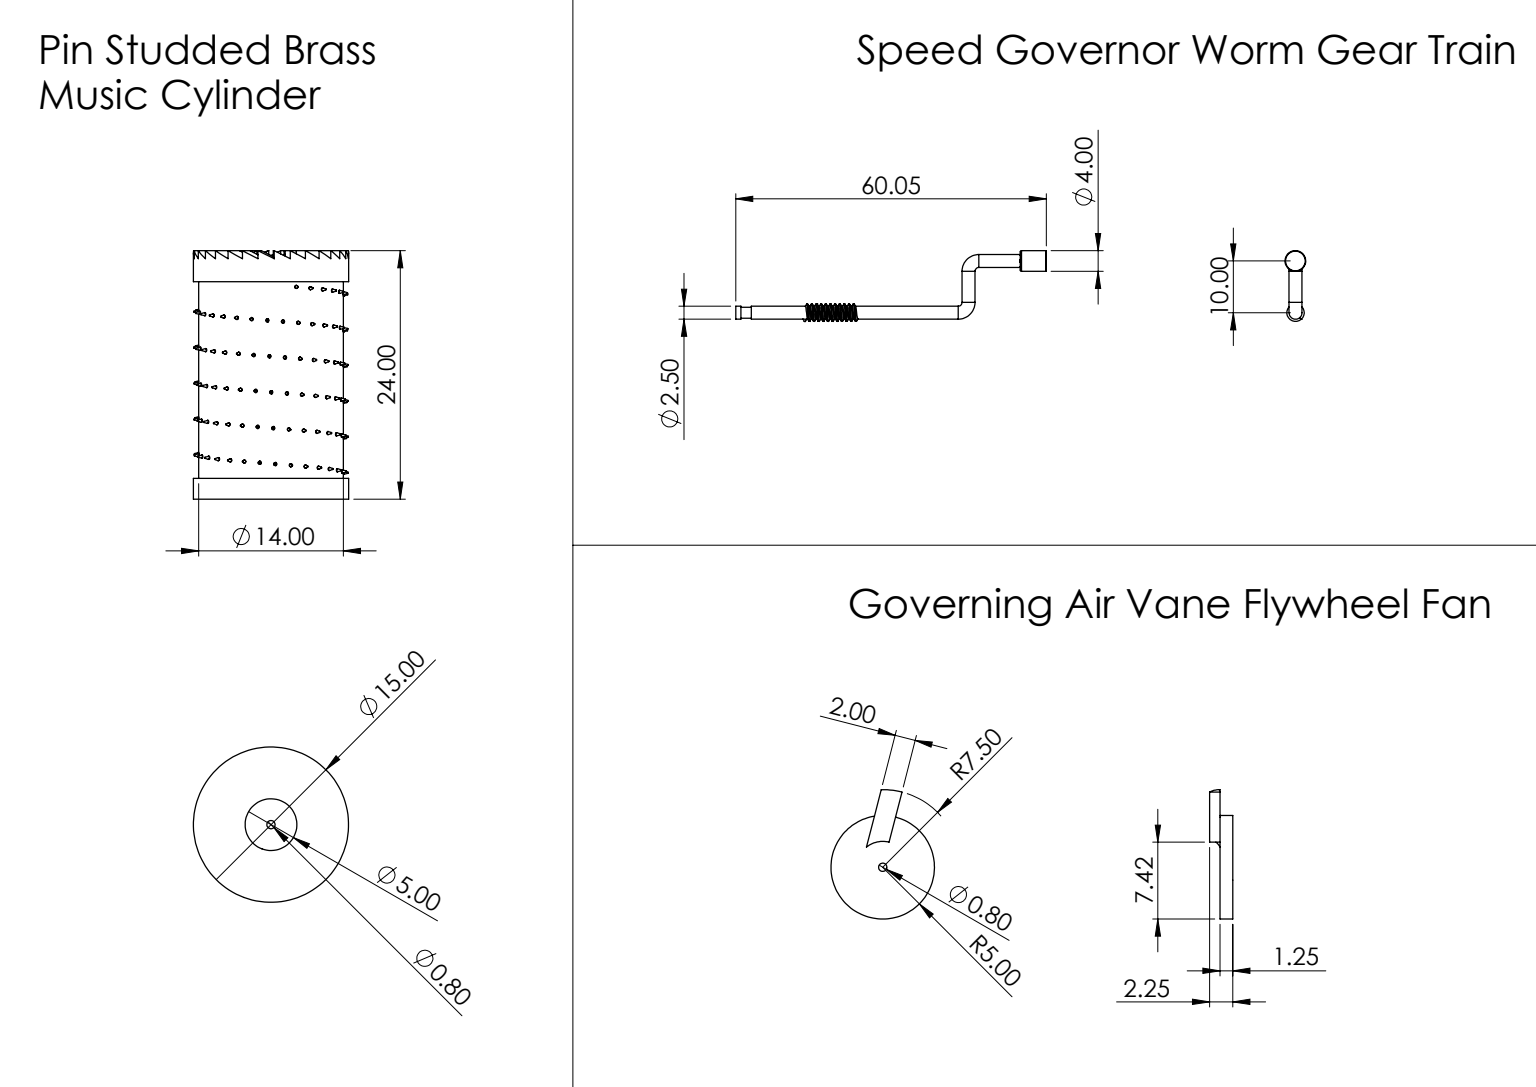
ISO-10303-21;
HEADER;
FILE_DESCRIPTION (('STEP AP214'),
    '1' );
FILE_NAME ('Pin Studded Brass Music Cylinder.step',
    '2026-10-09T09:51:18',
    ( '' ),
    ( '' ),
    'SwSTEP 2.0',
    'SolidWorks 2026',
    '' );
FILE_SCHEMA (( 'AUTOMOTIVE_DESIGN' ));
ENDSEC;

DATA;
#2=ADVANCED_FACE ( 'NONE', ( #22899 ), #34188, .F. ) ;
#3=CARTESIAN_POINT ( 'NONE',  ( -10.03625575236388201, -13.84871804469525891, 57.54850793716612856 ) ) ;
#4=CARTESIAN_POINT ( 'NONE',  ( -11.98370840013613225, -9.620047919863830899, 54.02312124697528617 ) ) ;
#8=ORIENTED_EDGE ( 'NONE', *, *, #40110, .F. ) ;
#9=CARTESIAN_POINT ( 'NONE',  ( -24.74075724160099554, -16.21284971877490122, 62.77824058731629009 ) ) ;
#10=CARTESIAN_POINT ( 'NONE',  ( -15.47038646904106685, -21.58309222549749506, 72.34575460768671462 ) ) ;
#11=CARTESIAN_POINT ( 'NONE',  ( -11.58081676984627073, -10.85831292256293068, 57.30083494179207548 ) ) ;
#13=EDGE_CURVE ( 'NONE', #13987, #23723, #5050, .T. ) ;
#14=VERTEX_POINT ( 'NONE', #21494 ) ;
#15=AXIS2_PLACEMENT_3D ( 'NONE', #40029, #47896, #25252 ) ;
#17=B_SPLINE_CURVE_WITH_KNOTS ( 'NONE', 3,
 ( #43534, #12980, #31711, #43034, #46503, #38613, #46737, #9313, #19907, #1178 ),
 .UNSPECIFIED., .F., .F.,
 ( 4, 2, 2, 2, 4 ),
 ( 0.1272669073658292960, 0.2522669073463885137, 0.3772669073268680728, 0.5022669073073477986, 0.6272669072878274132 ),
 .UNSPECIFIED. ) ;
#18=DIRECTION ( 'NONE',  ( 0.9939059412784551073, 0.1102314832132140626, 5.576311685107536405E-08 ) ) ;
#19=ORIENTED_EDGE ( 'NONE', *, *, #29500, .F. ) ;
#21=CARTESIAN_POINT ( 'NONE',  ( -10.31364510401727053, -17.03300888149450998, 57.80265138661536639 ) ) ;
#22=DIRECTION ( 'NONE',  ( -0.7107718805962432995, -0.7034225854731134264, -7.722840056494082694E-09 ) ) ;
#24=CARTESIAN_POINT ( 'NONE',  ( -21.68606299684865135, -9.256084799238676553, 66.66150029161380530 ) ) ;
#25=VERTEX_POINT ( 'NONE', #6474 ) ;
#26=PLANE ( 'NONE',  #30712 ) ;
#27=FACE_OUTER_BOUND ( 'NONE', #8967, .T. ) ;
#28=VERTEX_POINT ( 'NONE', #28867 ) ;
#30=CARTESIAN_POINT ( 'NONE',  ( -19.85891393954322837, -21.37210614461000091, 75.49999999999994316 ) ) ;
#32=CARTESIAN_POINT ( 'NONE',  ( -20.17268404433175633, -8.371407854712250796, 70.55100341248845552 ) ) ;
#34=CARTESIAN_POINT ( 'NONE',  ( -10.76587051450098542, -16.97017341121004463, 57.68760522235623966 ) ) ;
#36=CARTESIAN_POINT ( 'NONE',  ( -14.44705700679302574, -7.979876293330282699, 63.93978841086359211 ) ) ;
#37=ORIENTED_EDGE ( 'NONE', *, *, #6492, .T. ) ;
#40=LINE ( 'NONE', #15026, #36087 ) ;
#41=DIRECTION ( 'NONE',  ( -0.9942595023566571655, 0.1069955231469581908, -3.800058679842194246E-08 ) ) ;
#43=LINE ( 'NONE', #45603, #5826 ) ;
#46=AXIS2_PLACEMENT_3D ( 'NONE', #24798, #28249, #13682 ) ;
#47=CARTESIAN_POINT ( 'NONE',  ( -16.84904657224188540, -21.78683024590906925, 72.39373074617707005 ) ) ;
#48=CARTESIAN_POINT ( 'NONE',  ( -13.27770768808251134, -9.107454094634595876, 63.90946529206384241 ) ) ;
#50=CARTESIAN_POINT ( 'NONE',  ( -24.00746423591236933, -17.19188279365308603, 73.11165851276361138 ) ) ;
#51=CARTESIAN_POINT ( 'NONE',  ( -24.18314854330451169, -12.98801962294919932, 66.30246782466414857 ) ) ;
#52=CARTESIAN_POINT ( 'NONE',  ( -11.64944166978149909, -18.76574910929434736, 64.81995021385422717 ) ) ;
#53=CARTESIAN_POINT ( 'NONE',  ( -24.72694767484942702, -16.28301260341204326, 62.70833288210281609 ) ) ;
#54=DIRECTION ( 'NONE',  ( 0.5088156898428700670, 0.8608754809899750171, 5.922709712265242817E-08 ) ) ;
#55=CARTESIAN_POINT ( 'NONE',  ( -19.57699614054808634, -21.94144247634149281, 62.17999043330664222 ) ) ;
#57=CARTESIAN_POINT ( 'NONE',  ( -12.74071866071660075, -9.015263582886822391, 70.96429948631303830 ) ) ;
#58=DIRECTION ( 'NONE',  ( 0.5088156898428700670, 0.8608754809899751281, 5.922709712265243479E-08 ) ) ;
#59=CARTESIAN_POINT ( 'NONE',  ( -10.02934067034867915, -15.71522136325494579, 61.14450729704604015 ) ) ;
#60=ORIENTED_EDGE ( 'NONE', *, *, #2656, .T. ) ;
#61=CARTESIAN_POINT ( 'NONE',  ( -10.21764062494887781, -12.91954801228597915, 67.92327636273336111 ) ) ;
#63=VECTOR ( 'NONE', #41726, 1000.000000000000114 ) ;
#67=CARTESIAN_POINT ( 'NONE',  ( -11.89176969907138570, -10.51836715134331079, 74.66715118432504994 ) ) ;
#69=ORIENTED_EDGE ( 'NONE', *, *, #36924, .F. ) ;
#72=EDGE_CURVE ( 'NONE', #44245, #17093, #1589, .T. ) ;
#74=FACE_OUTER_BOUND ( 'NONE', #13777, .T. ) ;
#75=AXIS2_PLACEMENT_3D ( 'NONE', #46607, #16288, #28114 ) ;
#77=CYLINDRICAL_SURFACE ( 'NONE', #4036, 0.1500000000000066835 ) ;
#79=B_SPLINE_CURVE_WITH_KNOTS ( 'NONE', 1,
 ( #16390, #46203 ),
 .UNSPECIFIED., .F., .F.,
 ( 2, 2 ),
 ( 0.000000000000000000, 1.000000000000000000 ),
 .UNSPECIFIED. ) ;
#81=DIRECTION ( 'NONE',  ( 3.549360974555109863E-17, 1.977132801529350715E-16, 1.000000000000000000 ) ) ;
#82=CARTESIAN_POINT ( 'NONE',  ( -18.31357640787765817, -21.80286941108919763, 68.81514702304139064 ) ) ;
#85=PLANE ( 'NONE',  #90 ) ;
#86=CARTESIAN_POINT ( 'NONE',  ( -24.16097951573440383, -12.71927508598556322, 66.51066513624088827 ) ) ;
#87=ORIENTED_EDGE ( 'NONE', *, *, #46598, .F. ) ;
#88=CARTESIAN_POINT ( 'NONE',  ( -22.33685117127641817, -20.40992557423668430, 62.42777465437541196 ) ) ;
#89=EDGE_CURVE ( 'NONE', #5768, #15899, #14150, .T. ) ;
#90=AXIS2_PLACEMENT_3D ( 'NONE', #14327, #11160, #7719 ) ;
#91=CARTESIAN_POINT ( 'NONE',  ( -13.88293259567353743, -20.90532631576516565, 68.45625136994867432 ) ) ;
#92=EDGE_CURVE ( 'NONE', #20698, #38947, #146, .T. ) ;
#95=CARTESIAN_POINT ( 'NONE',  ( -10.02191625022346955, -15.65273779443635327, 61.15293638507743168 ) ) ;
#98=CARTESIAN_POINT ( 'NONE',  ( -10.46033444208452501, -13.68630826424936231, 57.74825279763368968 ) ) ;
#101=CARTESIAN_POINT ( 'NONE',  ( -11.81042834955647258, -10.54382735031610174, 74.45357240259568243 ) ) ;
#103=EDGE_LOOP ( 'NONE', ( #13179, #38410, #7478, #14746, #26186 ) ) ;
#104=CARTESIAN_POINT ( 'NONE',  ( -9.980660856333416930, -14.49625842079804272, 68.05788908589504160 ) ) ;
#106=CARTESIAN_POINT ( 'NONE',  ( -11.75774202113761113, -19.00384077433692909, 71.83685884782747166 ) ) ;
#107=CARTESIAN_POINT ( 'NONE',  ( -18.72484419698154667, -9.451406241145487996, 53.88362224778186516 ) ) ;
#108=CARTESIAN_POINT ( 'NONE',  ( -16.15310590563917970, -7.468295795601643583, 60.37745339520409971 ) ) ;
#109=CARTESIAN_POINT ( 'NONE',  ( -10.49291302059963193, -15.78914242734984263, 64.80771630040662501 ) ) ;
#111=AXIS2_PLACEMENT_3D ( 'NONE', #10985, #396, #26489 ) ;
#113=CARTESIAN_POINT ( 'NONE',  ( -16.59261295876471820, -7.800382739013279831, 60.34461612587266899 ) ) ;
#114=CARTESIAN_POINT ( 'NONE',  ( -14.54391382047218784, -7.937654553327920581, 63.97634087063163122 ) ) ;
#117=DIRECTION ( 'NONE',  ( 3.549360974554993999E-17, -6.371834667797928663E-18, -1.000000000000000000 ) ) ;
#119=( BOUNDED_CURVE ( )  B_SPLINE_CURVE ( 3, ( #27341, #33989, #3973, #288 ),
 .UNSPECIFIED., .F., .F. ) 
 B_SPLINE_CURVE_WITH_KNOTS ( ( 4, 4 ),
 ( 0.000000000000000000, 0.4074455897393676196 ),
 .UNSPECIFIED. ) 
 CURVE ( )  GEOMETRIC_REPRESENTATION_ITEM ( )  RATIONAL_B_SPLINE_CURVE ( ( 1.000000000000000000, 0.4567392136813337444, 0.3561768502900309330, 0.6983129098260915102 ) ) 
 REPRESENTATION_ITEM ( '' )  );
#120=ORIENTED_EDGE ( 'NONE', *, *, #48681, .F. ) ;
#121=( BOUNDED_SURFACE ( )  B_SPLINE_SURFACE ( 3, 1, ( 
 ( #32470, #2427 ),
 ( #20663, #20424 ),
 ( #39116, #24112 ),
 ( #35421, #5884 ),
 ( #1706, #35896 ),
 ( #28292, #43320 ),
 ( #17438, #47493 ) ),
 .UNSPECIFIED., .T., .F., .F. ) 
 B_SPLINE_SURFACE_WITH_KNOTS ( ( 4, 3, 4 ),
 ( 2, 2 ),
 ( 0.000000000000000000, 0.5000000000000000000, 1.000000000000000000 ),
 ( 0.000000000000000000, 1.000000000000000000 ),
 .UNSPECIFIED. ) 
 GEOMETRIC_REPRESENTATION_ITEM ( )  RATIONAL_B_SPLINE_SURFACE ( (
 ( 1.000000000000000000, 1.000000000000000000),
 ( 0.3333333333333335369, 0.3333333333333330373),
 ( 0.3333333333333335369, 0.3333333333333330373),
 ( 1.000000000000000000, 1.000000000000000000),
 ( 0.3333333333333333703, 0.3333333333333333703),
 ( 0.3333333333333333703, 0.3333333333333333703),
 ( 1.000000000000000000, 1.000000000000000000) ) ) 
 REPRESENTATION_ITEM ( '' )  SURFACE ( )  );
#122=DIRECTION ( 'NONE',  ( 0.06306825763707678278, -0.9980092158285026605, -2.415158932408153704E-08 ) ) ;
#125=EDGE_LOOP ( 'NONE', ( #26058, #18123, #34416, #18514, #29920 ) ) ;
#128=CARTESIAN_POINT ( 'NONE',  ( -14.34311167289324196, -8.523215816031258996, 71.01341051612104138 ) ) ;
#133=( BOUNDED_CURVE ( )  B_SPLINE_CURVE ( 3, ( #21288, #36284, #8992, #43458 ),
 .UNSPECIFIED., .F., .F. ) 
 B_SPLINE_CURVE_WITH_KNOTS ( ( 4, 4 ),
 ( 0.000000000000000000, 0.4074455897393643999 ),
 .UNSPECIFIED. ) 
 CURVE ( )  GEOMETRIC_REPRESENTATION_ITEM ( )  RATIONAL_B_SPLINE_CURVE ( ( 1.000000000000000000, 0.4567392136813379078, 0.3561768502900324873, 0.6983129098260837386 ) ) 
 REPRESENTATION_ITEM ( '' )  );
#134=ORIENTED_EDGE ( 'NONE', *, *, #4016, .F. ) ;
#137=ADVANCED_FACE ( 'NONE', ( #48154 ), #33338, .T. ) ;
#138=B_SPLINE_CURVE_WITH_KNOTS ( 'NONE', 1,
 ( #27125, #38191 ),
 .UNSPECIFIED., .F., .F.,
 ( 2, 2 ),
 ( 0.000000000000000000, 1.000000000000000000 ),
 .UNSPECIFIED. ) ;
#139=CARTESIAN_POINT ( 'NONE',  ( -10.44538189632046787, -14.26369805489357212, 61.02707267863189600 ) ) ;
#143=ORIENTED_EDGE ( 'NONE', *, *, #11819, .T. ) ;
#144=CARTESIAN_POINT ( 'NONE',  ( -15.46105799208929454, -21.99670631207736449, 72.15920124769014876 ) ) ;
#146=B_SPLINE_CURVE_WITH_KNOTS ( 'NONE', 3,
 ( #35431, #29443, #1718, #7046, #39128, #9108, #29205, #44244, #25744, #48389 ),
 .UNSPECIFIED., .F., .F.,
 ( 4, 2, 2, 2, 4 ),
 ( 0.000000000000000000, 0.2500000000000000000, 0.5000000000000000000, 0.7500000000000000000, 1.000000000000000000 ),
 .UNSPECIFIED. ) ;
#147=CARTESIAN_POINT ( 'NONE',  ( -23.80321451250838649, -17.81075939459467961, 59.00378417737415049 ) ) ;
#148=EDGE_LOOP ( 'NONE', ( #25559, #28549, #5036, #6443 ) ) ;
#149=DIRECTION ( 'NONE',  ( 0.3478314405900310158, 0.9375570856950865561, -9.567072274253695189E-17 ) ) ;
#150=EDGE_CURVE ( 'NONE', #31901, #23884, #35863, .T. ) ;
#153=CARTESIAN_POINT ( 'NONE',  ( -21.39967327233876304, -20.63170314183283693, 72.80974286114339122 ) ) ;
#154=CARTESIAN_POINT ( 'NONE',  ( -24.83423444544265379, -14.03910623769390220, 73.31609816701728732 ) ) ;
#157=ADVANCED_FACE ( 'NONE', ( #22300 ), #19091, .T. ) ;
#158=CARTESIAN_POINT ( 'NONE',  ( -11.08846142298070880, -18.82290330472913098, 53.49999999999994316 ) ) ;
#160=VECTOR ( 'NONE', #789, 1000.000000000000227 ) ;
#161=ORIENTED_EDGE ( 'NONE', *, *, #28229, .T. ) ;
#162=CARTESIAN_POINT ( 'NONE',  ( -10.40121522062585591, -17.29573862802152817, 61.20097198354311274 ) ) ;
#163=CARTESIAN_POINT ( 'NONE',  ( -24.09124995986085338, -12.51712822272146042, 73.53665784698486618 ) ) ;
#164=CARTESIAN_POINT ( 'NONE',  ( -23.56138404952065457, -11.33988834032952830, 70.19210750372964469 ) ) ;
#165=CYLINDRICAL_SURFACE ( 'NONE', #41008, 0.1500000000000034084 ) ;
#166=VERTEX_POINT ( 'NONE', #48638 ) ;
#168=CARTESIAN_POINT ( 'NONE',  ( -13.14998806103231566, -9.265559761403904915, 67.67942786032521951 ) ) ;
#170=FACE_BOUND ( 'NONE', #41683, .T. ) ;
#171=ORIENTED_EDGE ( 'NONE', *, *, #31245, .F. ) ;
#173=CARTESIAN_POINT ( 'NONE',  ( -15.68784259522275981, -9.576290808195315307, 53.69233794759168887 ) ) ;
#174=CARTESIAN_POINT ( 'NONE',  ( -9.939267784769082681, -14.33236412611010913, 54.27966884056655061 ) ) ;
#175=CARTESIAN_POINT ( 'NONE',  ( -21.55884032038934350, -8.611816057827914150, 73.78624026056009200 ) ) ;
#178=ORIENTED_EDGE ( 'NONE', *, *, #7182, .F. ) ;
#179=CARTESIAN_POINT ( 'NONE',  ( -12.18170095131842068, -10.17053037870675780, 64.02914326641410980 ) ) ;
#181=B_SPLINE_CURVE_WITH_KNOTS ( 'NONE', 1,
 ( #24932, #10158 ),
 .UNSPECIFIED., .F., .F.,
 ( 2, 2 ),
 ( 0.000000000000000000, 1.000000000000000000 ),
 .UNSPECIFIED. ) ;
#183=ORIENTED_EDGE ( 'NONE', *, *, #25838, .F. ) ;
#188=VERTEX_POINT ( 'NONE', #389 ) ;
#189=CARTESIAN_POINT ( 'NONE',  ( -15.39235221195410652, -21.97689038623625635, 72.08929527613493349 ) ) ;
#190=FACE_OUTER_BOUND ( 'NONE', #18555, .T. ) ;
#191=CARTESIAN_POINT ( 'NONE',  ( -24.42668993457695592, -13.99045928592870780, 73.40799407547365263 ) ) ;
#192=CARTESIAN_POINT ( 'NONE',  ( -11.32469211327616065, -18.34471187850051166, 57.95714594245092854 ) ) ;
#193=FACE_OUTER_BOUND ( 'NONE', #16201, .T. ) ;
#194=CARTESIAN_POINT ( 'NONE',  ( -14.55015457993596328, -8.362855509585410019, 70.87390454733632339 ) ) ;
#195=CARTESIAN_POINT ( 'NONE',  ( -15.34465393633500518, -21.54586957516256263, 68.86120835375241711 ) ) ;
#196=EDGE_LOOP ( 'NONE', ( #10385, #20529 ) ) ;
#197=ORIENTED_EDGE ( 'NONE', *, *, #3825, .F. ) ;
#198=CARTESIAN_POINT ( 'NONE',  ( -16.19792114999740562, -7.866354181730329742, 60.48556343814865954 ) ) ;
#199=B_SPLINE_CURVE_WITH_KNOTS ( 'NONE', 3,
 ( #36213, #17003, #17258, #47556, #32053, #25388, #10127, #47073, #46828, #2496 ),
 .UNSPECIFIED., .F., .F.,
 ( 4, 2, 2, 2, 4 ),
 ( 0.000000000000000000, 0.2500000000000000000, 0.5000000000000000000, 0.7500000000000000000, 1.000000000000000000 ),
 .UNSPECIFIED. ) ;
#201=EDGE_CURVE ( 'NONE', #20782, #44291, #26002, .T. ) ;
#202=CARTESIAN_POINT ( 'NONE',  ( -22.54212894027171643, -20.22308674935842276, 65.88138641420671604 ) ) ;
#204=CARTESIAN_POINT ( 'NONE',  ( -21.56183007311343758, -9.162502203718322136, 70.41516033260253948 ) ) ;
#207=ORIENTED_EDGE ( 'NONE', *, *, #41740, .T. ) ;
#210=DIRECTION ( 'NONE',  ( 0.2196488028684550897, 0.9755790093059856227, -7.835600157377411709E-08 ) ) ;
#211=( BOUNDED_SURFACE ( )  B_SPLINE_SURFACE ( 3, 1, ( 
 ( #3331, #29681 ),
 ( #37286, #39375 ),
 ( #13247, #28301 ),
 ( #9599, #24612 ),
 ( #39614, #20905 ),
 ( #29932, #18842 ),
 ( #11449, #11220 ) ),
 .UNSPECIFIED., .T., .F., .F. ) 
 B_SPLINE_SURFACE_WITH_KNOTS ( ( 4, 3, 4 ),
 ( 2, 2 ),
 ( 0.000000000000000000, 0.5000000000000000000, 1.000000000000000000 ),
 ( 0.000000000000000000, 1.000000000000000000 ),
 .UNSPECIFIED. ) 
 GEOMETRIC_REPRESENTATION_ITEM ( )  RATIONAL_B_SPLINE_SURFACE ( (
 ( 1.000000000000000000, 1.000000000000000000),
 ( 0.3333333333333335369, 0.3333333333333330373),
 ( 0.3333333333333335369, 0.3333333333333330373),
 ( 1.000000000000000000, 1.000000000000000000),
 ( 0.3333333333333333703, 0.3333333333333333703),
 ( 0.3333333333333333703, 0.3333333333333333703),
 ( 1.000000000000000000, 1.000000000000000000) ) ) 
 REPRESENTATION_ITEM ( '' )  SURFACE ( )  );
#212=ORIENTED_EDGE ( 'NONE', *, *, #4432, .T. ) ;
#213=B_SPLINE_CURVE_WITH_KNOTS ( 'NONE', 1,
 ( #33678, #3925 ),
 .UNSPECIFIED., .F., .F.,
 ( 2, 2 ),
 ( 0.000000000000000000, 1.000000000000000000 ),
 .UNSPECIFIED. ) ;
#214=CYLINDRICAL_SURFACE ( 'NONE', #2262, 0.1500000000000026867 ) ;
#215=CARTESIAN_POINT ( 'NONE',  ( -10.49912617938483628, -17.55847672437320028, 64.74084113084838066 ) ) ;
#216=EDGE_CURVE ( 'NONE', #42645, #18548, #11212, .T. ) ;
#218=EDGE_LOOP ( 'NONE', ( #34553, #46126, #27909, #171, #16080 ) ) ;
#219=DIRECTION ( 'NONE',  ( -0.03181436478788690625, -0.9994937949748078365, -6.982004198809110323E-09 ) ) ;
#220=CARTESIAN_POINT ( 'NONE',  ( -10.13411916705081950, -16.34564720852668884, 71.62467237673240561 ) ) ;
#221=CARTESIAN_POINT ( 'NONE',  ( -9.974215857974789046, -14.86484893678357544, 74.91283499353951925 ) ) ;
#223=CARTESIAN_POINT ( 'NONE',  ( -24.67958393122153282, -16.50120980550295613, 59.26299101463538221 ) ) ;
#225=CARTESIAN_POINT ( 'NONE',  ( -10.33531725737393181, -17.10115422170377641, 57.87255955594724810 ) ) ;
#227=EDGE_CURVE ( 'NONE', #31196, #14322, #2991, .T. ) ;
#228=DIRECTION ( 'NONE',  ( -0.8743548079231423520, -0.4852872034802501178, 5.778319183281970132E-08 ) ) ;
#230=CARTESIAN_POINT ( 'NONE',  ( -23.84087120742880117, -12.00869232914290841, 59.55405921996587892 ) ) ;
#231=EDGE_CURVE ( 'NONE', #5198, #11939, #41252, .T. ) ;
#232=CARTESIAN_POINT ( 'NONE',  ( -20.59081119662036485, -8.510278447070987795, 63.31681297810601450 ) ) ;
#234=CARTESIAN_POINT ( 'NONE',  ( -17.85728874018076340, -21.84618329174708151, 61.89007996730683203 ) ) ;
#235=CARTESIAN_POINT ( 'NONE',  ( -22.25933006198147623, -19.87095799428289666, 65.71924198175659626 ) ) ;
#236=LINE ( 'NONE', #3923, #40839 ) ;
#238=CARTESIAN_POINT ( 'NONE',  ( -24.03160980685186487, -17.26750534774173929, 69.41339792588560442 ) ) ;
#239=CARTESIAN_POINT ( 'NONE',  ( -20.81693178527791943, -20.99322608020143477, 65.67634157851000509 ) ) ;
#240=EDGE_CURVE ( 'NONE', #21614, #9195, #13538, .T. ) ;
#243=CARTESIAN_POINT ( 'NONE',  ( -10.49020387924836761, -15.76942919235743013, 61.26462351667871076 ) ) ;
#245=CARTESIAN_POINT ( 'NONE',  ( -19.86569447268030686, -19.73755174630646536, 54.07175714974878389 ) ) ;
#248=CARTESIAN_POINT ( 'NONE',  ( -24.42668993457695592, -13.99045928592870958, 73.40799407547365263 ) ) ;
#249=CARTESIAN_POINT ( 'NONE',  ( -11.10300703817161327, -10.86615712478015539, 57.39398594787093089 ) ) ;
#250=CARTESIAN_POINT ( 'NONE',  ( -20.50783493979771421, -8.027295371342848540, 66.96599508560271374 ) ) ;
#251=CARTESIAN_POINT ( 'NONE',  ( -9.974485213446937948, -14.88680260109476805, 74.89804658166208640 ) ) ;
#253=B_SPLINE_CURVE_WITH_KNOTS ( 'NONE', 3,
 ( #32293, #44346, #6180, #32750, #21450, #2715, #14493, #36434, #43618, #13547 ),
 .UNSPECIFIED., .F., .F.,
 ( 4, 2, 2, 2, 4 ),
 ( 0.6272669072877669061, 0.7522669073072844048, 0.8772669073268017925, 1.002266907346319291, 1.127266907365836790 ),
 .UNSPECIFIED. ) ;
#254=DIRECTION ( 'NONE',  ( -0.5022914217388750879, 0.8646984027090224290, 6.766381827299039861E-08 ) ) ;
#255=VECTOR ( 'NONE', #23047, 1000.000000000000000 ) ;
#256=CARTESIAN_POINT ( 'NONE',  ( -10.44916039635137039, -15.83526825291551177, 64.50771589744864798 ) ) ;
#257=FACE_OUTER_BOUND ( 'NONE', #41727, .T. ) ;
#258=( BOUNDED_SURFACE ( )  B_SPLINE_SURFACE ( 3, 1, ( 
 ( #12645, #30891 ),
 ( #19547, #27669 ),
 ( #35286, #42701 ),
 ( #8965, #19806 ),
 ( #23985, #34558 ),
 ( #34807, #16808 ),
 ( #38986, #27907 ) ),
 .UNSPECIFIED., .T., .F., .F. ) 
 B_SPLINE_SURFACE_WITH_KNOTS ( ( 4, 3, 4 ),
 ( 2, 2 ),
 ( 0.000000000000000000, 0.5000000000000000000, 1.000000000000000000 ),
 ( 0.000000000000000000, 1.000000000000000000 ),
 .UNSPECIFIED. ) 
 GEOMETRIC_REPRESENTATION_ITEM ( )  RATIONAL_B_SPLINE_SURFACE ( (
 ( 1.000000000000000000, 1.000000000000000000),
 ( 0.3333333333333335369, 0.3333333333333330373),
 ( 0.3333333333333335369, 0.3333333333333330373),
 ( 1.000000000000000000, 1.000000000000000000),
 ( 0.3333333333333333703, 0.3333333333333333703),
 ( 0.3333333333333333703, 0.3333333333333333703),
 ( 1.000000000000000000, 1.000000000000000000) ) ) 
 REPRESENTATION_ITEM ( '' )  SURFACE ( )  );
#259=EDGE_LOOP ( 'NONE', ( #11996, #26220, #36249, #37738, #32112 ) ) ;
#260=VERTEX_POINT ( 'NONE', #11960 ) ;
#263=DIRECTION ( 'NONE',  ( 0.8398192074808117358, 0.5428661886195298436, 7.907900705247678986E-08 ) ) ;
#264=FACE_OUTER_BOUND ( 'NONE', #3313, .T. ) ;
#265=ADVANCED_FACE ( 'NONE', ( #8266 ), #28714, .T. ) ;
#266=EDGE_LOOP ( 'NONE', ( #5129, #25117, #30541, #44712, #25689 ) ) ;
#267=( BOUNDED_SURFACE ( )  B_SPLINE_SURFACE ( 3, 1, ( 
 ( #4799, #23276 ),
 ( #30184, #27440 ),
 ( #41983, #42225 ),
 ( #11696, #4317 ),
 ( #23767, #8256 ),
 ( #38762, #38256 ),
 ( #19824, #20056 ) ),
 .UNSPECIFIED., .T., .F., .F. ) 
 B_SPLINE_SURFACE_WITH_KNOTS ( ( 4, 3, 4 ),
 ( 2, 2 ),
 ( 0.000000000000000000, 0.5000000000000000000, 1.000000000000000000 ),
 ( 0.000000000000000000, 1.000000000000000000 ),
 .UNSPECIFIED. ) 
 GEOMETRIC_REPRESENTATION_ITEM ( )  RATIONAL_B_SPLINE_SURFACE ( (
 ( 1.000000000000000000, 1.000000000000000000),
 ( 0.3333333333333335369, 0.3333333333333330373),
 ( 0.3333333333333335369, 0.3333333333333330373),
 ( 1.000000000000000000, 1.000000000000000000),
 ( 0.3333333333333333703, 0.3333333333333333703),
 ( 0.3333333333333333703, 0.3333333333333333703),
 ( 1.000000000000000000, 1.000000000000000000) ) ) 
 REPRESENTATION_ITEM ( '' )  SURFACE ( )  );
#268=CARTESIAN_POINT ( 'NONE',  ( -23.54782545260626136, -11.41793123268749532, 66.49502567849339130 ) ) ;
#269=CARTESIAN_POINT ( 'NONE',  ( -14.16114181629738589, -8.110937519819053421, 67.37319822901852717 ) ) ;
#270=EDGE_CURVE ( 'NONE', #48679, #8571, #43948, .T. ) ;
#272=CARTESIAN_POINT ( 'NONE',  ( -22.79960313759534074, -9.650943445293346912, 73.66656413195866548 ) ) ;
#273=CARTESIAN_POINT ( 'NONE',  ( -10.88209246082447912, -17.29963176008448400, 64.92739380462948873 ) ) ;
#274=ORIENTED_EDGE ( 'NONE', *, *, #1986, .F. ) ;
#275=CARTESIAN_POINT ( 'NONE',  ( -17.53144753494939323, -7.808750373834428160, 67.24869371032770005 ) ) ;
#276=ORIENTED_EDGE ( 'NONE', *, *, #38105, .F. ) ;
#277=ADVANCED_FACE ( 'NONE', ( #22486 ), #33722, .T. ) ;
#278=CARTESIAN_POINT ( 'NONE',  ( -22.73317970229575025, -20.03675580610048712, 72.83055794290764595 ) ) ;
#279=CARTESIAN_POINT ( 'NONE',  ( -11.10386160987148862, -10.86480171160796893, 57.25257256893876701 ) ) ;
#280=ORIENTED_EDGE ( 'NONE', *, *, #26061, .T. ) ;
#282=CARTESIAN_POINT ( 'NONE',  ( -10.40830226666251157, -14.07974499963562920, 64.47983968490285633 ) ) ;
#283=ADVANCED_FACE ( 'NONE', ( #26188 ), #36999, .T. ) ;
#285=CARTESIAN_POINT ( 'NONE',  ( -10.37840828709523322, -12.38598989307629061, 60.98508858522948373 ) ) ;
#287=PLANE ( 'NONE',  #36864 ) ;
#288=CARTESIAN_POINT ( 'NONE',  ( -10.48067290732983281, -16.03043740265091444, 67.97767830707738312 ) ) ;
#290=ORIENTED_EDGE ( 'NONE', *, *, #4920, .T. ) ;
#292=CARTESIAN_POINT ( 'NONE',  ( -13.12613471901881113, -20.89454346209081947, 58.16154795605982031 ) ) ;
#293=CARTESIAN_POINT ( 'NONE',  ( -23.48344415125163565, -18.41350569598871090, 73.04896097104848707 ) ) ;
#295=CARTESIAN_POINT ( 'NONE',  ( -24.20309392561631512, -13.06392267828124432, 63.11798765125330135 ) ) ;
#298=CARTESIAN_POINT ( 'NONE',  ( -16.94342153774571713, -21.79279417793566154, 72.16543237156788848 ) ) ;
#299=DIRECTION ( 'NONE',  ( 0.3636930986378153485, 0.9315188296557532777, -1.850371886801397451E-09 ) ) ;
#300=VERTEX_POINT ( 'NONE', #7486 ) ;
#301=CARTESIAN_POINT ( 'NONE',  ( -10.40860991809309155, -15.50898095412354571, 57.85320721669017985 ) ) ;
#302=CARTESIAN_POINT ( 'NONE',  ( -14.96339028783852676, -21.42433367428847291, 68.72025781230657060 ) ) ;
#303=CARTESIAN_POINT ( 'NONE',  ( -15.53265176333180619, -21.60105060138385014, 72.33103357390284316 ) ) ;
#304=CARTESIAN_POINT ( 'NONE',  ( -17.20139284005516700, -7.812749994621428051, 70.79035839633094440 ) ) ;
#305=EDGE_CURVE ( 'NONE', #24134, #2153, #45318, .T. ) ;
#306=CARTESIAN_POINT ( 'NONE',  ( -21.54495561387301450, -21.01579894740183363, 72.63172296156072605 ) ) ;
#308=CARTESIAN_POINT ( 'NONE',  ( -24.64621740481133116, -16.83181165628401033, 53.49999999999994316 ) ) ;
#311=DIRECTION ( 'NONE',  ( 0.9000732436326450703, 0.4357386327795698677, -2.072980810833656879E-08 ) ) ;
#313=VERTEX_POINT ( 'NONE', #41198 ) ;
#314=ORIENTED_EDGE ( 'NONE', *, *, #26794, .T. ) ;
#317=FACE_OUTER_BOUND ( 'NONE', #17345, .T. ) ;
#319=CARTESIAN_POINT ( 'NONE',  ( -14.41428173599358331, -7.994163662063686893, 63.97474278339937115 ) ) ;
#320=EDGE_CURVE ( 'NONE', #35558, #5311, #25190, .T. ) ;
#321=CARTESIAN_POINT ( 'NONE',  ( -13.54823245630065998, -20.69819609872913801, 61.81646323537676579 ) ) ;
#322=CARTESIAN_POINT ( 'NONE',  ( -16.10183008998876275, -22.14097689426727911, 58.47923897578370145 ) ) ;
#324=CARTESIAN_POINT ( 'NONE',  ( -15.94298218261998912, -7.507746547262916792, 63.83044349608796608 ) ) ;
#325=DIRECTION ( 'NONE',  ( -5.255974128148611414E-06, 1.684062796621483993E-06, 0.9999999999847694054 ) ) ;
#327=CARTESIAN_POINT ( 'NONE',  ( -11.49500183448702906, -10.99442376238782515, 57.22375354680192316 ) ) ;
#328=CARTESIAN_POINT ( 'NONE',  ( -23.97105477456146261, -17.28687578273886061, 69.41339789080815592 ) ) ;
#329=EDGE_LOOP ( 'NONE', ( #13838, #9851, #9267, #15936, #24444 ) ) ;
#330=CARTESIAN_POINT ( 'NONE',  ( -11.12758687547136383, -10.82717111148205547, 57.40914419403284086 ) ) ;
#331=CARTESIAN_POINT ( 'NONE',  ( -21.30368986256526043, -21.17021271237730318, 69.24105570176159574 ) ) ;
#332=B_SPLINE_CURVE_WITH_KNOTS ( 'NONE', 3,
 ( #32504, #47759, #36419, #3183, #39890, #36180, #13765, #28808, #48006, #29048 ),
 .UNSPECIFIED., .F., .F.,
 ( 4, 2, 2, 2, 4 ),
 ( 0.1272669073658393157, 0.2522669073463362222, 0.3772669073268331008, 0.5022669073073300350, 0.6272669072878269692 ),
 .UNSPECIFIED. ) ;
#334=ORIENTED_EDGE ( 'NONE', *, *, #2116, .T. ) ;
#335=CARTESIAN_POINT ( 'NONE',  ( -19.71243508403738076, -21.42506817177905631, 69.21865898670732520 ) ) ;
#336=EDGE_CURVE ( 'NONE', #12470, #9257, #14096, .T. ) ;
#337=CARTESIAN_POINT ( 'NONE',  ( -23.00442008925061899, -19.11762375203660724, 59.18410642057862248 ) ) ;
#338=ADVANCED_FACE ( 'NONE', ( #40464 ), #45710, .T. ) ;
#340=CARTESIAN_POINT ( 'NONE',  ( -10.93232766038821424, -17.55941949638709687, 68.38249893951126523 ) ) ;
#342=CARTESIAN_POINT ( 'NONE',  ( -14.78766009005058635, -21.34800739930362568, 58.45145834864037937 ) ) ;
#344=CARTESIAN_POINT ( 'NONE',  ( -23.52687218415512760, -18.35477548540580273, 69.44938804596051796 ) ) ;
#345=CARTESIAN_POINT ( 'NONE',  ( -23.93414946104399377, -11.18647762192129314, 70.05357276016361823 ) ) ;
#346=AXIS2_PLACEMENT_3D ( 'NONE', #48605, #22512, #26210 ) ;
#351=ORIENTED_EDGE ( 'NONE', *, *, #40500, .T. ) ;
#352=CARTESIAN_POINT ( 'NONE',  ( -23.66133310609451712, -18.88359296917171903, 69.40876596050124192 ) ) ;
#354=ORIENTED_EDGE ( 'NONE', *, *, #17755, .F. ) ;
#355=CARTESIAN_POINT ( 'NONE',  ( -22.36289160583321944, -19.84024478656301937, 69.17417986619062731 ) ) ;
#356=CARTESIAN_POINT ( 'NONE',  ( -24.45810293133404656, -14.28236561102681534, 73.42271650780452319 ) ) ;
#357=CARTESIAN_POINT ( 'NONE',  ( -10.37762151648083808, -12.38827872426728050, 57.44202070861023657 ) ) ;
#359=ORIENTED_EDGE ( 'NONE', *, *, #35784, .F. ) ;
#361=CARTESIAN_POINT ( 'NONE',  ( -10.37534642380570027, -14.67419306300129733, 71.32782691282784526 ) ) ;
#362=CARTESIAN_POINT ( 'NONE',  ( -10.05862335131466700, -15.92885902279982524, 64.69266873560974318 ) ) ;
#363=CARTESIAN_POINT ( 'NONE',  ( -18.41375667457423759, -22.19335022249702050, 68.97548045702603758 ) ) ;
#364=EDGE_LOOP ( 'NONE', ( #29959, #8982, #8125, #35145, #33682 ) ) ;
#366=CARTESIAN_POINT ( 'NONE',  ( -11.64235247690698927, -18.84330696305777764, 68.51689631558762983 ) ) ;
#367=CARTESIAN_POINT ( 'NONE',  ( -24.80769062643263467, -15.80232089486973557, 69.71802876059763321 ) ) ;
#368=CARTESIAN_POINT ( 'NONE',  ( -21.95692851765875631, -9.409391401937881483, 60.01611433801762985 ) ) ;
#377=LINE ( 'NONE', #48205, #37863 ) ;
#378=CARTESIAN_POINT ( 'NONE',  ( -10.25416474409032652, -12.78293385988982678, 67.92487701448251869 ) ) ;
#382=( BOUNDED_SURFACE ( )  B_SPLINE_SURFACE ( 3, 1, ( 
 ( #13535, #28583 ),
 ( #23695, #17952 ),
 ( #6413, #44567 ),
 ( #40381, #25848 ),
 ( #9867, #14250 ),
 ( #43853, #25598 ),
 ( #24883, #43609 ) ),
 .UNSPECIFIED., .T., .F., .F. ) 
 B_SPLINE_SURFACE_WITH_KNOTS ( ( 4, 3, 4 ),
 ( 2, 2 ),
 ( 0.000000000000000000, 0.5000000000000000000, 1.000000000000000000 ),
 ( 0.000000000000000000, 1.000000000000000000 ),
 .UNSPECIFIED. ) 
 GEOMETRIC_REPRESENTATION_ITEM ( )  RATIONAL_B_SPLINE_SURFACE ( (
 ( 1.000000000000000000, 1.000000000000000000),
 ( 0.3333333333333335369, 0.3333333333333330373),
 ( 0.3333333333333335369, 0.3333333333333330373),
 ( 1.000000000000000000, 1.000000000000000000),
 ( 0.3333333333333333703, 0.3333333333333333703),
 ( 0.3333333333333333703, 0.3333333333333333703),
 ( 1.000000000000000000, 1.000000000000000000) ) ) 
 REPRESENTATION_ITEM ( '' )  SURFACE ( )  );
#383=VERTEX_POINT ( 'NONE', #19774 ) ;
#384=CARTESIAN_POINT ( 'NONE',  ( -23.03651728895758666, -18.99332342978600252, 62.63790370423207321 ) ) ;
#385=EDGE_CURVE ( 'NONE', #1629, #41284, #30866, .T. ) ;
#386=ORIENTED_EDGE ( 'NONE', *, *, #34512, .T. ) ;
#387=CARTESIAN_POINT ( 'NONE',  ( -13.33011785382929126, -9.069340661520646663, 63.92418669539090814 ) ) ;
#388=CARTESIAN_POINT ( 'NONE',  ( -23.42532328873747005, -19.22384396101403681, 62.46911485589509994 ) ) ;
#389=CARTESIAN_POINT ( 'NONE',  ( -19.22579631480732587, -21.57336711704104104, 58.82507384991394872 ) ) ;
#392=CARTESIAN_POINT ( 'NONE',  ( -17.98584054083101691, -22.23808389992613499, 62.06031238270200845 ) ) ;
#393=DIRECTION ( 'NONE',  ( 0.9372362738803844406, 0.3486949482324239735, -5.386914174890154601E-09 ) ) ;
#394=( BOUNDED_CURVE ( )  B_SPLINE_CURVE ( 3, ( #3848, #18104, #7543, #37546 ),
 .UNSPECIFIED., .F., .F. ) 
 B_SPLINE_CURVE_WITH_KNOTS ( ( 4, 4 ),
 ( 0.9074455897393690629, 1.000000000000000000 ),
 .UNSPECIFIED. ) 
 CURVE ( )  GEOMETRIC_REPRESENTATION_ITEM ( )  RATIONAL_B_SPLINE_CURVE ( ( 0.6983129098260929535, 0.7760317562606982023, 0.8765941196520005141, 1.000000000000000000 ) ) 
 REPRESENTATION_ITEM ( '' )  );
#395=CARTESIAN_POINT ( 'NONE',  ( -14.09914643654217947, -8.649277595337252933, 74.49954655170296292 ) ) ;
#396=DIRECTION ( 'NONE',  ( -0.9000732436326450703, -0.4357386327795698677, 2.072980810273451787E-08 ) ) ;
#397=ORIENTED_EDGE ( 'NONE', *, *, #17162, .F. ) ;
#398=FACE_OUTER_BOUND ( 'NONE', #46859, .T. ) ;
#399=CARTESIAN_POINT ( 'NONE',  ( -10.90759844528708911, -17.49952021360972765, 68.24721944423116327 ) ) ;
#400=( BOUNDED_SURFACE ( )  B_SPLINE_SURFACE ( 3, 1, ( 
 ( #20895, #24356 ),
 ( #27793, #42821 ),
 ( #39365, #5650 ),
 ( #4919, #20658 ),
 ( #35890, #2171 ),
 ( #13488, #43558 ),
 ( #34933, #1199 ) ),
 .UNSPECIFIED., .T., .F., .F. ) 
 B_SPLINE_SURFACE_WITH_KNOTS ( ( 4, 3, 4 ),
 ( 2, 2 ),
 ( 0.000000000000000000, 0.5000000000000000000, 1.000000000000000000 ),
 ( 0.000000000000000000, 1.000000000000000000 ),
 .UNSPECIFIED. ) 
 GEOMETRIC_REPRESENTATION_ITEM ( )  RATIONAL_B_SPLINE_SURFACE ( (
 ( 1.000000000000000000, 1.000000000000000000),
 ( 0.3333333333333335369, 0.3333333333333330373),
 ( 0.3333333333333335369, 0.3333333333333330373),
 ( 1.000000000000000000, 1.000000000000000000),
 ( 0.3333333333333333703, 0.3333333333333333703),
 ( 0.3333333333333333703, 0.3333333333333333703),
 ( 1.000000000000000000, 1.000000000000000000) ) ) 
 REPRESENTATION_ITEM ( '' )  SURFACE ( )  );
#401=CARTESIAN_POINT ( 'NONE',  ( -23.27571566865760033, -18.75553318983527262, 72.90801392080540211 ) ) ;
#402=FACE_BOUND ( 'NONE', #15605, .T. ) ;
#404=ORIENTED_EDGE ( 'NONE', *, *, #13134, .T. ) ;
#405=EDGE_CURVE ( 'NONE', #45877, #29512, #47050, .T. ) ;
#406=CARTESIAN_POINT ( 'NONE',  ( -10.33531692083374587, -17.10115316349580894, 57.87255846826901262 ) ) ;
#407=CARTESIAN_POINT ( 'NONE',  ( -18.18338144371267617, -21.81849904615365432, 65.63060065626805795 ) ) ;
#408=CARTESIAN_POINT ( 'NONE',  ( -23.11971029740161754, -18.96910916387263768, 66.23878312252503520 ) ) ;
#411=CARTESIAN_POINT ( 'NONE',  ( -11.64902330566212463, -10.02396254413167576, 54.27966884056655061 ) ) ;
#412=EDGE_LOOP ( 'NONE', ( #31242, #8262, #36518, #17032, #48604 ) ) ;
#414=CARTESIAN_POINT ( 'NONE',  ( -20.84119928492008000, -20.97572016636869918, 62.41471400470057773 ) ) ;
#417=( BOUNDED_SURFACE ( )  B_SPLINE_SURFACE ( 3, 1, ( 
 ( #9732, #43708 ),
 ( #24518, #28912 ),
 ( #16610, #13866 ),
 ( #28443, #43468 ),
 ( #32380, #47398 ),
 ( #9963, #10214 ),
 ( #28194, #17083 ) ),
 .UNSPECIFIED., .T., .F., .F. ) 
 B_SPLINE_SURFACE_WITH_KNOTS ( ( 4, 3, 4 ),
 ( 2, 2 ),
 ( 0.000000000000000000, 0.5000000000000000000, 1.000000000000000000 ),
 ( 0.000000000000000000, 1.000000000000000000 ),
 .UNSPECIFIED. ) 
 GEOMETRIC_REPRESENTATION_ITEM ( )  RATIONAL_B_SPLINE_SURFACE ( (
 ( 1.000000000000000000, 1.000000000000000000),
 ( 0.3333333333333335369, 0.3333333333333330373),
 ( 0.3333333333333335369, 0.3333333333333330373),
 ( 1.000000000000000000, 1.000000000000000000),
 ( 0.3333333333333333703, 0.3333333333333333703),
 ( 0.3333333333333333703, 0.3333333333333333703),
 ( 1.000000000000000000, 1.000000000000000000) ) ) 
 REPRESENTATION_ITEM ( '' )  SURFACE ( )  );
#418=AXIS2_PLACEMENT_3D ( 'NONE', #26156, #2536, #11134 ) ;
#420=ORIENTED_EDGE ( 'NONE', *, *, #27980, .F. ) ;
#424=CARTESIAN_POINT ( 'NONE',  ( -15.49416032233947504, -8.028509233753512220, 74.07985659018982005 ) ) ;
#425=CARTESIAN_POINT ( 'NONE',  ( -22.31677934746245384, -19.81551963994498777, 69.17417984703425304 ) ) ;
#426=CARTESIAN_POINT ( 'NONE',  ( -12.84615363328625826, -20.17103110633857455, 72.09181604382622766 ) ) ;
#427=CARTESIAN_POINT ( 'NONE',  ( -16.65185932245351808, -21.81708442718849383, 65.51092266128213737 ) ) ;
#429=EDGE_CURVE ( 'NONE', #3477, #10747, #43455, .T. ) ;
#431=CARTESIAN_POINT ( 'NONE',  ( -12.49710231520240988, -20.39756436883700630, 71.96800174581260023 ) ) ;
#433=ORIENTED_EDGE ( 'NONE', *, *, #28932, .T. ) ;
#435=CARTESIAN_POINT ( 'NONE',  ( -17.70854774853812330, -7.363889232077062807, 63.73712292196469065 ) ) ;
#436=EDGE_CURVE ( 'NONE', #14770, #31554, #12369, .T. ) ;
#437=ADVANCED_FACE ( 'NONE', ( #38213 ), #30235, .T. ) ;
#438=ADVANCED_FACE ( 'NONE', ( #31329 ), #8225, .T. ) ;
#439=B_SPLINE_CURVE_WITH_KNOTS ( 'NONE', 3,
 ( #35789, #17792, #14089, #39984, #9946, #6255, #13849, #21279, #28423, #32818 ),
 .UNSPECIFIED., .F., .F.,
 ( 4, 2, 2, 2, 4 ),
 ( 0.6272669072782633970, 0.7522669073001574391, 0.8772669073220515923, 1.002266907343945634, 1.127266907365839677 ),
 .UNSPECIFIED. ) ;
#440=CARTESIAN_POINT ( 'NONE',  ( -11.87789744022826355, -9.834800395276692697, 64.16880944724786673 ) ) ;
#441=CARTESIAN_POINT ( 'NONE',  ( -13.50285511730657184, -21.14374568559905399, 65.13628878216876217 ) ) ;
#442=CARTESIAN_POINT ( 'NONE',  ( -23.70015231925135168, -18.82353928378165975, 69.47867257277708575 ) ) ;
#443=ORIENTED_EDGE ( 'NONE', *, *, #4482, .T. ) ;
#445=VERTEX_POINT ( 'NONE', #23953 ) ;
#446=CARTESIAN_POINT ( 'NONE',  ( -14.71758685070772366, -21.32224385381664788, 62.05089037315948275 ) ) ;
#447=CARTESIAN_POINT ( 'NONE',  ( -16.78411710364782650, -21.83009890335197767, 68.99560651669348488 ) ) ;
#448=DIRECTION ( 'NONE',  ( 0.6478992145799701285, -0.7617260713318518839, 1.927832152310587152E-08 ) ) ;
#449=EDGE_LOOP ( 'NONE', ( #43040, #18031 ) ) ;
#450=B_SPLINE_CURVE_WITH_KNOTS ( 'NONE', 1,
 ( #9421, #42674 ),
 .UNSPECIFIED., .F., .F.,
 ( 2, 2 ),
 ( 0.000000000000000000, 1.000000000000000000 ),
 .UNSPECIFIED. ) ;
#453=CARTESIAN_POINT ( 'NONE',  ( -24.20884359724224311, -11.73171579724705005, 59.59740298356196320 ) ) ;
#455=DIRECTION ( 'NONE',  ( 0.9904243694481096316, 0.1380563957348939774, 6.973877024228147881E-08 ) ) ;
#456=CARTESIAN_POINT ( 'NONE',  ( -10.04844915070208344, -15.85969764522557668, 64.76417530519553623 ) ) ;
#457=ORIENTED_EDGE ( 'NONE', *, *, #29503, .T. ) ;
#458=FACE_OUTER_BOUND ( 'NONE', #9913, .T. ) ;
#459=EDGE_LOOP ( 'NONE', ( #3422, #20688, #46896, #525, #3593 ) ) ;
#460=CARTESIAN_POINT ( 'NONE',  ( -23.21283044961208830, -10.11939778159179859, 63.25681392212788268 ) ) ;
#462=ORIENTED_EDGE ( 'NONE', *, *, #6730, .F. ) ;
#463=DIRECTION ( 'NONE',  ( -1.404489950266683237E-08, 6.428047446179355909E-07, 0.9999999999997932765 ) ) ;
#464=CARTESIAN_POINT ( 'NONE',  ( -24.57916482434842820, -12.73107666121563142, 69.95898344571149607 ) ) ;
#465=CARTESIAN_POINT ( 'NONE',  ( -24.24046553926340408, -13.21446260159300934, 62.84880869836692341 ) ) ;
#466=EDGE_CURVE ( 'NONE', #32966, #27479, #6623, .T. ) ;
#468=DIRECTION ( 'NONE',  ( 0.6621635203543606574, 0.7493593746073508033, 2.316976118889566110E-08 ) ) ;
#469=CARTESIAN_POINT ( 'NONE',  ( -22.20320178312271153, -19.92390373660361291, 65.70421731406698029 ) ) ;
#470=CARTESIAN_POINT ( 'NONE',  ( -10.95381480682210373, -17.48044017699314523, 68.09721944380058289 ) ) ;
#472=CARTESIAN_POINT ( 'NONE',  ( -22.42594789675818845, -19.77792426076253918, 69.45945937764655298 ) ) ;
#473=CARTESIAN_POINT ( 'NONE',  ( -21.35994700726987006, -8.956524206332462157, 70.01643677269403554 ) ) ;
#474=EDGE_LOOP ( 'NONE', ( #18767, #45773, #10429, #4944, #46509 ) ) ;
#475=ORIENTED_EDGE ( 'NONE', *, *, #24304, .T. ) ;
#476=CARTESIAN_POINT ( 'NONE',  ( -23.23616409499837587, -18.79948708312782557, 65.82389430043846801 ) ) ;
#477=CARTESIAN_POINT ( 'NONE',  ( -10.16749015965427105, -13.12235144340169235, 71.39323866028058774 ) ) ;
#478=CARTESIAN_POINT ( 'NONE',  ( -23.00190342510993347, -19.12578814502481350, 62.76895730438863552 ) ) ;
#481=CARTESIAN_POINT ( 'NONE',  ( -24.37683887807358474, -15.97618392648307584, 66.36324926629207255 ) ) ;
#482=CARTESIAN_POINT ( 'NONE',  ( -12.45682740369385044, -20.36257741321750103, 68.45002181329043367 ) ) ;
#483=CARTESIAN_POINT ( 'NONE',  ( -17.00835460083030881, -7.370762356853859387, 74.06744117325925458 ) ) ;
#484=CARTESIAN_POINT ( 'NONE',  ( -19.85891393954322837, -21.37210614461000446, 56.49999999999994316 ) ) ;
#486=VERTEX_POINT ( 'NONE', #35972 ) ;
#488=ADVANCED_FACE ( 'NONE', ( #39448 ), #12614, .T. ) ;
#490=CARTESIAN_POINT ( 'NONE',  ( -10.90759836534377492, -17.49952001658422063, 68.39721944423101263 ) ) ;
#493=EDGE_CURVE ( 'NONE', #23300, #44829, #34132, .T. ) ;
#495=CARTESIAN_POINT ( 'NONE',  ( -19.92081508208725182, -21.34881959396637541, 69.03314256940365112 ) ) ;
#496=CARTESIAN_POINT ( 'NONE',  ( -11.73260704738458671, -10.00184175524024610, 67.61401452035728710 ) ) ;
#497=DIRECTION ( 'NONE',  ( 0.04108628546905145756, 0.9991556020692450302, -4.908153721456555400E-18 ) ) ;
#498=ORIENTED_EDGE ( 'NONE', *, *, #14731, .T. ) ;
#502=CARTESIAN_POINT ( 'NONE',  ( -17.00708426123225436, -7.821638799215111071, 74.26018273346642218 ) ) ;
#503=CARTESIAN_POINT ( 'NONE',  ( -24.14992822999210276, -18.01341164000503525, 59.11882993461590274 ) ) ;
#504=EDGE_LOOP ( 'NONE', ( #46695, #33574, #44849, #33318, #47655 ) ) ;
#505=CARTESIAN_POINT ( 'NONE',  ( -11.65812116532299036, -18.87225936251257252, 64.74706785490784000 ) ) ;
#506=AXIS2_PLACEMENT_3D ( 'NONE', #33969, #37910, #7652 ) ;
#508=VERTEX_POINT ( 'NONE', #15199 ) ;
#510=CARTESIAN_POINT ( 'NONE',  ( -14.90981263331598150, -21.39562362703504306, 61.93600440604522817 ) ) ;
#511=ORIENTED_EDGE ( 'NONE', *, *, #39173, .T. ) ;
#512=CARTESIAN_POINT ( 'NONE',  ( -10.49862840407593367, -15.82799419795606966, 64.80771590052736997 ) ) ;
#513=DIRECTION ( 'NONE',  ( 0.9939059412784551073, 0.1102314832132140626, 5.576311685107536405E-08 ) ) ;
#515=DIRECTION ( 'NONE',  ( 0.7437128929774846631, -0.6684991644116392573, 1.736198598216997869E-08 ) ) ;
#519=CARTESIAN_POINT ( 'NONE',  ( -8.185066236809714013, -9.969861568386987116, 54.58422952202461431 ) ) ;
#520=CARTESIAN_POINT ( 'NONE',  ( -18.15518557434651825, -21.77104687284236917, 65.34532137711126154 ) ) ;
#521=FACE_BOUND ( 'NONE', #21781, .T. ) ;
#522=FACE_OUTER_BOUND ( 'NONE', #47386, .T. ) ;
#523=CARTESIAN_POINT ( 'NONE',  ( -17.12428427367203199, -7.815570071381127804, 70.50538321838570255 ) ) ;
#524=EDGE_LOOP ( 'NONE', ( #29055, #13582, #18581, #24516, #22203 ) ) ;
#525=ORIENTED_EDGE ( 'NONE', *, *, #13658, .F. ) ;
#526=DIRECTION ( 'NONE',  ( 1.770046472388780670E-07, -8.183081107261190203E-08, -0.9999999999999809042 ) ) ;
#527=CARTESIAN_POINT ( 'NONE',  ( -19.98813031515369332, -21.37641424997302053, 72.70478737316021522 ) ) ;
#528=ORIENTED_EDGE ( 'NONE', *, *, #23306, .F. ) ;
#530=CARTESIAN_POINT ( 'NONE',  ( -15.73904783414571362, -7.552099178812579083, 67.27860723075241367 ) ) ;
#531=CARTESIAN_POINT ( 'NONE',  ( -10.28012408155893986, -12.69583279732615821, 64.36812482108923916 ) ) ;
#532=CARTESIAN_POINT ( 'NONE',  ( -24.72842049104188433, -16.27552959397571897, 62.70054543384251389 ) ) ;
#533=( BOUNDED_SURFACE ( )  B_SPLINE_SURFACE ( 3, 1, ( 
 ( #15389, #11243 ),
 ( #34355, #642 ),
 ( #3600, #25764 ),
 ( #3357, #18603 ),
 ( #48657, #29958 ),
 ( #39030, #9249 ),
 ( #1607, #15643 ) ),
 .UNSPECIFIED., .T., .F., .F. ) 
 B_SPLINE_SURFACE_WITH_KNOTS ( ( 4, 3, 4 ),
 ( 2, 2 ),
 ( 0.000000000000000000, 0.5000000000000000000, 1.000000000000000000 ),
 ( 0.000000000000000000, 1.000000000000000000 ),
 .UNSPECIFIED. ) 
 GEOMETRIC_REPRESENTATION_ITEM ( )  RATIONAL_B_SPLINE_SURFACE ( (
 ( 1.000000000000000000, 1.000000000000000000),
 ( 0.3333333333333335369, 0.3333333333333330373),
 ( 0.3333333333333335369, 0.3333333333333330373),
 ( 1.000000000000000000, 1.000000000000000000),
 ( 0.3333333333333333703, 0.3333333333333333703),
 ( 0.3333333333333333703, 0.3333333333333333703),
 ( 1.000000000000000000, 1.000000000000000000) ) ) 
 REPRESENTATION_ITEM ( '' )  SURFACE ( )  );
#534=CARTESIAN_POINT ( 'NONE',  ( -12.04615335961045908, -19.96505441190284813, 61.53645242954323891 ) ) ;
#535=CARTESIAN_POINT ( 'NONE',  ( -11.41043474416280823, -19.20696576352171903, 71.80969020189922958 ) ) ;
#537=CARTESIAN_POINT ( 'NONE',  ( -24.38600087812161377, -15.53966288334215307, 73.00303710413747638 ) ) ;
#538=EDGE_CURVE ( 'NONE', #30207, #6304, #36209, .T. ) ;
#539=CARTESIAN_POINT ( 'NONE',  ( -14.48548941065489970, -8.400516866317895293, 67.27447142263336843 ) ) ;
#540=CARTESIAN_POINT ( 'NONE',  ( -24.17882124642622088, -12.77733483093900091, 73.54225673225543858 ) ) ;
#541=PLANE ( 'NONE',  #23265 ) ;
#542=CARTESIAN_POINT ( 'NONE',  ( -12.77099621783261263, -20.03938943333788814, 71.82270288656182800 ) ) ;
#544=( BOUNDED_CURVE ( )  B_SPLINE_CURVE ( 3, ( #29925, #40748, #21791, #48141 ),
 .UNSPECIFIED., .F., .F. ) 
 B_SPLINE_CURVE_WITH_KNOTS ( ( 4, 4 ),
 ( 0.000000000000000000, 0.4074455897393696180 ),
 .UNSPECIFIED. ) 
 CURVE ( )  GEOMETRIC_REPRESENTATION_ITEM ( )  RATIONAL_B_SPLINE_CURVE ( ( 1.000000000000000000, 0.4567392136813236969, 0.3561768502900272138, 0.6983129098261106060 ) ) 
 REPRESENTATION_ITEM ( '' )  );
#545=VERTEX_POINT ( 'NONE', #33927 ) ;
#552=CARTESIAN_POINT ( 'NONE',  ( -11.71665266943325534, -18.96132379659194100, 64.90273906658698877 ) ) ;
#553=EDGE_CURVE ( 'NONE', #43090, #13641, #7363, .T. ) ;
#554=CARTESIAN_POINT ( 'NONE',  ( -16.53261792465593771, -21.75226837608146369, 61.82856087129801637 ) ) ;
#556=ADVANCED_FACE ( 'NONE', ( #40403 ), #3646, .T. ) ;
#557=CARTESIAN_POINT ( 'NONE',  ( -12.84690951644825851, -8.931012861620404308, 67.56438176077992352 ) ) ;
#558=CARTESIAN_POINT ( 'NONE',  ( -16.15628411965152722, -22.15059256196195037, 58.47859698976697729 ) ) ;
#560=ORIENTED_EDGE ( 'NONE', *, *, #10649, .F. ) ;
#561=B_SPLINE_CURVE_WITH_KNOTS ( 'NONE', 3,
 ( #45712, #8272, #26976, #30926, #4564, #8764, #34595, #879, #15881, #45938 ),
 .UNSPECIFIED., .F., .F.,
 ( 4, 2, 2, 2, 4 ),
 ( 0.6272669072877743446, 0.7522669073072931756, 0.8772669073268121176, 1.002266907346331060, 1.127266907365849891 ),
 .UNSPECIFIED. ) ;
#562=CARTESIAN_POINT ( 'NONE',  ( -20.95714566783631483, -8.250050064981410358, 60.00271774409104353 ) ) ;
#563=CARTESIAN_POINT ( 'NONE',  ( -17.57575749508838925, -7.360700902354934350, 63.65718735946740736 ) ) ;
#564=EDGE_LOOP ( 'NONE', ( #27318, #12069 ) ) ;
#565=DIRECTION ( 'NONE',  ( 0.5420872618288284928, 0.8403222004463034578, -7.592316861453148064E-08 ) ) ;
#566=VERTEX_POINT ( 'NONE', #10386 ) ;
#567=CARTESIAN_POINT ( 'NONE',  ( -11.14114473067313682, -10.80566704772025233, 57.32407823191172014 ) ) ;
#569=CARTESIAN_POINT ( 'NONE',  ( -12.37350074511489595, -12.59798860466149861, 53.69233794759168887 ) ) ;
#571=CARTESIAN_POINT ( 'NONE',  ( -19.66015584026798280, -21.44380816191627659, 69.00652708242157019 ) ) ;
#572=CARTESIAN_POINT ( 'NONE',  ( -11.77150565662344484, -19.02841119382535950, 68.42509345399683696 ) ) ;
#573=CARTESIAN_POINT ( 'NONE',  ( -14.56525312440409081, -21.68886035253952116, 58.36629080999882291 ) ) ;
#575=VERTEX_POINT ( 'NONE', #221 ) ;
#579=FACE_OUTER_BOUND ( 'NONE', #40950, .T. ) ;
#580=CYLINDRICAL_SURFACE ( 'NONE', #31369, 0.1499999999999984401 ) ;
#584=CARTESIAN_POINT ( 'NONE',  ( -15.11195830621016256, -21.41632612911037370, 65.40596681519618016 ) ) ;
#585=CARTESIAN_POINT ( 'NONE',  ( -24.28035819322802880, -16.22076492358945998, 59.35005677771162880 ) ) ;
#586=ORIENTED_EDGE ( 'NONE', *, *, #6608, .F. ) ;
#587=CARTESIAN_POINT ( 'NONE',  ( -17.19980194945414809, -7.762775306501539241, 70.64035839668011363 ) ) ;
#588=VECTOR ( 'NONE', #14745, 1000.000000000000114 ) ;
#590=DIRECTION ( 'NONE',  ( -0.6105870317843966610, -0.7919491628991827126, 6.540688078712155195E-08 ) ) ;
#591=EDGE_CURVE ( 'NONE', #27215, #5198, #21725, .T. ) ;
#592=ORIENTED_EDGE ( 'NONE', *, *, #8079, .F. ) ;
#593=CARTESIAN_POINT ( 'NONE',  ( -10.37857782286507025, -14.46928323978489317, 71.62782678106509593 ) ) ;
#594=CARTESIAN_POINT ( 'NONE',  ( -10.43972881942000086, -15.77115500203794873, 64.52243715390834211 ) ) ;
#596=VERTEX_POINT ( 'NONE', #40174 ) ;
#598=CARTESIAN_POINT ( 'NONE',  ( -24.14981099001045095, -11.60321323961852258, 59.59580478148293992 ) ) ;
#602=ORIENTED_EDGE ( 'NONE', *, *, #29857, .F. ) ;
#603=EDGE_LOOP ( 'NONE', ( #36733, #18281 ) ) ;
#605=DIRECTION ( 'NONE',  ( -5.731567514496413899E-31, -1.020425574103664789E-16, -1.000000000000000000 ) ) ;
#606=ADVANCED_FACE ( 'NONE', ( #47562 ), #26776, .T. ) ;
#607=CARTESIAN_POINT ( 'NONE',  ( -10.45137630651438698, -14.19109027996143801, 61.20355913676015547 ) ) ;
#608=LINE ( 'NONE', #7525, #26051 ) ;
#609=EDGE_CURVE ( 'NONE', #19293, #40234, #36450, .T. ) ;
#610=AXIS2_PLACEMENT_3D ( 'NONE', #22135, #10795, #30262 ) ;
#612=EDGE_CURVE ( 'NONE', #42866, #14276, #37609, .T. ) ;
#613=CARTESIAN_POINT ( 'NONE',  ( -20.35208293893518672, -8.450992964911224092, 67.08104082230126153 ) ) ;
#615=( BOUNDED_CURVE ( )  B_SPLINE_CURVE ( 3, ( #7951, #41907, #8185, #539 ),
 .UNSPECIFIED., .F., .F. ) 
 B_SPLINE_CURVE_WITH_KNOTS ( ( 4, 4 ),
 ( 0.4074455897393645665, 0.5000000000000000000 ),
 .UNSPECIFIED. ) 
 CURVE ( )  GEOMETRIC_REPRESENTATION_ITEM ( )  RATIONAL_B_SPLINE_CURVE ( ( 0.6983129098261017242, 0.7760317562606843245, 0.8765941196519773104, 0.9999999999999659162 ) ) 
 REPRESENTATION_ITEM ( '' )  );
#617=CYLINDRICAL_SURFACE ( 'NONE', #6832, 0.1500000000000042966 ) ;
#618=EDGE_CURVE ( 'NONE', #14550, #43562, #17736, .T. ) ;
#619=EDGE_LOOP ( 'NONE', ( #6254, #15796, #31967, #18011, #32295 ) ) ;
#620=CARTESIAN_POINT ( 'NONE',  ( -9.927469056236301270, -15.37997598727726611, 54.02312124697527906 ) ) ;
#622=ORIENTED_EDGE ( 'NONE', *, *, #12533, .F. ) ;
#623=CARTESIAN_POINT ( 'NONE',  ( -13.22529448846758804, -9.145569705956512863, 64.19474388871357462 ) ) ;
#624=CARTESIAN_POINT ( 'NONE',  ( -9.975093145215874202, -14.93635225021824198, 74.98274299234972773 ) ) ;
#625=CARTESIAN_POINT ( 'NONE',  ( -19.11145557798581152, -7.964112677450091660, 63.73089235102099792 ) ) ;
#626=CARTESIAN_POINT ( 'NONE',  ( -18.11514229927295716, -22.22721396694290164, 65.46815266832128088 ) ) ;
#627=ORIENTED_EDGE ( 'NONE', *, *, #4548, .T. ) ;
#628=CARTESIAN_POINT ( 'NONE',  ( -10.78967749848787427, -12.41559940729129785, 61.21342246320382685 ) ) ;
#631=CARTESIAN_POINT ( 'NONE',  ( -19.36518065869528726, -8.031383756764064685, 59.97565108339750850 ) ) ;
#633=CARTESIAN_POINT ( 'NONE',  ( -18.30602013973305020, -21.80685202924323463, 72.69999788315199396 ) ) ;
#636=DIRECTION ( 'NONE',  ( -0.3478314405900309603, -0.9375570856950864451, 0.000000000000000000 ) ) ;
#637=ORIENTED_EDGE ( 'NONE', *, *, #2970, .F. ) ;
#638=CARTESIAN_POINT ( 'NONE',  ( -22.15985579531568916, -19.96414753270404674, 62.46112518014844284 ) ) ;
#639=CARTESIAN_POINT ( 'NONE',  ( -15.32718698399739132, -9.710093178977245998, 53.88362224778187226 ) ) ;
#640=CARTESIAN_POINT ( 'NONE',  ( -12.27729947935473476, -9.991218615320081042, 60.85918086709605745 ) ) ;
#641=AXIS2_PLACEMENT_3D ( 'NONE', #12908, #32598, #42958 ) ;
#642=CARTESIAN_POINT ( 'NONE',  ( -15.88847107554206062, -7.518423027132939751, 63.78355628068795369 ) ) ;
#643=ORIENTED_EDGE ( 'NONE', *, *, #45775, .F. ) ;
#644=CARTESIAN_POINT ( 'NONE',  ( -10.53028993777715883, -16.28642212234895226, 71.73278239416407587 ) ) ;
#647=CARTESIAN_POINT ( 'NONE',  ( -17.85555652284939043, -7.772123375420258107, 60.09532845646905486 ) ) ;
#648=CARTESIAN_POINT ( 'NONE',  ( -22.97806213383195484, -10.54588184283626262, 63.18259140678883767 ) ) ;
#651=VECTOR ( 'NONE', #27035, 1000.000000000000000 ) ;
#654=ORIENTED_EDGE ( 'NONE', *, *, #8134, .F. ) ;
#655=ORIENTED_EDGE ( 'NONE', *, *, #42876, .F. ) ;
#656=VERTEX_POINT ( 'NONE', #26546 ) ;
#657=CARTESIAN_POINT ( 'NONE',  ( -17.98584054083101691, -22.23808389992613499, 62.06031238270200845 ) ) ;
#661=CARTESIAN_POINT ( 'NONE',  ( -24.13556280029956724, -12.81997495155604483, 66.52920008143310326 ) ) ;
#662=CARTESIAN_POINT ( 'NONE',  ( -11.81594133544200709, -9.904820009267291780, 64.20631235510137458 ) ) ;
#664=DIRECTION ( 'NONE',  ( 0.8565259173193583431, -0.5161040137028850561, 6.301967848571307172E-08 ) ) ;
#668=CARTESIAN_POINT ( 'NONE',  ( -12.77013062424865630, -8.927826924028671840, 54.27966884056655061 ) ) ;
#670=CARTESIAN_POINT ( 'NONE',  ( -23.62338436797153918, -18.94230004192412409, 69.48027381658378943 ) ) ;
#672=( BOUNDED_CURVE ( )  B_SPLINE_CURVE ( 3, ( #30748, #35382, #4629, #16422 ),
 .UNSPECIFIED., .F., .F. ) 
 B_SPLINE_CURVE_WITH_KNOTS ( ( 4, 4 ),
 ( 0.000000000000000000, 0.4074455897393622905 ),
 .UNSPECIFIED. ) 
 CURVE ( )  GEOMETRIC_REPRESENTATION_ITEM ( )  RATIONAL_B_SPLINE_CURVE ( ( 1.000000000000000000, 0.4567392136813403503, 0.3561768502900334310, 0.6983129098260791867 ) ) 
 REPRESENTATION_ITEM ( '' )  );
#674=ORIENTED_EDGE ( 'NONE', *, *, #17450, .F. ) ;
#677=CARTESIAN_POINT ( 'NONE',  ( -10.47203305924008632, -16.00180800482426235, 71.53930669669551889 ) ) ;
#679=B_SPLINE_CURVE_WITH_KNOTS ( 'NONE', 3,
 ( #24698, #25641, #33011, #47812, #14293, #21236, #32326, #29343, #28392, #40655 ),
 .UNSPECIFIED., .F., .F.,
 ( 4, 2, 2, 2, 4 ),
 ( 0.000000000000000000, 0.2500000000000000000, 0.5000000000000000000, 0.7500000000000000000, 1.000000000000000000 ),
 .UNSPECIFIED. ) ;
#680=CARTESIAN_POINT ( 'NONE',  ( -13.43921569888383694, -8.993430976374535035, 60.58950277493168812 ) ) ;
#683=ORIENTED_EDGE ( 'NONE', *, *, #38447, .F. ) ;
#684=CARTESIAN_POINT ( 'NONE',  ( -18.50931870666621037, -21.77518001355031529, 72.28510940651260341 ) ) ;
#685=( BOUNDED_CURVE ( )  B_SPLINE_CURVE ( 3, ( #11024, #29002, #44052, #44773 ),
 .UNSPECIFIED., .F., .F. ) 
 B_SPLINE_CURVE_WITH_KNOTS ( ( 4, 4 ),
 ( 0.4074455897393601256, 0.5000000000000000000 ),
 .UNSPECIFIED. ) 
 CURVE ( )  GEOMETRIC_REPRESENTATION_ITEM ( )  RATIONAL_B_SPLINE_CURVE ( ( 0.6983129098260726364, 0.7760317562606952047, 0.8765941196520086187, 1.000000000000023093 ) ) 
 REPRESENTATION_ITEM ( '' )  );
#686=AXIS2_PLACEMENT_3D ( 'NONE', #14516, #18238, #33745 ) ;
#688=FACE_OUTER_BOUND ( 'NONE', #15519, .T. ) ;
#692=CARTESIAN_POINT ( 'NONE',  ( -24.87290000513101873, -14.67112934921935974, 62.82801050733710468 ) ) ;
#694=CARTESIAN_POINT ( 'NONE',  ( -22.47468696571113256, -17.02042448482726300, 53.69233794759168887 ) ) ;
#697=CARTESIAN_POINT ( 'NONE',  ( -11.12358174778395714, -11.75903488045733347, 71.38860871064898106 ) ) ;
#699=( BOUNDED_SURFACE ( )  B_SPLINE_SURFACE ( 3, 1, ( 
 ( #9049, #1648 ),
 ( #43268, #35371 ),
 ( #31689, #46714 ),
 ( #27984, #43009 ),
 ( #5601, #26605 ),
 ( #35609, #1886 ),
 ( #31927, #24558 ) ),
 .UNSPECIFIED., .T., .F., .F. ) 
 B_SPLINE_SURFACE_WITH_KNOTS ( ( 4, 3, 4 ),
 ( 2, 2 ),
 ( 0.000000000000000000, 0.5000000000000000000, 1.000000000000000000 ),
 ( 0.000000000000000000, 1.000000000000000000 ),
 .UNSPECIFIED. ) 
 GEOMETRIC_REPRESENTATION_ITEM ( )  RATIONAL_B_SPLINE_SURFACE ( (
 ( 1.000000000000000000, 1.000000000000000000),
 ( 0.3333333333333335369, 0.3333333333333330373),
 ( 0.3333333333333335369, 0.3333333333333330373),
 ( 1.000000000000000000, 1.000000000000000000),
 ( 0.3333333333333333703, 0.3333333333333333703),
 ( 0.3333333333333333703, 0.3333333333333333703),
 ( 1.000000000000000000, 1.000000000000000000) ) ) 
 REPRESENTATION_ITEM ( '' )  SURFACE ( )  );
#700=VERTEX_POINT ( 'NONE', #42551 ) ;
#702=ORIENTED_EDGE ( 'NONE', *, *, #13629, .T. ) ;
#704=CARTESIAN_POINT ( 'NONE',  ( -16.59509239138002101, -21.81331869282671221, 61.64079261740195648 ) ) ;
#709=LINE ( 'NONE', #30519, #41682 ) ;
#710=CARTESIAN_POINT ( 'NONE',  ( -24.69852204723760281, -16.41745771733451775, 59.30827817708741634 ) ) ;
#711=ORIENTED_EDGE ( 'NONE', *, *, #23137, .T. ) ;
#712=CARTESIAN_POINT ( 'NONE',  ( -14.97188219925329378, -8.199429090594037461, 56.84999999999995168 ) ) ;
#713=CARTESIAN_POINT ( 'NONE',  ( -12.76547314785493192, -9.517330534081262172, 74.60450883341005124 ) ) ;
#715=ORIENTED_EDGE ( 'NONE', *, *, #7569, .F. ) ;
#723=CARTESIAN_POINT ( 'NONE',  ( -11.68391713028079515, -10.70246380009546527, 71.12460117624890188 ) ) ;
#724=CARTESIAN_POINT ( 'NONE',  ( -23.28150499554093500, -18.64225713161144782, 69.29372035757846504 ) ) ;
#726=VECTOR ( 'NONE', #11983, 1000.000000000000000 ) ;
#727=CARTESIAN_POINT ( 'NONE',  ( -11.13733870171179596, -11.61806121328042174, 67.90392505421056057 ) ) ;
#728=ORIENTED_EDGE ( 'NONE', *, *, #17278, .F. ) ;
#729=CARTESIAN_POINT ( 'NONE',  ( -22.52972399543339677, -9.943266245822872662, 69.89689837695897268 ) ) ;
#731=CARTESIAN_POINT ( 'NONE',  ( -10.03104929242693544, -13.88935366066504251, 57.55486709734128681 ) ) ;
#735=EDGE_CURVE ( 'NONE', #35067, #41098, #33494, .T. ) ;
#736=CARTESIAN_POINT ( 'NONE',  ( -20.54979492810923603, -8.489990406890694175, 63.46121512946601229 ) ) ;
#739=CARTESIAN_POINT ( 'NONE',  ( -10.16925234506895670, -13.11493237325164429, 71.40102718425720241 ) ) ;
#740=ORIENTED_EDGE ( 'NONE', *, *, #28298, .F. ) ;
#741=CARTESIAN_POINT ( 'NONE',  ( -23.53718313364170456, -11.39868142885006641, 69.89210781356229063 ) ) ;
#746=CARTESIAN_POINT ( 'NONE',  ( -12.93303430567921808, -20.17867969065821399, 72.03327057247898324 ) ) ;
#747=CARTESIAN_POINT ( 'NONE',  ( -14.01837044221388595, -8.636059239884618322, 74.48482605064899076 ) ) ;
#748=VERTEX_POINT ( 'NONE', #46232 ) ;
#749=CARTESIAN_POINT ( 'NONE',  ( -12.74802523442671465, -20.09592109768945889, 65.02242199588995675 ) ) ;
#752=EDGE_CURVE ( 'NONE', #21025, #27231, #29425, .T. ) ;
#753=EDGE_LOOP ( 'NONE', ( #38139, #35733, #34548, #4648, #26737 ) ) ;
#755=CARTESIAN_POINT ( 'NONE',  ( -11.17842666812006769, -10.74653426074781848, 57.39558607234117460 ) ) ;
#759=EDGE_CURVE ( 'NONE', #33339, #19087, #2389, .T. ) ;
#760=FACE_OUTER_BOUND ( 'NONE', #17758, .T. ) ;
#762=CARTESIAN_POINT ( 'NONE',  ( -24.47161816259883338, -14.62087121170030635, 63.01296490870000611 ) ) ;
#763=CARTESIAN_POINT ( 'NONE',  ( -10.52750029887962491, -17.62704889381915407, 68.29060234424891007 ) ) ;
#765=ORIENTED_EDGE ( 'NONE', *, *, #18837, .F. ) ;
#766=CARTESIAN_POINT ( 'NONE',  ( -10.43360882127813838, -14.44320667503941458, 64.46091912948344316 ) ) ;
#769=DIRECTION ( 'NONE',  ( 2.654446662475610288E-06, -3.134491601460476904E-06, 0.9999999999915645255 ) ) ;
#770=CARTESIAN_POINT ( 'NONE',  ( -24.76424570620368115, -16.08454870407971882, 66.24137714576976066 ) ) ;
#771=VECTOR ( 'NONE', #3922, 1000.000000000000000 ) ;
#772=ORIENTED_EDGE ( 'NONE', *, *, #31833, .F. ) ;
#773=VERTEX_POINT ( 'NONE', #35134 ) ;
#774=CARTESIAN_POINT ( 'NONE',  ( -21.40187103850036721, -9.048701367307623755, 73.61745452359328112 ) ) ;
#776=ORIENTED_EDGE ( 'NONE', *, *, #46959, .F. ) ;
#777=CARTESIAN_POINT ( 'NONE',  ( -20.99713037368098156, -21.34662133218488833, 62.23754514806859817 ) ) ;
#778=CARTESIAN_POINT ( 'NONE',  ( -15.08687585379459506, -21.46369733121157708, 68.99081615631787656 ) ) ;
#780=CARTESIAN_POINT ( 'NONE',  ( -24.73909915436057716, -16.22127400844152234, 62.69990344863494869 ) ) ;
#781=CARTESIAN_POINT ( 'NONE',  ( -24.38811233016677704, -14.09928486418781901, 73.42271532469474948 ) ) ;
#782=CARTESIAN_POINT ( 'NONE',  ( -11.19706266256277694, -11.50303319689152914, 67.63336710488009373 ) ) ;
#783=CARTESIAN_POINT ( 'NONE',  ( -13.96760974046062920, -8.722112190022174971, 74.39057940708781302 ) ) ;
#784=VERTEX_POINT ( 'NONE', #9055 ) ;
#785=CARTESIAN_POINT ( 'NONE',  ( -12.23301264461619553, -10.03852782535897958, 60.84446034103241630 ) ) ;
#786=EDGE_CURVE ( 'NONE', #31226, #12218, #6500, .T. ) ;
#788=CARTESIAN_POINT ( 'NONE',  ( -13.71338950266841472, -20.80363499509022773, 64.98628881289567971 ) ) ;
#789=DIRECTION ( 'NONE',  ( 0.5327540375067997269, 0.8462701315302331162, 7.203825861310633201E-08 ) ) ;
#793=EDGE_LOOP ( 'NONE', ( #35327, #32327, #24506, #37244, #18270 ) ) ;
#794=CARTESIAN_POINT ( 'NONE',  ( -20.10179291524702805, -21.76144317846600629, 72.66124644823618439 ) ) ;
#795=EDGE_LOOP ( 'NONE', ( #9092, #33098, #976, #11055, #17567 ) ) ;
#797=EDGE_CURVE ( 'NONE', #30726, #47586, #41867, .T. ) ;
#798=CARTESIAN_POINT ( 'NONE',  ( -10.47387877723939731, -13.58059689071059495, 57.59258137113961595 ) ) ;
#799=AXIS2_PLACEMENT_3D ( 'NONE', #38007, #22270, #37510 ) ;
#800=CARTESIAN_POINT ( 'NONE',  ( -16.23116076413911557, -7.455249184188991407, 60.31533086125586607 ) ) ;
#802=CARTESIAN_POINT ( 'NONE',  ( -17.91716493482169525, -7.374790294242734134, 60.26716059546817661 ) ) ;
#805=ORIENTED_EDGE ( 'NONE', *, *, #5345, .T. ) ;
#806=CARTESIAN_POINT ( 'NONE',  ( -18.39951368268757648, -22.19516171751901368, 69.00010101991060196 ) ) ;
#807=CARTESIAN_POINT ( 'NONE',  ( -13.82689732469268407, -20.87277619789260186, 68.47097268802275494 ) ) ;
#808=ORIENTED_EDGE ( 'NONE', *, *, #15982, .F. ) ;
#810=CARTESIAN_POINT ( 'NONE',  ( -16.78181722113097152, -22.23154757984593388, 68.73914717078854153 ) ) ;
#811=CARTESIAN_POINT ( 'NONE',  ( -17.15134030326023051, -7.364115279526828317, 70.67531275522621570 ) ) ;
#813=EDGE_CURVE ( 'NONE', #22280, #24254, #2851, .T. ) ;
#814=CARTESIAN_POINT ( 'NONE',  ( -24.11099954625066744, -11.52470009423637620, 63.05244027053452527 ) ) ;
#817=( BOUNDED_CURVE ( )  B_SPLINE_CURVE ( 3, ( #15565, #572, #29890, #7247 ),
 .UNSPECIFIED., .F., .F. ) 
 B_SPLINE_CURVE_WITH_KNOTS ( ( 4, 4 ),
 ( 0.000000000000000000, 0.4074455897393677306 ),
 .UNSPECIFIED. ) 
 CURVE ( )  GEOMETRIC_REPRESENTATION_ITEM ( )  RATIONAL_B_SPLINE_CURVE ( ( 1.000000000000000000, 0.4567392136813272496, 0.3561768502900285460, 0.6983129098261039447 ) ) 
 REPRESENTATION_ITEM ( '' )  );
#818=CARTESIAN_POINT ( 'NONE',  ( -14.52870633129714406, -21.67373273928137323, 58.32764366538068401 ) ) ;
#824=EDGE_CURVE ( 'NONE', #29117, #42781, #29212, .T. ) ;
#825=ADVANCED_FACE ( 'NONE', ( #25279 ), #2620, .T. ) ;
#828=VERTEX_POINT ( 'NONE', #14155 ) ;
#829=EDGE_CURVE ( 'NONE', #42076, #28542, #17636, .T. ) ;
#830=FACE_OUTER_BOUND ( 'NONE', #37021, .T. ) ;
#831=DIRECTION ( 'NONE',  ( 4.924618305738831318E-06, 4.007739938527551184E-06, 0.9999999999798430128 ) ) ;
#832=ORIENTED_EDGE ( 'NONE', *, *, #19343, .T. ) ;
#833=DIRECTION ( 'NONE',  ( 2.846534188916127659E-06, 1.189262794724463340E-05, 0.9999999999252312533 ) ) ;
#834=VECTOR ( 'NONE', #24049, 999.9999999999998863 ) ;
#835=CARTESIAN_POINT ( 'NONE',  ( -21.51679988820674438, -20.55329806219026523, 72.40957539702174017 ) ) ;
#840=( BOUNDED_CURVE ( )  B_SPLINE_CURVE ( 3, ( #7888, #8613, #41856, #11814 ),
 .UNSPECIFIED., .F., .F. ) 
 B_SPLINE_CURVE_WITH_KNOTS ( ( 4, 4 ),
 ( 0.5000000000000000000, 0.9074455897393669535 ),
 .UNSPECIFIED. ) 
 CURVE ( )  GEOMETRIC_REPRESENTATION_ITEM ( )  RATIONAL_B_SPLINE_CURVE ( ( 1.000000000000006883, 0.4567392136813371306, 0.3561768502900272693, 0.6983129098260848489 ) ) 
 REPRESENTATION_ITEM ( '' )  );
#841=CARTESIAN_POINT ( 'NONE',  ( -24.42310880397785411, -14.69177626764110300, 59.43403519634394172 ) ) ;
#843=ADVANCED_FACE ( 'NONE', ( #17390 ), #6566, .T. ) ;
#844=ORIENTED_EDGE ( 'NONE', *, *, #40091, .F. ) ;
#845=AXIS2_PLACEMENT_3D ( 'NONE', #36479, #32795, #13827 ) ;
#847=CARTESIAN_POINT ( 'NONE',  ( -24.20817551436923765, -11.73026151181330512, 59.73881638530829008 ) ) ;
#848=CARTESIAN_POINT ( 'NONE',  ( -20.37299714182666222, -8.405577154986387356, 67.08104082189564110 ) ) ;
#850=CARTESIAN_POINT ( 'NONE',  ( -23.12753516214766591, -18.86773028979367695, 62.63941477998005780 ) ) ;
#851=B_SPLINE_CURVE_WITH_KNOTS ( 'NONE', 1,
 ( #38087, #15187 ),
 .UNSPECIFIED., .F., .F.,
 ( 2, 2 ),
 ( 0.000000000000000000, 1.000000000000000000 ),
 .UNSPECIFIED. ) ;
#852=ORIENTED_EDGE ( 'NONE', *, *, #26295, .F. ) ;
#853=ORIENTED_EDGE ( 'NONE', *, *, #18315, .F. ) ;
#855=CARTESIAN_POINT ( 'NONE',  ( -19.13461862846645900, -7.969822530380906933, 63.43089260374607363 ) ) ;
#860=CARTESIAN_POINT ( 'NONE',  ( -17.93190708896392493, -21.84390349538901077, 58.29064763788917958 ) ) ;
#861=CARTESIAN_POINT ( 'NONE',  ( -15.27269024242438533, -21.52607325516635939, 72.46064223565690554 ) ) ;
#862=CARTESIAN_POINT ( 'NONE',  ( -10.37795889460693033, -14.56696403379599403, 68.14328054657653411 ) ) ;
#863=AXIS2_PLACEMENT_3D ( 'NONE', #23090, #7832, #22851 ) ;
#866=ORIENTED_EDGE ( 'NONE', *, *, #5394, .T. ) ;
#867=CARTESIAN_POINT ( 'NONE',  ( -21.52107272639815960, -9.068161724387254097, 66.54661176836198422 ) ) ;
#868=CARTESIAN_POINT ( 'NONE',  ( -18.92057448382017526, -7.919863665830077615, 67.20071783788056052 ) ) ;
#869=ORIENTED_EDGE ( 'NONE', *, *, #30060, .T. ) ;
#870=PLANE ( 'NONE',  #23720 ) ;
#871=DIRECTION ( 'NONE',  ( 0.6264825908887947659, -0.7794354131762691873, 3.858680029754496192E-08 ) ) ;
#872=EDGE_LOOP ( 'NONE', ( #3030, #44945, #18541, #2230, #9303 ) ) ;
#873=EDGE_CURVE ( 'NONE', #19668, #43006, #40632, .T. ) ;
#875=EDGE_LOOP ( 'NONE', ( #46633, #12055, #15072, #2979, #36505 ) ) ;
#876=FACE_OUTER_BOUND ( 'NONE', #32788, .T. ) ;
#877=B_SPLINE_CURVE_WITH_KNOTS ( 'NONE', 3,
 ( #3640, #3903, #18909, #33656, #30250, #45269, #11518, #7845, #22865, #4148 ),
 .UNSPECIFIED., .F., .F.,
 ( 4, 2, 2, 2, 4 ),
 ( 0.1272669073657703986, 0.2522669073462747713, 0.3772669073267791440, 0.5022669073072835166, 0.6272669072877878893 ),
 .UNSPECIFIED. ) ;
#878=CARTESIAN_POINT ( 'NONE',  ( -21.67414471755420635, -8.689506427787394571, 70.24477150985708818 ) ) ;
#879=CARTESIAN_POINT ( 'NONE',  ( -20.92525905000154296, -8.233149033200417577, 59.94151005296296120 ) ) ;
#880=EDGE_LOOP ( 'NONE', ( #22050, #8932, #18939, #35498, #20588 ) ) ;
#881=CARTESIAN_POINT ( 'NONE',  ( -10.32029913342570815, -17.05393162916765348, 57.78786302709333000 ) ) ;
#882=CARTESIAN_POINT ( 'NONE',  ( -17.70776835051902864, -22.25388969026799657, 58.52057945155585372 ) ) ;
#883=CARTESIAN_POINT ( 'NONE',  ( -23.84653597794508784, -18.58622903642730151, 72.87712840465626130 ) ) ;
#884=CYLINDRICAL_SURFACE ( 'NONE', #28170, 7.000000000000000888 ) ;
#886=B_SPLINE_CURVE_WITH_KNOTS ( 'NONE', 3,
 ( #32581, #5996, #36496, #32358, #36018, #2778, #5527, #43684, #20547, #16819 ),
 .UNSPECIFIED., .F., .F.,
 ( 4, 2, 2, 2, 4 ),
 ( 0.000000000000000000, 0.2500000000000000000, 0.5000000000000000000, 0.7500000000000000000, 1.000000000000000000 ),
 .UNSPECIFIED. ) ;
#887=CARTESIAN_POINT ( 'NONE',  ( -22.17083152876919527, -19.95395936491961209, 62.42542368773413131 ) ) ;
#891=VERTEX_POINT ( 'NONE', #28962 ) ;
#892=CARTESIAN_POINT ( 'NONE',  ( -12.91576191806997365, -9.388722997169709927, 71.13453240065665284 ) ) ;
#893=ADVANCED_FACE ( 'NONE', ( #21099 ), #39805, .T. ) ;
#894=ORIENTED_EDGE ( 'NONE', *, *, #44461, .T. ) ;
#895=DIRECTION ( 'NONE',  ( 0.7621627669932625748, -0.6473854467078884456, 3.680865982637999047E-08 ) ) ;
#897=VERTEX_POINT ( 'NONE', #43756 ) ;
#899=CARTESIAN_POINT ( 'NONE',  ( -10.99582121268164414, -11.91441617825094923, 74.70840195586961840 ) ) ;
#900=CARTESIAN_POINT ( 'NONE',  ( -12.69123082366038702, -9.055659981287114135, 71.04199494340680587 ) ) ;
#902=ORIENTED_EDGE ( 'NONE', *, *, #1866, .F. ) ;
#903=ORIENTED_EDGE ( 'NONE', *, *, #44528, .F. ) ;
#904=CARTESIAN_POINT ( 'NONE',  ( -10.39906353449755372, -15.43672942677450521, 61.45277822496478848 ) ) ;
#907=CARTESIAN_POINT ( 'NONE',  ( -16.59183161123116079, -7.337091670555837553, 53.76227901944321985 ) ) ;
#909=CARTESIAN_POINT ( 'NONE',  ( -17.44602373156464026, -7.359070285474746065, 67.16006197583749326 ) ) ;
#910=CARTESIAN_POINT ( 'NONE',  ( -10.27345486655506868, -12.71824029969684844, 64.45331411623358520 ) ) ;
#913=EDGE_LOOP ( 'NONE', ( #34629, #10370 ) ) ;
#915=CARTESIAN_POINT ( 'NONE',  ( -11.87343833590673192, -9.839839846620931141, 64.15197417175610894 ) ) ;
#916=CARTESIAN_POINT ( 'NONE',  ( -21.02300714775091706, -21.33228198917356977, 62.21497154950080954 ) ) ;
#917=FACE_OUTER_BOUND ( 'NONE', #9999, .T. ) ;
#918=VERTEX_POINT ( 'NONE', #21585 ) ;
#920=ORIENTED_EDGE ( 'NONE', *, *, #12268, .T. ) ;
#922=CARTESIAN_POINT ( 'NONE',  ( -16.07504053214564976, -21.67928428602438018, 58.35755945890704766 ) ) ;
#923=CARTESIAN_POINT ( 'NONE',  ( -19.08829560879351206, -7.958403603969639306, 63.73089209831277202 ) ) ;
#925=CARTESIAN_POINT ( 'NONE',  ( -24.64621740481133116, -16.83181165628401033, 54.27966884056654351 ) ) ;
#926=ADVANCED_FACE ( 'NONE', ( #44984 ), #7796, .T. ) ;
#928=CARTESIAN_POINT ( 'NONE',  ( -14.36817892824948473, -8.455618309860652104, 67.54503025475186462 ) ) ;
#929=CARTESIAN_POINT ( 'NONE',  ( -10.60176812795113932, -13.01736012961602817, 64.26835978638996494 ) ) ;
#930=CARTESIAN_POINT ( 'NONE',  ( -24.17299910500858928, -11.65368927744445315, 59.64269123915968152 ) ) ;
#931=ORIENTED_EDGE ( 'NONE', *, *, #15875, .F. ) ;
#932=VECTOR ( 'NONE', #39496, 1000.000000000000114 ) ;
#934=CARTESIAN_POINT ( 'NONE',  ( -17.43166475307565122, -7.359124600834268115, 67.13544264266099049 ) ) ;
#936=VERTEX_POINT ( 'NONE', #44482 ) ;
#937=CARTESIAN_POINT ( 'NONE',  ( -18.92057448382017526, -7.919863665830077615, 67.20071783788056052 ) ) ;
#938=ORIENTED_EDGE ( 'NONE', *, *, #45364, .F. ) ;
#942=CARTESIAN_POINT ( 'NONE',  ( -16.29760782986628342, -22.17363506107604110, 61.87072849596245305 ) ) ;
#943=CARTESIAN_POINT ( 'NONE',  ( -15.99215991861623110, -7.498114659224332179, 63.82011026836138967 ) ) ;
#944=CARTESIAN_POINT ( 'NONE',  ( -14.21141923640507443, -8.087321911531361707, 67.42008472022612864 ) ) ;
#945=ADVANCED_FACE ( 'NONE', ( #22813 ), #37804, .T. ) ;
#946=VERTEX_POINT ( 'NONE', #25750 ) ;
#952=ORIENTED_EDGE ( 'NONE', *, *, #23272, .T. ) ;
#955=CARTESIAN_POINT ( 'NONE',  ( -11.39216336840796373, -18.45920852072106300, 61.29182966166492719 ) ) ;
#956=VERTEX_POINT ( 'NONE', #29693 ) ;
#961=EDGE_CURVE ( 'NONE', #37207, #21586, #14391, .T. ) ;
#964=( BOUNDED_CURVE ( )  B_SPLINE_CURVE ( 3, ( #31982, #46997, #18156, #19569 ),
 .UNSPECIFIED., .F., .F. ) 
 B_SPLINE_CURVE_WITH_KNOTS ( ( 4, 4 ),
 ( 0.4074455897393637893, 0.5000000000000000000 ),
 .UNSPECIFIED. ) 
 CURVE ( )  GEOMETRIC_REPRESENTATION_ITEM ( )  RATIONAL_B_SPLINE_CURVE ( ( 0.6983129098261027234, 0.7760317562606876551, 0.8765941196519810852, 0.9999999999999698019 ) ) 
 REPRESENTATION_ITEM ( '' )  );
#965=CARTESIAN_POINT ( 'NONE',  ( -12.16393509928502503, -9.533249887265045075, 57.25082014697580490 ) ) ;
#967=CARTESIAN_POINT ( 'NONE',  ( -11.39127492490111315, -11.16067319722467843, 60.69357916181100876 ) ) ;
#968=ORIENTED_EDGE ( 'NONE', *, *, #7075, .F. ) ;
#971=CARTESIAN_POINT ( 'NONE',  ( -11.85857808612905195, -10.56289456917895642, 74.72268611605147726 ) ) ;
#972=CARTESIAN_POINT ( 'NONE',  ( -17.22941483204795432, -7.758281381365547347, 74.05198360041919159 ) ) ;
#973=CARTESIAN_POINT ( 'NONE',  ( -19.05639634586962572, -7.942579960324152921, 70.51501210008177623 ) ) ;
#974=ADVANCED_FACE ( 'NONE', ( #10732 ), #37298, .T. ) ;
#975=( BOUNDED_SURFACE ( )  B_SPLINE_SURFACE ( 3, 1, ( 
 ( #15684, #37861 ),
 ( #45763, #35130 ),
 ( #8324, #12015 ),
 ( #1395, #19394 ),
 ( #42293, #16414 ),
 ( #42050, #15927 ),
 ( #30498, #4874 ) ),
 .UNSPECIFIED., .T., .F., .F. ) 
 B_SPLINE_SURFACE_WITH_KNOTS ( ( 4, 3, 4 ),
 ( 2, 2 ),
 ( 0.000000000000000000, 0.5000000000000000000, 1.000000000000000000 ),
 ( 0.000000000000000000, 1.000000000000000000 ),
 .UNSPECIFIED. ) 
 GEOMETRIC_REPRESENTATION_ITEM ( )  RATIONAL_B_SPLINE_SURFACE ( (
 ( 1.000000000000000000, 1.000000000000000000),
 ( 0.3333333333333335369, 0.3333333333333330373),
 ( 0.3333333333333335369, 0.3333333333333330373),
 ( 1.000000000000000000, 1.000000000000000000),
 ( 0.3333333333333333703, 0.3333333333333333703),
 ( 0.3333333333333333703, 0.3333333333333333703),
 ( 1.000000000000000000, 1.000000000000000000) ) ) 
 REPRESENTATION_ITEM ( '' )  SURFACE ( )  );
#976=ORIENTED_EDGE ( 'NONE', *, *, #26378, .F. ) ;
#977=EDGE_CURVE ( 'NONE', #20038, #21955, #394, .T. ) ;
#980=FACE_OUTER_BOUND ( 'NONE', #44154, .T. ) ;
#981=CYLINDRICAL_SURFACE ( 'NONE', #44959, 0.1499999999999991063 ) ;
#983=B_SPLINE_CURVE_WITH_KNOTS ( 'NONE', 3,
 ( #47931, #10510, #28251, #25516, #40529, #21823, #43277, #9548, #5844, #20858 ),
 .UNSPECIFIED., .F., .F.,
 ( 4, 2, 2, 2, 4 ),
 ( 0.000000000000000000, 0.2500000000000000000, 0.5000000000000000000, 0.7500000000000000000, 1.000000000000000000 ),
 .UNSPECIFIED. ) ;
#984=ADVANCED_FACE ( 'NONE', ( #19099 ), #165, .T. ) ;
#985=ORIENTED_EDGE ( 'NONE', *, *, #33172, .T. ) ;
#986=CARTESIAN_POINT ( 'NONE',  ( -13.11378338524245812, -9.291623327890567552, 71.03852466965894052 ) ) ;
#987=( BOUNDED_CURVE ( )  B_SPLINE_CURVE ( 3, ( #24182, #17000, #25146, #42894 ),
 .UNSPECIFIED., .F., .F. ) 
 B_SPLINE_CURVE_WITH_KNOTS ( ( 4, 4 ),
 ( 0.5000000000000000000, 0.9074455897393701731 ),
 .UNSPECIFIED. ) 
 CURVE ( )  GEOMETRIC_REPRESENTATION_ITEM ( )  RATIONAL_B_SPLINE_CURVE ( ( 0.9999999999999765743, 0.4567392136813188119, 0.3561768502900417022, 0.6983129098261199319 ) ) 
 REPRESENTATION_ITEM ( '' )  );
#989=EDGE_LOOP ( 'NONE', ( #28713, #41829, #48612, #29103, #37851 ) ) ;
#990=CARTESIAN_POINT ( 'NONE',  ( -14.01118748589247964, -10.49619482288619565, 54.07175714974879099 ) ) ;
#991=CARTESIAN_POINT ( 'NONE',  ( -22.20320197231171733, -19.92390356480266433, 66.00421731406686376 ) ) ;
#994=ORIENTED_EDGE ( 'NONE', *, *, #18757, .T. ) ;
#995=DIRECTION ( 'NONE',  ( 1.069446452691264255E-06, -1.103879811633194674E-06, 0.9999999999988189447 ) ) ;
#996=CARTESIAN_POINT ( 'NONE',  ( -20.84119837601463487, -20.97572066283330727, 62.26471400470415318 ) ) ;
#997=VERTEX_POINT ( 'NONE', #15378 ) ;
#998=CARTESIAN_POINT ( 'NONE',  ( -24.85359104829803911, -14.25571788259268402, 69.76779960783916579 ) ) ;
#999=DIRECTION ( 'NONE',  ( -1.011289380576387089E-05, 7.260693218591336108E-06, -0.9999999999225059888 ) ) ;
#1001=CARTESIAN_POINT ( 'NONE',  ( -17.59048621110443023, -21.80850830133927687, 58.47723572191701891 ) ) ;
#1002=CARTESIAN_POINT ( 'NONE',  ( -22.26145519751894852, -9.143288655575599222, 59.82196963377553089 ) ) ;
#1003=CARTESIAN_POINT ( 'NONE',  ( -13.40837994833333546, -8.534074693662999422, 57.16306079917540472 ) ) ;
#1004=ORIENTED_EDGE ( 'NONE', *, *, #35816, .F. ) ;
#1005=CARTESIAN_POINT ( 'NONE',  ( -19.15013611399638904, -21.59351999776188080, 58.80890875055925449 ) ) ;
#1008=EDGE_CURVE ( 'NONE', #1447, #6775, #44248, .T. ) ;
#1009=CARTESIAN_POINT ( 'NONE',  ( -22.47245519635065492, -19.73066437834766873, 72.65872596779033188 ) ) ;
#1010=CARTESIAN_POINT ( 'NONE',  ( -20.78261395438590853, -20.95102100293006941, 62.11471427793520661 ) ) ;
#1011=ORIENTED_EDGE ( 'NONE', *, *, #31859, .F. ) ;
#1012=VERTEX_POINT ( 'NONE', #18856 ) ;
#1013=EDGE_CURVE ( 'NONE', #39358, #7816, #7643, .T. ) ;
#1015=FACE_OUTER_BOUND ( 'NONE', #21866, .T. ) ;
#1016=EDGE_LOOP ( 'NONE', ( #44504, #29127 ) ) ;
#1017=CARTESIAN_POINT ( 'NONE',  ( -10.38423141237398895, -15.23952324640539935, 57.98281521108167880 ) ) ;
#1018=FACE_OUTER_BOUND ( 'NONE', #3445, .T. ) ;
#1020=CARTESIAN_POINT ( 'NONE',  ( -24.73624204583532205, -16.23579025085892269, 62.69305037171274364 ) ) ;
#1021=CARTESIAN_POINT ( 'NONE',  ( -23.08280660609100110, -10.60377317445056811, 59.61675562601556067 ) ) ;
#1022=CARTESIAN_POINT ( 'NONE',  ( -12.22219652746809793, -10.12507141233243502, 60.78591508415431832 ) ) ;
#1023=CARTESIAN_POINT ( 'NONE',  ( -14.09914604623946488, -8.649277798895779412, 74.19954655170327840 ) ) ;
#1024=ORIENTED_EDGE ( 'NONE', *, *, #31564, .F. ) ;
#1027=CARTESIAN_POINT ( 'NONE',  ( -23.05195072219661512, -10.55808160950470409, 63.48674805708738234 ) ) ;
#1028=FACE_OUTER_BOUND ( 'NONE', #36065, .T. ) ;
#1029=CARTESIAN_POINT ( 'NONE',  ( -12.83007325466668114, -20.09077588727113550, 72.10653676829758751 ) ) ;
#1030=EDGE_CURVE ( 'NONE', #42456, #13644, #12331, .T. ) ;
#1033=ORIENTED_EDGE ( 'NONE', *, *, #19899, .F. ) ;
#1034=CARTESIAN_POINT ( 'NONE',  ( -20.04849592361258104, -21.35284569240296548, 72.69006679631316103 ) ) ;
#1035=ORIENTED_EDGE ( 'NONE', *, *, #3687, .F. ) ;
#1036=EDGE_CURVE ( 'NONE', #25854, #1499, #47567, .T. ) ;
#1039=CARTESIAN_POINT ( 'NONE',  ( -11.21695167451617792, -18.92928555840075688, 64.79061121450172323 ) ) ;
#1040=CARTESIAN_POINT ( 'NONE',  ( -24.09512891293812586, -12.68832253202152671, 70.05777624906316703 ) ) ;
#1041=ORIENTED_EDGE ( 'NONE', *, *, #14345, .F. ) ;
#1042=DIRECTION ( 'NONE',  ( -5.731567514496413899E-31, -1.020425574103664789E-16, -1.000000000000000000 ) ) ;
#1044=EDGE_LOOP ( 'NONE', ( #8822, #28243, #26604, #26293, #18594 ) ) ;
#1045=CARTESIAN_POINT ( 'NONE',  ( -17.77205755976807566, -21.85076284820492987, 58.69993615557697098 ) ) ;
#1046=CARTESIAN_POINT ( 'NONE',  ( -19.17604249790256077, -21.63836284480991878, 58.53979515915469278 ) ) ;
#1047=ORIENTED_EDGE ( 'NONE', *, *, #28049, .F. ) ;
#1048=CARTESIAN_POINT ( 'NONE',  ( -20.11870507851999079, -21.33255209822014820, 69.09049654866474555 ) ) ;
#1049=CARTESIAN_POINT ( 'NONE',  ( -13.38554957454228500, -8.548802447020154460, 57.11967752468037673 ) ) ;
#1050=ORIENTED_EDGE ( 'NONE', *, *, #3461, .T. ) ;
#1051=CARTESIAN_POINT ( 'NONE',  ( -11.89179040387956832, -10.43929601004734664, 70.96893105543333036 ) ) ;
#1055=CARTESIAN_POINT ( 'NONE',  ( -10.43949455435184603, -13.84896052950683476, 57.46297163929641982 ) ) ;
#1057=CARTESIAN_POINT ( 'NONE',  ( -17.76558202972499245, -21.80099470530900163, 58.40553380166819153 ) ) ;
#1058=CARTESIAN_POINT ( 'NONE',  ( -11.54697730414119228, -10.23050705058286525, 71.10746578893807168 ) ) ;
#1059=CARTESIAN_POINT ( 'NONE',  ( -21.35673258969865174, -10.96416394607318701, 54.07175714974879099 ) ) ;
#1060=DIRECTION ( 'NONE',  ( -0.3478314405900308492, -0.9375570856950864451, 0.000000000000000000 ) ) ;
#1061=CYLINDRICAL_SURFACE ( 'NONE', #12882, 0.1500000000000023259 ) ;
#1063=CARTESIAN_POINT ( 'NONE',  ( -24.31482341358216104, -13.31912415075585088, 59.51267924675325816 ) ) ;
#1064=CARTESIAN_POINT ( 'NONE',  ( -22.14133254371160930, -20.05921860014851532, 69.31850691956374533 ) ) ;
#1066=VERTEX_POINT ( 'NONE', #31148 ) ;
#1067=EDGE_CURVE ( 'NONE', #31867, #31795, #5431, .T. ) ;
#1068=CARTESIAN_POINT ( 'NONE',  ( -21.79028809537168243, -9.273590339475653366, 63.47681654923867711 ) ) ;
#1069=CARTESIAN_POINT ( 'NONE',  ( -24.25171796977671335, -16.35308120058899206, 59.42332432118549690 ) ) ;
#1071=CARTESIAN_POINT ( 'NONE',  ( -15.09544296547830022, -21.46351980780830715, 65.25596681500472585 ) ) ;
#1072=FACE_OUTER_BOUND ( 'NONE', #12499, .T. ) ;
#1073=CARTESIAN_POINT ( 'NONE',  ( -20.27839375093418184, -21.74978099588899028, 54.02222386812612598 ) ) ;
#1074=ORIENTED_EDGE ( 'NONE', *, *, #35715, .T. ) ;
#1075=CARTESIAN_POINT ( 'NONE',  ( -24.41055578522490066, -14.37307875356631648, 66.46827409029781109 ) ) ;
#1076=CARTESIAN_POINT ( 'NONE',  ( -10.04844915070208344, -15.85969764522557668, 64.76417530519553623 ) ) ;
#1077=DIRECTION ( 'NONE',  ( -5.731567514496413899E-31, -1.020425574103664789E-16, -1.000000000000000000 ) ) ;
#1078=ORIENTED_EDGE ( 'NONE', *, *, #40792, .F. ) ;
#1079=VECTOR ( 'NONE', #1783, 1000.000000000000000 ) ;
#1080=CARTESIAN_POINT ( 'NONE',  ( -18.53556552080321751, -22.17591605216722428, 72.40015545304112266 ) ) ;
#1081=CARTESIAN_POINT ( 'NONE',  ( -24.38910862430834570, -17.45374016378893955, 69.57486276871010489 ) ) ;
#1082=CARTESIAN_POINT ( 'NONE',  ( -10.40245588357037043, -14.17414831712846990, 61.20349182037644198 ) ) ;
#1083=CARTESIAN_POINT ( 'NONE',  ( -15.61945779041031201, -7.581001026129836617, 70.86635785818099009 ) ) ;
#1084=B_SPLINE_CURVE_WITH_KNOTS ( 'NONE', 1,
 ( #15887, #15640 ),
 .UNSPECIFIED., .F., .F.,
 ( 2, 2 ),
 ( 0.000000000000000000, 1.000000000000000000 ),
 .UNSPECIFIED. ) ;
#1086=VERTEX_POINT ( 'NONE', #42491 ) ;
#1087=ORIENTED_EDGE ( 'NONE', *, *, #5470, .F. ) ;
#1089=EDGE_CURVE ( 'NONE', #566, #12811, #46892, .T. ) ;
#1090=EDGE_CURVE ( 'NONE', #31795, #26956, #3163, .T. ) ;
#1091=CARTESIAN_POINT ( 'NONE',  ( -10.73979281777117301, -12.56761926564778875, 60.80413345197664654 ) ) ;
#1092=CARTESIAN_POINT ( 'NONE',  ( -23.34884119489251475, -11.08117399487719545, 73.58866568711046341 ) ) ;
#1093=EDGE_CURVE ( 'NONE', #8618, #44086, #38759, .T. ) ;
#1094=EDGE_CURVE ( 'NONE', #2492, #18208, #561, .T. ) ;
#1095=CARTESIAN_POINT ( 'NONE',  ( -23.14423626907140985, -18.93653154422199236, 58.88410448318015256 ) ) ;
#1098=ORIENTED_EDGE ( 'NONE', *, *, #43731, .F. ) ;
#1100=FACE_OUTER_BOUND ( 'NONE', #23068, .T. ) ;
#1103=CARTESIAN_POINT ( 'NONE',  ( -13.37018359880637064, -21.05987222909415735, 61.67679642377481741 ) ) ;
#1105=VERTEX_POINT ( 'NONE', #16362 ) ;
#1106=DIRECTION ( 'NONE',  ( 0.3124635249310678264, 0.8422251632096484641, -0.4393441931380601684 ) ) ;
#1109=CARTESIAN_POINT ( 'NONE',  ( -23.85820194903862657, -17.69173191509663567, 62.48833042115954584 ) ) ;
#1111=CARTESIAN_POINT ( 'NONE',  ( -20.88948204121561503, -21.40431582783964970, 58.82192061885749013 ) ) ;
#1112=CARTESIAN_POINT ( 'NONE',  ( -10.88909980223564666, -11.23174460660519713, 64.32598909751834526 ) ) ;
#1113=( BOUNDED_CURVE ( )  B_SPLINE_CURVE ( 3, ( #40647, #6685, #32776, #6455 ),
 .UNSPECIFIED., .F., .F. ) 
 B_SPLINE_CURVE_WITH_KNOTS ( ( 4, 4 ),
 ( 0.000000000000000000, 0.4074455897393638448 ),
 .UNSPECIFIED. ) 
 CURVE ( )  GEOMETRIC_REPRESENTATION_ITEM ( )  RATIONAL_B_SPLINE_CURVE ( ( 1.000000000000000000, 0.4567392136813325787, 0.3561768502900305444, 0.6983129098260937306 ) ) 
 REPRESENTATION_ITEM ( '' )  );
#1114=FACE_BOUND ( 'NONE', #9980, .T. ) ;
#1116=CARTESIAN_POINT ( 'NONE',  ( -22.05923734882601295, -20.05472318235705131, 62.53439162613685909 ) ) ;
#1119=EDGE_LOOP ( 'NONE', ( #2792, #21677 ) ) ;
#1120=CARTESIAN_POINT ( 'NONE',  ( -7.112004074929013875, -11.66554931205259749, 54.49999999999995026 ) ) ;
#1122=CARTESIAN_POINT ( 'NONE',  ( -20.08692735517319861, -21.76724714254084248, 72.54445348735094967 ) ) ;
#1123=CARTESIAN_POINT ( 'NONE',  ( -16.79037046003568179, -22.23232723477725514, 68.81747882983158604 ) ) ;
#1126=FACE_BOUND ( 'NONE', #38167, .T. ) ;
#1129=ORIENTED_EDGE ( 'NONE', *, *, #22650, .F. ) ;
#1131=FACE_OUTER_BOUND ( 'NONE', #31473, .T. ) ;
#1133=CARTESIAN_POINT ( 'NONE',  ( -21.76676701690912807, -20.36762673175126181, 59.06443059911789106 ) ) ;
#1134=CARTESIAN_POINT ( 'NONE',  ( -10.31379496977684340, -12.58270390103710668, 64.45491433821949556 ) ) ;
#1136=VERTEX_POINT ( 'NONE', #42244 ) ;
#1137=VERTEX_POINT ( 'NONE', #1109 ) ;
#1139=B_SPLINE_CURVE_WITH_KNOTS ( 'NONE', 3,
 ( #28112, #43139, #5725, #9663, #31572, #46605, #12612, #20971, #42669, #35970 ),
 .UNSPECIFIED., .F., .F.,
 ( 4, 2, 2, 2, 4 ),
 ( 0.000000000000000000, 0.2500000000000000000, 0.5000000000000000000, 0.7500000000000000000, 1.000000000000000000 ),
 .UNSPECIFIED. ) ;
#1140=EDGE_CURVE ( 'NONE', #18330, #38687, #43488, .T. ) ;
#1142=CARTESIAN_POINT ( 'NONE',  ( -10.51635438871963579, -15.94466521842666573, 68.26151329549378488 ) ) ;
#1143=CARTESIAN_POINT ( 'NONE',  ( -19.60046948880987117, -21.46228020301366257, 65.76486213989072382 ) ) ;
#1144=ORIENTED_EDGE ( 'NONE', *, *, #15305, .F. ) ;
#1146=B_SPLINE_CURVE_WITH_KNOTS ( 'NONE', 3,
 ( #11930, #13594, #21257, #28153, #25427, #9697, #3003, #21500, #17541, #14065 ),
 .UNSPECIFIED., .F., .F.,
 ( 4, 2, 2, 2, 4 ),
 ( 0.1272669073658299899, 0.2522669073463197353, 0.3772669073268094531, 0.5022669073072967283, 0.6272669072877841145 ),
 .UNSPECIFIED. ) ;
#1147=EDGE_CURVE ( 'NONE', #22754, #16663, #38134, .T. ) ;
#1149=CARTESIAN_POINT ( 'NONE',  ( -13.27770768808251134, -9.107454094634597652, 63.90946529206384241 ) ) ;
#1150=CARTESIAN_POINT ( 'NONE',  ( -12.60165769527841384, -19.96275654529059906, 61.55245915020547898 ) ) ;
#1151=EDGE_CURVE ( 'NONE', #13240, #35848, #24263, .T. ) ;
#1152=B_SPLINE_CURVE_WITH_KNOTS ( 'NONE', 3,
 ( #34203, #26107, #3694, #33459, #11566, #14993, #41123, #37398, #3946, #22408 ),
 .UNSPECIFIED., .F., .F.,
 ( 4, 2, 2, 2, 4 ),
 ( 0.000000000000000000, 0.2500000000000000000, 0.5000000000000000000, 0.7500000000000000000, 1.000000000000000000 ),
 .UNSPECIFIED. ) ;
#1153=CARTESIAN_POINT ( 'NONE',  ( -18.53556552080321751, -22.17591605216722428, 72.40015545304112266 ) ) ;
#1154=EDGE_CURVE ( 'NONE', #38392, #6133, #13214, .T. ) ;
#1155=ORIENTED_EDGE ( 'NONE', *, *, #22793, .F. ) ;
#1158=CARTESIAN_POINT ( 'NONE',  ( -18.15831417771707379, -22.22293841580443186, 65.49532158008852889 ) ) ;
#1159=ORIENTED_EDGE ( 'NONE', *, *, #43377, .F. ) ;
#1161=CARTESIAN_POINT ( 'NONE',  ( -17.43006558257920346, -7.359130651351934560, 67.27685495689534889 ) ) ;
#1162=CARTESIAN_POINT ( 'NONE',  ( -12.35277332135121675, -20.26681466537264242, 68.45162004874669037 ) ) ;
#1163=ORIENTED_EDGE ( 'NONE', *, *, #43106, .T. ) ;
#1165=VERTEX_POINT ( 'NONE', #31647 ) ;
#1166=VECTOR ( 'NONE', #3129, 1000.000000000000114 ) ;
#1167=CARTESIAN_POINT ( 'NONE',  ( -24.30164805153987473, -16.37256343635084477, 63.00817566860099106 ) ) ;
#1169=LINE ( 'NONE', #30984, #35251 ) ;
#1172=DIRECTION ( 'NONE',  ( -0.8324837747691418155, -0.5540494244615011832, 1.585791776141941048E-16 ) ) ;
#1173=DIRECTION ( 'NONE',  ( 0.7841839494287637935, -0.6205284308219133349, 1.653628654373097423E-16 ) ) ;
#1174=VERTEX_POINT ( 'NONE', #40250 ) ;
#1175=CARTESIAN_POINT ( 'NONE',  ( -9.992360566757833240, -14.28769768793135242, 64.58792641534920165 ) ) ;
#1176=CARTESIAN_POINT ( 'NONE',  ( -20.56282556578965881, -8.552218022744439097, 63.61121530278081337 ) ) ;
#1177=CARTESIAN_POINT ( 'NONE',  ( -20.91306683646873310, -8.226686726328479082, 59.99125248244220643 ) ) ;
#1178=CARTESIAN_POINT ( 'NONE',  ( -23.46741973463711872, -19.16603908095663655, 62.53902270128352825 ) ) ;
#1182=ORIENTED_EDGE ( 'NONE', *, *, #7623, .F. ) ;
#1183=ORIENTED_EDGE ( 'NONE', *, *, #16284, .T. ) ;
#1185=CARTESIAN_POINT ( 'NONE',  ( -10.69671328391030229, -11.60805651651419446, 71.24894240167931514 ) ) ;
#1187=( BOUNDED_CURVE ( )  B_SPLINE_CURVE ( 3, ( #39103, #5387, #31961, #47229 ),
 .UNSPECIFIED., .F., .F. ) 
 B_SPLINE_CURVE_WITH_KNOTS ( ( 4, 4 ),
 ( 0.000000000000000000, 0.4074455897393669535 ),
 .UNSPECIFIED. ) 
 CURVE ( )  GEOMETRIC_REPRESENTATION_ITEM ( )  RATIONAL_B_SPLINE_CURVE ( ( 1.000000000000000000, 0.4567392136813300807, 0.3561768502900296007, 0.6983129098260987266 ) ) 
 REPRESENTATION_ITEM ( '' )  );
#1189=CARTESIAN_POINT ( 'NONE',  ( -14.27319436148695431, -8.558459998996717388, 71.02957628730779049 ) ) ;
#1190=EDGE_CURVE ( 'NONE', #8240, #40764, #32130, .T. ) ;
#1191=PLANE ( 'NONE',  #1559 ) ;
#1192=CARTESIAN_POINT ( 'NONE',  ( -18.64436893707341980, -7.459652816704011258, 73.98031072975879852 ) ) ;
#1193=CARTESIAN_POINT ( 'NONE',  ( -12.39637281836977145, -9.867031899960309715, 57.38935535270289279 ) ) ;
#1194=EDGE_LOOP ( 'NONE', ( #42954, #43904 ) ) ;
#1195=ORIENTED_EDGE ( 'NONE', *, *, #20298, .T. ) ;
#1199=CARTESIAN_POINT ( 'NONE',  ( -13.35550522631041837, -8.568183888810063209, 57.15463030501995689 ) ) ;
#1200=CARTESIAN_POINT ( 'NONE',  ( -23.91010245674826251, -17.57297063409389537, 62.75888927877479517 ) ) ;
#1201=AXIS2_PLACEMENT_3D ( 'NONE', #10044, #25064, #40081 ) ;
#1204=AXIS2_PLACEMENT_3D ( 'NONE', #899, #11308, #33434 ) ;
#1205=CARTESIAN_POINT ( 'NONE',  ( -23.49605051889219709, -11.22618518380361330, 73.37665428612797314 ) ) ;
#1208=CARTESIAN_POINT ( 'NONE',  ( -15.83660554694375477, -7.530134340792297820, 67.27973953361981785 ) ) ;
#1209=EDGE_CURVE ( 'NONE', #24622, #36187, #40491, .T. ) ;
#1210=ORIENTED_EDGE ( 'NONE', *, *, #10005, .F. ) ;
#1211=CARTESIAN_POINT ( 'NONE',  ( -22.22370946352282672, -9.111183370010303761, 59.90666632495347699 ) ) ;
#1213=CARTESIAN_POINT ( 'NONE',  ( -24.36028583763659583, -16.11466138999042030, 69.67740616536292464 ) ) ;
#1214=VERTEX_POINT ( 'NONE', #43216 ) ;
#1215=PLANE ( 'NONE',  #24172 ) ;
#1216=EDGE_CURVE ( 'NONE', #24840, #28874, #3510, .T. ) ;
#1217=CARTESIAN_POINT ( 'NONE',  ( -13.85393748347032528, -8.270264590973253505, 74.38449983516251507 ) ) ;
#1218=EDGE_LOOP ( 'NONE', ( #25656, #20939 ) ) ;
#1219=CARTESIAN_POINT ( 'NONE',  ( -23.68696726785515949, -18.84393668709636671, 69.49360751211669651 ) ) ;
#1220=VERTEX_POINT ( 'NONE', #5793 ) ;
#1221=CYLINDRICAL_SURFACE ( 'NONE', #33799, 0.1500000000000061007 ) ;
#1222=CARTESIAN_POINT ( 'NONE',  ( -21.55884032038934350, -8.611816057827914150, 73.78624026056009200 ) ) ;
#1223=VERTEX_POINT ( 'NONE', #13390 ) ;
#1224=CARTESIAN_POINT ( 'NONE',  ( -24.26499744607890818, -17.75976858747020160, 62.65856309191605789 ) ) ;
#1225=CARTESIAN_POINT ( 'NONE',  ( -10.29794926819780088, -12.63594297046838477, 64.40802751477502852 ) ) ;
#1227=CARTESIAN_POINT ( 'NONE',  ( -11.95536787350534169, -10.43947220190359637, 70.96893134409420156 ) ) ;
#1228=( BOUNDED_SURFACE ( )  B_SPLINE_SURFACE ( 3, 1, ( 
 ( #16012, #34743 ),
 ( #46073, #12578 ),
 ( #42386, #27354 ),
 ( #8656, #23682 ),
 ( #43101, #4964 ),
 ( #1977, #9632 ),
 ( #35692, #19973 ) ),
 .UNSPECIFIED., .T., .F., .F. ) 
 B_SPLINE_SURFACE_WITH_KNOTS ( ( 4, 3, 4 ),
 ( 2, 2 ),
 ( 0.000000000000000000, 0.5000000000000000000, 1.000000000000000000 ),
 ( 0.000000000000000000, 1.000000000000000000 ),
 .UNSPECIFIED. ) 
 GEOMETRIC_REPRESENTATION_ITEM ( )  RATIONAL_B_SPLINE_SURFACE ( (
 ( 1.000000000000000000, 1.000000000000000000),
 ( 0.3333333333333335369, 0.3333333333333330373),
 ( 0.3333333333333335369, 0.3333333333333330373),
 ( 1.000000000000000000, 1.000000000000000000),
 ( 0.3333333333333333703, 0.3333333333333333703),
 ( 0.3333333333333333703, 0.3333333333333333703),
 ( 1.000000000000000000, 1.000000000000000000) ) ) 
 REPRESENTATION_ITEM ( '' )  SURFACE ( )  );
#1229=CARTESIAN_POINT ( 'NONE',  ( -23.85748962928175132, -11.92509172808648543, 59.49707787073156595 ) ) ;
#1232=CARTESIAN_POINT ( 'NONE',  ( -23.89706228095030482, -17.47391663821368724, 62.66464254354016106 ) ) ;
#1233=CARTESIAN_POINT ( 'NONE',  ( -17.13503149044196761, -7.764836982087094164, 70.77563787455143540 ) ) ;
#1234=VECTOR ( 'NONE', #9390, 1000.000000000000114 ) ;
#1235=DIRECTION ( 'NONE',  ( 2.842893050599252319E-07, -1.090087279701840163E-07, 0.9999999999999535927 ) ) ;
#1237=EDGE_LOOP ( 'NONE', ( #17891, #42021, #3568, #14310, #27860 ) ) ;
#1238=ORIENTED_EDGE ( 'NONE', *, *, #42119, .T. ) ;
#1239=DIRECTION ( 'NONE',  ( -0.9930145540378109148, 0.1179919296777755394, 4.526730167978063816E-08 ) ) ;
#1240=CARTESIAN_POINT ( 'NONE',  ( -10.36108929241354382, -12.43876823780533947, 60.93820193749152025 ) ) ;
#1242=CARTESIAN_POINT ( 'NONE',  ( -24.32752796592761158, -15.96791130369872391, 66.06324927019940674 ) ) ;
#1243=CARTESIAN_POINT ( 'NONE',  ( -15.73882891167430564, -7.552148466825388873, 67.30040598401383534 ) ) ;
#1244=CARTESIAN_POINT ( 'NONE',  ( -20.75918756122348441, -8.147305293919229641, 63.42626095967343502 ) ) ;
#1247=CARTESIAN_POINT ( 'NONE',  ( -10.60635910294346651, -17.81289749453643978, 71.82364097624930821 ) ) ;
#1249=( BOUNDED_CURVE ( )  B_SPLINE_CURVE ( 3, ( #38551, #45061, #26087, #37376 ),
 .UNSPECIFIED., .F., .F. ) 
 B_SPLINE_CURVE_WITH_KNOTS ( ( 4, 4 ),
 ( 0.000000000000000000, 0.4074455897393611248 ),
 .UNSPECIFIED. ) 
 CURVE ( )  GEOMETRIC_REPRESENTATION_ITEM ( )  RATIONAL_B_SPLINE_CURVE ( ( 1.000000000000000000, 0.4567392136813308023, 0.3561768502900298783, 0.6983129098260971723 ) ) 
 REPRESENTATION_ITEM ( '' )  );
#1250=CARTESIAN_POINT ( 'NONE',  ( -19.41474593944376537, -21.52019035999878938, 61.99503644832097393 ) ) ;
#1251=VERTEX_POINT ( 'NONE', #9961 ) ;
#1254=CARTESIAN_POINT ( 'NONE',  ( -10.44916082259176093, -15.83527127794237543, 64.80771589743309846 ) ) ;
#1255=CARTESIAN_POINT ( 'NONE',  ( -13.87409053989354923, -20.84236645762476314, 68.45625181054862196 ) ) ;
#1256=CARTESIAN_POINT ( 'NONE',  ( -11.86732220369407997, -9.846751984446582284, 64.28560238571537866 ) ) ;
#1257=B_SPLINE_CURVE_WITH_KNOTS ( 'NONE', 1,
 ( #34397, #692 ),
 .UNSPECIFIED., .F., .F.,
 ( 2, 2 ),
 ( 0.000000000000000000, 1.000000000000000000 ),
 .UNSPECIFIED. ) ;
#1258=ADVANCED_FACE ( 'NONE', ( #24981 ), #10468, .T. ) ;
#1259=ORIENTED_EDGE ( 'NONE', *, *, #41275, .F. ) ;
#1260=VERTEX_POINT ( 'NONE', #26196 ) ;
#1262=ORIENTED_EDGE ( 'NONE', *, *, #42956, .T. ) ;
#1263=DIRECTION ( 'NONE',  ( 0.1675476790616363121, -0.9858639740050647582, 1.006000811662237932E-16 ) ) ;
#1264=CARTESIAN_POINT ( 'NONE',  ( -10.99225178418778448, -18.56881356696312579, 57.91376274275113900 ) ) ;
#1270=VERTEX_POINT ( 'NONE', #37243 ) ;
#1272=CARTESIAN_POINT ( 'NONE',  ( -15.96549791049196543, -7.503336649694742455, 63.77672698436073517 ) ) ;
#1273=EDGE_CURVE ( 'NONE', #48456, #39905, #41114, .T. ) ;
#1274=CARTESIAN_POINT ( 'NONE',  ( -23.77826927976139970, -17.74977700416402726, 62.58433988291946548 ) ) ;
#1277=CARTESIAN_POINT ( 'NONE',  ( -17.59331747086620368, -7.761237804118462869, 63.85057029381062677 ) ) ;
#1278=ORIENTED_EDGE ( 'NONE', *, *, #12418, .F. ) ;
#1279=CARTESIAN_POINT ( 'NONE',  ( -22.17130234749883044, -20.55096496926394778, 58.87947491310501391 ) ) ;
#1280=CARTESIAN_POINT ( 'NONE',  ( -19.43748438392636402, -21.56872497219108098, 58.41018533341049590 ) ) ;
#1283=CARTESIAN_POINT ( 'NONE',  ( -22.22619359738691003, -20.50513629785891823, 58.94938195453792673 ) ) ;
#1288=CARTESIAN_POINT ( 'NONE',  ( -20.50877865959810364, -8.469702366710405883, 63.60561728082600297 ) ) ;
#1290=CARTESIAN_POINT ( 'NONE',  ( -14.42683419600289163, -8.428067575814653267, 67.55975083869262221 ) ) ;
#1291=CARTESIAN_POINT ( 'NONE',  ( -13.15543723850287172, -20.91502918201612005, 58.19650074752242830 ) ) ;
#1292=DIRECTION ( 'NONE',  ( 0.2573866790907599622, 0.9663084897829603559, 6.714855467380900338E-08 ) ) ;
#1293=ADVANCED_FACE ( 'NONE', ( #3040 ), #14576, .T. ) ;
#1294=EDGE_CURVE ( 'NONE', #9944, #13421, #17053, .T. ) ;
#1296=EDGE_LOOP ( 'NONE', ( #29061, #23387 ) ) ;
#1297=CARTESIAN_POINT ( 'NONE',  ( -15.70730708645226237, -24.91091750872855215, 53.49999999999995026 ) ) ;
#1299=EDGE_LOOP ( 'NONE', ( #12670, #21956, #20899, #18516 ) ) ;
#1301=CARTESIAN_POINT ( 'NONE',  ( -14.13242279744181573, -8.574497162196568212, 74.21426705364891063 ) ) ;
#1302=CARTESIAN_POINT ( 'NONE',  ( -21.17484060445739757, -20.78220707328100403, 72.93935319279944451 ) ) ;
#1303=CARTESIAN_POINT ( 'NONE',  ( -12.68381388925888587, -19.95990997655619381, 68.63657438305759229 ) ) ;
#1305=ORIENTED_EDGE ( 'NONE', *, *, #4285, .F. ) ;
#1308=CARTESIAN_POINT ( 'NONE',  ( -20.66848101912799862, -8.549761622307149977, 60.12653141481577990 ) ) ;
#1309=CARTESIAN_POINT ( 'NONE',  ( -14.54176566789882585, -21.67913831930545854, 58.28122448549703449 ) ) ;
#1310=ORIENTED_EDGE ( 'NONE', *, *, #609, .T. ) ;
#1311=CARTESIAN_POINT ( 'NONE',  ( -18.56068362409587280, -22.17200289566820715, 72.48522146388405929 ) ) ;
#1312=CARTESIAN_POINT ( 'NONE',  ( -24.56076101444288184, -12.67091080028054684, 69.95055769627768427 ) ) ;
#1313=CARTESIAN_POINT ( 'NONE',  ( -21.71949691563504459, -8.721965781586035860, 70.26985989995344539 ) ) ;
#1314=B_SPLINE_CURVE_WITH_KNOTS ( 'NONE', 3,
 ( #34476, #30573, #38411, #45109, #4700, #8645, #15024, #1005, #34732, #4450 ),
 .UNSPECIFIED., .F., .F.,
 ( 4, 2, 2, 2, 4 ),
 ( 0.000000000000000000, 0.2500000000000000000, 0.5000000000000000000, 0.7500000000000000000, 1.000000000000000000 ),
 .UNSPECIFIED. ) ;
#1316=ORIENTED_EDGE ( 'NONE', *, *, #11587, .F. ) ;
#1317=VERTEX_POINT ( 'NONE', #18540 ) ;
#1319=EDGE_CURVE ( 'NONE', #38388, #48213, #47870, .T. ) ;
#1320=LINE ( 'NONE', #16332, #34267 ) ;
#1321=CARTESIAN_POINT ( 'NONE',  ( -19.02055866782680482, -21.67977764378408878, 58.61687627430667646 ) ) ;
#1322=ADVANCED_FACE ( 'NONE', ( #14104 ), #48109, .T. ) ;
#1324=CARTESIAN_POINT ( 'NONE',  ( -10.21764062494887781, -12.91954801228597915, 67.92327636273336111 ) ) ;
#1325=CARTESIAN_POINT ( 'NONE',  ( -9.985760891864103428, -14.37924521898145258, 68.04455407903930109 ) ) ;
#1326=CARTESIAN_POINT ( 'NONE',  ( -24.23356459391621343, -17.83169477672529624, 62.65173719855710033 ) ) ;
#1327=ORIENTED_EDGE ( 'NONE', *, *, #34215, .T. ) ;
#1328=CARTESIAN_POINT ( 'NONE',  ( -21.95217610637629946, -9.395202297576263462, 66.80583047767832738 ) ) ;
#1334=DIRECTION ( 'NONE',  ( -0.2479245821708770392, -0.9687793358424796608, -2.626836608334273943E-18 ) ) ;
#1335=ORIENTED_EDGE ( 'NONE', *, *, #12126, .T. ) ;
#1336=CARTESIAN_POINT ( 'NONE',  ( -10.90759852523040330, -17.49952041063523467, 68.09721944423131390 ) ) ;
#1339=DIRECTION ( 'NONE',  ( -0.04108628546905146450, -0.9991556020692451412, 1.019563928860402566E-16 ) ) ;
#1340=CARTESIAN_POINT ( 'NONE',  ( -24.46752114747617313, -17.23684389422572849, 72.99061869212614795 ) ) ;
#1341=ORIENTED_EDGE ( 'NONE', *, *, #15090, .T. ) ;
#1342=FACE_OUTER_BOUND ( 'NONE', #17900, .T. ) ;
#1343=CARTESIAN_POINT ( 'NONE',  ( -20.54031095723443556, -8.042250736733803862, 66.93104081865082833 ) ) ;
#1344=CARTESIAN_POINT ( 'NONE',  ( -10.92380316157302467, -11.16921865325121388, 64.25607897268513113 ) ) ;
#1345=ADVANCED_FACE ( 'NONE', ( #6990 ), #22113, .T. ) ;
#1348=B_SPLINE_CURVE_WITH_KNOTS ( 'NONE', 3,
 ( #18275, #25673, #13843, #13610, #33280, #2554, #47612, #7228, #6726, #32583 ),
 .UNSPECIFIED., .F., .F.,
 ( 4, 2, 2, 2, 4 ),
 ( 0.000000000000000000, 0.2500000000000000000, 0.5000000000000000000, 0.7500000000000000000, 1.000000000000000000 ),
 .UNSPECIFIED. ) ;
#1352=CARTESIAN_POINT ( 'NONE',  ( -14.21975182572090901, -8.525335417369671376, 67.25975088330713447 ) ) ;
#1354=ORIENTED_EDGE ( 'NONE', *, *, #2508, .T. ) ;
#1355=DIRECTION ( 'NONE',  ( 0.8788484374452886216, -0.3260506722428096471, 0.3483050145059451985 ) ) ;
#1356=VERTEX_POINT ( 'NONE', #45397 ) ;
#1357=CARTESIAN_POINT ( 'NONE',  ( -11.21157628577468657, -11.58358644131346082, 67.61864608155907774 ) ) ;
#1358=CARTESIAN_POINT ( 'NONE',  ( -14.80624607021532135, -8.317144234858641738, 60.31996281969095719 ) ) ;
#1360=CARTESIAN_POINT ( 'NONE',  ( -23.89200480383413350, -11.11192299349349533, 70.07706151945906470 ) ) ;
#1362=FACE_BOUND ( 'NONE', #14356, .T. ) ;
#1364=ORIENTED_EDGE ( 'NONE', *, *, #30212, .F. ) ;
#1365=VERTEX_POINT ( 'NONE', #1059 ) ;
#1366=CARTESIAN_POINT ( 'NONE',  ( -10.02210521578421520, -15.65432817399831045, 61.29434977362033976 ) ) ;
#1368=( BOUNDED_SURFACE ( )  B_SPLINE_SURFACE ( 3, 1, ( 
 ( #11356, #10627 ),
 ( #29339, #10866 ),
 ( #41388, #7191 ),
 ( #6689, #36689 ),
 ( #22198, #7680 ),
 ( #15025, #14045 ),
 ( #37185, #18481 ) ),
 .UNSPECIFIED., .T., .F., .F. ) 
 B_SPLINE_SURFACE_WITH_KNOTS ( ( 4, 3, 4 ),
 ( 2, 2 ),
 ( 0.000000000000000000, 0.5000000000000000000, 1.000000000000000000 ),
 ( 0.000000000000000000, 1.000000000000000000 ),
 .UNSPECIFIED. ) 
 GEOMETRIC_REPRESENTATION_ITEM ( )  RATIONAL_B_SPLINE_SURFACE ( (
 ( 1.000000000000000000, 1.000000000000000000),
 ( 0.3333333333333335369, 0.3333333333333330373),
 ( 0.3333333333333335369, 0.3333333333333330373),
 ( 1.000000000000000000, 1.000000000000000000),
 ( 0.3333333333333333703, 0.3333333333333333703),
 ( 0.3333333333333333703, 0.3333333333333333703),
 ( 1.000000000000000000, 1.000000000000000000) ) ) 
 REPRESENTATION_ITEM ( '' )  SURFACE ( )  );
#1369=CARTESIAN_POINT ( 'NONE',  ( -21.30260081908322078, -8.981780046862946065, 73.60128699524366880 ) ) ;
#1370=CARTESIAN_POINT ( 'NONE',  ( -10.29339667142563819, -12.65123896477911103, 64.52482037846105811 ) ) ;
#1375=ORIENTED_EDGE ( 'NONE', *, *, #8206, .T. ) ;
#1378=CARTESIAN_POINT ( 'NONE',  ( -22.73618463404748624, -20.03370227938794912, 69.28762739622011679 ) ) ;
#1379=CARTESIAN_POINT ( 'NONE',  ( -21.13453391143521287, -20.81317186429504673, 62.27038425631170782 ) ) ;
#1380=AXIS2_PLACEMENT_3D ( 'NONE', #46005, #19661, #23351 ) ;
#1382=( BOUNDED_CURVE ( )  B_SPLINE_CURVE ( 3, ( #26147, #36954, #36698, #41158 ),
 .UNSPECIFIED., .F., .F. ) 
 B_SPLINE_CURVE_WITH_KNOTS ( ( 4, 4 ),
 ( 1.570796326794896780, 1.780235837034217283 ),
 .UNSPECIFIED. ) 
 CURVE ( )  GEOMETRIC_REPRESENTATION_ITEM ( )  RATIONAL_B_SPLINE_CURVE ( ( 1.000000000000000000, 0.9963479302455154896, 0.9963479302455154896, 1.000000000000000000 ) ) 
 REPRESENTATION_ITEM ( '' )  );
#1384=( BOUNDED_CURVE ( )  B_SPLINE_CURVE ( 3, ( #40696, #6976, #39986, #29140 ),
 .UNSPECIFIED., .F., .F. ) 
 B_SPLINE_CURVE_WITH_KNOTS ( ( 4, 4 ),
 ( 0.4074455897393629566, 0.5000000000000000000 ),
 .UNSPECIFIED. ) 
 CURVE ( )  GEOMETRIC_REPRESENTATION_ITEM ( )  RATIONAL_B_SPLINE_CURVE ( ( 0.6983129098260889567, 0.7760317562606786623, 0.8765941196519776435, 0.9999999999999744649 ) ) 
 REPRESENTATION_ITEM ( '' )  );
#1385=VECTOR ( 'NONE', #24930, 1000.000000000000227 ) ;
#1386=ORIENTED_EDGE ( 'NONE', *, *, #25635, .F. ) ;
#1387=CARTESIAN_POINT ( 'NONE',  ( -14.72722737765066725, -21.75407789377580059, 61.81413171700139486 ) ) ;
#1388=CARTESIAN_POINT ( 'NONE',  ( -12.00744322407076226, -19.92521668911118482, 61.58333889064303435 ) ) ;
#1389=DIRECTION ( 'NONE',  ( -1.198821490631147214E-05, 1.588017923320057101E-05, -0.9999999998020512315 ) ) ;
#1390=ORIENTED_EDGE ( 'NONE', *, *, #13785, .F. ) ;
#1392=( BOUNDED_CURVE ( )  B_SPLINE_CURVE ( 3, ( #29079, #29560, #17975, #40635 ),
 .UNSPECIFIED., .F., .F. ) 
 B_SPLINE_CURVE_WITH_KNOTS ( ( 4, 4 ),
 ( 0.000000000000000000, 0.4074455897393638448 ),
 .UNSPECIFIED. ) 
 CURVE ( )  GEOMETRIC_REPRESENTATION_ITEM ( )  RATIONAL_B_SPLINE_CURVE ( ( 1.000000000000000000, 0.4567392136813337444, 0.3561768502900309330, 0.6983129098260915102 ) ) 
 REPRESENTATION_ITEM ( '' )  );
#1393=CARTESIAN_POINT ( 'NONE',  ( -22.75144419618436586, -9.600271701911582412, 73.59505825258622735 ) ) ;
#1395=CARTESIAN_POINT ( 'NONE',  ( -12.45873566688478107, -9.804017486950373339, 57.10407583662104258 ) ) ;
#1396=ORIENTED_EDGE ( 'NONE', *, *, #19094, .T. ) ;
#1398=CARTESIAN_POINT ( 'NONE',  ( -10.43905172760979028, -15.29054532034250968, 57.67865882576857928 ) ) ;
#1399=B_SPLINE_CURVE_WITH_KNOTS ( 'NONE', 1,
 ( #10508, #44486 ),
 .UNSPECIFIED., .F., .F.,
 ( 2, 2 ),
 ( 0.000000000000000000, 1.000000000000000000 ),
 .UNSPECIFIED. ) ;
#1402=ORIENTED_EDGE ( 'NONE', *, *, #48076, .F. ) ;
#1403=CARTESIAN_POINT ( 'NONE',  ( -10.40245588357037043, -14.17414831712846990, 61.20349182037644198 ) ) ;
#1405=VECTOR ( 'NONE', #20685, 1000.000000000000114 ) ;
#1406=VERTEX_POINT ( 'NONE', #42678 ) ;
#1407=CARTESIAN_POINT ( 'NONE',  ( -19.15875595501757545, -7.563798684503558967, 63.56942691188406513 ) ) ;
#1408=CARTESIAN_POINT ( 'NONE',  ( -16.36003348549149550, -21.72797215718117414, 61.75568179790091961 ) ) ;
#1409=B_SPLINE_CURVE_WITH_KNOTS ( 'NONE', 3,
 ( #19579, #27449, #16355, #8039, #38033, #31387, #42236, #8264, #34336, #624 ),
 .UNSPECIFIED., .F., .F.,
 ( 4, 2, 2, 2, 4 ),
 ( 0.1272669073658067862, 0.2522669073462858735, 0.3772669073267650441, 0.5022669073072441037, 0.6272669072877232743 ),
 .UNSPECIFIED. ) ;
#1411=ADVANCED_FACE ( 'NONE', ( #41942 ), #27138, .T. ) ;
#1412=CARTESIAN_POINT ( 'NONE',  ( -16.43749525924751964, -22.19434601430465293, 61.86912739712975906 ) ) ;
#1413=CARTESIAN_POINT ( 'NONE',  ( -24.25757938109993717, -13.28409109838451663, 62.94337370252653585 ) ) ;
#1415=ORIENTED_EDGE ( 'NONE', *, *, #28603, .T. ) ;
#1416=CARTESIAN_POINT ( 'NONE',  ( -11.06939607882469190, -17.86905163984256006, 71.45229597776977926 ) ) ;
#1419=CARTESIAN_POINT ( 'NONE',  ( -10.46944733747312917, -15.96661384539355133, 67.99239968927004441 ) ) ;
#1421=CARTESIAN_POINT ( 'NONE',  ( -23.38410589725464916, -10.33907962427212190, 59.71708035543083071 ) ) ;
#1425=ORIENTED_EDGE ( 'NONE', *, *, #13096, .T. ) ;
#1427=ADVANCED_FACE ( 'NONE', ( #30872 ), #32174, .T. ) ;
#1429=CARTESIAN_POINT ( 'NONE',  ( -19.85889901765038346, -21.37233916515964438, 69.21353063550283480 ) ) ;
#1433=CARTESIAN_POINT ( 'NONE',  ( -18.75025350711597483, -7.885019284943789231, 70.37068061249377138 ) ) ;
#1434=CARTESIAN_POINT ( 'NONE',  ( -23.55661029900229053, -18.29303667177271464, 72.64879359478229048 ) ) ;
#1436=CARTESIAN_POINT ( 'NONE',  ( -11.19706266256277694, -11.50303319689152914, 67.63336710488009373 ) ) ;
#1437=VERTEX_POINT ( 'NONE', #28614 ) ;
#1439=DIRECTION ( 'NONE',  ( -0.9959323210854038599, 0.09010444948746665350, 2.601165157765156148E-08 ) ) ;
#1440=ADVANCED_FACE ( 'NONE', ( #20254 ), #9182, .T. ) ;
#1442=CARTESIAN_POINT ( 'NONE',  ( -22.02472224376031562, -20.08502103662938865, 58.95546057814475205 ) ) ;
#1444=CARTESIAN_POINT ( 'NONE',  ( -18.69688219364054049, -7.467975623574482746, 70.48412626434020467 ) ) ;
#1446=AXIS2_PLACEMENT_3D ( 'NONE', #48714, #34408, #463 ) ;
#1447=VERTEX_POINT ( 'NONE', #24199 ) ;
#1448=CARTESIAN_POINT ( 'NONE',  ( -12.23301264461619553, -10.03852782535897958, 60.84446034103241630 ) ) ;
#1449=CARTESIAN_POINT ( 'NONE',  ( -23.78758865751629514, -10.93498413477609255, 73.40547355347567304 ) ) ;
#1451=CARTESIAN_POINT ( 'NONE',  ( -13.88719209496301943, -21.36615830865247645, 72.11881843497792488 ) ) ;
#1452=AXIS2_PLACEMENT_3D ( 'NONE', #39269, #42964, #17079 ) ;
#1454=CARTESIAN_POINT ( 'NONE',  ( -24.44689184067228638, -14.18710713894228093, 69.93803194250310185 ) ) ;
#1456=EDGE_LOOP ( 'NONE', ( #20244, #40710 ) ) ;
#1457=CARTESIAN_POINT ( 'NONE',  ( -22.62555253132729050, -20.14304347834919540, 69.33564472231955733 ) ) ;
#1458=CARTESIAN_POINT ( 'NONE',  ( -13.91686182480500200, -8.236299899141551251, 74.31459327626868117 ) ) ;
#1459=EDGE_CURVE ( 'NONE', #35558, #25977, #35780, .T. ) ;
#1461=CARTESIAN_POINT ( 'NONE',  ( -10.49786169981450712, -13.78684623552789290, 57.67654978352396000 ) ) ;
#1464=CARTESIAN_POINT ( 'NONE',  ( -10.42407743915653562, -14.83384553516632032, 71.40070817709548123 ) ) ;
#1466=CARTESIAN_POINT ( 'NONE',  ( -10.70566809389435647, -16.94585225683366048, 57.68760548748759476 ) ) ;
#1468=CARTESIAN_POINT ( 'NONE',  ( -21.79028809537168243, -9.273590339475653366, 63.47681654923867711 ) ) ;
#1473=( BOUNDED_CURVE ( )  B_SPLINE_CURVE ( 3, ( #20747, #32073, #35025, #24694 ),
 .UNSPECIFIED., .F., .F. ) 
 B_SPLINE_CURVE_WITH_KNOTS ( ( 4, 4 ),
 ( 0.5000000000000000000, 0.9074455897393608472 ),
 .UNSPECIFIED. ) 
 CURVE ( )  GEOMETRIC_REPRESENTATION_ITEM ( )  RATIONAL_B_SPLINE_CURVE ( ( 0.9999999999999960032, 0.4567392136813388515, 0.3561768502900354849, 0.6983129098260817402 ) ) 
 REPRESENTATION_ITEM ( '' )  );
#1475=CARTESIAN_POINT ( 'NONE',  ( -24.10630238842451689, -12.71861100898961361, 73.35298647045775056 ) ) ;
#1476=CARTESIAN_POINT ( 'NONE',  ( -14.73375663737576247, -21.75657035701089370, 61.75105113489106401 ) ) ;
#1477=ORIENTED_EDGE ( 'NONE', *, *, #13657, .F. ) ;
#1478=CARTESIAN_POINT ( 'NONE',  ( -23.89140331848801679, -17.48778192296385470, 62.70034397296751649 ) ) ;
#1479=AXIS2_PLACEMENT_3D ( 'NONE', #19965, #27346, #5685 ) ;
#1481=CARTESIAN_POINT ( 'NONE',  ( -11.42962537269896117, -10.38539323336976494, 74.62380298385740218 ) ) ;
#1483=CARTESIAN_POINT ( 'NONE',  ( -20.52907107024056188, -8.037074714175183487, 66.88080459870857908 ) ) ;
#1484=CARTESIAN_POINT ( 'NONE',  ( -24.77597654615908240, -16.01465712210608316, 66.25599054112966257 ) ) ;
#1485=ORIENTED_EDGE ( 'NONE', *, *, #10961, .T. ) ;
#1486=ORIENTED_EDGE ( 'NONE', *, *, #25832, .T. ) ;
#1488=CARTESIAN_POINT ( 'NONE',  ( -21.36950980536903444, -9.026885639815656504, 73.60128804931920854 ) ) ;
#1489=CARTESIAN_POINT ( 'NONE',  ( -24.29232374648589854, -16.16102685949518403, 62.89328677060923667 ) ) ;
#1490=ORIENTED_EDGE ( 'NONE', *, *, #35013, .F. ) ;
#1492=CARTESIAN_POINT ( 'NONE',  ( -21.94242186726961208, -9.397052521110282441, 60.00699132926281010 ) ) ;
#1494=CARTESIAN_POINT ( 'NONE',  ( -10.27146132483092522, -12.72493829394020892, 64.39023348442692907 ) ) ;
#1495=EDGE_CURVE ( 'NONE', #25885, #2066, #44599, .T. ) ;
#1496=CARTESIAN_POINT ( 'NONE',  ( -23.82727386091907462, -11.00084565854733043, 73.54006079994626077 ) ) ;
#1497=CARTESIAN_POINT ( 'NONE',  ( -11.01197672498280866, -17.74032467813711378, 71.85246142747085685 ) ) ;
#1498=CARTESIAN_POINT ( 'NONE',  ( -16.27008412796014625, -7.904986034540439022, 60.20028479263386600 ) ) ;
#1499=VERTEX_POINT ( 'NONE', #23961 ) ;
#1501=CARTESIAN_POINT ( 'NONE',  ( -16.43513463834741728, -22.19403045546258468, 65.41219756188628764 ) ) ;
#1502=CARTESIAN_POINT ( 'NONE',  ( -19.30978178441422699, -7.601027468210772575, 63.61744607541091767 ) ) ;
#1503=CARTESIAN_POINT ( 'NONE',  ( -24.34502428176253019, -17.56683243011407924, 66.12852677468319484 ) ) ;
#1504=CARTESIAN_POINT ( 'NONE',  ( -19.85890256509918572, -21.37233786973231275, 68.95612130754568625 ) ) ;
#1505=CARTESIAN_POINT ( 'NONE',  ( -12.72909380574049187, -20.00294183919138291, 71.87823903238121659 ) ) ;
#1507=B_SPLINE_CURVE_WITH_KNOTS ( 'NONE', 3,
 ( #9863, #43104, #32276, #5696, #5922, #46803, #28080, #16977, #1749, #12581 ),
 .UNSPECIFIED., .F., .F.,
 ( 4, 2, 2, 2, 4 ),
 ( 0.000000000000000000, 0.2500000000000000000, 0.5000000000000000000, 0.7500000000000000000, 1.000000000000000000 ),
 .UNSPECIFIED. ) ;
#1508=ORIENTED_EDGE ( 'NONE', *, *, #17222, .F. ) ;
#1510=VERTEX_POINT ( 'NONE', #35983 ) ;
#1511=B_SPLINE_CURVE_WITH_KNOTS ( 'NONE', 1,
 ( #39387, #24131 ),
 .UNSPECIFIED., .F., .F.,
 ( 2, 2 ),
 ( 0.000000000000000000, 1.000000000000000000 ),
 .UNSPECIFIED. ) ;
#1512=CARTESIAN_POINT ( 'NONE',  ( -24.47066272824306665, -14.57993217219608795, 62.99824437345093031 ) ) ;
#1513=CARTESIAN_POINT ( 'NONE',  ( -19.98813031515369332, -21.37641424997302053, 72.70478737316020101 ) ) ;
#1514=ORIENTED_EDGE ( 'NONE', *, *, #11665, .T. ) ;
#1517=CARTESIAN_POINT ( 'NONE',  ( -22.23733845922741637, -19.96043711175405733, 66.00421731380802726 ) ) ;
#1518=CARTESIAN_POINT ( 'NONE',  ( -23.65624057141237202, -11.51332318074561911, 66.72214514605293800 ) ) ;
#1519=ORIENTED_EDGE ( 'NONE', *, *, #553, .F. ) ;
#1520=CARTESIAN_POINT ( 'NONE',  ( -10.63483715323753565, -17.87674169505483235, 71.75213630217804450 ) ) ;
#1522=CARTESIAN_POINT ( 'NONE',  ( -23.17996796428253603, -10.73203099773195568, 59.69383679455673075 ) ) ;
#1523=ORIENTED_EDGE ( 'NONE', *, *, #46433, .T. ) ;
#1526=EDGE_CURVE ( 'NONE', #35369, #1693, #24644, .T. ) ;
#1527=CARTESIAN_POINT ( 'NONE',  ( -10.13628521134413774, -13.26287664204559391, 74.78543499488121427 ) ) ;
#1528=ORIENTED_EDGE ( 'NONE', *, *, #27294, .F. ) ;
#1529=CARTESIAN_POINT ( 'NONE',  ( -16.02724665508026192, -7.491242618400526077, 63.78515750052793010 ) ) ;
#1530=CARTESIAN_POINT ( 'NONE',  ( -19.17604249790256077, -21.63836284480991878, 58.53979515915469278 ) ) ;
#1531=VERTEX_POINT ( 'NONE', #39455 ) ;
#1532=CARTESIAN_POINT ( 'NONE',  ( -24.24515474721203745, -17.80517362172114559, 62.57386731182483430 ) ) ;
#1533=CARTESIAN_POINT ( 'NONE',  ( -9.979603215878100286, -14.52052451035377345, 68.04295550616701860 ) ) ;
#1534=CARTESIAN_POINT ( 'NONE',  ( -19.49109506855409180, -21.54969648977046148, 62.28031529404344013 ) ) ;
#1535=CARTESIAN_POINT ( 'NONE',  ( -15.45014681279580238, -8.041036458835323586, 74.37425853534905684 ) ) ;
#1536=CARTESIAN_POINT ( 'NONE',  ( -21.24554520941113367, -21.20453976546471608, 65.76949229983627276 ) ) ;
#1537=CARTESIAN_POINT ( 'NONE',  ( -20.52513369171654745, -21.08626508430529611, 58.71645414705509580 ) ) ;
#1538=VERTEX_POINT ( 'NONE', #2021 ) ;
#1540=( BOUNDED_SURFACE ( )  B_SPLINE_SURFACE ( 3, 1, ( 
 ( #28727, #2623 ),
 ( #39139, #5422 ),
 ( #36344, #4945 ),
 ( #36099, #998 ),
 ( #2381, #17394 ),
 ( #12313, #43760 ),
 ( #46301, #10014 ) ),
 .UNSPECIFIED., .T., .F., .F. ) 
 B_SPLINE_SURFACE_WITH_KNOTS ( ( 4, 3, 4 ),
 ( 2, 2 ),
 ( 0.000000000000000000, 0.5000000000000000000, 1.000000000000000000 ),
 ( 0.000000000000000000, 1.000000000000000000 ),
 .UNSPECIFIED. ) 
 GEOMETRIC_REPRESENTATION_ITEM ( )  RATIONAL_B_SPLINE_SURFACE ( (
 ( 1.000000000000000000, 1.000000000000000000),
 ( 0.3333333333333335369, 0.3333333333333330373),
 ( 0.3333333333333335369, 0.3333333333333330373),
 ( 1.000000000000000000, 1.000000000000000000),
 ( 0.3333333333333333703, 0.3333333333333333703),
 ( 0.3333333333333333703, 0.3333333333333333703),
 ( 1.000000000000000000, 1.000000000000000000) ) ) 
 REPRESENTATION_ITEM ( '' )  SURFACE ( )  );
#1542=CARTESIAN_POINT ( 'NONE',  ( -16.23116076413911557, -7.455249184188991407, 60.31533086125586607 ) ) ;
#1544=CARTESIAN_POINT ( 'NONE',  ( -22.07022430586338402, -11.86582892075562334, 54.07175714974878389 ) ) ;
#1547=ADVANCED_FACE ( 'NONE', ( #5737 ), #42910, .T. ) ;
#1550=CARTESIAN_POINT ( 'NONE',  ( -11.01935386438909426, -11.00369580034137229, 60.87896987096186763 ) ) ;
#1554=CARTESIAN_POINT ( 'NONE',  ( -17.98584164848810474, -22.23808382151284491, 62.06031347038508983 ) ) ;
#1556=CARTESIAN_POINT ( 'NONE',  ( -16.94046182855944949, -22.24350478419641419, 72.26568972578677119 ) ) ;
#1557=ORIENTED_EDGE ( 'NONE', *, *, #33788, .T. ) ;
#1558=CARTESIAN_POINT ( 'NONE',  ( -23.73600443614001776, -11.78168025344282555, 63.23601694537735085 ) ) ;
#1559=AXIS2_PLACEMENT_3D ( 'NONE', #31240, #24098, #39593 ) ;
#1560=CARTESIAN_POINT ( 'NONE',  ( -16.26183941974026581, -7.855670460422400581, 60.35028478908645155 ) ) ;
#1562=CYLINDRICAL_SURFACE ( 'NONE', #14930, 0.1499999999999990508 ) ;
#1565=EDGE_CURVE ( 'NONE', #24279, #997, #4665, .T. ) ;
#1566=CARTESIAN_POINT ( 'NONE',  ( -23.48885089983262020, -11.31111638938591568, 73.43363640969468520 ) ) ;
#1567=CARTESIAN_POINT ( 'NONE',  ( -10.39693166811831304, -15.37990016280386740, 57.58264896457095006 ) ) ;
#1568=CARTESIAN_POINT ( 'NONE',  ( -15.62222905942472018, -7.993050613273783966, 70.89517703929612935 ) ) ;
#1569=CARTESIAN_POINT ( 'NONE',  ( -10.73729132840935740, -12.73729855581346371, 64.55219560051592964 ) ) ;
#1573=CARTESIAN_POINT ( 'NONE',  ( -22.98291842025556164, -9.849094896122194243, 70.20516821032623511 ) ) ;
#1574=CARTESIAN_POINT ( 'NONE',  ( -13.26872317195175199, -21.05283485551296607, 54.27966884056655061 ) ) ;
#1577=CARTESIAN_POINT ( 'NONE',  ( -14.23618716594424960, -8.577114723333041368, 71.02957618500911963 ) ) ;
#1580=B_SPLINE_CURVE_WITH_KNOTS ( 'NONE', 3,
 ( #11793, #26560, #45784, #18930, #12032, #3658, #27044, #30272, #15702, #8340 ),
 .UNSPECIFIED., .F., .F.,
 ( 4, 2, 2, 2, 4 ),
 ( 0.000000000000000000, 0.2500000000000000000, 0.5000000000000000000, 0.7500000000000000000, 1.000000000000000000 ),
 .UNSPECIFIED. ) ;
#1582=FACE_OUTER_BOUND ( 'NONE', #1299, .T. ) ;
#1584=CARTESIAN_POINT ( 'NONE',  ( -18.18338144371267617, -21.81849904615365432, 65.63060065626805795 ) ) ;
#1585=ORIENTED_EDGE ( 'NONE', *, *, #46453, .F. ) ;
#1586=CARTESIAN_POINT ( 'NONE',  ( -23.94599579101543796, -17.50730996363388314, 59.15945600998260545 ) ) ;
#1587=VECTOR ( 'NONE', #20656, 1000.000000000000000 ) ;
#1589=( BOUNDED_CURVE ( )  B_SPLINE_CURVE ( 3, ( #26328, #41341, #26575, #7634 ),
 .UNSPECIFIED., .F., .F. ) 
 B_SPLINE_CURVE_WITH_KNOTS ( ( 4, 4 ),
 ( 0.4074455897393671755, 0.5000000000000000000 ),
 .UNSPECIFIED. ) 
 CURVE ( )  GEOMETRIC_REPRESENTATION_ITEM ( )  RATIONAL_B_SPLINE_CURVE ( ( 0.6983129098261091627, 0.7760317562607096376, 0.8765941196520059542, 0.9999999999999961142 ) ) 
 REPRESENTATION_ITEM ( '' )  );
#1591=DIRECTION ( 'NONE',  ( 0.9858639740050647582, 0.1675476790616363121, 8.494556375077916271E-17 ) ) ;
#1592=CARTESIAN_POINT ( 'NONE',  ( -11.30598245021123560, -18.31969919398564528, 61.57711092061642688 ) ) ;
#1595=PLANE ( 'NONE',  #42242 ) ;
#1596=AXIS2_PLACEMENT_3D ( 'NONE', #28882, #21509, #13601 ) ;
#1597=LINE ( 'NONE', #38043, #29795 ) ;
#1598=CARTESIAN_POINT ( 'NONE',  ( -24.47217469005601131, -14.64471752244405067, 62.71296487297676947 ) ) ;
#1599=EDGE_LOOP ( 'NONE', ( #1789, #47994, #48137, #2642, #27619 ) ) ;
#1600=B_SPLINE_CURVE_WITH_KNOTS ( 'NONE', 1,
 ( #12862, #38970 ),
 .UNSPECIFIED., .F., .F.,
 ( 2, 2 ),
 ( 0.000000000000000000, 1.000000000000000000 ),
 .UNSPECIFIED. ) ;
#1601=CARTESIAN_POINT ( 'NONE',  ( -18.53714847821261458, -22.17566945187693506, 72.54156883610106377 ) ) ;
#1602=CARTESIAN_POINT ( 'NONE',  ( -24.37683822056718697, -15.97618770311995462, 66.06324926631656069 ) ) ;
#1603=CARTESIAN_POINT ( 'NONE',  ( -16.45566506110110438, -21.79267588865899086, 62.04095995016087528 ) ) ;
#1604=FACE_BOUND ( 'NONE', #24485, .T. ) ;
#1606=CARTESIAN_POINT ( 'NONE',  ( -17.50157081909136991, -7.358860168393607459, 67.20694839074946003 ) ) ;
#1607=CARTESIAN_POINT ( 'NONE',  ( -16.00544582274271477, -7.903112417841744453, 63.95538887075813506 ) ) ;
#1609=FACE_OUTER_BOUND ( 'NONE', #22444, .T. ) ;
#1610=ORIENTED_EDGE ( 'NONE', *, *, #4998, .T. ) ;
#1611=CARTESIAN_POINT ( 'NONE',  ( -11.45656716003344933, -19.26928393672501727, 71.73039932227760573 ) ) ;
#1612=CARTESIAN_POINT ( 'NONE',  ( -13.30358910455570332, -20.46953808992088852, 58.27480040995169475 ) ) ;
#1614=CARTESIAN_POINT ( 'NONE',  ( -16.84865286310842336, -21.83598151670433296, 68.98088545748413480 ) ) ;
#1615=CARTESIAN_POINT ( 'NONE',  ( -12.75166747855125493, -9.006326174502946813, 71.01071880285634563 ) ) ;
#1617=ORIENTED_EDGE ( 'NONE', *, *, #34829, .T. ) ;
#1618=ORIENTED_EDGE ( 'NONE', *, *, #4581, .F. ) ;
#1622=CARTESIAN_POINT ( 'NONE',  ( -17.98657259272421172, -21.83703102787368167, 62.16063850355641307 ) ) ;
#1623=CARTESIAN_POINT ( 'NONE',  ( -24.43362379028604536, -14.05489247495133753, 73.12271507725591846 ) ) ;
#1624=CARTESIAN_POINT ( 'NONE',  ( -21.33694466872984918, -9.004932385753821933, 73.90128753631783809 ) ) ;
#1625=CARTESIAN_POINT ( 'NONE',  ( -11.85383375607109713, -9.861995938241047810, 64.12940074489686992 ) ) ;
#1629=VERTEX_POINT ( 'NONE', #17744 ) ;
#1631=DIRECTION ( 'NONE',  ( -0.5263399769092093061, 0.8502742079512979334, 7.678741024442198749E-08 ) ) ;
#1632=CARTESIAN_POINT ( 'NONE',  ( -20.89788161767221197, -20.94431024770144489, 62.39999296070408974 ) ) ;
#1634=CARTESIAN_POINT ( 'NONE',  ( -12.64995486802317082, -19.99670083032576429, 68.33657438322859434 ) ) ;
#1636=ADVANCED_FACE ( 'NONE', ( #2977 ), #48524, .T. ) ;
#1637=ORIENTED_EDGE ( 'NONE', *, *, #35530, .F. ) ;
#1638=ADVANCED_FACE ( 'NONE', ( #48045 ), #14760, .T. ) ;
#1639=ADVANCED_FACE ( 'NONE', ( #25163 ), #32775, .T. ) ;
#1640=CARTESIAN_POINT ( 'NONE',  ( -23.02753126890070590, -10.61360989481728367, 59.90203474228974301 ) ) ;
#1642=CARTESIAN_POINT ( 'NONE',  ( -23.83043773139749888, -11.86620498678314384, 59.78235732590889739 ) ) ;
#1644=CARTESIAN_POINT ( 'NONE',  ( -12.43502697965553416, -19.72161038572663472, 64.97747870948867899 ) ) ;
#1646=CARTESIAN_POINT ( 'NONE',  ( -11.68335550665270794, -18.81469308649876737, 68.21689631955439381 ) ) ;
#1648=CARTESIAN_POINT ( 'NONE',  ( -9.974456290884534226, -14.72748455880875795, 71.51278017970571454 ) ) ;
#1649=CARTESIAN_POINT ( 'NONE',  ( -21.40283924303304985, -8.989053705293313712, 73.60688577834839919 ) ) ;
#1650=CARTESIAN_POINT ( 'NONE',  ( -14.40787616456130493, -7.996955972674248514, 63.91166111565177488 ) ) ;
#1651=CIRCLE ( 'NONE', #4022, 7.500000000000002665 ) ;
#1653=CARTESIAN_POINT ( 'NONE',  ( -14.30855566557790404, -8.484641631233271752, 70.74429704309763167 ) ) ;
#1654=CARTESIAN_POINT ( 'NONE',  ( -24.82316860084702981, -15.68024280754056576, 73.14270404762098110 ) ) ;
#1656=VERTEX_POINT ( 'NONE', #25402 ) ;
#1657=CARTESIAN_POINT ( 'NONE',  ( -10.00731251637046881, -14.10555026099538978, 61.10316585833331260 ) ) ;
#1660=CARTESIAN_POINT ( 'NONE',  ( -19.16569461048236889, -7.565509106446075549, 63.55276450808027278 ) ) ;
#1661=PLANE ( 'NONE',  #32724 ) ;
#1663=DIRECTION ( 'NONE',  ( -0.1539336739619741878, -0.9880811829098681276, -6.607022904161600477E-08 ) ) ;
#1664=CARTESIAN_POINT ( 'NONE',  ( -10.42492065060444872, -12.25670954885047692, 57.58503240040955262 ) ) ;
#1665=ADVANCED_FACE ( 'NONE', ( #7187 ), #10860, .T. ) ;
#1666=CARTESIAN_POINT ( 'NONE',  ( -13.18362886651731358, -8.683667069837246899, 60.62445550483372614 ) ) ;
#1667=PLANE ( 'NONE',  #25087 ) ;
#1669=FACE_OUTER_BOUND ( 'NONE', #19095, .T. ) ;
#1670=AXIS2_PLACEMENT_3D ( 'NONE', #43867, #36919, #25140 ) ;
#1672=( BOUNDED_CURVE ( )  B_SPLINE_CURVE ( 3, ( #30031, #34181, #23127, #7627 ),
 .UNSPECIFIED., .F., .F. ) 
 B_SPLINE_CURVE_WITH_KNOTS ( ( 4, 4 ),
 ( 0.5000000000000000000, 0.9074455897393662873 ),
 .UNSPECIFIED. ) 
 CURVE ( )  GEOMETRIC_REPRESENTATION_ITEM ( )  RATIONAL_B_SPLINE_CURVE ( ( 1.000000000000003553, 0.4567392136813320791, 0.3561768502900277689, 0.6983129098260943968 ) ) 
 REPRESENTATION_ITEM ( '' )  );
#1673=CARTESIAN_POINT ( 'NONE',  ( -20.48427295952909688, -21.16374346551129548, 59.05963865090804887 ) ) ;
#1674=CARTESIAN_POINT ( 'NONE',  ( -10.44503168371052837, -15.82779754136115002, 68.39256704124431963 ) ) ;
#1675=ORIENTED_EDGE ( 'NONE', *, *, #18667, .F. ) ;
#1676=CARTESIAN_POINT ( 'NONE',  ( -16.20274916913749408, -7.857711080649619539, 67.28440454693885897 ) ) ;
#1681=ORIENTED_EDGE ( 'NONE', *, *, #24884, .T. ) ;
#1686=DIRECTION ( 'NONE',  ( -0.8201047403141396019, 0.5722134347551370848, 7.883065731424289661E-08 ) ) ;
#1688=CARTESIAN_POINT ( 'NONE',  ( -20.03282965983824226, -21.84088468745754597, 53.89198173725360874 ) ) ;
#1689=CARTESIAN_POINT ( 'NONE',  ( -18.63772371551852913, -7.458595371860563539, 73.96347537936300398 ) ) ;
#1690=( BOUNDED_SURFACE ( )  B_SPLINE_SURFACE ( 3, 1, ( 
 ( #31567, #12129 ),
 ( #24434, #8928 ),
 ( #12843, #32051 ),
 ( #1046, #27146 ),
 ( #31809, #23947 ),
 ( #38949, #16530 ),
 ( #28107, #46601 ) ),
 .UNSPECIFIED., .T., .F., .F. ) 
 B_SPLINE_SURFACE_WITH_KNOTS ( ( 4, 3, 4 ),
 ( 2, 2 ),
 ( 0.000000000000000000, 0.5000000000000000000, 1.000000000000000000 ),
 ( 0.000000000000000000, 1.000000000000000000 ),
 .UNSPECIFIED. ) 
 GEOMETRIC_REPRESENTATION_ITEM ( )  RATIONAL_B_SPLINE_SURFACE ( (
 ( 1.000000000000000000, 1.000000000000000000),
 ( 0.3333333333333335369, 0.3333333333333330373),
 ( 0.3333333333333335369, 0.3333333333333330373),
 ( 1.000000000000000000, 1.000000000000000000),
 ( 0.3333333333333333703, 0.3333333333333333703),
 ( 0.3333333333333333703, 0.3333333333333333703),
 ( 1.000000000000000000, 1.000000000000000000) ) ) 
 REPRESENTATION_ITEM ( '' )  SURFACE ( )  );
#1691=FACE_OUTER_BOUND ( 'NONE', #46233, .T. ) ;
#1693=VERTEX_POINT ( 'NONE', #10623 ) ;
#1694=AXIS2_PLACEMENT_3D ( 'NONE', #37655, #18697, #48252 ) ;
#1695=FACE_OUTER_BOUND ( 'NONE', #989, .T. ) ;
#1698=CARTESIAN_POINT ( 'NONE',  ( -19.81157080418587313, -21.44583120317290081, 65.34997476282926243 ) ) ;
#1700=CARTESIAN_POINT ( 'NONE',  ( -11.10553262954647380, -11.79631758389720986, 71.08860856935916672 ) ) ;
#1701=B_SPLINE_CURVE_WITH_KNOTS ( 'NONE', 3,
 ( #20000, #8923, #5221, #12838, #46822, #42165, #13066, #42415, #31076, #34769 ),
 .UNSPECIFIED., .F., .F.,
 ( 4, 2, 2, 2, 4 ),
 ( 0.000000000000000000, 0.2500000000000000000, 0.5000000000000000000, 0.7500000000000000000, 1.000000000000000000 ),
 .UNSPECIFIED. ) ;
#1703=ORIENTED_EDGE ( 'NONE', *, *, #4007, .T. ) ;
#1704=EDGE_CURVE ( 'NONE', #3004, #2922, #3547, .T. ) ;
#1705=EDGE_CURVE ( 'NONE', #16276, #23858, #39886, .T. ) ;
#1706=CARTESIAN_POINT ( 'NONE',  ( -19.67573413203048460, -21.49838315979392789, 72.54911470401957274 ) ) ;
#1710=VERTEX_POINT ( 'NONE', #41638 ) ;
#1711=CARTESIAN_POINT ( 'NONE',  ( -10.55459683810411775, -16.15489166977095437, 68.20441073976071777 ) ) ;
#1712=EDGE_CURVE ( 'NONE', #28108, #14347, #13600, .T. ) ;
#1717=B_SPLINE_CURVE_WITH_KNOTS ( 'NONE', 1,
 ( #29535, #22159 ),
 .UNSPECIFIED., .F., .F.,
 ( 2, 2 ),
 ( 0.000000000000000000, 1.000000000000000000 ),
 .UNSPECIFIED. ) ;
#1718=CARTESIAN_POINT ( 'NONE',  ( -24.42364818358896272, -14.92042579261047131, 59.25916823501875541 ) ) ;
#1719=FACE_OUTER_BOUND ( 'NONE', #11856, .T. ) ;
#1722=CARTESIAN_POINT ( 'NONE',  ( -20.30948038729556515, -7.940514767581826838, 70.42817259598375301 ) ) ;
#1724=CARTESIAN_POINT ( 'NONE',  ( -19.19606154404358378, -7.572994735369867669, 63.63078005410717708 ) ) ;
#1725=CARTESIAN_POINT ( 'NONE',  ( -18.66311988809301425, -7.868636481342422329, 70.65595886192740238 ) ) ;
#1730=AXIS2_PLACEMENT_3D ( 'NONE', #10893, #311, #44637 ) ;
#1731=VERTEX_POINT ( 'NONE', #41886 ) ;
#1732=CARTESIAN_POINT ( 'NONE',  ( -24.43107140960042756, -14.03117428492017105, 73.42271492810181144 ) ) ;
#1733=CARTESIAN_POINT ( 'NONE',  ( -24.10630227758727173, -12.71861067290860703, 73.43152628679671068 ) ) ;
#1734=CARTESIAN_POINT ( 'NONE',  ( -13.62541112515491903, -8.865852518713435160, 60.53130564717850604 ) ) ;
#1735=ORIENTED_EDGE ( 'NONE', *, *, #9269, .T. ) ;
#1736=CARTESIAN_POINT ( 'NONE',  ( -23.89679824780917627, -17.47455792287359344, 62.58247085085636030 ) ) ;
#1737=CARTESIAN_POINT ( 'NONE',  ( -10.42394424466950476, -17.36098423042032124, 64.81394647623933736 ) ) ;
#1739=CARTESIAN_POINT ( 'NONE',  ( -23.44980453451080749, -18.46889374286061525, 73.06368236440982855 ) ) ;
#1742=ORIENTED_EDGE ( 'NONE', *, *, #4645, .T. ) ;
#1743=CARTESIAN_POINT ( 'NONE',  ( -23.81024829756716343, -18.64597716098235836, 72.94863620959463901 ) ) ;
#1744=FACE_OUTER_BOUND ( 'NONE', #26665, .T. ) ;
#1745=ORIENTED_EDGE ( 'NONE', *, *, #45560, .T. ) ;
#1746=CARTESIAN_POINT ( 'NONE',  ( -24.33988733120284564, -15.89210004164691092, 66.34859510278248251 ) ) ;
#1747=CARTESIAN_POINT ( 'NONE',  ( -10.66703363856100317, -12.79807828486586629, 64.26836111018113229 ) ) ;
#1749=CARTESIAN_POINT ( 'NONE',  ( -10.42512903781134881, -14.93652116780334893, 75.09778865157521466 ) ) ;
#1751=CARTESIAN_POINT ( 'NONE',  ( -19.23866403772855449, -21.62168293227472660, 58.67507384656568092 ) ) ;
#1753=CARTESIAN_POINT ( 'NONE',  ( -16.64495962069230117, -22.21910613783234822, 65.33909019606271329 ) ) ;
#1754=CARTESIAN_POINT ( 'NONE',  ( -10.42334091404133645, -15.64104667191196185, 61.33789045260130024 ) ) ;
#1756=CARTESIAN_POINT ( 'NONE',  ( -22.79960237261627398, -9.650942640399760464, 73.66656521964461035 ) ) ;
#1758=EDGE_CURVE ( 'NONE', #11201, #12343, #4218, .T. ) ;
#1759=EDGE_LOOP ( 'NONE', ( #35753, #14719 ) ) ;
#1760=ORIENTED_EDGE ( 'NONE', *, *, #5934, .F. ) ;
#1762=EDGE_CURVE ( 'NONE', #9814, #25893, #21566, .T. ) ;
#1763=CARTESIAN_POINT ( 'NONE',  ( -17.63706249495991685, -7.362172851917661909, 63.80702937774674410 ) ) ;
#1765=CARTESIAN_POINT ( 'NONE',  ( -21.70346447568910264, -9.269547348209590254, 63.26441786439349357 ) ) ;
#1766=ORIENTED_EDGE ( 'NONE', *, *, #35518, .F. ) ;
#1767=CARTESIAN_POINT ( 'NONE',  ( -21.63336539757928634, -9.153348366551478321, 66.94677872351418557 ) ) ;
#1768=EDGE_CURVE ( 'NONE', #9708, #19538, #43282, .T. ) ;
#1769=LINE ( 'NONE', #1518, #6831 ) ;
#1770=ORIENTED_EDGE ( 'NONE', *, *, #47997, .F. ) ;
#1771=EDGE_CURVE ( 'NONE', #4886, #36512, #119, .T. ) ;
#1772=( BOUNDED_SURFACE ( )  B_SPLINE_SURFACE ( 3, 1, ( 
 ( #43639, #33236 ),
 ( #28843, #17509 ),
 ( #2733, #3224 ),
 ( #2506, #9901 ),
 ( #17741, #44598 ),
 ( #29086, #25878 ),
 ( #40892, #10139 ) ),
 .UNSPECIFIED., .T., .F., .F. ) 
 B_SPLINE_SURFACE_WITH_KNOTS ( ( 4, 3, 4 ),
 ( 2, 2 ),
 ( 0.000000000000000000, 0.5000000000000000000, 1.000000000000000000 ),
 ( 0.000000000000000000, 1.000000000000000000 ),
 .UNSPECIFIED. ) 
 GEOMETRIC_REPRESENTATION_ITEM ( )  RATIONAL_B_SPLINE_SURFACE ( (
 ( 1.000000000000000000, 1.000000000000000000),
 ( 0.3333333333333335369, 0.3333333333333330373),
 ( 0.3333333333333335369, 0.3333333333333330373),
 ( 1.000000000000000000, 1.000000000000000000),
 ( 0.3333333333333333703, 0.3333333333333333703),
 ( 0.3333333333333333703, 0.3333333333333333703),
 ( 1.000000000000000000, 1.000000000000000000) ) ) 
 REPRESENTATION_ITEM ( '' )  SURFACE ( )  );
#1773=CARTESIAN_POINT ( 'NONE',  ( -23.83833621072449560, -17.61232891644574394, 62.47360984984814536 ) ) ;
#1776=CARTESIAN_POINT ( 'NONE',  ( -10.81118781404325446, -12.51348630141821339, 57.61392014802877526 ) ) ;
#1777=ORIENTED_EDGE ( 'NONE', *, *, #43793, .T. ) ;
#1778=CARTESIAN_POINT ( 'NONE',  ( -10.55941254297143672, -13.20321188299672066, 71.50828559427667130 ) ) ;
#1779=VERTEX_POINT ( 'NONE', #45340 ) ;
#1780=CARTESIAN_POINT ( 'NONE',  ( -15.88847107554206062, -7.518423027132939751, 63.78355628068795369 ) ) ;
#1781=CARTESIAN_POINT ( 'NONE',  ( -13.43921569888383694, -8.993430976374535035, 60.58950277493168812 ) ) ;
#1782=ORIENTED_EDGE ( 'NONE', *, *, #41587, .T. ) ;
#1783=DIRECTION ( 'NONE',  ( -3.549360974554993999E-17, 6.371834667797928663E-18, 1.000000000000000000 ) ) ;
#1784=CARTESIAN_POINT ( 'NONE',  ( -14.62732312719877115, -7.904084895095371266, 60.51985068470025908 ) ) ;
#1786=CARTESIAN_POINT ( 'NONE',  ( -12.64995486802316904, -19.99670083032576429, 68.33657438322859434 ) ) ;
#1788=CARTESIAN_POINT ( 'NONE',  ( -11.93522140360746242, -14.45952210441258501, 53.49899999999994549 ) ) ;
#1789=ORIENTED_EDGE ( 'NONE', *, *, #26530, .F. ) ;
#1790=CARTESIAN_POINT ( 'NONE',  ( -17.55070634552562581, -7.810229109950414639, 63.55057029484540010 ) ) ;
#1791=CARTESIAN_POINT ( 'NONE',  ( -11.88868080670210503, -19.09397054066711164, 71.87788967464850032 ) ) ;
#1792=CARTESIAN_POINT ( 'NONE',  ( -14.09463846823036981, -8.088735815341543400, 54.27966884056655061 ) ) ;
#1793=CARTESIAN_POINT ( 'NONE',  ( -14.39716994511728387, -8.437976179034702540, 63.78978877716816243 ) ) ;
#1797=CARTESIAN_POINT ( 'NONE',  ( -21.06702863216100141, -20.84540773593991148, 65.86981821684420879 ) ) ;
#1798=CARTESIAN_POINT ( 'NONE',  ( -24.43827367352892210, -15.52193379869737377, 73.28831629023289906 ) ) ;
#1799=ORIENTED_EDGE ( 'NONE', *, *, #28644, .T. ) ;
#1800=CARTESIAN_POINT ( 'NONE',  ( -11.33476804054750531, -19.10151225439055978, 68.40184904730287485 ) ) ;
#1801=DIRECTION ( 'NONE',  ( -7.357566627711770083E-06, -1.068273751865974396E-05, 0.9999999999158726283 ) ) ;
#1802=CARTESIAN_POINT ( 'NONE',  ( -22.93054552543627977, -10.40195957496224644, 66.95671006072360854 ) ) ;
#1803=CARTESIAN_POINT ( 'NONE',  ( -19.36518065869528726, -8.031383756764064685, 59.97565108339750850 ) ) ;
#1804=CARTESIAN_POINT ( 'NONE',  ( -15.47038452772150841, -21.58309165278561537, 72.04575460769355288 ) ) ;
#1805=ORIENTED_EDGE ( 'NONE', *, *, #45521, .F. ) ;
#1806=CARTESIAN_POINT ( 'NONE',  ( -12.09877737032034872, -9.599088377814357642, 57.21122801541561387 ) ) ;
#1807=CARTESIAN_POINT ( 'NONE',  ( -17.01596658974409593, -7.370308080546169371, 74.07522964315150205 ) ) ;
#1808=FACE_OUTER_BOUND ( 'NONE', #20776, .T. ) ;
#1810=CARTESIAN_POINT ( 'NONE',  ( -17.26457240846633567, -7.760713630915982542, 70.50507891880883449 ) ) ;
#1811=CARTESIAN_POINT ( 'NONE',  ( -13.24838165316469052, -8.639299380175261334, 60.61763066408384759 ) ) ;
#1812=CARTESIAN_POINT ( 'NONE',  ( -10.40277073914389661, -15.44443991871667343, 57.56792809063193772 ) ) ;
#1813=ADVANCED_FACE ( 'NONE', ( #42371 ), #18634, .T. ) ;
#1814=CARTESIAN_POINT ( 'NONE',  ( -15.88442554950127139, -7.926310505211968227, 71.02478706424572863 ) ) ;
#1816=ORIENTED_EDGE ( 'NONE', *, *, #47084, .T. ) ;
#1818=B_SPLINE_CURVE_WITH_KNOTS ( 'NONE', 1,
 ( #2349, #36311 ),
 .UNSPECIFIED., .F., .F.,
 ( 2, 2 ),
 ( 0.000000000000000000, 1.000000000000000000 ),
 .UNSPECIFIED. ) ;
#1820=CARTESIAN_POINT ( 'NONE',  ( -21.23484681875272528, -20.74088929683185611, 69.33978048267414351 ) ) ;
#1822=CARTESIAN_POINT ( 'NONE',  ( -14.09489777434381530, -8.144396602184544420, 70.92295928270578997 ) ) ;
#1823=( BOUNDED_CURVE ( )  B_SPLINE_CURVE ( 3, ( #46798, #9378, #24397, #5690 ),
 .UNSPECIFIED., .F., .F. ) 
 B_SPLINE_CURVE_WITH_KNOTS ( ( 4, 4 ),
 ( 0.000000000000000000, 0.4074455897393636228 ),
 .UNSPECIFIED. ) 
 CURVE ( )  GEOMETRIC_REPRESENTATION_ITEM ( )  RATIONAL_B_SPLINE_CURVE ( ( 1.000000000000000000, 0.4567392136813388515, 0.3561768502900328204, 0.6983129098260818513 ) ) 
 REPRESENTATION_ITEM ( '' )  );
#1824=CARTESIAN_POINT ( 'NONE',  ( -11.59906938467913484, -10.16455840884576389, 71.22539037155303276 ) ) ;
#1826=CARTESIAN_POINT ( 'NONE',  ( -24.34216731694079527, -17.57390378916213436, 66.13631411268475802 ) ) ;
#1827=ORIENTED_EDGE ( 'NONE', *, *, #39300, .T. ) ;
#1828=EDGE_CURVE ( 'NONE', #30777, #24975, #38778, .T. ) ;
#1830=DIRECTION ( 'NONE',  ( 8.478320013641884810E-07, -8.009068454735622942E-06, 0.9999999999675679430 ) ) ;
#1831=EDGE_CURVE ( 'NONE', #7816, #31055, #36783, .T. ) ;
#1833=CARTESIAN_POINT ( 'NONE',  ( -23.89081516821958218, -17.62458393556817171, 58.88889748697027926 ) ) ;
#1834=( BOUNDED_CURVE ( )  B_SPLINE_CURVE ( 3, ( #35321, #46422, #13630, #28670 ),
 .UNSPECIFIED., .F., .F. ) 
 B_SPLINE_CURVE_WITH_KNOTS ( ( 4, 4 ),
 ( 0.9074455897393596260, 1.000000000000000000 ),
 .UNSPECIFIED. ) 
 CURVE ( )  GEOMETRIC_REPRESENTATION_ITEM ( )  RATIONAL_B_SPLINE_CURVE ( ( 0.6983129098260900669, 0.7760317562606956487, 0.8765941196519989598, 1.000000000000000000 ) ) 
 REPRESENTATION_ITEM ( '' )  );
#1835=CARTESIAN_POINT ( 'NONE',  ( -24.87417962317557496, -14.80849170857717567, 59.42795673386487465 ) ) ;
#1837=EDGE_CURVE ( 'NONE', #44556, #19371, #43833, .T. ) ;
#1839=CARTESIAN_POINT ( 'NONE',  ( -12.21605502382481490, -19.48707594822949218, 58.21065790830979125 ) ) ;
#1840=ORIENTED_EDGE ( 'NONE', *, *, #42876, .T. ) ;
#1841=CARTESIAN_POINT ( 'NONE',  ( -17.66159697976433307, -21.85550285805611637, 58.42025434932890704 ) ) ;
#1843=EDGE_CURVE ( 'NONE', #40764, #24808, #28001, .T. ) ;
#1844=CARTESIAN_POINT ( 'NONE',  ( -15.43182990062313564, -8.046249867383863830, 74.36513541778452918 ) ) ;
#1845=CARTESIAN_POINT ( 'NONE',  ( -11.09366621811533093, -17.79679521274233167, 71.67604308249768508 ) ) ;
#1846=VERTEX_POINT ( 'NONE', #13267 ) ;
#1847=CYLINDRICAL_SURFACE ( 'NONE', #44106, 0.1500000000000072387 ) ;
#1849=ADVANCED_FACE ( 'NONE', ( #6148 ), #39783, .T. ) ;
#1850=CARTESIAN_POINT ( 'NONE',  ( -12.37908165583508158, -20.29102667443158126, 68.48657438459629532 ) ) ;
#1851=PLANE ( 'NONE',  #30540 ) ;
#1852=CARTESIAN_POINT ( 'NONE',  ( -19.28352822169459202, -22.07505156356299381, 54.27966884056655061 ) ) ;
#1853=CARTESIAN_POINT ( 'NONE',  ( -21.99178464560338497, -9.439038884874848989, 59.87171213140518944 ) ) ;
#1862=VERTEX_POINT ( 'NONE', #9618 ) ;
#1864=CARTESIAN_POINT ( 'NONE',  ( -21.29196722032537537, -20.70380199363842877, 72.53918572867779346 ) ) ;
#1865=CARTESIAN_POINT ( 'NONE',  ( -23.78500256881436314, -11.88707711785523635, 59.48235732566631384 ) ) ;
#1866=EDGE_CURVE ( 'NONE', #34062, #1531, #36887, .T. ) ;
#1868=CARTESIAN_POINT ( 'NONE',  ( -14.37682202087475680, -19.38786730597467667, 53.49999999999995026 ) ) ;
#1869=CARTESIAN_POINT ( 'NONE',  ( -13.35650607536230261, -9.112225995665673040, 60.66623508672251575 ) ) ;
#1870=ORIENTED_EDGE ( 'NONE', *, *, #11942, .T. ) ;
#1871=ORIENTED_EDGE ( 'NONE', *, *, #38515, .F. ) ;
#1873=CARTESIAN_POINT ( 'NONE',  ( -21.65613231742964473, -20.94137680209911423, 72.63791026777079196 ) ) ;
#1874=CARTESIAN_POINT ( 'NONE',  ( -16.50258162057404832, -20.23145840177225452, 53.49899999999994549 ) ) ;
#1875=CARTESIAN_POINT ( 'NONE',  ( -10.37818533259200748, -17.22973363664382873, 61.27247698181179913 ) ) ;
#1877=EDGE_CURVE ( 'NONE', #46048, #31463, #48255, .T. ) ;
#1879=LINE ( 'NONE', #1149, #36667 ) ;
#1880=FACE_OUTER_BOUND ( 'NONE', #39765, .T. ) ;
#1882=CYLINDRICAL_SURFACE ( 'NONE', #14989, 0.1500000000000043521 ) ;
#1883=ORIENTED_EDGE ( 'NONE', *, *, #19647, .F. ) ;
#1884=CARTESIAN_POINT ( 'NONE',  ( -11.66088473761816324, -18.78248764865968568, 68.21689682892682072 ) ) ;
#1886=CARTESIAN_POINT ( 'NONE',  ( -9.975558569371616002, -14.65758674969880104, 71.58428599250275681 ) ) ;
#1887=CARTESIAN_POINT ( 'NONE',  ( -10.43128225812950305, -13.88506779950195202, 61.01001469056328119 ) ) ;
#1890=ORIENTED_EDGE ( 'NONE', *, *, #37328, .T. ) ;
#1891=B_SPLINE_CURVE_WITH_KNOTS ( 'NONE', 3,
 ( #14049, #36693, #2988, #37691, #18738, #30091, #41892, #295, #22951, #26630 ),
 .UNSPECIFIED., .F., .F.,
 ( 4, 2, 2, 2, 4 ),
 ( 0.000000000000000000, 0.2500000000000000000, 0.5000000000000000000, 0.7500000000000000000, 1.000000000000000000 ),
 .UNSPECIFIED. ) ;
#1894=CARTESIAN_POINT ( 'NONE',  ( -11.74434772961222961, -10.63247619797795629, 74.73325195789129793 ) ) ;
#1895=CARTESIAN_POINT ( 'NONE',  ( -18.11396590982544197, -21.77512906430638040, 65.64532159443497505 ) ) ;
#1896=EDGE_LOOP ( 'NONE', ( #20916, #20589 ) ) ;
#1898=ORIENTED_EDGE ( 'NONE', *, *, #25020, .T. ) ;
#1899=CARTESIAN_POINT ( 'NONE',  ( -9.975583804105555785, -14.65598652642324673, 71.44287259100559595 ) ) ;
#1900=CARTESIAN_POINT ( 'NONE',  ( -16.26649175736496744, -21.71412290693840319, 61.98398093021437916 ) ) ;
#1901=ORIENTED_EDGE ( 'NONE', *, *, #25081, .T. ) ;
#1902=CARTESIAN_POINT ( 'NONE',  ( -10.31364544024427410, -17.03300993871772562, 57.80265247535063367 ) ) ;
#1903=CARTESIAN_POINT ( 'NONE',  ( -21.91034545428830782, -20.18261758176410936, 58.76442899736473180 ) ) ;
#1904=CARTESIAN_POINT ( 'NONE',  ( -23.44980260057078070, -18.46889688393208573, 72.76368236443251192 ) ) ;
#1905=VERTEX_POINT ( 'NONE', #43832 ) ;
#1906=CARTESIAN_POINT ( 'NONE',  ( -9.996749499990320587, -14.22650194697012260, 64.54950375361089243 ) ) ;
#1907=CARTESIAN_POINT ( 'NONE',  ( -20.66696855643225561, -21.06909979829504209, 58.94475164909855636 ) ) ;
#1908=CARTESIAN_POINT ( 'NONE',  ( -15.28303595616968913, -7.672713470548185200, 74.19330299898706471 ) ) ;
#1909=ADVANCED_FACE ( 'NONE', ( #18179 ), #38192, .T. ) ;
#1911=CARTESIAN_POINT ( 'NONE',  ( -15.67484944857656082, -7.976566202440097619, 67.02518389757648265 ) ) ;
#1913=VECTOR ( 'NONE', #46444, 1000.000000000000227 ) ;
#1914=LINE ( 'NONE', #31953, #16475 ) ;
#1918=VERTEX_POINT ( 'NONE', #13985 ) ;
#1920=CARTESIAN_POINT ( 'NONE',  ( -14.88579407610268035, -21.33278181836255882, 58.27504001164205505 ) ) ;
#1921=PLANE ( 'NONE',  #3674 ) ;
#1922=CARTESIAN_POINT ( 'NONE',  ( -24.87384330133638599, -14.87999890626018384, 59.35804801245023299 ) ) ;
#1924=DIRECTION ( 'NONE',  ( -7.357566627711770083E-06, -1.068273751865974396E-05, 0.9999999999158726283 ) ) ;
#1925=CARTESIAN_POINT ( 'NONE',  ( -19.78726556874234888, -21.93198837902608744, 53.76173960638111993 ) ) ;
#1926=CARTESIAN_POINT ( 'NONE',  ( -13.14998806103231566, -9.265559761403904915, 67.67942786032521951 ) ) ;
#1927=CARTESIAN_POINT ( 'NONE',  ( -10.79572441526863180, -11.40795732096215254, 67.80359905390240272 ) ) ;
#1929=ORIENTED_EDGE ( 'NONE', *, *, #16604, .T. ) ;
#1930=CARTESIAN_POINT ( 'NONE',  ( -10.61641629527463770, -11.78277212779517136, 74.74335553404092991 ) ) ;
#1931=CARTESIAN_POINT ( 'NONE',  ( -21.94216005978649875, -20.15605564530504878, 59.06442870682581514 ) ) ;
#1932=CARTESIAN_POINT ( 'NONE',  ( -20.60942684424193416, -21.09890871138989965, 58.65947248567252359 ) ) ;
#1933=CARTESIAN_POINT ( 'NONE',  ( -22.37742512587845312, -19.75764156297556795, 72.75473533163390982 ) ) ;
#1934=PLANE ( 'NONE',  #7963 ) ;
#1935=ORIENTED_EDGE ( 'NONE', *, *, #21287, .T. ) ;
#1936=B_SPLINE_CURVE_WITH_KNOTS ( 'NONE', 3,
 ( #23055, #45715, #19843, #34843, #42002, #16110, #12437, #8275, #23291, #882 ),
 .UNSPECIFIED., .F., .F.,
 ( 4, 2, 2, 2, 4 ),
 ( 0.6272669072877771201, 0.7522669073072866253, 0.8772669073267960194, 1.002266907346305524, 1.127266907365815030 ),
 .UNSPECIFIED. ) ;
#1938=CARTESIAN_POINT ( 'NONE',  ( -14.96634385547669055, -21.36368446393953846, 61.63600446054231696 ) ) ;
#1941=CARTESIAN_POINT ( 'NONE',  ( -24.07704370891653767, -17.14264987453632827, 72.89808101046212130 ) ) ;
#1943=CARTESIAN_POINT ( 'NONE',  ( -11.86838291625971742, -9.845553222893467904, 64.14418898700822069 ) ) ;
#1948=CARTESIAN_POINT ( 'NONE',  ( -18.65633333895540602, -7.917218528759340401, 73.91234765977904431 ) ) ;
#1949=CARTESIAN_POINT ( 'NONE',  ( -16.77572482835368817, -7.785357162821431309, 73.96018178516708019 ) ) ;
#1951=CARTESIAN_POINT ( 'NONE',  ( -23.45015259912689132, -11.24725851716134883, 70.11884051640547000 ) ) ;
#1952=ORIENTED_EDGE ( 'NONE', *, *, #21868, .F. ) ;
#1953=CARTESIAN_POINT ( 'NONE',  ( -10.49991623338872415, -13.77081093687474578, 57.63752186588624937 ) ) ;
#1955=CARTESIAN_POINT ( 'NONE',  ( -19.24190894175819366, -7.584296403803404196, 63.54593838833191910 ) ) ;
#1956=FACE_OUTER_BOUND ( 'NONE', #11602, .T. ) ;
#1958=FACE_OUTER_BOUND ( 'NONE', #4292, .T. ) ;
#1960=ORIENTED_EDGE ( 'NONE', *, *, #10650, .F. ) ;
#1961=CARTESIAN_POINT ( 'NONE',  ( -17.93803624496681692, -7.826487624369620200, 60.26987800131050932 ) ) ;
#1962=CARTESIAN_POINT ( 'NONE',  ( -19.04853579327176760, -7.948602568230340282, 63.71617106789811658 ) ) ;
#1964=ORIENTED_EDGE ( 'NONE', *, *, #31188, .T. ) ;
#1965=( BOUNDED_CURVE ( )  B_SPLINE_CURVE ( 3, ( #15785, #42398, #24411, #35471 ),
 .UNSPECIFIED., .F., .F. ) 
 B_SPLINE_CURVE_WITH_KNOTS ( ( 4, 4 ),
 ( 0.5000000000000000000, 0.9074455897393689519 ),
 .UNSPECIFIED. ) 
 CURVE ( )  GEOMETRIC_REPRESENTATION_ITEM ( )  RATIONAL_B_SPLINE_CURVE ( ( 0.9999999999999952260, 0.4567392136813272496, 0.3561768502900317102, 0.6983129098261036116 ) ) 
 REPRESENTATION_ITEM ( '' )  );
#1968=CARTESIAN_POINT ( 'NONE',  ( -20.88147576600584543, -8.209942340109883219, 60.02620652709861560 ) ) ;
#1969=CARTESIAN_POINT ( 'NONE',  ( -23.38313847423633263, -10.33780256150599541, 59.85849373767491954 ) ) ;
#1972=ORIENTED_EDGE ( 'NONE', *, *, #4173, .T. ) ;
#1974=CARTESIAN_POINT ( 'NONE',  ( -10.40127070788197017, -12.32249518151173895, 57.51352764219546998 ) ) ;
#1976=VERTEX_POINT ( 'NONE', #48225 ) ;
#1977=CARTESIAN_POINT ( 'NONE',  ( -22.08699904183838214, -20.10091237387970153, 66.11910372887342646 ) ) ;
#1978=CARTESIAN_POINT ( 'NONE',  ( -19.37709988573221054, -21.53135720868301561, 62.29503678468425676 ) ) ;
#1980=CARTESIAN_POINT ( 'NONE',  ( -20.04849592361258104, -21.35284569240296548, 72.69006679631317525 ) ) ;
#1981=LINE ( 'NONE', #24159, #47153 ) ;
#1982=CARTESIAN_POINT ( 'NONE',  ( -12.21269597510284832, -10.13573543075226624, 60.66804197197834014 ) ) ;
#1983=( BOUNDED_CURVE ( )  B_SPLINE_CURVE ( 3, ( #30625, #34043, #23472, #30136 ),
 .UNSPECIFIED., .F., .F. ) 
 B_SPLINE_CURVE_WITH_KNOTS ( ( 4, 4 ),
 ( 4.712388980384689674, 4.921828490624008623 ),
 .UNSPECIFIED. ) 
 CURVE ( )  GEOMETRIC_REPRESENTATION_ITEM ( )  RATIONAL_B_SPLINE_CURVE ( ( 1.000000000000000000, 0.9963479302455156006, 0.9963479302455156006, 1.000000000000000000 ) ) 
 REPRESENTATION_ITEM ( '' )  );
#1985=EDGE_LOOP ( 'NONE', ( #44529, #25437, #11830, #4342 ) ) ;
#1986=EDGE_CURVE ( 'NONE', #15214, #38842, #45039, .T. ) ;
#1987=EDGE_CURVE ( 'NONE', #38799, #28542, #25823, .T. ) ;
#1988=CARTESIAN_POINT ( 'NONE',  ( -16.25451963475149952, -21.76959929332391397, 65.36997467570328979 ) ) ;
#1990=CARTESIAN_POINT ( 'NONE',  ( -13.03244235208782698, -8.791229364947284353, 64.00922890431560575 ) ) ;
#1992=FACE_OUTER_BOUND ( 'NONE', #28263, .T. ) ;
#1994=ORIENTED_EDGE ( 'NONE', *, *, #10445, .T. ) ;
#1995=VERTEX_POINT ( 'NONE', #22379 ) ;
#1996=ORIENTED_EDGE ( 'NONE', *, *, #29658, .T. ) ;
#1997=EDGE_CURVE ( 'NONE', #16426, #3920, #37880, .T. ) ;
#1998=CYLINDRICAL_SURFACE ( 'NONE', #35118, 0.1500000000000061007 ) ;
#1999=CARTESIAN_POINT ( 'NONE',  ( -22.53865852806102765, -10.02986705568149439, 70.23851888881135608 ) ) ;
#2000=CARTESIAN_POINT ( 'NONE',  ( -21.77718901952371766, -9.327210708589092292, 63.19153729619897319 ) ) ;
#2002=CARTESIAN_POINT ( 'NONE',  ( -10.52215087187021325, -13.37195826583270630, 74.67817647370829093 ) ) ;
#2005=CARTESIAN_POINT ( 'NONE',  ( -14.17008229276201625, -21.58685878473828268, 54.02312124697527906 ) ) ;
#2008=CARTESIAN_POINT ( 'NONE',  ( -16.84865286310842336, -21.83598151670433296, 68.98088545748413480 ) ) ;
#2009=ORIENTED_EDGE ( 'NONE', *, *, #14134, .T. ) ;
#2010=CARTESIAN_POINT ( 'NONE',  ( -10.82867520472564848, -11.34449427682889677, 67.73369198428547122 ) ) ;
#2016=ORIENTED_EDGE ( 'NONE', *, *, #28654, .F. ) ;
#2018=CARTESIAN_POINT ( 'NONE',  ( -14.61186971177858496, -7.910316301228372815, 60.51270451696741048 ) ) ;
#2019=CARTESIAN_POINT ( 'NONE',  ( -22.87594641915088900, -21.30847235828355579, 54.49999999999995026 ) ) ;
#2021=CARTESIAN_POINT ( 'NONE',  ( -18.60622205832422082, -22.16490843864383109, 72.47006330605313451 ) ) ;
#2022=B_SPLINE_CURVE_WITH_KNOTS ( 'NONE', 1,
 ( #3617, #8296 ),
 .UNSPECIFIED., .F., .F.,
 ( 2, 2 ),
 ( 0.000000000000000000, 1.000000000000000000 ),
 .UNSPECIFIED. ) ;
#2024=ORIENTED_EDGE ( 'NONE', *, *, #5945, .T. ) ;
#2026=CARTESIAN_POINT ( 'NONE',  ( -24.65205681464681930, -13.00370337554185340, 63.02538306434979631 ) ) ;
#2027=CARTESIAN_POINT ( 'NONE',  ( -24.86649340934961927, -14.46998543962672734, 66.30575816177258730 ) ) ;
#2028=CARTESIAN_POINT ( 'NONE',  ( -15.14827875528926349, -21.90310222313125266, 68.67618668865188170 ) ) ;
#2029=B_SPLINE_CURVE_WITH_KNOTS ( 'NONE', 1,
 ( #43508, #13438 ),
 .UNSPECIFIED., .F., .F.,
 ( 2, 2 ),
 ( 0.000000000000000000, 1.000000000000000000 ),
 .UNSPECIFIED. ) ;
#2030=CARTESIAN_POINT ( 'NONE',  ( -15.92022003474064995, -7.921321712309766561, 67.14567102837528978 ) ) ;
#2034=CARTESIAN_POINT ( 'NONE',  ( -22.66067231502460544, -10.16396745975044169, 66.73285430075826241 ) ) ;
#2035=EDGE_LOOP ( 'NONE', ( #12037, #14708, #12029, #7360, #35912 ) ) ;
#2038=CARTESIAN_POINT ( 'NONE',  ( -22.66414149941106260, -10.08832384041532926, 66.42693508874704378 ) ) ;
#2039=CYLINDRICAL_SURFACE ( 'NONE', #8558, 0.1499999999999953315 ) ;
#2040=CARTESIAN_POINT ( 'NONE',  ( -16.98134802626198336, -22.24608854931921087, 72.27204916158488857 ) ) ;
#2041=ORIENTED_EDGE ( 'NONE', *, *, #10651, .T. ) ;
#2043=CARTESIAN_POINT ( 'NONE',  ( -20.84119928492008000, -20.97572016636869918, 62.41471400470057773 ) ) ;
#2044=EDGE_CURVE ( 'NONE', #8287, #11201, #709, .T. ) ;
#2045=CARTESIAN_POINT ( 'NONE',  ( -20.63243265594276110, -8.084608023805090582, 63.42466202532494890 ) ) ;
#2046=ORIENTED_EDGE ( 'NONE', *, *, #2590, .T. ) ;
#2047=CARTESIAN_POINT ( 'NONE',  ( -9.981160085348813382, -14.48480431966832782, 68.00800125641796967 ) ) ;
#2048=CARTESIAN_POINT ( 'NONE',  ( -10.17575246482357088, -13.08756589590406172, 71.35828583495015209 ) ) ;
#2049=EDGE_CURVE ( 'NONE', #35577, #24336, #13021, .T. ) ;
#2050=ADVANCED_FACE ( 'NONE', ( #8109 ), #27287, .T. ) ;
#2051=CARTESIAN_POINT ( 'NONE',  ( -13.18362795047878144, -8.683667697493742565, 60.62445659250467145 ) ) ;
#2052=CARTESIAN_POINT ( 'NONE',  ( -20.81921389985186721, -21.44071754855728784, 58.75979745677555854 ) ) ;
#2054=CARTESIAN_POINT ( 'NONE',  ( -10.75774575360340002, -12.66857492743335634, 64.37909207168219439 ) ) ;
#2055=ORIENTED_EDGE ( 'NONE', *, *, #28089, .F. ) ;
#2056=ORIENTED_EDGE ( 'NONE', *, *, #23925, .F. ) ;
#2059=EDGE_CURVE ( 'NONE', #4075, #6465, #16471, .T. ) ;
#2060=CARTESIAN_POINT ( 'NONE',  ( -21.20019206555516078, -20.76270557045113208, 69.35450156465000759 ) ) ;
#2061=CARTESIAN_POINT ( 'NONE',  ( -15.43182990062313742, -8.046249867383863830, 74.36513541778452918 ) ) ;
#2062=B_SPLINE_CURVE_WITH_KNOTS ( 'NONE', 3,
 ( #46138, #45673, #26944, #4063, #42454, #841, #30653, #41964, #5027, #12163 ),
 .UNSPECIFIED., .F., .F.,
 ( 4, 2, 2, 2, 4 ),
 ( 0.000000000000000000, 0.2500000000000000000, 0.5000000000000000000, 0.7500000000000000000, 1.000000000000000000 ),
 .UNSPECIFIED. ) ;
#2063=B_SPLINE_CURVE_WITH_KNOTS ( 'NONE', 3,
 ( #40094, #19752, #10053, #30843, #31973, #23443, #47488, #6358, #15788, #25074 ),
 .UNSPECIFIED., .F., .F.,
 ( 4, 2, 2, 2, 4 ),
 ( 0.000000000000000000, 0.2500000000000000000, 0.5000000000000000000, 0.7500000000000000000, 1.000000000000000000 ),
 .UNSPECIFIED. ) ;
#2065=CARTESIAN_POINT ( 'NONE',  ( -24.32145319184211729, -17.62517394100480672, 66.13695529097154235 ) ) ;
#2066=VERTEX_POINT ( 'NONE', #4169 ) ;
#2067=CARTESIAN_POINT ( 'NONE',  ( -16.02724774380223849, -7.491242405164911133, 63.78515641179975404 ) ) ;
#2068=VERTEX_POINT ( 'NONE', #19665 ) ;
#2069=CARTESIAN_POINT ( 'NONE',  ( -24.42256168760463808, -14.59956870196896794, 66.37219723247810066 ) ) ;
#2070=CARTESIAN_POINT ( 'NONE',  ( -17.08524437268610896, -7.816974296902328589, 73.97634902203346030 ) ) ;
#2073=CARTESIAN_POINT ( 'NONE',  ( -10.55151208239364635, -17.68521041179895548, 68.28217381303441869 ) ) ;
#2074=ORIENTED_EDGE ( 'NONE', *, *, #44042, .T. ) ;
#2075=DIRECTION ( 'NONE',  ( -9.444166282346144476E-07, 1.975884201625194781E-06, 0.9999999999976019183 ) ) ;
#2078=CARTESIAN_POINT ( 'NONE',  ( -16.73854499263307716, -21.82594486583910864, 68.70120449160850740 ) ) ;
#2079=CARTESIAN_POINT ( 'NONE',  ( -11.04812374654697926, -17.69862217806955229, 71.86718199155660614 ) ) ;
#2080=ORIENTED_EDGE ( 'NONE', *, *, #22426, .F. ) ;
#2081=CARTESIAN_POINT ( 'NONE',  ( -14.31331640305492847, -8.538396089775591946, 67.36861181020977085 ) ) ;
#2082=CARTESIAN_POINT ( 'NONE',  ( -23.19494587819374942, -18.77118419879135303, 66.12389430422854275 ) ) ;
#2083=CYLINDRICAL_SURFACE ( 'NONE', #41994, 0.1500000000000002998 ) ;
#2086=DIRECTION ( 'NONE',  ( -0.02843338833657841139, 0.4463087971659328024, 0.8944271909999156334 ) ) ;
#2089=EDGE_CURVE ( 'NONE', #38102, #21018, #1580, .T. ) ;
#2090=DIRECTION ( 'NONE',  ( -7.105595949593054157E-06, -6.912614924914188927E-07, 0.9999999999745162738 ) ) ;
#2092=VERTEX_POINT ( 'NONE', #18668 ) ;
#2093=CARTESIAN_POINT ( 'NONE',  ( -13.89754221028031189, -8.246728053280408588, 74.29980400178126843 ) ) ;
#2094=CARTESIAN_POINT ( 'NONE',  ( -20.16691314815865255, -21.73601827195274794, 72.58974169946205279 ) ) ;
#2095=CARTESIAN_POINT ( 'NONE',  ( -24.29779380370725406, -16.39214576242591193, 62.68508962089565273 ) ) ;
#2096=ORIENTED_EDGE ( 'NONE', *, *, #6143, .T. ) ;
#2097=CARTESIAN_POINT ( 'NONE',  ( -19.74200936563730124, -21.46758226568296024, 68.94954551542706156 ) ) ;
#2098=ORIENTED_EDGE ( 'NONE', *, *, #46762, .T. ) ;
#2099=EDGE_LOOP ( 'NONE', ( #8926, #32290, #25724, #17549, #12791 ) ) ;
#2101=EDGE_CURVE ( 'NONE', #47078, #1710, #26793, .T. ) ;
#2102=CARTESIAN_POINT ( 'NONE',  ( -10.03204778417131315, -15.73800432700728891, 61.19822393253001991 ) ) ;
#2104=CYLINDRICAL_SURFACE ( 'NONE', #13770, 0.1500000000000006883 ) ;
#2105=B_SPLINE_CURVE_WITH_KNOTS ( 'NONE', 3,
 ( #5626, #18991, #19905, #8836, #31223, #12752, #12507, #20636, #1176, #35147 ),
 .UNSPECIFIED., .F., .F.,
 ( 4, 2, 2, 2, 4 ),
 ( 0.000000000000000000, 0.2500000000000000000, 0.5000000000000000000, 0.7500000000000000000, 1.000000000000000000 ),
 .UNSPECIFIED. ) ;
#2106=( BOUNDED_CURVE ( )  B_SPLINE_CURVE ( 3, ( #27989, #35377, #46720, #12962 ),
 .UNSPECIFIED., .F., .F. ) 
 B_SPLINE_CURVE_WITH_KNOTS ( ( 4, 4 ),
 ( 1.570796326794896780, 1.780235837034217727 ),
 .UNSPECIFIED. ) 
 CURVE ( )  GEOMETRIC_REPRESENTATION_ITEM ( )  RATIONAL_B_SPLINE_CURVE ( ( 1.000000000000000000, 0.9963479302455154896, 0.9963479302455154896, 1.000000000000000000 ) ) 
 REPRESENTATION_ITEM ( '' )  );
#2107=CYLINDRICAL_SURFACE ( 'NONE', #34581, 0.1499999999999994671 ) ;
#2108=CARTESIAN_POINT ( 'NONE',  ( -19.83021825064065524, -21.38439211167239051, 72.52195586376959113 ) ) ;
#2109=CARTESIAN_POINT ( 'NONE',  ( -10.74141492653277119, -16.89327574454988223, 57.68760574265544250 ) ) ;
#2111=ORIENTED_EDGE ( 'NONE', *, *, #20851, .T. ) ;
#2114=CARTESIAN_POINT ( 'NONE',  ( -24.28619334359350290, -16.42731978468327014, 59.13804568661029037 ) ) ;
#2116=EDGE_CURVE ( 'NONE', #32914, #3385, #19945, .T. ) ;
#2118=B_SPLINE_CURVE_WITH_KNOTS ( 'NONE', 1,
 ( #25903, #37199 ),
 .UNSPECIFIED., .F., .F.,
 ( 2, 2 ),
 ( 0.000000000000000000, 1.000000000000000000 ),
 .UNSPECIFIED. ) ;
#2119=( BOUNDED_CURVE ( )  B_SPLINE_CURVE ( 3, ( #13062, #28100, #41735, #30667 ),
 .UNSPECIFIED., .F., .F. ) 
 B_SPLINE_CURVE_WITH_KNOTS ( ( 4, 4 ),
 ( 0.4074455897393666204, 0.5000000000000000000 ),
 .UNSPECIFIED. ) 
 CURVE ( )  GEOMETRIC_REPRESENTATION_ITEM ( )  RATIONAL_B_SPLINE_CURVE ( ( 0.6983129098260953960, 0.7760317562607160768, 0.8765941196520221634, 1.000000000000025091 ) ) 
 REPRESENTATION_ITEM ( '' )  );
#2124=CARTESIAN_POINT ( 'NONE',  ( -10.47425561207849753, -17.49314520081206936, 64.81234810402725088 ) ) ;
#2126=CYLINDRICAL_SURFACE ( 'NONE', #37468, 0.1499999999999955536 ) ;
#2127=CARTESIAN_POINT ( 'NONE',  ( -22.39379392724509898, -9.879492423591733186, 73.59047181297640350 ) ) ;
#2128=CARTESIAN_POINT ( 'NONE',  ( -16.24765015213137076, -21.70976432975602677, 58.58585518740712672 ) ) ;
#2130=CARTESIAN_POINT ( 'NONE',  ( -19.99112905230247961, -8.296885111154901793, 73.72096600045514947 ) ) ;
#2133=ORIENTED_EDGE ( 'NONE', *, *, #7357, .T. ) ;
#2136=CYLINDRICAL_SURFACE ( 'NONE', #21103, 0.1500000000000035194 ) ;
#2138=EDGE_LOOP ( 'NONE', ( #7753, #21053, #39584, #11585, #9532 ) ) ;
#2141=CARTESIAN_POINT ( 'NONE',  ( -24.48810873059073856, -17.17637193698283582, 73.06831349224263761 ) ) ;
#2142=CARTESIAN_POINT ( 'NONE',  ( -21.19137721460013779, -21.23655545966798996, 65.77792262113059962 ) ) ;
#2144=CARTESIAN_POINT ( 'NONE',  ( -22.06133474718976117, -9.563836317021298328, 59.79341455809256445 ) ) ;
#2145=CARTESIAN_POINT ( 'NONE',  ( -11.29134393598116759, -11.33126488396075437, 64.16354160640879911 ) ) ;
#2147=ORIENTED_EDGE ( 'NONE', *, *, #36326, .F. ) ;
#2148=FACE_OUTER_BOUND ( 'NONE', #24875, .T. ) ;
#2151=CARTESIAN_POINT ( 'NONE',  ( -12.05749060505181269, -9.640721912800795934, 60.74573338552316670 ) ) ;
#2152=ORIENTED_EDGE ( 'NONE', *, *, #31958, .T. ) ;
#2153=VERTEX_POINT ( 'NONE', #42569 ) ;
#2155=CARTESIAN_POINT ( 'NONE',  ( -11.45752044641470668, -19.27057170535650954, 71.87181270239314301 ) ) ;
#2157=CARTESIAN_POINT ( 'NONE',  ( -13.43773910423563400, -20.62433115109003268, 58.33177939114180788 ) ) ;
#2160=CARTESIAN_POINT ( 'NONE',  ( -18.32857646159318676, -22.20418385865972155, 68.93019298464047040 ) ) ;
#2161=CARTESIAN_POINT ( 'NONE',  ( -19.48828226429125365, -21.49800194790059038, 62.28038260443739205 ) ) ;
#2162=CARTESIAN_POINT ( 'NONE',  ( -23.81024772113315890, -18.64597811008791695, 72.94863512192290500 ) ) ;
#2163=DIRECTION ( 'NONE',  ( 2.654446662475610288E-06, -3.134491601460476904E-06, 0.9999999999915645255 ) ) ;
#2164=CARTESIAN_POINT ( 'NONE',  ( -13.90650143624606017, -21.37666829811961478, 72.08641044951055221 ) ) ;
#2165=ORIENTED_EDGE ( 'NONE', *, *, #6143, .F. ) ;
#2166=ORIENTED_EDGE ( 'NONE', *, *, #44966, .F. ) ;
#2167=EDGE_CURVE ( 'NONE', #3943, #30787, #25048, .T. ) ;
#2168=CARTESIAN_POINT ( 'NONE',  ( -24.31477923169101629, -16.30090137217950996, 59.40860294853779777 ) ) ;
#2170=CARTESIAN_POINT ( 'NONE',  ( -19.42045769886998841, -21.57377358197381412, 65.87974951360257592 ) ) ;
#2171=CARTESIAN_POINT ( 'NONE',  ( -13.47433711440449144, -8.491526086692950059, 57.15623147539552917 ) ) ;
#2173=CARTESIAN_POINT ( 'NONE',  ( -20.88270717056239789, -21.40782548341276481, 58.82970473467946704 ) ) ;
#2175=ORIENTED_EDGE ( 'NONE', *, *, #39104, .F. ) ;
#2176=CARTESIAN_POINT ( 'NONE',  ( -23.27284462870851911, -18.74605969774991010, 66.10917289053097079 ) ) ;
#2177=DIRECTION ( 'NONE',  ( 0.02400335114476204179, -0.9997118780597843424, -1.529429985666831130E-10 ) ) ;
#2180=CARTESIAN_POINT ( 'NONE',  ( -18.17062816029565653, -22.22171889179154292, 65.44508531174115262 ) ) ;
#2183=CARTESIAN_POINT ( 'NONE',  ( -10.14072131497136198, -13.24157352934983578, 74.83964170301820218 ) ) ;
#2185=ADVANCED_FACE ( 'NONE', ( #34911 ), #10463, .T. ) ;
#2186=CARTESIAN_POINT ( 'NONE',  ( -14.74690617566109019, -21.27702427001963414, 58.46617884968173229 ) ) ;
#2187=ADVANCED_FACE ( 'NONE', ( #13640 ), #40259, .T. ) ;
#2188=CARTESIAN_POINT ( 'NONE',  ( -17.72612443559818018, -7.765381109175947927, 60.36588690973874094 ) ) ;
#2189=VECTOR ( 'NONE', #17984, 1000.000000000000227 ) ;
#2190=CARTESIAN_POINT ( 'NONE',  ( -15.62840352080693407, -7.578723969186683895, 70.73272974284665793 ) ) ;
#2191=CARTESIAN_POINT ( 'NONE',  ( -11.09893839327029674, -10.87261039219572289, 57.38620067505767963 ) ) ;
#2192=CARTESIAN_POINT ( 'NONE',  ( -24.39763799706551950, -15.84669482609578317, 69.54779622430706354 ) ) ;
#2193=EDGE_LOOP ( 'NONE', ( #17391, #27532, #19360, #48710, #15901 ) ) ;
#2194=CARTESIAN_POINT ( 'NONE',  ( -17.42409385541300892, -14.80920654474439324, 54.49999999999995026 ) ) ;
#2196=EDGE_LOOP ( 'NONE', ( #24186, #38155, #39682, #34907, #5739 ) ) ;
#2197=CARTESIAN_POINT ( 'NONE',  ( -13.60238289842205894, -8.884932333444998775, 57.26967755503795132 ) ) ;
#2198=CARTESIAN_POINT ( 'NONE',  ( -12.68532267716109985, -9.060482739934947460, 71.03420753023118550 ) ) ;
#2199=ORIENTED_EDGE ( 'NONE', *, *, #8542, .T. ) ;
#2201=EDGE_LOOP ( 'NONE', ( #2898, #13217, #22546, #31209, #5524 ) ) ;
#2202=CARTESIAN_POINT ( 'NONE',  ( -10.88209242003807908, -17.29963164818252608, 64.62739380462950578 ) ) ;
#2203=CARTESIAN_POINT ( 'NONE',  ( -16.59509239138002101, -21.81331869282671221, 61.64079261740195648 ) ) ;
#2204=B_SPLINE_CURVE_WITH_KNOTS ( 'NONE', 1,
 ( #8286, #38293 ),
 .UNSPECIFIED., .F., .F.,
 ( 2, 2 ),
 ( 0.000000000000000000, 1.000000000000000000 ),
 .UNSPECIFIED. ) ;
#2205=VERTEX_POINT ( 'NONE', #6277 ) ;
#2207=FACE_OUTER_BOUND ( 'NONE', #30152, .T. ) ;
#2210=EDGE_LOOP ( 'NONE', ( #34424, #7088, #36305, #33321, #23569 ) ) ;
#2212=CARTESIAN_POINT ( 'NONE',  ( -11.70705814868712835, -18.84866425382743671, 68.21689578225554840 ) ) ;
#2213=CARTESIAN_POINT ( 'NONE',  ( -21.30368986256526043, -21.17021271237730318, 69.24105570176159574 ) ) ;
#2216=CARTESIAN_POINT ( 'NONE',  ( -17.74687306060290837, -7.816529701066174951, 60.08060757092961524 ) ) ;
#2220=AXIS2_PLACEMENT_3D ( 'NONE', #12101, #45356, #41402 ) ;
#2222=CARTESIAN_POINT ( 'NONE',  ( -12.40526392040721682, -9.927684496520663870, 60.63088272232361930 ) ) ;
#2223=AXIS2_PLACEMENT_3D ( 'NONE', #6931, #44372, #25887 ) ;
#2225=ADVANCED_FACE ( 'NONE', ( #32615 ), #13400, .T. ) ;
#2226=CARTESIAN_POINT ( 'NONE',  ( -22.14133254371160930, -20.05921860014851532, 69.31850691956374533 ) ) ;
#2228=CARTESIAN_POINT ( 'NONE',  ( -12.47302444406249933, -9.241390648102244754, 74.43267637782378188 ) ) ;
#2230=ORIENTED_EDGE ( 'NONE', *, *, #32245, .F. ) ;
#2231=B_SPLINE_CURVE_WITH_KNOTS ( 'NONE', 3,
 ( #37857, #11767, #26788, #41811, #37349, #23099, #18640, #4371, #19389, #33652 ),
 .UNSPECIFIED., .F., .F.,
 ( 4, 2, 2, 2, 4 ),
 ( 0.000000000000000000, 0.2500000000000000000, 0.5000000000000000000, 0.7500000000000000000, 1.000000000000000000 ),
 .UNSPECIFIED. ) ;
#2234=CARTESIAN_POINT ( 'NONE',  ( -19.83346284351035393, -21.43866980266018274, 65.46486087551818400 ) ) ;
#2236=( BOUNDED_CURVE ( )  B_SPLINE_CURVE ( 3, ( #4241, #12585, #19980, #5455 ),
 .UNSPECIFIED., .F., .F. ) 
 B_SPLINE_CURVE_WITH_KNOTS ( ( 4, 4 ),
 ( 0.000000000000000000, 0.4074455897393641779 ),
 .UNSPECIFIED. ) 
 CURVE ( )  GEOMETRIC_REPRESENTATION_ITEM ( )  RATIONAL_B_SPLINE_CURVE ( ( 1.000000000000000000, 0.4567392136813311909, 0.3561768502900300448, 0.6983129098260966172 ) ) 
 REPRESENTATION_ITEM ( '' )  );
#2238=ADVANCED_FACE ( 'NONE', ( #32141 ), #2953, .T. ) ;
#2240=CARTESIAN_POINT ( 'NONE',  ( -10.00761937521931522, -15.51608998476985946, 57.75288115419267854 ) ) ;
#2241=ADVANCED_FACE ( 'NONE', ( #47640 ), #6431, .T. ) ;
#2243=VERTEX_POINT ( 'NONE', #10690 ) ;
#2244=CARTESIAN_POINT ( 'NONE',  ( -11.35719102664687874, -18.40077844947705543, 58.09242476654641507 ) ) ;
#2245=AXIS2_PLACEMENT_3D ( 'NONE', #4042, #46368, #1060 ) ;
#2246=CARTESIAN_POINT ( 'NONE',  ( -12.88266153074016529, -9.482350759114249072, 70.95811324639576867 ) ) ;
#2249=CARTESIAN_POINT ( 'NONE',  ( -22.71059208588729561, -10.14448404190931186, 70.02650598627910483 ) ) ;
#2250=ORIENTED_EDGE ( 'NONE', *, *, #12608, .T. ) ;
#2251=( BOUNDED_CURVE ( )  B_SPLINE_CURVE ( 3, ( #18763, #44636, #21976, #3260 ),
 .UNSPECIFIED., .F., .F. ) 
 B_SPLINE_CURVE_WITH_KNOTS ( ( 4, 4 ),
 ( 0.000000000000000000, 0.4074455897279358751 ),
 .UNSPECIFIED. ) 
 CURVE ( )  GEOMETRIC_REPRESENTATION_ITEM ( )  RATIONAL_B_SPLINE_CURVE ( ( 1.000000000000000000, 0.4567392136965727767, 0.3561768502956727533, 0.6983129097972999855 ) ) 
 REPRESENTATION_ITEM ( '' )  );
#2254=ORIENTED_EDGE ( 'NONE', *, *, #41350, .F. ) ;
#2255=CARTESIAN_POINT ( 'NONE',  ( -15.95707318215220205, -7.504986700048139170, 63.85506303619484214 ) ) ;
#2257=LINE ( 'NONE', #12616, #35981 ) ;
#2258=VERTEX_POINT ( 'NONE', #34061 ) ;
#2260=CARTESIAN_POINT ( 'NONE',  ( -24.21281492007539526, -12.87834259335418530, 73.38658464541695992 ) ) ;
#2261=CARTESIAN_POINT ( 'NONE',  ( -13.01616685277437568, -9.306763517318225709, 70.86397465682092900 ) ) ;
#2262=AXIS2_PLACEMENT_3D ( 'NONE', #44784, #42047, #11034 ) ;
#2264=CARTESIAN_POINT ( 'NONE',  ( -10.45720011525486015, -15.50224624050967037, 61.10959345291067280 ) ) ;
#2268=( BOUNDED_CURVE ( )  B_SPLINE_CURVE ( 3, ( #46000, #11783, #4161, #5121 ),
 .UNSPECIFIED., .F., .F. ) 
 B_SPLINE_CURVE_WITH_KNOTS ( ( 4, 4 ),
 ( 0.5000000000000000000, 0.9074455897393647330 ),
 .UNSPECIFIED. ) 
 CURVE ( )  GEOMETRIC_REPRESENTATION_ITEM ( )  RATIONAL_B_SPLINE_CURVE ( ( 1.000000000000011324, 0.4567392136813218095, 0.3561768502900186650, 0.6983129098261137147 ) ) 
 REPRESENTATION_ITEM ( '' )  );
#2269=CARTESIAN_POINT ( 'NONE',  ( -24.66912536856318994, -13.07314766736345746, 62.95547313412625101 ) ) ;
#2270=DIRECTION ( 'NONE',  ( 0.5729733056696845184, -0.8195740302071247152, -7.403245353804670970E-08 ) ) ;
#2271=LINE ( 'NONE', #14047, #18701 ) ;
#2272=CARTESIAN_POINT ( 'NONE',  ( -15.87557863975121641, -7.931372594209569193, 67.14007279017359053 ) ) ;
#2275=VERTEX_POINT ( 'NONE', #14350 ) ;
#2277=CARTESIAN_POINT ( 'NONE',  ( -24.82492784865917201, -15.66438054851105832, 73.25949685721523963 ) ) ;
#2279=CARTESIAN_POINT ( 'NONE',  ( -10.36968235478426870, -15.03336378326449285, 71.48349971081816534 ) ) ;
#2280=FACE_OUTER_BOUND ( 'NONE', #266, .T. ) ;
#2282=CARTESIAN_POINT ( 'NONE',  ( -22.62394951084894146, -10.04809318868971424, 70.29706442286226320 ) ) ;
#2284=ORIENTED_EDGE ( 'NONE', *, *, #40405, .F. ) ;
#2285=CARTESIAN_POINT ( 'NONE',  ( -24.83515304063678286, -14.04764234229505959, 73.23776096988058271 ) ) ;
#2287=EDGE_LOOP ( 'NONE', ( #25145, #9987, #602, #9804, #31501 ) ) ;
#2291=AXIS2_PLACEMENT_3D ( 'NONE', #23123, #45785, #8341 ) ;
#2292=CARTESIAN_POINT ( 'NONE',  ( -13.33887157028844150, -9.124797958614562887, 64.20946578470248767 ) ) ;
#2294=CARTESIAN_POINT ( 'NONE',  ( -24.14992822999210276, -18.01341164000503525, 59.11882993461590274 ) ) ;
#2295=FACE_OUTER_BOUND ( 'NONE', #8756, .T. ) ;
#2296=CARTESIAN_POINT ( 'NONE',  ( -11.52367966561213386, -11.04268899456634578, 57.20903262758894670 ) ) ;
#2302=CARTESIAN_POINT ( 'NONE',  ( -10.37462440636232053, -14.89569459299594278, 75.09778901493891112 ) ) ;
#2303=CARTESIAN_POINT ( 'NONE',  ( -12.83203711565397676, -20.76220377597121214, 54.02312124697528617 ) ) ;
#2307=CARTESIAN_POINT ( 'NONE',  ( -12.12094469647606942, -10.15824389949702322, 60.55918111604575671 ) ) ;
#2308=ORIENTED_EDGE ( 'NONE', *, *, #39276, .T. ) ;
#2309=FACE_OUTER_BOUND ( 'NONE', #25049, .T. ) ;
#2311=ORIENTED_EDGE ( 'NONE', *, *, #21050, .T. ) ;
#2312=CARTESIAN_POINT ( 'NONE',  ( -17.98584164848810474, -22.23808382151284491, 62.06031347038508983 ) ) ;
#2313=CARTESIAN_POINT ( 'NONE',  ( -17.08524326626993428, -7.816974356186509709, 74.24401709311408126 ) ) ;
#2316=ADVANCED_FACE ( 'NONE', ( #14586 ), #37255, .T. ) ;
#2318=CARTESIAN_POINT ( 'NONE',  ( -18.50162202296811742, -21.72577595440482057, 72.28510940981611554 ) ) ;
#2319=EDGE_LOOP ( 'NONE', ( #48567, #44736, #34467, #39848, #16752 ) ) ;
#2320=FACE_OUTER_BOUND ( 'NONE', #24702, .T. ) ;
#2321=ADVANCED_FACE ( 'NONE', ( #37503 ), #9879, .T. ) ;
#2322=CARTESIAN_POINT ( 'NONE',  ( -24.83498170362974022, -14.04605013716215822, 73.37917436033832530 ) ) ;
#2323=ADVANCED_FACE ( 'NONE', ( #37756 ), #40479, .T. ) ;
#2324=CARTESIAN_POINT ( 'NONE',  ( -15.49416032233947682, -8.028509233753512220, 74.07985659018983426 ) ) ;
#2325=CARTESIAN_POINT ( 'NONE',  ( -22.57384314992541263, -19.55061350403557441, 72.87073974848900093 ) ) ;
#2326=ORIENTED_EDGE ( 'NONE', *, *, #20906, .F. ) ;
#2327=DIRECTION ( 'NONE',  ( -0.9991556020692448081, 0.04108628546905851442, 9.785000776664589550E-17 ) ) ;
#2330=PLANE ( 'NONE',  #34101 ) ;
#2331=CARTESIAN_POINT ( 'NONE',  ( -11.96181355942711910, -19.87549434724351727, 58.11177690156993947 ) ) ;
#2332=B_SPLINE_CURVE_WITH_KNOTS ( 'NONE', 3,
 ( #45193, #8016, #18564, #15600, #44699, #38013, #22036, #25974, #34314, #37032 ),
 .UNSPECIFIED., .F., .F.,
 ( 4, 2, 2, 2, 4 ),
 ( 0.6272669072877752328, 0.7522669073072968393, 0.8772669073268184459, 1.002266907346339941, 1.127266907365861659 ),
 .UNSPECIFIED. ) ;
#2335=CARTESIAN_POINT ( 'NONE',  ( -16.85302834907681557, -22.23803867529147738, 68.80905311428833215 ) ) ;
#2336=CARTESIAN_POINT ( 'NONE',  ( -23.58616457878146377, -18.99640866789479432, 66.00884704819274873 ) ) ;
#2337=ORIENTED_EDGE ( 'NONE', *, *, #735, .F. ) ;
#2339=AXIS2_PLACEMENT_3D ( 'NONE', #46570, #16501, #17223 ) ;
#2341=CARTESIAN_POINT ( 'NONE',  ( -13.29033873113971076, -20.46027459610395027, 58.15723269990255062 ) ) ;
#2344=VERTEX_POINT ( 'NONE', #35030 ) ;
#2345=ORIENTED_EDGE ( 'NONE', *, *, #44104, .T. ) ;
#2346=EDGE_LOOP ( 'NONE', ( #48110, #34485, #12786, #14619, #18151 ) ) ;
#2347=CARTESIAN_POINT ( 'NONE',  ( -16.17465015159496744, -21.74764722426833075, 58.28585602925419806 ) ) ;
#2348=CARTESIAN_POINT ( 'NONE',  ( -23.11004562739756096, -18.89484649831948104, 66.01316609496412013 ) ) ;
#2349=CARTESIAN_POINT ( 'NONE',  ( -17.46222794319647775, -7.759011850482251837, 67.03511641684839617 ) ) ;
#2350=CARTESIAN_POINT ( 'NONE',  ( -17.18480517372767125, -21.85814792571105514, 72.05054515682328997 ) ) ;
#2353=VERTEX_POINT ( 'NONE', #34298 ) ;
#2356=CARTESIAN_POINT ( 'NONE',  ( -18.55956930788366677, -7.446158750330262421, 74.02559786541287679 ) ) ;
#2357=DIRECTION ( 'NONE',  ( 0.4846961512978548159, 0.8746825943832683414, 4.196010046976494103E-08 ) ) ;
#2358=VECTOR ( 'NONE', #20615, 999.9999999999998863 ) ;
#2359=EDGE_CURVE ( 'NONE', #46199, #23813, #14442, .T. ) ;
#2364=CARTESIAN_POINT ( 'NONE',  ( -10.37406300525030645, -14.84993649218493417, 74.80338706735179244 ) ) ;
#2365=CARTESIAN_POINT ( 'NONE',  ( -24.87406966366976135, -14.83187089386463775, 59.34276618600990361 ) ) ;
#2367=VERTEX_POINT ( 'NONE', #11921 ) ;
#2369=ORIENTED_EDGE ( 'NONE', *, *, #38500, .F. ) ;
#2372=CARTESIAN_POINT ( 'NONE',  ( -22.28468842640968006, -19.91619389767071269, 65.98949666203347419 ) ) ;
#2373=EDGE_CURVE ( 'NONE', #2586, #15392, #2704, .T. ) ;
#2374=VERTEX_POINT ( 'NONE', #5018 ) ;
#2378=CARTESIAN_POINT ( 'NONE',  ( -23.12302755141047683, -18.95946607990388699, 62.50406880580509750 ) ) ;
#2380=CARTESIAN_POINT ( 'NONE',  ( -24.83168737706420615, -15.60343295348776138, 73.10965427473990985 ) ) ;
#2381=CARTESIAN_POINT ( 'NONE',  ( -24.47853618617655158, -14.58602005854247174, 69.79708117814310242 ) ) ;
#2382=ORIENTED_EDGE ( 'NONE', *, *, #22006, .T. ) ;
#2383=CARTESIAN_POINT ( 'NONE',  ( -13.35685195715142193, -21.05109796036597913, 61.56000367517481919 ) ) ;
#2384=FACE_OUTER_BOUND ( 'NONE', #40725, .T. ) ;
#2385=ORIENTED_EDGE ( 'NONE', *, *, #5184, .T. ) ;
#2386=CARTESIAN_POINT ( 'NONE',  ( -13.17196901619666605, -8.691656238230125453, 60.57803720896963995 ) ) ;
#2387=CARTESIAN_POINT ( 'NONE',  ( -24.65023647254185590, -12.99629722456026393, 63.01759562046499497 ) ) ;
#2388=CARTESIAN_POINT ( 'NONE',  ( -24.16424020987968646, -16.88652737071335252, 72.76847378359866525 ) ) ;
#2389=B_SPLINE_CURVE_WITH_KNOTS ( 'NONE', 3,
 ( #16166, #12963, #20127, #19890, #19650, #42784, #31208, #15689, #34894, #1162 ),
 .UNSPECIFIED., .F., .F.,
 ( 4, 2, 2, 2, 4 ),
 ( 0.6272669072977071769, 0.7522669073147385532, 0.8772669073317700406, 1.002266907348801528, 1.127266907365832793 ),
 .UNSPECIFIED. ) ;
#2390=VECTOR ( 'NONE', #515, 1000.000000000000114 ) ;
#2392=ORIENTED_EDGE ( 'NONE', *, *, #47249, .F. ) ;
#2393=CYLINDRICAL_SURFACE ( 'NONE', #9540, 0.1500000000000057399 ) ;
#2395=CARTESIAN_POINT ( 'NONE',  ( -24.14981099001045095, -11.60321323961852258, 59.59580478148293992 ) ) ;
#2396=( BOUNDED_CURVE ( )  B_SPLINE_CURVE ( 3, ( #17141, #5621, #9554, #35389 ),
 .UNSPECIFIED., .F., .F. ) 
 B_SPLINE_CURVE_WITH_KNOTS ( ( 4, 4 ),
 ( 0.9074455897393687298, 1.000000000000000000 ),
 .UNSPECIFIED. ) 
 CURVE ( )  GEOMETRIC_REPRESENTATION_ITEM ( )  RATIONAL_B_SPLINE_CURVE ( ( 0.6983129098261148249, 0.7760317562607169650, 0.8765941196520120604, 1.000000000000000000 ) ) 
 REPRESENTATION_ITEM ( '' )  );
#2397=CARTESIAN_POINT ( 'NONE',  ( -10.83536385990051798, -17.31742045656482176, 64.77739380450887552 ) ) ;
#2401=CARTESIAN_POINT ( 'NONE',  ( -12.00971629994662493, -9.691756596678954949, 60.67422760384662439 ) ) ;
#2403=EDGE_LOOP ( 'NONE', ( #47008, #18455, #19113, #12704, #9164 ) ) ;
#2404=CARTESIAN_POINT ( 'NONE',  ( -24.18037300165767434, -17.94870813986570113, 59.18873840842728384 ) ) ;
#2405=CARTESIAN_POINT ( 'NONE',  ( -13.11130243257871264, -9.228466417706050251, 63.79457649077198056 ) ) ;
#2406=CARTESIAN_POINT ( 'NONE',  ( -10.02292926433220011, -15.66126330378499176, 61.23127357194864828 ) ) ;
#2410=CARTESIAN_POINT ( 'NONE',  ( -23.52949419687348964, -11.28347464189849703, 70.17738639980606763 ) ) ;
#2412=CARTESIAN_POINT ( 'NONE',  ( -12.22131315432520537, -20.14153059940332824, 65.06686082697517293 ) ) ;
#2413=( BOUNDED_SURFACE ( )  B_SPLINE_SURFACE ( 3, 1, ( 
 ( #12751, #39335 ),
 ( #46962, #12506 ),
 ( #27527, #43286 ),
 ( #42566, #8835 ),
 ( #23848, #27770 ),
 ( #38849, #14404 ),
 ( #44496, #44262 ) ),
 .UNSPECIFIED., .T., .F., .F. ) 
 B_SPLINE_SURFACE_WITH_KNOTS ( ( 4, 3, 4 ),
 ( 2, 2 ),
 ( 0.000000000000000000, 0.5000000000000000000, 1.000000000000000000 ),
 ( 0.000000000000000000, 1.000000000000000000 ),
 .UNSPECIFIED. ) 
 GEOMETRIC_REPRESENTATION_ITEM ( )  RATIONAL_B_SPLINE_SURFACE ( (
 ( 1.000000000000000000, 1.000000000000000000),
 ( 0.3333333333333335369, 0.3333333333333330373),
 ( 0.3333333333333335369, 0.3333333333333330373),
 ( 1.000000000000000000, 1.000000000000000000),
 ( 0.3333333333333333703, 0.3333333333333333703),
 ( 0.3333333333333333703, 0.3333333333333333703),
 ( 1.000000000000000000, 1.000000000000000000) ) ) 
 REPRESENTATION_ITEM ( '' )  SURFACE ( )  );
#2414=CARTESIAN_POINT ( 'NONE',  ( -23.20936678059565494, -18.85217346302747643, 59.03977614772677640 ) ) ;
#2419=CARTESIAN_POINT ( 'NONE',  ( -23.08461988266076048, -9.965480423839858659, 66.64843946037336764 ) ) ;
#2420=B_SPLINE_CURVE_WITH_KNOTS ( 'NONE', 1,
 ( #45954, #34611 ),
 .UNSPECIFIED., .F., .F.,
 ( 2, 2 ),
 ( 0.000000000000000000, 1.000000000000000000 ),
 .UNSPECIFIED. ) ;
#2421=CARTESIAN_POINT ( 'NONE',  ( -27.51331730537552289, -17.63476259924578926, 53.49999999999995026 ) ) ;
#2422=CARTESIAN_POINT ( 'NONE',  ( -10.99934521469463888, -17.58926687486790641, 71.85101586268936558 ) ) ;
#2423=CARTESIAN_POINT ( 'NONE',  ( -11.09028998197301874, -11.82864193257709751, 71.10363318086781703 ) ) ;
#2424=ADVANCED_FACE ( 'NONE', ( #31599 ), #4517, .T. ) ;
#2427=CARTESIAN_POINT ( 'NONE',  ( -20.16691211377460391, -21.73601867580754288, 72.58974061177721637 ) ) ;
#2430=CARTESIAN_POINT ( 'NONE',  ( -16.43682605374082684, -21.78988669087135222, 62.05008312678486249 ) ) ;
#2431=CARTESIAN_POINT ( 'NONE',  ( -10.43098718212803000, -15.70539730037032911, 61.32316937334011442 ) ) ;
#2432=ORIENTED_EDGE ( 'NONE', *, *, #42135, .F. ) ;
#2436=EDGE_CURVE ( 'NONE', #36242, #8916, #22700, .T. ) ;
#2437=CARTESIAN_POINT ( 'NONE',  ( -15.61268995836261375, -7.582723730348911673, 70.80328162622285504 ) ) ;
#2438=ADVANCED_FACE ( 'NONE', ( #46128 ), #46378, .T. ) ;
#2439=PLANE ( 'NONE',  #31439 ) ;
#2440=ORIENTED_EDGE ( 'NONE', *, *, #5872, .F. ) ;
#2441=CARTESIAN_POINT ( 'NONE',  ( -20.72573862760241070, -8.580110178657996300, 60.14125250079693785 ) ) ;
#2442=ORIENTED_EDGE ( 'NONE', *, *, #5184, .F. ) ;
#2443=CARTESIAN_POINT ( 'NONE',  ( -24.36926384684218050, -16.02131533650774031, 66.06884749925394829 ) ) ;
#2445=EDGE_CURVE ( 'NONE', #22471, #22864, #30025, .T. ) ;
#2446=VERTEX_POINT ( 'NONE', #23974 ) ;
#2449=CARTESIAN_POINT ( 'NONE',  ( -12.56171917241870695, -20.45376946399996854, 71.99148991968543498 ) ) ;
#2450=ORIENTED_EDGE ( 'NONE', *, *, #9696, .T. ) ;
#2452=EDGE_CURVE ( 'NONE', #3868, #47072, #33150, .T. ) ;
#2453=CARTESIAN_POINT ( 'NONE',  ( -10.64577744754535082, -11.71757184301072563, 74.67344733366148546 ) ) ;
#2454=CARTESIAN_POINT ( 'NONE',  ( -24.86287066056264550, -14.39952644145777327, 66.28954435112517274 ) ) ;
#2457=CARTESIAN_POINT ( 'NONE',  ( -17.19980177718173309, -7.762775310937221285, 70.49035839668022163 ) ) ;
#2460=CARTESIAN_POINT ( 'NONE',  ( -11.31430947714633994, -19.07219073454920277, 68.36689628406799102 ) ) ;
#2461=VERTEX_POINT ( 'NONE', #9440 ) ;
#2462=ORIENTED_EDGE ( 'NONE', *, *, #320, .T. ) ;
#2463=CARTESIAN_POINT ( 'NONE',  ( -11.72760323093659807, -18.87748041585143710, 68.50224213730197675 ) ) ;
#2464=CARTESIAN_POINT ( 'NONE',  ( -11.01197672498281044, -17.74032467813711733, 71.85246142747087106 ) ) ;
#2468=CARTESIAN_POINT ( 'NONE',  ( -22.88264614489240856, -10.34704276773305764, 63.35713876973677827 ) ) ;
#2469=EDGE_CURVE ( 'NONE', #20234, #33331, #5750, .T. ) ;
#2470=CARTESIAN_POINT ( 'NONE',  ( -13.89388974506275787, -21.36980381032900667, 72.11102993026078423 ) ) ;
#2471=CARTESIAN_POINT ( 'NONE',  ( -15.55171241031346696, -7.598245096497682205, 70.79485117658632021 ) ) ;
#2472=EDGE_CURVE ( 'NONE', #18626, #38687, #28140, .T. ) ;
#2473=ORIENTED_EDGE ( 'NONE', *, *, #41030, .T. ) ;
#2474=CYLINDRICAL_SURFACE ( 'NONE', #6091, 0.1499999999999986899 ) ;
#2477=CARTESIAN_POINT ( 'NONE',  ( -22.83135259498468628, -9.684349502702678691, 73.68172289069366343 ) ) ;
#2479=EDGE_CURVE ( 'NONE', #1105, #31075, #36241, .T. ) ;
#2480=ORIENTED_EDGE ( 'NONE', *, *, #3951, .F. ) ;
#2482=CARTESIAN_POINT ( 'NONE',  ( -17.56717618076180187, -7.360494862701306928, 63.73552352176282909 ) ) ;
#2483=AXIS2_PLACEMENT_3D ( 'NONE', #18053, #41205, #10682 ) ;
#2484=CARTESIAN_POINT ( 'NONE',  ( -22.63008487438422733, -10.12971324841507581, 70.31178520543817001 ) ) ;
#2488=B_SPLINE_CURVE_WITH_KNOTS ( 'NONE', 1,
 ( #31694, #45991 ),
 .UNSPECIFIED., .F., .F.,
 ( 2, 2 ),
 ( 0.000000000000000000, 1.000000000000000000 ),
 .UNSPECIFIED. ) ;
#2489=DIRECTION ( 'NONE',  ( -0.6771828760946863035, 0.7358147540815750398, -3.419290845356464001E-09 ) ) ;
#2491=CARTESIAN_POINT ( 'NONE',  ( -10.92672688430831229, -11.16395088679539249, 64.40527978002718612 ) ) ;
#2492=VERTEX_POINT ( 'NONE', #31837 ) ;
#2494=CARTESIAN_POINT ( 'NONE',  ( -23.56592830594333421, -19.02588402289573466, 65.97389426991706785 ) ) ;
#2495=CARTESIAN_POINT ( 'NONE',  ( -12.96547641683174312, -9.412684695659720546, 71.14925319132085235 ) ) ;
#2496=CARTESIAN_POINT ( 'NONE',  ( -15.88655729437939534, -7.980152340574909076, 67.44007279406643818 ) ) ;
#2497=EDGE_LOOP ( 'NONE', ( #26654, #9011, #31857, #48087, #29228 ) ) ;
#2498=CARTESIAN_POINT ( 'NONE',  ( -24.34138212120913991, -16.17068457824029792, 62.74328676669021831 ) ) ;
#2500=DIRECTION ( 'NONE',  ( -0.6264825908887947659, 0.7794354131762692983, -3.858680030446929083E-08 ) ) ;
#2501=CARTESIAN_POINT ( 'NONE',  ( -13.49409790474204840, -20.66256726344224504, 61.53118467422925164 ) ) ;
#2503=FACE_OUTER_BOUND ( 'NONE', #26474, .T. ) ;
#2506=CARTESIAN_POINT ( 'NONE',  ( -10.68551981713787136, -12.73596763222149519, 64.28308208171728211 ) ) ;
#2507=CARTESIAN_POINT ( 'NONE',  ( -17.42409385541300892, -14.80920654474439502, 77.49999999999994316 ) ) ;
#2508=EDGE_CURVE ( 'NONE', #47594, #260, #21486, .T. ) ;
#2510=CARTESIAN_POINT ( 'NONE',  ( -13.69528297853595511, -8.884503987240256251, 57.25351257252668091 ) ) ;
#2512=CARTESIAN_POINT ( 'NONE',  ( -10.40404453354760683, -17.30384760780096087, 61.27930367573277692 ) ) ;
#2514=DIRECTION ( 'NONE',  ( 0.7621627669932625748, -0.6473854467078884456, 3.680865982637999047E-08 ) ) ;
#2515=CARTESIAN_POINT ( 'NONE',  ( -12.14849447404118088, -10.12808629081546563, 67.91385578414299573 ) ) ;
#2516=CARTESIAN_POINT ( 'NONE',  ( -22.93575444817954079, -9.796624443348585842, 70.18895421311056282 ) ) ;
#2517=CARTESIAN_POINT ( 'NONE',  ( -13.72009916595086132, -20.81131062084115513, 61.40157432139535842 ) ) ;
#2518=DIRECTION ( 'NONE',  ( -0.5351595679979644915, -0.8447509909909737269, 1.882431089060611027E-16 ) ) ;
#2522=CARTESIAN_POINT ( 'NONE',  ( -22.73241942378198388, -10.24594066210862486, 66.54182232569581856 ) ) ;
#2523=CYLINDRICAL_SURFACE ( 'NONE', #18704, 0.1500000000000014655 ) ;
#2524=ORIENTED_EDGE ( 'NONE', *, *, #9769, .F. ) ;
#2525=CARTESIAN_POINT ( 'NONE',  ( -11.60526899143904345, -18.79015832504765271, 68.23161775275829655 ) ) ;
#2526=CARTESIAN_POINT ( 'NONE',  ( -10.11857101092534528, -16.26968670661729632, 71.70396332877544410 ) ) ;
#2529=CARTESIAN_POINT ( 'NONE',  ( -11.42622260759249286, -18.51434353338492400, 61.57710833179551457 ) ) ;
#2530=DIRECTION ( 'NONE',  ( 0.07061531369766044230, 0.9975036227860933913, 1.268851335910971019E-08 ) ) ;
#2531=ORIENTED_EDGE ( 'NONE', *, *, #20559, .F. ) ;
#2532=ADVANCED_FACE ( 'NONE', ( #39948 ), #43164, .T. ) ;
#2533=FACE_BOUND ( 'NONE', #17002, .T. ) ;
#2534=CARTESIAN_POINT ( 'NONE',  ( -13.43921408130402817, -8.993432070331126127, 60.73950277491898220 ) ) ;
#2536=DIRECTION ( 'NONE',  ( 0.7248509490090242480, -0.6889057277456162032, 1.880377065355303572E-09 ) ) ;
#2537=CARTESIAN_POINT ( 'NONE',  ( -23.72463700453396385, -17.86031891732679355, 59.01995031396651825 ) ) ;
#2538=ADVANCED_FACE ( 'NONE', ( #9194 ), #2523, .T. ) ;
#2540=ADVANCED_FACE ( 'NONE', ( #47585 ), #4550, .T. ) ;
#2542=PLANE ( 'NONE',  #3893 ) ;
#2543=CARTESIAN_POINT ( 'NONE',  ( -11.49052871324551717, -18.52330408776863280, 61.27710786653850761 ) ) ;
#2544=VECTOR ( 'NONE', #20952, 1000.000000000000227 ) ;
#2545=CARTESIAN_POINT ( 'NONE',  ( -23.00441852451001523, -19.11762575345012749, 58.88410642058937583 ) ) ;
#2546=CARTESIAN_POINT ( 'NONE',  ( -20.81300959806216966, -21.44393162792159657, 58.82287916276853679 ) ) ;
#2547=( BOUNDED_CURVE ( )  B_SPLINE_CURVE ( 3, ( #47206, #6806, #6323, #32191 ),
 .UNSPECIFIED., .F., .F. ) 
 B_SPLINE_CURVE_WITH_KNOTS ( ( 4, 4 ),
 ( 1.570796326794896780, 1.780235837034217727 ),
 .UNSPECIFIED. ) 
 CURVE ( )  GEOMETRIC_REPRESENTATION_ITEM ( )  RATIONAL_B_SPLINE_CURVE ( ( 1.000000000000000000, 0.9963479302455154896, 0.9963479302455154896, 1.000000000000000000 ) ) 
 REPRESENTATION_ITEM ( '' )  );
#2548=CARTESIAN_POINT ( 'NONE',  ( -10.73412800634210029, -11.53077167852495677, 71.20365559628196195 ) ) ;
#2549=CARTESIAN_POINT ( 'NONE',  ( -12.23220206747518013, -19.57856285391799034, 58.22682373937799838 ) ) ;
#2551=ORIENTED_EDGE ( 'NONE', *, *, #34875, .T. ) ;
#2554=CARTESIAN_POINT ( 'NONE',  ( -24.03565964049345283, -17.10859733140495464, 69.60443069367661906 ) ) ;
#2555=( BOUNDED_CURVE ( )  B_SPLINE_CURVE ( 3, ( #40590, #29775, #28796, #36408 ),
 .UNSPECIFIED., .F., .F. ) 
 B_SPLINE_CURVE_WITH_KNOTS ( ( 4, 4 ),
 ( 0.4074455897393630122, 0.5000000000000000000 ),
 .UNSPECIFIED. ) 
 CURVE ( )  GEOMETRIC_REPRESENTATION_ITEM ( )  RATIONAL_B_SPLINE_CURVE ( ( 0.6983129098260923984, 0.7760317562606954267, 0.8765941196519972944, 0.9999999999999964473 ) ) 
 REPRESENTATION_ITEM ( '' )  );
#2556=CARTESIAN_POINT ( 'NONE',  ( -15.35027035934970918, -7.653577032698213323, 74.26481056556292515 ) ) ;
#2558=CARTESIAN_POINT ( 'NONE',  ( -10.37541943412130863, -14.96049300415475436, 75.08306784598362071 ) ) ;
#2559=ORIENTED_EDGE ( 'NONE', *, *, #13, .F. ) ;
#2560=CARTESIAN_POINT ( 'NONE',  ( -19.33163353770262205, -22.01086598974156772, 58.72518590534810556 ) ) ;
#2562=ORIENTED_EDGE ( 'NONE', *, *, #47541, .F. ) ;
#2565=( BOUNDED_CURVE ( )  B_SPLINE_CURVE ( 3, ( #31181, #42758, #35102, #16866 ),
 .UNSPECIFIED., .F., .F. ) 
 B_SPLINE_CURVE_WITH_KNOTS ( ( 4, 4 ),
 ( 0.5000000000000000000, 0.9074455897393640669 ),
 .UNSPECIFIED. ) 
 CURVE ( )  GEOMETRIC_REPRESENTATION_ITEM ( )  RATIONAL_B_SPLINE_CURVE ( ( 1.000000000000005995, 0.4567392136813334114, 0.3561768502900266586, 0.6983129098260919543 ) ) 
 REPRESENTATION_ITEM ( '' )  );
#2566=ORIENTED_EDGE ( 'NONE', *, *, #39163, .T. ) ;
#2569=ORIENTED_EDGE ( 'NONE', *, *, #8542, .F. ) ;
#2570=CARTESIAN_POINT ( 'NONE',  ( -18.59601872632196518, -7.856991649524070809, 73.85536540707786912 ) ) ;
#2571=CARTESIAN_POINT ( 'NONE',  ( -24.10335570753463230, -17.07466383872621307, 69.29851186845237976 ) ) ;
#2572=CARTESIAN_POINT ( 'NONE',  ( -16.59344411340201475, -21.75974756046277747, 65.22564390621562325 ) ) ;
#2573=CARTESIAN_POINT ( 'NONE',  ( -22.53398831605844421, -19.59353892774318595, 72.92935240240784367 ) ) ;
#2574=VERTEX_POINT ( 'NONE', #37695 ) ;
#2575=CARTESIAN_POINT ( 'NONE',  ( -15.32518304399999387, -21.95751765168108349, 72.16080051677664642 ) ) ;
#2576=CARTESIAN_POINT ( 'NONE',  ( -24.06765785688162751, -12.42634649716644013, 69.92810001462744651 ) ) ;
#2577=CARTESIAN_POINT ( 'NONE',  ( -12.00910550946480093, -19.92697606054074910, 58.04027092519303466 ) ) ;
#2580=CARTESIAN_POINT ( 'NONE',  ( -16.78341102624552050, -22.23169286577646986, 68.88055947109249644 ) ) ;
#2581=CARTESIAN_POINT ( 'NONE',  ( -23.54659830298692569, -19.05403935986104003, 66.08035378328281695 ) ) ;
#2583=CARTESIAN_POINT ( 'NONE',  ( -23.58068229492725720, -11.36663999465536179, 73.66193538997137580 ) ) ;
#2585=CARTESIAN_POINT ( 'NONE',  ( -10.00543091975737831, -15.49190080042082940, 57.76781588145245649 ) ) ;
#2586=VERTEX_POINT ( 'NONE', #18000 ) ;
#2587=CARTESIAN_POINT ( 'NONE',  ( -19.78614083979442029, -21.39864764726399216, 69.23482476778590922 ) ) ;
#2588=B_SPLINE_CURVE_WITH_KNOTS ( 'NONE', 3,
 ( #3821, #34572, #15856, #12176, #33841, #42218, #1092, #8482, #4795, #34818 ),
 .UNSPECIFIED., .F., .F.,
 ( 4, 2, 2, 2, 4 ),
 ( 0.000000000000000000, 0.2500000000000000000, 0.5000000000000000000, 0.7500000000000000000, 1.000000000000000000 ),
 .UNSPECIFIED. ) ;
#2589=ORIENTED_EDGE ( 'NONE', *, *, #27980, .T. ) ;
#2590=EDGE_CURVE ( 'NONE', #42959, #3873, #28148, .T. ) ;
#2595=CARTESIAN_POINT ( 'NONE',  ( -21.34581862946232889, -20.66775363590295100, 72.52446429492309221 ) ) ;
#2596=DIRECTION ( 'NONE',  ( -3.298726454030011118E-06, 1.683524824177191357E-06, 0.9999999999931419303 ) ) ;
#2598=ORIENTED_EDGE ( 'NONE', *, *, #24802, .F. ) ;
#2601=EDGE_CURVE ( 'NONE', #5056, #18999, #47288, .T. ) ;
#2603=CARTESIAN_POINT ( 'NONE',  ( -14.81535805098777736, -7.777528402031247623, 53.89198173725363716 ) ) ;
#2604=CARTESIAN_POINT ( 'NONE',  ( -10.82849721076305194, -17.15437656679925738, 61.45743105333846756 ) ) ;
#2606=ORIENTED_EDGE ( 'NONE', *, *, #47427, .F. ) ;
#2607=EDGE_CURVE ( 'NONE', #17100, #6762, #1382, .T. ) ;
#2608=DIRECTION ( 'NONE',  ( -3.549360974554993999E-17, 6.371834667797928663E-18, 1.000000000000000000 ) ) ;
#2612=VERTEX_POINT ( 'NONE', #3242 ) ;
#2615=CARTESIAN_POINT ( 'NONE',  ( -19.03885666732217885, -7.536228653801991584, 67.15717731432056326 ) ) ;
#2617=VERTEX_POINT ( 'NONE', #29348 ) ;
#2618=CARTESIAN_POINT ( 'NONE',  ( -18.97948276208418150, -7.924750873940990203, 60.11659987143988815 ) ) ;
#2619=CARTESIAN_POINT ( 'NONE',  ( -11.36942910905634108, -11.19057675027386800, 64.24062247360485856 ) ) ;
#2620=CYLINDRICAL_SURFACE ( 'NONE', #45748, 0.1500000000000020206 ) ;
#2621=ORIENTED_EDGE ( 'NONE', *, *, #27337, .F. ) ;
#2622=CARTESIAN_POINT ( 'NONE',  ( -20.71200339104809274, -20.98905351909935035, 58.93009817979976361 ) ) ;
#2623=CARTESIAN_POINT ( 'NONE',  ( -24.84793648988037518, -14.18443574041886457, 69.83770584630335065 ) ) ;
#2624=ORIENTED_EDGE ( 'NONE', *, *, #12755, .F. ) ;
#2625=CARTESIAN_POINT ( 'NONE',  ( -10.64512080333459387, -11.71903002653516168, 74.81486074884371362 ) ) ;
#2628=CARTESIAN_POINT ( 'NONE',  ( -13.71293330176565384, -21.26916511146244915, 68.64120417180296840 ) ) ;
#2630=CARTESIAN_POINT ( 'NONE',  ( -22.73035995389123798, -10.24127042357611650, 70.20105554212841525 ) ) ;
#2632=CARTESIAN_POINT ( 'NONE',  ( -21.95939004544374740, -9.477125498926222136, 59.72171213236985921 ) ) ;
#2633=CARTESIAN_POINT ( 'NONE',  ( -18.97054302448013985, -7.521389842619064403, 67.08567168106696954 ) ) ;
#2634=CARTESIAN_POINT ( 'NONE',  ( -21.54712039243748833, -8.603915288790302540, 73.73982196406554124 ) ) ;
#2635=B_SPLINE_CURVE_WITH_KNOTS ( 'NONE', 3,
 ( #33569, #47894, #40492, #37772, #25720, #40735, #11430, #128, #37028, #48615 ),
 .UNSPECIFIED., .F., .F.,
 ( 4, 2, 2, 2, 4 ),
 ( 0.000000000000000000, 0.2500000000000000000, 0.5000000000000000000, 0.7500000000000000000, 1.000000000000000000 ),
 .UNSPECIFIED. ) ;
#2636=VERTEX_POINT ( 'NONE', #48 ) ;
#2637=CARTESIAN_POINT ( 'NONE',  ( -9.976559278833523337, -14.59036342035520306, 67.97144843379662404 ) ) ;
#2639=B_SPLINE_CURVE_WITH_KNOTS ( 'NONE', 3,
 ( #44834, #11087, #22659, #18700, #26109, #37657, #3949, #18961, #1451, #24115 ),
 .UNSPECIFIED., .F., .F.,
 ( 4, 2, 2, 2, 4 ),
 ( 0.1272669073657988204, 0.2522669073462828204, 0.3772669073267668205, 0.5022669073072507651, 0.6272669072877348206 ),
 .UNSPECIFIED. ) ;
#2641=VERTEX_POINT ( 'NONE', #25896 ) ;
#2642=ORIENTED_EDGE ( 'NONE', *, *, #41119, .F. ) ;
#2643=CARTESIAN_POINT ( 'NONE',  ( -18.35035633668588773, -22.20141378626043860, 68.91540458395735413 ) ) ;
#2644=FACE_OUTER_BOUND ( 'NONE', #29928, .T. ) ;
#2646=CARTESIAN_POINT ( 'NONE',  ( -10.45378225047720200, -13.70027870591744446, 74.83384660681542755 ) ) ;
#2647=CARTESIAN_POINT ( 'NONE',  ( -19.45739170982025357, -7.641871707264925817, 60.12239523375242101 ) ) ;
#2648=CARTESIAN_POINT ( 'NONE',  ( -12.40380833417894912, -19.68739609921301792, 61.39678633575574906 ) ) ;
#2649=CARTESIAN_POINT ( 'NONE',  ( -12.60227155074094441, -19.95281705956671559, 68.35129494334645983 ) ) ;
#2650=CARTESIAN_POINT ( 'NONE',  ( -20.63628304827270199, -8.086446354347476273, 66.96759359044023086 ) ) ;
#2651=ORIENTED_EDGE ( 'NONE', *, *, #6993, .F. ) ;
#2652=ORIENTED_EDGE ( 'NONE', *, *, #4389, .F. ) ;
#2653=EDGE_CURVE ( 'NONE', #7442, #5861, #37310, .T. ) ;
#2654=CARTESIAN_POINT ( 'NONE',  ( -13.25048244539004827, -9.122748337194952484, 60.43949979652826698 ) ) ;
#2656=EDGE_CURVE ( 'NONE', #32569, #18851, #21802, .T. ) ;
#2657=FACE_OUTER_BOUND ( 'NONE', #4683, .T. ) ;
#2658=CARTESIAN_POINT ( 'NONE',  ( -10.57990114081760957, -13.11695186304740979, 71.22300718686658172 ) ) ;
#2659=CARTESIAN_POINT ( 'NONE',  ( -18.97893323490226791, -7.523212336634692576, 67.00733453731432121 ) ) ;
#2660=CYLINDRICAL_SURFACE ( 'NONE', #30778, 0.1500000000000035194 ) ;
#2663=VERTEX_POINT ( 'NONE', #14053 ) ;
#2665=CARTESIAN_POINT ( 'NONE',  ( -10.22367903246940557, -12.89696208012659717, 67.83808713863969331 ) ) ;
#2667=FACE_OUTER_BOUND ( 'NONE', #21033, .T. ) ;
#2669=CARTESIAN_POINT ( 'NONE',  ( -10.57458986182457750, -16.25351003539013561, 71.74750329799698534 ) ) ;
#2670=CARTESIAN_POINT ( 'NONE',  ( -17.91716493482169525, -7.374790294242734134, 60.26716059546817661 ) ) ;
#2672=( BOUNDED_CURVE ( )  B_SPLINE_CURVE ( 3, ( #18114, #32892, #15152, #7554 ),
 .UNSPECIFIED., .F., .F. ) 
 B_SPLINE_CURVE_WITH_KNOTS ( ( 4, 4 ),
 ( 0.9074455897393624015, 1.000000000000000000 ),
 .UNSPECIFIED. ) 
 CURVE ( )  GEOMETRIC_REPRESENTATION_ITEM ( )  RATIONAL_B_SPLINE_CURVE ( ( 0.6983129098260865142, 0.7760317562606925401, 0.8765941196519970724, 1.000000000000000000 ) ) 
 REPRESENTATION_ITEM ( '' )  );
#2673=ORIENTED_EDGE ( 'NONE', *, *, #27858, .F. ) ;
#2674=CARTESIAN_POINT ( 'NONE',  ( -20.98580030992770418, -20.83533690608478040, 65.88453944791919525 ) ) ;
#2675=ORIENTED_EDGE ( 'NONE', *, *, #43911, .T. ) ;
#2676=VECTOR ( 'NONE', #40730, 1000.000000000000000 ) ;
#2678=CARTESIAN_POINT ( 'NONE',  ( -10.00972249263052838, -14.08138219831849014, 61.11810067724670148 ) ) ;
#2679=ORIENTED_EDGE ( 'NONE', *, *, #33077, .T. ) ;
#2684=CARTESIAN_POINT ( 'NONE',  ( -18.84909840123831160, -7.954480093619391567, 70.59898004676588812 ) ) ;
#2685=EDGE_CURVE ( 'NONE', #32730, #38697, #8034, .T. ) ;
#2687=CARTESIAN_POINT ( 'NONE',  ( -20.95545100651803594, -20.91135505560678354, 65.59926067308570907 ) ) ;
#2689=CARTESIAN_POINT ( 'NONE',  ( -19.94877900550811844, -21.81838596911105554, 69.13471258482660176 ) ) ;
#2690=( BOUNDED_CURVE ( )  B_SPLINE_CURVE ( 3, ( #21308, #28682, #2583, #17586 ),
 .UNSPECIFIED., .F., .F. ) 
 B_SPLINE_CURVE_WITH_KNOTS ( ( 4, 4 ),
 ( 0.5000000000000000000, 0.9074455897393649551 ),
 .UNSPECIFIED. ) 
 CURVE ( )  GEOMETRIC_REPRESENTATION_ITEM ( )  RATIONAL_B_SPLINE_CURVE ( ( 1.000000000000019540, 0.4567392136813264170, 0.3561768502900144462, 0.6983129098261048329 ) ) 
 REPRESENTATION_ITEM ( '' )  );
#2691=CARTESIAN_POINT ( 'NONE',  ( -10.95687064503993824, -18.50777464695341479, 57.92997716917032136 ) ) ;
#2692=CARTESIAN_POINT ( 'NONE',  ( -23.29452124531334434, -19.39641313704064629, 59.00693762799269848 ) ) ;
#2693=CYLINDRICAL_SURFACE ( 'NONE', #31866, 0.1500000000000002720 ) ;
#2694=ORIENTED_EDGE ( 'NONE', *, *, #16466, .T. ) ;
#2695=VERTEX_POINT ( 'NONE', #25415 ) ;
#2696=CARTESIAN_POINT ( 'NONE',  ( -22.54039128431939787, -19.66481624898402458, 69.38238023638768937 ) ) ;
#2697=CARTESIAN_POINT ( 'NONE',  ( -24.69852180232685157, -16.41745880042978101, 59.30827708941524889 ) ) ;
#2698=EDGE_LOOP ( 'NONE', ( #2462, #46521, #11217, #2598, #14273 ) ) ;
#2699=CARTESIAN_POINT ( 'NONE',  ( -23.80321479583337307, -17.81075880182941873, 59.30378417737343710 ) ) ;
#2701=CARTESIAN_POINT ( 'NONE',  ( -15.55326400670571196, -7.597850160029695488, 70.65343888371961611 ) ) ;
#2702=ORIENTED_EDGE ( 'NONE', *, *, #30237, .T. ) ;
#2703=CARTESIAN_POINT ( 'NONE',  ( -10.54203096409779050, -13.52967128519119200, 74.86920801952661009 ) ) ;
#2704=B_SPLINE_CURVE_WITH_KNOTS ( 'NONE', 3,
 ( #26937, #41955, #41711, #23015, #8231, #16067, #1550, #4287, #23246, #38734 ),
 .UNSPECIFIED., .F., .F.,
 ( 4, 2, 2, 2, 4 ),
 ( 0.1272669073658395933, 0.2522669073439455234, 0.3772669073220514813, 0.5022669073001573281, 0.6272669072782632860 ),
 .UNSPECIFIED. ) ;
#2706=CARTESIAN_POINT ( 'NONE',  ( -18.92057809895272413, -7.919864474132485732, 66.90071783790344284 ) ) ;
#2707=CARTESIAN_POINT ( 'NONE',  ( -13.57571756020798581, -20.65642803140422856, 61.51646323935151628 ) ) ;
#2708=EDGE_CURVE ( 'NONE', #1365, #25, #30583, .T. ) ;
#2709=EDGE_LOOP ( 'NONE', ( #11574, #17305 ) ) ;
#2711=ADVANCED_FACE ( 'NONE', ( #7936 ), #8654, .T. ) ;
#2715=CARTESIAN_POINT ( 'NONE',  ( -10.00816431203761780, -14.09700820520310671, 61.02482976538944826 ) ) ;
#2717=EDGE_CURVE ( 'NONE', #5348, #47871, #23400, .T. ) ;
#2718=ORIENTED_EDGE ( 'NONE', *, *, #25374, .F. ) ;
#2719=CARTESIAN_POINT ( 'NONE',  ( -24.23275881451340297, -13.18375842335132830, 59.47153824729769411 ) ) ;
#2720=CYLINDRICAL_SURFACE ( 'NONE', #46137, 0.1500000000000029365 ) ;
#2723=CARTESIAN_POINT ( 'NONE',  ( -12.57255317706665387, -20.46319310760117816, 71.96687053577548454 ) ) ;
#2724=DIRECTION ( 'NONE',  ( 0.3374354101627465297, 0.9413486835218388693, 1.423378189492272923E-08 ) ) ;
#2728=DIRECTION ( 'NONE',  ( -0.2196488028684550620, -0.9755790093059855117, 7.835600157697873389E-08 ) ) ;
#2729=CARTESIAN_POINT ( 'NONE',  ( -22.74914502862361587, -19.44157078561079999, 72.79967855327656423 ) ) ;
#2730=CARTESIAN_POINT ( 'NONE',  ( -19.37066084507306130, -21.53310995536324413, 58.71610482352626548 ) ) ;
#2732=CARTESIAN_POINT ( 'NONE',  ( -21.43551424305475450, -21.08722505841212680, 69.21483509587649507 ) ) ;
#2733=CARTESIAN_POINT ( 'NONE',  ( -10.60833884242739522, -12.99528357717770355, 64.15347367985145866 ) ) ;
#2735=B_SPLINE_CURVE_WITH_KNOTS ( 'NONE', 1,
 ( #17329, #21763 ),
 .UNSPECIFIED., .F., .F.,
 ( 2, 2 ),
 ( 0.000000000000000000, 1.000000000000000000 ),
 .UNSPECIFIED. ) ;
#2740=ORIENTED_EDGE ( 'NONE', *, *, #6979, .F. ) ;
#2741=DIRECTION ( 'NONE',  ( -0.3478314405900309603, -0.9375570856950864451, 9.567072274253696421E-17 ) ) ;
#2745=CARTESIAN_POINT ( 'NONE',  ( -10.99586697244644640, -11.04334986774487781, 60.86381167495338929 ) ) ;
#2746=CARTESIAN_POINT ( 'NONE',  ( -24.76540221579651302, -16.07765826482591365, 66.17829537637275905 ) ) ;
#2750=CARTESIAN_POINT ( 'NONE',  ( -21.24554520941113367, -21.20453976546471608, 65.76949229983627276 ) ) ;
#2751=DIRECTION ( 'NONE',  ( -0.8356905716187448263, 0.5492005722024784209, 7.728900804118606451E-08 ) ) ;
#2753=CARTESIAN_POINT ( 'NONE',  ( -11.64235137327199610, -18.84330536064715034, 68.36689631560025759 ) ) ;
#2755=CARTESIAN_POINT ( 'NONE',  ( -11.32868513771122743, -18.25189784781867530, 58.09098068066235498 ) ) ;
#2756=CARTESIAN_POINT ( 'NONE',  ( -11.82099749022622426, -9.899105802180386604, 64.21409645106085406 ) ) ;
#2757=CARTESIAN_POINT ( 'NONE',  ( -24.74075724160099554, -16.21284971877490122, 62.77824058731629009 ) ) ;
#2759=FACE_BOUND ( 'NONE', #17471, .T. ) ;
#2760=EDGE_CURVE ( 'NONE', #23333, #37436, #4711, .T. ) ;
#2761=CARTESIAN_POINT ( 'NONE',  ( -23.89968659910968185, -17.46782286739716028, 65.94357233134253704 ) ) ;
#2762=CARTESIAN_POINT ( 'NONE',  ( -23.19916440516392697, -19.59445054535707698, 54.27966884056655061 ) ) ;
#2763=CYLINDRICAL_SURFACE ( 'NONE', #13360, 0.1500000000000011879 ) ;
#2764=VERTEX_POINT ( 'NONE', #34972 ) ;
#2765=FACE_OUTER_BOUND ( 'NONE', #22404, .T. ) ;
#2766=LINE ( 'NONE', #41410, #46308 ) ;
#2767=B_SPLINE_CURVE_WITH_KNOTS ( 'NONE', 3,
 ( #19081, #4318, #26472, #33102, #44969, #7037, #7778, #15128, #26229, #30428 ),
 .UNSPECIFIED., .F., .F.,
 ( 4, 2, 2, 2, 4 ),
 ( 0.000000000000000000, 0.2500000000000000000, 0.5000000000000000000, 0.7500000000000000000, 1.000000000000000000 ),
 .UNSPECIFIED. ) ;
#2770=CARTESIAN_POINT ( 'NONE',  ( -24.18648589646226910, -17.93571655855329894, 59.16411793359512217 ) ) ;
#2771=CARTESIAN_POINT ( 'NONE',  ( -24.03385203260749847, -12.34657780677343375, 73.45045475050159212 ) ) ;
#2772=CARTESIAN_POINT ( 'NONE',  ( -24.87123160714014958, -14.59964084223042491, 62.89791924484052998 ) ) ;
#2774=ORIENTED_EDGE ( 'NONE', *, *, #14832, .F. ) ;
#2776=EDGE_CURVE ( 'NONE', #26191, #18567, #4861, .T. ) ;
#2777=ORIENTED_EDGE ( 'NONE', *, *, #12545, .T. ) ;
#2778=CARTESIAN_POINT ( 'NONE',  ( -13.18646824325598566, -9.237624247784513187, 64.10049605889102509 ) ) ;
#2779=FACE_OUTER_BOUND ( 'NONE', #6573, .T. ) ;
#2780=ADVANCED_FACE ( 'NONE', ( #1015 ), #9606, .T. ) ;
#2781=B_SPLINE_CURVE_WITH_KNOTS ( 'NONE', 3,
 ( #29394, #11171, #14100, #36286, #3035, #10451, #48587, #28905, #36747, #29150 ),
 .UNSPECIFIED., .F., .F.,
 ( 4, 2, 2, 2, 4 ),
 ( 0.1272669073657631822, 0.2522669073462648903, 0.3772669073267665429, 0.5022669073072681956, 0.6272669072877699037 ),
 .UNSPECIFIED. ) ;
#2782=DIRECTION ( 'NONE',  ( -5.731567514496413899E-31, -1.020425574103664789E-16, -1.000000000000000000 ) ) ;
#2783=LINE ( 'NONE', #7477, #19926 ) ;
#2787=VERTEX_POINT ( 'NONE', #27108 ) ;
#2788=LINE ( 'NONE', #32118, #47745 ) ;
#2789=EDGE_CURVE ( 'NONE', #46311, #784, #47891, .T. ) ;
#2790=CARTESIAN_POINT ( 'NONE',  ( -13.18904211892903078, -11.30002761096173813, 53.49999999999995026 ) ) ;
#2791=EDGE_CURVE ( 'NONE', #29130, #43276, #45840, .T. ) ;
#2792=ORIENTED_EDGE ( 'NONE', *, *, #42325, .F. ) ;
#2795=CARTESIAN_POINT ( 'NONE',  ( -9.979271025556270658, -14.52814615614862070, 68.03517031705335683 ) ) ;
#2796=EDGE_CURVE ( 'NONE', #31355, #46961, #19730, .T. ) ;
#2797=ORIENTED_EDGE ( 'NONE', *, *, #11598, .T. ) ;
#2798=ADVANCED_FACE ( 'NONE', ( #47291 ), #16736, .T. ) ;
#2800=CARTESIAN_POINT ( 'NONE',  ( -23.38668381416880138, -18.47650297087272975, 73.06368285098588444 ) ) ;
#2802=CARTESIAN_POINT ( 'NONE',  ( -23.94296205860991122, -17.35973477539799603, 65.95859725740298529 ) ) ;
#2803=ORIENTED_EDGE ( 'NONE', *, *, #48449, .F. ) ;
#2805=FACE_OUTER_BOUND ( 'NONE', #13035, .T. ) ;
#2806=CARTESIAN_POINT ( 'NONE',  ( -15.51710240044429590, -8.021979398744527145, 74.07985680213998592 ) ) ;
#2807=CARTESIAN_POINT ( 'NONE',  ( -14.42683416945219221, -8.428067588089273698, 67.40975083869261653 ) ) ;
#2811=CARTESIAN_POINT ( 'NONE',  ( -24.31823732957325745, -17.63313362019280106, 66.05861802595141796 ) ) ;
#2812=CARTESIAN_POINT ( 'NONE',  ( -13.22252872046149541, -18.37919617513480475, 53.88362224778187226 ) ) ;
#2814=( BOUNDED_SURFACE ( )  B_SPLINE_SURFACE ( 3, 1, ( 
 ( #3506, #34515 ),
 ( #15547, #41918 ),
 ( #12119, #26176 ),
 ( #18518, #34029 ),
 ( #798, #27135 ),
 ( #15795, #22979 ),
 ( #8198, #42162 ) ),
 .UNSPECIFIED., .T., .F., .F. ) 
 B_SPLINE_SURFACE_WITH_KNOTS ( ( 4, 3, 4 ),
 ( 2, 2 ),
 ( 0.000000000000000000, 0.5000000000000000000, 1.000000000000000000 ),
 ( 0.000000000000000000, 1.000000000000000000 ),
 .UNSPECIFIED. ) 
 GEOMETRIC_REPRESENTATION_ITEM ( )  RATIONAL_B_SPLINE_SURFACE ( (
 ( 1.000000000000000000, 1.000000000000000000),
 ( 0.3333333333333335369, 0.3333333333333330373),
 ( 0.3333333333333335369, 0.3333333333333330373),
 ( 1.000000000000000000, 1.000000000000000000),
 ( 0.3333333333333333703, 0.3333333333333333703),
 ( 0.3333333333333333703, 0.3333333333333333703),
 ( 1.000000000000000000, 1.000000000000000000) ) ) 
 REPRESENTATION_ITEM ( '' )  SURFACE ( )  );
#2815=ORIENTED_EDGE ( 'NONE', *, *, #13611, .T. ) ;
#2816=CARTESIAN_POINT ( 'NONE',  ( -10.04615901573667003, -15.84412989934948257, 64.66918126557563085 ) ) ;
#2817=AXIS2_PLACEMENT_3D ( 'NONE', #28652, #42942, #35546 ) ;
#2818=EDGE_LOOP ( 'NONE', ( #13739, #45229, #28599, #41545, #46357 ) ) ;
#2819=ORIENTED_EDGE ( 'NONE', *, *, #8829, .T. ) ;
#2820=ORIENTED_EDGE ( 'NONE', *, *, #43969, .T. ) ;
#2821=CYLINDRICAL_SURFACE ( 'NONE', #6860, 6.899999999999999467 ) ;
#2822=DIRECTION ( 'NONE',  ( 1.235321093103353499E-06, 4.801898924785047334E-07, 0.9999999999991215915 ) ) ;
#2824=CARTESIAN_POINT ( 'NONE',  ( -22.65132463393941364, -10.07854832284319890, 70.31178513642615258 ) ) ;
#2825=( BOUNDED_CURVE ( )  B_SPLINE_CURVE ( 3, ( #23416, #15507, #41387, #34232 ),
 .UNSPECIFIED., .F., .F. ) 
 B_SPLINE_CURVE_WITH_KNOTS ( ( 4, 4 ),
 ( 0.4074455897393645110, 0.5000000000000000000 ),
 .UNSPECIFIED. ) 
 CURVE ( )  GEOMETRIC_REPRESENTATION_ITEM ( )  RATIONAL_B_SPLINE_CURVE ( ( 0.6983129098261006140, 0.7760317562606882102, 0.8765941196519829726, 0.9999999999999736877 ) ) 
 REPRESENTATION_ITEM ( '' )  );
#2827=VERTEX_POINT ( 'NONE', #5917 ) ;
#2829=EDGE_CURVE ( 'NONE', #7981, #22280, #35037, .T. ) ;
#2831=LINE ( 'NONE', #7283, #21418 ) ;
#2833=( BOUNDED_SURFACE ( )  B_SPLINE_SURFACE ( 3, 1, ( 
 ( #4361, #8306 ),
 ( #41799, #19136 ),
 ( #30722, #45749 ),
 ( #12232, #30483 ),
 ( #27252, #11999 ),
 ( #42035, #38314 ),
 ( #45021, #41296 ) ),
 .UNSPECIFIED., .T., .F., .F. ) 
 B_SPLINE_SURFACE_WITH_KNOTS ( ( 4, 3, 4 ),
 ( 2, 2 ),
 ( 0.000000000000000000, 0.5000000000000000000, 1.000000000000000000 ),
 ( 0.000000000000000000, 1.000000000000000000 ),
 .UNSPECIFIED. ) 
 GEOMETRIC_REPRESENTATION_ITEM ( )  RATIONAL_B_SPLINE_SURFACE ( (
 ( 1.000000000000000000, 1.000000000000000000),
 ( 0.3333333333333335369, 0.3333333333333330373),
 ( 0.3333333333333335369, 0.3333333333333330373),
 ( 1.000000000000000000, 1.000000000000000000),
 ( 0.3333333333333333703, 0.3333333333333333703),
 ( 0.3333333333333333703, 0.3333333333333333703),
 ( 1.000000000000000000, 1.000000000000000000) ) ) 
 REPRESENTATION_ITEM ( '' )  SURFACE ( )  );
#2834=ORIENTED_EDGE ( 'NONE', *, *, #16274, .F. ) ;
#2835=CYLINDRICAL_SURFACE ( 'NONE', #36295, 5.500000000000000000 ) ;
#2837=ORIENTED_EDGE ( 'NONE', *, *, #17489, .F. ) ;
#2838=DIRECTION ( 'NONE',  ( -8.993561335472250294E-07, 8.977735684497376994E-07, 0.9999999999991925348 ) ) ;
#2842=VERTEX_POINT ( 'NONE', #13278 ) ;
#2844=CARTESIAN_POINT ( 'NONE',  ( -19.60046790782316251, -21.46228069541063732, 65.46486213989528835 ) ) ;
#2845=EDGE_CURVE ( 'NONE', #20172, #38891, #14574, .T. ) ;
#2846=EDGE_CURVE ( 'NONE', #14728, #2636, #43547, .T. ) ;
#2847=CARTESIAN_POINT ( 'NONE',  ( -10.40127070788197017, -12.32249518151173895, 57.51352764219546998 ) ) ;
#2848=VERTEX_POINT ( 'NONE', #17224 ) ;
#2849=CARTESIAN_POINT ( 'NONE',  ( -12.81450527785482230, -9.474959380418823685, 74.61923006088066757 ) ) ;
#2850=CARTESIAN_POINT ( 'NONE',  ( -22.83585279654753109, -10.36919270525743464, 63.35720607436116580 ) ) ;
#2851=LINE ( 'NONE', #47925, #29984 ) ;
#2852=ORIENTED_EDGE ( 'NONE', *, *, #16604, .F. ) ;
#2853=CARTESIAN_POINT ( 'NONE',  ( -23.61204160381034711, -11.53669949605622769, 66.42214514747726639 ) ) ;
#2854=DIRECTION ( 'NONE',  ( -0.6973657521612035559, 0.7167154300785205656, -1.015100525525034718E-08 ) ) ;
#2856=ORIENTED_EDGE ( 'NONE', *, *, #466, .T. ) ;
#2857=DIRECTION ( 'NONE',  ( -0.5497669574358331479, 0.8353180786453390239, 7.898837271846010071E-08 ) ) ;
#2858=EDGE_CURVE ( 'NONE', #12172, #21456, #30294, .T. ) ;
#2860=CARTESIAN_POINT ( 'NONE',  ( -11.00561500425097528, -11.89266776388777380, 74.55840173649494318 ) ) ;
#2861=CARTESIAN_POINT ( 'NONE',  ( -20.19231683483797468, -8.325423577284542631, 70.55100341277885434 ) ) ;
#2863=CARTESIAN_POINT ( 'NONE',  ( -24.31482381427648676, -13.31912605980313558, 59.36267924676594276 ) ) ;
#2864=ORIENTED_EDGE ( 'NONE', *, *, #37278, .T. ) ;
#2866=CARTESIAN_POINT ( 'NONE',  ( -14.72778340125292651, -21.32322296975913645, 58.46617885012763338 ) ) ;
#2867=DIRECTION ( 'NONE',  ( -0.8447509909909772796, 0.5351595679979588294, -3.339321029457348113E-17 ) ) ;
#2868=ORIENTED_EDGE ( 'NONE', *, *, #10235, .F. ) ;
#2869=CARTESIAN_POINT ( 'NONE',  ( -9.985760891864103428, -14.37924521898145258, 68.04455407903930109 ) ) ;
#2870=B_SPLINE_CURVE_WITH_KNOTS ( 'NONE', 3,
 ( #20789, #35794, #2070, #5289, #12669, #35066, #27694, #2313, #31637, #24253 ),
 .UNSPECIFIED., .F., .F.,
 ( 4, 2, 2, 2, 4 ),
 ( 0.000000000000000000, 0.2500000000000000000, 0.5000000000000000000, 0.7500000000000000000, 1.000000000000000000 ),
 .UNSPECIFIED. ) ;
#2871=CARTESIAN_POINT ( 'NONE',  ( -24.65023673758593148, -12.99629830290576038, 63.01759453279318279 ) ) ;
#2872=EDGE_CURVE ( 'NONE', #18814, #29649, #26858, .T. ) ;
#2873=VERTEX_POINT ( 'NONE', #32018 ) ;
#2874=ORIENTED_EDGE ( 'NONE', *, *, #17770, .F. ) ;
#2875=DIRECTION ( 'NONE',  ( 2.201155577252676169E-06, 7.355553122608190330E-06, 0.9999999999705252440 ) ) ;
#2876=CARTESIAN_POINT ( 'NONE',  ( -16.00544582274271477, -7.903112417841744453, 63.95538887075813506 ) ) ;
#2877=CARTESIAN_POINT ( 'NONE',  ( -23.82048026265336560, -11.84452950502918256, 59.78235734495926579 ) ) ;
#2878=CARTESIAN_POINT ( 'NONE',  ( -10.40277084706750621, -15.44444119821074679, 57.86792809062918508 ) ) ;
#2881=CARTESIAN_POINT ( 'NONE',  ( -14.80056147340629380, -21.78207226143426922, 61.82095877133116346 ) ) ;
#2882=VECTOR ( 'NONE', #26574, 1000.000000000000000 ) ;
#2884=EDGE_LOOP ( 'NONE', ( #1523, #40900, #27884, #43501, #37097, #9722, #42896, #35000, #19040, #35792, #47064, #39509, #13409, #25009, #19684, #35865, #7342, #1386, #11327, #8219, #32206, #23486, #2559, #24103, #30649, #7267, #45817, #22573, #43360, #8362, #48431, #22142, #2392, #41518 ) ) ;
#2885=ORIENTED_EDGE ( 'NONE', *, *, #22335, .T. ) ;
#2886=CARTESIAN_POINT ( 'NONE',  ( -19.11145865927416310, -7.964113456900453691, 63.43089235103782642 ) ) ;
#2887=CARTESIAN_POINT ( 'NONE',  ( -21.55204993259905066, -9.089641334111684401, 73.69309041467538179 ) ) ;
#2888=DIRECTION ( 'NONE',  ( 0.8459089628457130416, 0.5333273165489315071, -7.771812505054809235E-08 ) ) ;
#2889=CARTESIAN_POINT ( 'NONE',  ( -18.96371539328398725, -7.519906776682348415, 67.02258991573486924 ) ) ;
#2890=VECTOR ( 'NONE', #15166, 1000.000000000000000 ) ;
#2891=CARTESIAN_POINT ( 'NONE',  ( -10.00368807899092971, -15.89896712085359098, 53.49999999999994316 ) ) ;
#2894=ORIENTED_EDGE ( 'NONE', *, *, #29597, .F. ) ;
#2895=CARTESIAN_POINT ( 'NONE',  ( -22.05923648098858791, -20.05472392750071720, 62.23439162613904330 ) ) ;
#2897=CARTESIAN_POINT ( 'NONE',  ( -10.03035355355731006, -15.72374577095404824, 61.22284339518546403 ) ) ;
#2898=ORIENTED_EDGE ( 'NONE', *, *, #33030, .F. ) ;
#2899=CARTESIAN_POINT ( 'NONE',  ( -22.21990939174572333, -19.97672261113873660, 65.70421733412537435 ) ) ;
#2900=CARTESIAN_POINT ( 'NONE',  ( -17.70613249112851761, -7.363797380145674865, 60.19405475747598899 ) ) ;
#2901=EDGE_CURVE ( 'NONE', #30726, #42456, #39690, .T. ) ;
#2902=CARTESIAN_POINT ( 'NONE',  ( -21.56832988282965857, -21.00015211897737899, 72.67446426350551292 ) ) ;
#2903=CARTESIAN_POINT ( 'NONE',  ( -16.03618328653303848, -7.893388160315826241, 60.20028212586171890 ) ) ;
#2907=ORIENTED_EDGE ( 'NONE', *, *, #21080, .T. ) ;
#2908=CARTESIAN_POINT ( 'NONE',  ( -24.37288983953117594, -15.99971190300345292, 66.06324957111131368 ) ) ;
#2909=ADVANCED_FACE ( 'NONE', ( #1744 ), #13043, .T. ) ;
#2910=ADVANCED_FACE ( 'NONE', ( #9379 ), #30316, .T. ) ;
#2911=CARTESIAN_POINT ( 'NONE',  ( -11.25989503537269698, -11.38792718504117829, 64.29882039368452240 ) ) ;
#2913=CARTESIAN_POINT ( 'NONE',  ( -18.50162525266306091, -21.72577549820248421, 72.58510940979837756 ) ) ;
#2915=CARTESIAN_POINT ( 'NONE',  ( -12.84615363328625826, -20.17103110633857455, 72.09181604382622766 ) ) ;
#2919=ADVANCED_FACE ( 'NONE', ( #3670 ), #41960, .T. ) ;
#2921=CARTESIAN_POINT ( 'NONE',  ( -21.57897937893636353, -8.625392431642884716, 73.80117520113515184 ) ) ;
#2922=VERTEX_POINT ( 'NONE', #21658 ) ;
#2923=CARTESIAN_POINT ( 'NONE',  ( -19.90432934692537614, -21.83431937171774706, 69.04987052938618319 ) ) ;
#2924=B_SPLINE_CURVE_WITH_KNOTS ( 'NONE', 3,
 ( #47172, #10477, #28467, #6041, #44452, #3065, #21067, #10237, #48133, #47421 ),
 .UNSPECIFIED., .F., .F.,
 ( 4, 2, 2, 2, 4 ),
 ( 0.000000000000000000, 0.2500000000000000000, 0.5000000000000000000, 0.7500000000000000000, 1.000000000000000000 ),
 .UNSPECIFIED. ) ;
#2925=CARTESIAN_POINT ( 'NONE',  ( -24.04756562706866418, -17.22461864935846876, 69.70780031821135481 ) ) ;
#2926=DIRECTION ( 'NONE',  ( 0.3926557917762824590, -0.9196855055857630079, -5.808111619717073930E-09 ) ) ;
#2928=ORIENTED_EDGE ( 'NONE', *, *, #735, .T. ) ;
#2929=EDGE_LOOP ( 'NONE', ( #36857, #38318, #26533, #30939, #12333 ) ) ;
#2931=CARTESIAN_POINT ( 'NONE',  ( -11.84831518238830839, -10.57700509508930686, 71.04181123525845010 ) ) ;
#2932=CARTESIAN_POINT ( 'NONE',  ( -17.78823985852933731, -7.818684566706888717, 60.08060768393342954 ) ) ;
#2934=CARTESIAN_POINT ( 'NONE',  ( -22.88264614489240856, -10.34704276773305764, 63.35713876973677827 ) ) ;
#2935=CARTESIAN_POINT ( 'NONE',  ( -13.83108396514174565, -21.33561889020367630, 72.04112409899799729 ) ) ;
#2937=DIRECTION ( 'NONE',  ( 1.684279440454093594E-06, -5.535644408139047379E-06, 0.9999999999832598352 ) ) ;
#2938=ORIENTED_EDGE ( 'NONE', *, *, #34457, .T. ) ;
#2939=CARTESIAN_POINT ( 'NONE',  ( -10.54215788045047653, -13.52898884568911519, 74.78703633234691495 ) ) ;
#2940=CYLINDRICAL_SURFACE ( 'NONE', #40810, 0.1500000000000014932 ) ;
#2942=CARTESIAN_POINT ( 'NONE',  ( -12.35878062960998669, -9.253330100773967004, 53.76227901944321985 ) ) ;
#2943=( BOUNDED_SURFACE ( )  B_SPLINE_SURFACE ( 3, 1, ( 
 ( #44270, #47221 ),
 ( #13466, #36833 ),
 ( #5859, #3119 ),
 ( #21371, #2401 ),
 ( #21120, #2151 ),
 ( #25303, #36359 ),
 ( #6092, #20875 ) ),
 .UNSPECIFIED., .T., .F., .F. ) 
 B_SPLINE_SURFACE_WITH_KNOTS ( ( 4, 3, 4 ),
 ( 2, 2 ),
 ( 0.000000000000000000, 0.5000000000000000000, 1.000000000000000000 ),
 ( 0.000000000000000000, 1.000000000000000000 ),
 .UNSPECIFIED. ) 
 GEOMETRIC_REPRESENTATION_ITEM ( )  RATIONAL_B_SPLINE_SURFACE ( (
 ( 1.000000000000000000, 1.000000000000000000),
 ( 0.3333333333333335369, 0.3333333333333330373),
 ( 0.3333333333333335369, 0.3333333333333330373),
 ( 1.000000000000000000, 1.000000000000000000),
 ( 0.3333333333333333703, 0.3333333333333333703),
 ( 0.3333333333333333703, 0.3333333333333333703),
 ( 1.000000000000000000, 1.000000000000000000) ) ) 
 REPRESENTATION_ITEM ( '' )  SURFACE ( )  );
#2944=ORIENTED_EDGE ( 'NONE', *, *, #23691, .T. ) ;
#2946=ORIENTED_EDGE ( 'NONE', *, *, #46580, .T. ) ;
#2948=CARTESIAN_POINT ( 'NONE',  ( -22.60239429201187278, -10.09890714409725199, 70.01178508710252402 ) ) ;
#2949=CARTESIAN_POINT ( 'NONE',  ( -23.33763712988734440, -19.34056874305829510, 58.99072323483983382 ) ) ;
#2953=( BOUNDED_SURFACE ( )  B_SPLINE_SURFACE ( 3, 1, ( 
 ( #9739, #2336 ),
 ( #17344, #29166 ),
 ( #32387, #16182 ),
 ( #28680, #36527 ),
 ( #43715, #9969 ),
 ( #36298, #2581 ),
 ( #17584, #31224 ) ),
 .UNSPECIFIED., .T., .F., .F. ) 
 B_SPLINE_SURFACE_WITH_KNOTS ( ( 4, 3, 4 ),
 ( 2, 2 ),
 ( 0.000000000000000000, 0.5000000000000000000, 1.000000000000000000 ),
 ( 0.000000000000000000, 1.000000000000000000 ),
 .UNSPECIFIED. ) 
 GEOMETRIC_REPRESENTATION_ITEM ( )  RATIONAL_B_SPLINE_SURFACE ( (
 ( 1.000000000000000000, 1.000000000000000000),
 ( 0.3333333333333335369, 0.3333333333333330373),
 ( 0.3333333333333335369, 0.3333333333333330373),
 ( 1.000000000000000000, 1.000000000000000000),
 ( 0.3333333333333333703, 0.3333333333333333703),
 ( 0.3333333333333333703, 0.3333333333333333703),
 ( 1.000000000000000000, 1.000000000000000000) ) ) 
 REPRESENTATION_ITEM ( '' )  SURFACE ( )  );
#2955=CARTESIAN_POINT ( 'NONE',  ( -24.45714095472541771, -14.31630891555219165, 69.66747352629326429 ) ) ;
#2956=CARTESIAN_POINT ( 'NONE',  ( -11.29134393598116759, -11.33126488396075437, 64.16354160640879911 ) ) ;
#2958=ORIENTED_EDGE ( 'NONE', *, *, #33706, .F. ) ;
#2960=CARTESIAN_POINT ( 'NONE',  ( -24.47697530877170990, -14.85041752174647733, 63.12785080464042409 ) ) ;
#2961=DIRECTION ( 'NONE',  ( -0.9918916210775229336, -0.1270866320121812332, 6.503929234589265847E-08 ) ) ;
#2962=ORIENTED_EDGE ( 'NONE', *, *, #8108, .F. ) ;
#2963=DIRECTION ( 'NONE',  ( -0.9294853595766551235, -0.3688590060343601706, 1.396818737099928616E-16 ) ) ;
#2964=( BOUNDED_CURVE ( )  B_SPLINE_CURVE ( 3, ( #28897, #33534, #39990, #6740 ),
 .UNSPECIFIED., .F., .F. ) 
 B_SPLINE_CURVE_WITH_KNOTS ( ( 4, 4 ),
 ( 0.5000000000000000000, 0.9074455897393621795 ),
 .UNSPECIFIED. ) 
 CURVE ( )  GEOMETRIC_REPRESENTATION_ITEM ( )  RATIONAL_B_SPLINE_CURVE ( ( 1.000000000000000888, 0.4567392136813415160, 0.3561768502900331534, 0.6983129098260766332 ) ) 
 REPRESENTATION_ITEM ( '' )  );
#2965=ORIENTED_EDGE ( 'NONE', *, *, #48207, .F. ) ;
#2966=CARTESIAN_POINT ( 'NONE',  ( -10.99582063857411995, -11.91441743271276188, 74.55840195587596497 ) ) ;
#2968=LINE ( 'NONE', #32769, #20724 ) ;
#2969=CARTESIAN_POINT ( 'NONE',  ( -24.49635618495769407, -12.46679672499890046, 73.35730262454691797 ) ) ;
#2970=EDGE_CURVE ( 'NONE', #47542, #18577, #3182, .T. ) ;
#2972=B_SPLINE_CURVE_WITH_KNOTS ( 'NONE', 1,
 ( #44519, #3143 ),
 .UNSPECIFIED., .F., .F.,
 ( 2, 2 ),
 ( 0.000000000000000000, 1.000000000000000000 ),
 .UNSPECIFIED. ) ;
#2974=EDGE_CURVE ( 'NONE', #41284, #24527, #39070, .T. ) ;
#2975=AXIS2_PLACEMENT_3D ( 'NONE', #21900, #21437, #33442 ) ;
#2976=CARTESIAN_POINT ( 'NONE',  ( -24.86610161942810038, -14.46236550061385984, 66.29797407254456232 ) ) ;
#2977=FACE_OUTER_BOUND ( 'NONE', #38275, .T. ) ;
#2979=ORIENTED_EDGE ( 'NONE', *, *, #32814, .T. ) ;
#2980=CARTESIAN_POINT ( 'NONE',  ( -20.57801275890795267, -8.499987852562307822, 66.87284105708988591 ) ) ;
#2985=FACE_OUTER_BOUND ( 'NONE', #21104, .T. ) ;
#2986=EDGE_CURVE ( 'NONE', #12909, #43562, #43194, .T. ) ;
#2987=CARTESIAN_POINT ( 'NONE',  ( -16.52839481157216639, -21.81011260682906183, 58.44152394349971047 ) ) ;
#2988=CARTESIAN_POINT ( 'NONE',  ( -24.20300570612225499, -13.06358601049079482, 62.84766556631919343 ) ) ;
#2989=ORIENTED_EDGE ( 'NONE', *, *, #43931, .F. ) ;
#2991=B_SPLINE_CURVE_WITH_KNOTS ( 'NONE', 3,
 ( #15371, #3839, #22543, #15622, #30193, #26970, #14625, #44977, #11226, #30678 ),
 .UNSPECIFIED., .F., .F.,
 ( 4, 2, 2, 2, 4 ),
 ( 0.6272669072877863350, 0.7522669073072822954, 0.8772669073267782558, 1.002266907346274216, 1.127266907365770177 ),
 .UNSPECIFIED. ) ;
#2992=CARTESIAN_POINT ( 'NONE',  ( -16.98261445675647963, -21.79527095473675402, 72.46543221550747660 ) ) ;
#2994=ORIENTED_EDGE ( 'NONE', *, *, #25328, .T. ) ;
#2997=CARTESIAN_POINT ( 'NONE',  ( -11.34825743494507400, -18.28566363406474693, 58.10714629622172112 ) ) ;
#2999=CARTESIAN_POINT ( 'NONE',  ( -12.10599122619147749, -20.02663529450013513, 61.58173959111590534 ) ) ;
#3000=ADVANCED_FACE ( 'NONE', ( #44558 ), #25834, .T. ) ;
#3001=CARTESIAN_POINT ( 'NONE',  ( -24.83433702558981082, -14.04005949775414663, 73.22997357260834406 ) ) ;
#3002=CARTESIAN_POINT ( 'NONE',  ( -23.33103958787803478, -18.66444169543841269, 73.06368517745727331 ) ) ;
#3003=CARTESIAN_POINT ( 'NONE',  ( -14.84243821726248314, -7.820811810980328183, 57.05011197146747293 ) ) ;
#3004=VERTEX_POINT ( 'NONE', #10814 ) ;
#3006=CARTESIAN_POINT ( 'NONE',  ( -10.59656512619885227, -13.05092609425065220, 68.02360230423869325 ) ) ;
#3007=CARTESIAN_POINT ( 'NONE',  ( -18.05440415122280839, -21.83127237841607027, 65.36004252941745563 ) ) ;
#3008=CARTESIAN_POINT ( 'NONE',  ( -24.18639045584301428, -17.93591939540326408, 59.14231917793316740 ) ) ;
#3009=CYLINDRICAL_SURFACE ( 'NONE', #19699, 0.1499999999999981903 ) ;
#3011=VERTEX_POINT ( 'NONE', #22154 ) ;
#3014=ORIENTED_EDGE ( 'NONE', *, *, #17654, .F. ) ;
#3015=CARTESIAN_POINT ( 'NONE',  ( -16.98261445675647963, -21.79527095473675402, 72.46543221550747660 ) ) ;
#3020=VECTOR ( 'NONE', #117, 1000.000000000000000 ) ;
#3021=CARTESIAN_POINT ( 'NONE',  ( -15.74783386771837890, -7.961078896070159061, 70.62461975990308360 ) ) ;
#3022=CARTESIAN_POINT ( 'NONE',  ( -16.52839481157216639, -21.81011260682906183, 58.44152394349971047 ) ) ;
#3023=ORIENTED_EDGE ( 'NONE', *, *, #40879, .T. ) ;
#3024=CARTESIAN_POINT ( 'NONE',  ( -16.27008067537174796, -7.904986561263926959, 60.50028479261354875 ) ) ;
#3028=CARTESIAN_POINT ( 'NONE',  ( -24.42173158788804699, -14.58342405553281473, 66.41122531969938336 ) ) ;
#3029=CARTESIAN_POINT ( 'NONE',  ( -12.55198883488284878, -12.25722835735234639, 54.07175714974878389 ) ) ;
#3030=ORIENTED_EDGE ( 'NONE', *, *, #37682, .T. ) ;
#3031=CARTESIAN_POINT ( 'NONE',  ( -19.36683724782897897, -21.58655468785150688, 62.00975759738177118 ) ) ;
#3033=CARTESIAN_POINT ( 'NONE',  ( -9.978987780385143225, -14.53464483151434372, 67.99653628095502711 ) ) ;
#3034=ORIENTED_EDGE ( 'NONE', *, *, #36794, .T. ) ;
#3035=CARTESIAN_POINT ( 'NONE',  ( -20.19591720527444778, -7.893910298445437235, 73.89909326007249035 ) ) ;
#3037=CARTESIAN_POINT ( 'NONE',  ( -24.82767328945774210, -13.97813652794827988, 73.16625576376715401 ) ) ;
#3038=EDGE_CURVE ( 'NONE', #41056, #11741, #29724, .T. ) ;
#3039=CARTESIAN_POINT ( 'NONE',  ( -24.69822986944709697, -13.19963441799314197, 59.54763197719577761 ) ) ;
#3040=FACE_OUTER_BOUND ( 'NONE', #35287, .T. ) ;
#3042=DIRECTION ( 'NONE',  ( -2.584300828889512628E-08, -1.497441464807615962E-06, 0.9999999999988784527 ) ) ;
#3043=CARTESIAN_POINT ( 'NONE',  ( -22.92319923916556590, -10.39759239192951235, 63.07185995337425055 ) ) ;
#3044=EDGE_CURVE ( 'NONE', #13463, #20348, #16117, .T. ) ;
#3047=CYLINDRICAL_SURFACE ( 'NONE', #37681, 0.1500000000000007716 ) ;
#3048=CARTESIAN_POINT ( 'NONE',  ( -17.95017679193155047, -22.24060860892481628, 62.02535923035622289 ) ) ;
#3049=VERTEX_POINT ( 'NONE', #30769 ) ;
#3051=( BOUNDED_CURVE ( )  B_SPLINE_CURVE ( 3, ( #15242, #11570, #25611, #33463 ),
 .UNSPECIFIED., .F., .F. ) 
 B_SPLINE_CURVE_WITH_KNOTS ( ( 4, 4 ),
 ( 0.000000000000000000, 0.4074455897393602921 ),
 .UNSPECIFIED. ) 
 CURVE ( )  GEOMETRIC_REPRESENTATION_ITEM ( )  RATIONAL_B_SPLINE_CURVE ( ( 1.000000000000000000, 0.4567392136813441250, 0.3561768502900348188, 0.6983129098260720813 ) ) 
 REPRESENTATION_ITEM ( '' )  );
#3052=EDGE_CURVE ( 'NONE', #27215, #13964, #26178, .T. ) ;
#3053=CARTESIAN_POINT ( 'NONE',  ( -15.50784783684063051, -8.076599273749138774, 74.07985659288991087 ) ) ;
#3054=CARTESIAN_POINT ( 'NONE',  ( -18.56115164150112662, -7.446410555819776178, 73.88418448558978469 ) ) ;
#3055=B_SPLINE_CURVE_WITH_KNOTS ( 'NONE', 3,
 ( #24468, #13823, #16801, #43423, #39710, #28864, #17035, #39472, #13344, #36001 ),
 .UNSPECIFIED., .F., .F.,
 ( 4, 2, 2, 2, 4 ),
 ( 0.000000000000000000, 0.2500000000000000000, 0.5000000000000000000, 0.7500000000000000000, 1.000000000000000000 ),
 .UNSPECIFIED. ) ;
#3056=VERTEX_POINT ( 'NONE', #42080 ) ;
#3057=CARTESIAN_POINT ( 'NONE',  ( -10.05862351292959467, -15.92886012141397245, 64.69266982328383619 ) ) ;
#3059=B_SPLINE_CURVE_WITH_KNOTS ( 'NONE', 3,
 ( #19339, #1111, #27221, #23539, #23784, #31151, #38277, #42736, #38537, #30446 ),
 .UNSPECIFIED., .F., .F.,
 ( 4, 2, 2, 2, 4 ),
 ( 0.6272669072782822708, 0.7522669073001799767, 0.8772669073220777936, 1.002266907343975610, 1.127266907365873205 ),
 .UNSPECIFIED. ) ;
#3060=VERTEX_POINT ( 'NONE', #16192 ) ;
#3061=ORIENTED_EDGE ( 'NONE', *, *, #29431, .F. ) ;
#3062=ORIENTED_EDGE ( 'NONE', *, *, #43174, .F. ) ;
#3063=VECTOR ( 'NONE', #10142, 1000.000000000000114 ) ;
#3064=CARTESIAN_POINT ( 'NONE',  ( -11.32522400900782067, -11.27219014254736074, 60.96413645226084554 ) ) ;
#3065=CARTESIAN_POINT ( 'NONE',  ( -15.93141941972390008, -7.970206387582725149, 63.86114100741836808 ) ) ;
#3066=EDGE_CURVE ( 'NONE', #22327, #5003, #23365, .T. ) ;
#3072=B_SPLINE_CURVE_WITH_KNOTS ( 'NONE', 3,
 ( #28973, #6812, #13456, #20865, #21362, #2630, #36352, #10276, #21829, #18116 ),
 .UNSPECIFIED., .F., .F.,
 ( 4, 2, 2, 2, 4 ),
 ( 0.000000000000000000, 0.2500000000000000000, 0.5000000000000000000, 0.7500000000000000000, 1.000000000000000000 ),
 .UNSPECIFIED. ) ;
#3074=B_SPLINE_CURVE_WITH_KNOTS ( 'NONE', 3,
 ( #40611, #41116, #26588, #14483, #33963, #48247, #3196, #6895, #17955, #18445 ),
 .UNSPECIFIED., .F., .F.,
 ( 4, 2, 2, 2, 4 ),
 ( 0.000000000000000000, 0.2500000000000000000, 0.5000000000000000000, 0.7500000000000000000, 1.000000000000000000 ),
 .UNSPECIFIED. ) ;
#3075=CARTESIAN_POINT ( 'NONE',  ( -19.88388893082392528, -8.193741602349351894, 70.40667630031393287 ) ) ;
#3076=EDGE_CURVE ( 'NONE', #14119, #42743, #38360, .T. ) ;
#3077=CARTESIAN_POINT ( 'NONE',  ( -22.05923734882601295, -20.05472318235705131, 62.53439162613685909 ) ) ;
#3079=EDGE_LOOP ( 'NONE', ( #19123, #47899 ) ) ;
#3081=CARTESIAN_POINT ( 'NONE',  ( -22.11022017764905456, -20.07639638992645104, 62.53439153403956396 ) ) ;
#3082=CARTESIAN_POINT ( 'NONE',  ( -22.09234508783963236, -20.09219152016766685, 62.38439162497947166 ) ) ;
#3083=EDGE_LOOP ( 'NONE', ( #26250, #25541, #27967, #44915, #38356 ) ) ;
#3089=CARTESIAN_POINT ( 'NONE',  ( -24.83010077369927515, -14.00069395148988605, 73.32260284066204292 ) ) ;
#3090=CARTESIAN_POINT ( 'NONE',  ( -21.59804182614902146, -20.98026282434625500, 72.70941811628220819 ) ) ;
#3091=ORIENTED_EDGE ( 'NONE', *, *, #46108, .F. ) ;
#3092=CARTESIAN_POINT ( 'NONE',  ( -10.70532053225239366, -12.67267096592666675, 61.08381491717225487 ) ) ;
#3094=( BOUNDED_SURFACE ( )  B_SPLINE_SURFACE ( 3, 1, ( 
 ( #24431, #27863 ),
 ( #43386, #42890 ),
 ( #35488, #16766 ),
 ( #27629, #31805 ),
 ( #35720, #13069 ),
 ( #9406, #9655 ),
 ( #8685, #2240 ) ),
 .UNSPECIFIED., .T., .F., .F. ) 
 B_SPLINE_SURFACE_WITH_KNOTS ( ( 4, 3, 4 ),
 ( 2, 2 ),
 ( 0.000000000000000000, 0.5000000000000000000, 1.000000000000000000 ),
 ( 0.000000000000000000, 1.000000000000000000 ),
 .UNSPECIFIED. ) 
 GEOMETRIC_REPRESENTATION_ITEM ( )  RATIONAL_B_SPLINE_SURFACE ( (
 ( 1.000000000000000000, 1.000000000000000000),
 ( 0.3333333333333335369, 0.3333333333333330373),
 ( 0.3333333333333335369, 0.3333333333333330373),
 ( 1.000000000000000000, 1.000000000000000000),
 ( 0.3333333333333333703, 0.3333333333333333703),
 ( 0.3333333333333333703, 0.3333333333333333703),
 ( 1.000000000000000000, 1.000000000000000000) ) ) 
 REPRESENTATION_ITEM ( '' )  SURFACE ( )  );
#3095=CARTESIAN_POINT ( 'NONE',  ( -22.96475595555910942, -9.828888949534857034, 70.16178519762588905 ) ) ;
#3096=CARTESIAN_POINT ( 'NONE',  ( -10.09159279195849379, -16.12743201725144360, 68.17041960190522332 ) ) ;
#3097=ORIENTED_EDGE ( 'NONE', *, *, #33554, .T. ) ;
#3099=CARTESIAN_POINT ( 'NONE',  ( -21.36564388993269148, -20.65448255276599809, 72.82446398674419186 ) ) ;
#3100=CARTESIAN_POINT ( 'NONE',  ( -21.52725980274252393, -9.076272844571150245, 70.43132538913752683 ) ) ;
#3101=ORIENTED_EDGE ( 'NONE', *, *, #17983, .T. ) ;
#3102=LINE ( 'NONE', #11720, #25007 ) ;
#3103=ORIENTED_EDGE ( 'NONE', *, *, #32752, .F. ) ;
#3105=CARTESIAN_POINT ( 'NONE',  ( -13.12040755923265500, -20.89053954678383462, 58.22462863256119903 ) ) ;
#3106=CARTESIAN_POINT ( 'NONE',  ( -12.79725838692604434, -20.12850099319811292, 71.80653676770127447 ) ) ;
#3108=ADVANCED_FACE ( 'NONE', ( #11803 ), #34756, .T. ) ;
#3109=CARTESIAN_POINT ( 'NONE',  ( -21.17162584072666220, -21.24822939621656559, 65.72420603834571295 ) ) ;
#3111=CARTESIAN_POINT ( 'NONE',  ( -22.07364868997043672, -9.574310151912669653, 59.83244270001737419 ) ) ;
#3113=CARTESIAN_POINT ( 'NONE',  ( -11.16004581379495342, -11.56782820372427167, 64.03393219759587396 ) ) ;
#3114=B_SPLINE_CURVE_WITH_KNOTS ( 'NONE', 3,
 ( #6814, #39577, #21831, #29464, #21599, #32669, #10746, #39817, #32896, #40536 ),
 .UNSPECIFIED., .F., .F.,
 ( 4, 2, 2, 2, 4 ),
 ( 0.000000000000000000, 0.2500000000000000000, 0.5000000000000000000, 0.7500000000000000000, 1.000000000000000000 ),
 .UNSPECIFIED. ) ;
#3115=CARTESIAN_POINT ( 'NONE',  ( -15.41750689856725565, -7.634439986883705842, 74.33631595678771475 ) ) ;
#3116=ORIENTED_EDGE ( 'NONE', *, *, #38582, .F. ) ;
#3118=( BOUNDED_CURVE ( )  B_SPLINE_CURVE ( 3, ( #3780, #37739, #30382, #42181 ),
 .UNSPECIFIED., .F., .F. ) 
 B_SPLINE_CURVE_WITH_KNOTS ( ( 4, 4 ),
 ( 0.5000000000000000000, 0.9074455897393630677 ),
 .UNSPECIFIED. ) 
 CURVE ( )  GEOMETRIC_REPRESENTATION_ITEM ( )  RATIONAL_B_SPLINE_CURVE ( ( 0.9999999999999968914, 0.4567392136813352987, 0.3561768502900335975, 0.6983129098260885126 ) ) 
 REPRESENTATION_ITEM ( '' )  );
#3119=CARTESIAN_POINT ( 'NONE',  ( -11.96194199484143539, -9.742791280557115741, 60.60272182217008208 ) ) ;
#3120=ORIENTED_EDGE ( 'NONE', *, *, #23272, .F. ) ;
#3122=CARTESIAN_POINT ( 'NONE',  ( -14.93108437845038594, -21.82978844404615160, 65.36242591972883531 ) ) ;
#3124=CARTESIAN_POINT ( 'NONE',  ( -15.19549097431359463, -21.91815212410659086, 68.76088336006283441 ) ) ;
#3126=CARTESIAN_POINT ( 'NONE',  ( -23.46236539141196076, -19.17297946188329405, 62.46068554577072263 ) ) ;
#3127=DIRECTION ( 'NONE',  ( 1.916827916228666765E-06, 6.156520255201565618E-06, -0.9999999999792115180 ) ) ;
#3129=DIRECTION ( 'NONE',  ( 0.9753750245375037986, 0.2205528542287732707, 7.244220459260263973E-08 ) ) ;
#3130=CARTESIAN_POINT ( 'NONE',  ( -20.31413516131974362, -8.378470924821744603, 67.06632013881642251 ) ) ;
#3132=EDGE_CURVE ( 'NONE', #9892, #28, #32626, .T. ) ;
#3135=CARTESIAN_POINT ( 'NONE',  ( -24.30048588269890431, -16.36411231998812710, 59.12332431758469653 ) ) ;
#3136=EDGE_CURVE ( 'NONE', #35971, #9441, #7968, .T. ) ;
#3138=ADVANCED_FACE ( 'NONE', ( #43542 ), #1921, .F. ) ;
#3142=CARTESIAN_POINT ( 'NONE',  ( -18.96308807049092238, -7.519770507884219413, 67.07788641161226906 ) ) ;
#3143=CARTESIAN_POINT ( 'NONE',  ( -23.34092575347512266, -10.28207967581048088, 59.78698817202694471 ) ) ;
#3145=B_SPLINE_CURVE_WITH_KNOTS ( 'NONE', 3,
 ( #25114, #2692, #27050, #11799, #26085, #7871, #19415, #42075, #48474, #4397 ),
 .UNSPECIFIED., .F., .F.,
 ( 4, 2, 2, 2, 4 ),
 ( 0.1272669073658451999, 0.2522669073488033042, 0.3772669073317613808, 0.5022669073147194574, 0.6272669072976775340 ),
 .UNSPECIFIED. ) ;
#3149=CARTESIAN_POINT ( 'NONE',  ( -11.05034076241727625, -11.79557573020262318, 71.37388789199357575 ) ) ;
#3150=CARTESIAN_POINT ( 'NONE',  ( -18.20818224600564150, -22.21799970308342154, 65.50565518846025270 ) ) ;
#3152=CYLINDRICAL_SURFACE ( 'NONE', #21202, 0.1500000000000048794 ) ;
#3153=CARTESIAN_POINT ( 'NONE',  ( -21.39967327233876304, -20.63170314183283693, 72.80974286114339122 ) ) ;
#3155=VECTOR ( 'NONE', #7116, 1000.000000000000227 ) ;
#3156=ORIENTED_EDGE ( 'NONE', *, *, #27149, .T. ) ;
#3157=FACE_OUTER_BOUND ( 'NONE', #880, .T. ) ;
#3159=ORIENTED_EDGE ( 'NONE', *, *, #34982, .F. ) ;
#3160=DIRECTION ( 'NONE',  ( -3.549360974554993999E-17, 6.371834667797928663E-18, 1.000000000000000000 ) ) ;
#3162=ORIENTED_EDGE ( 'NONE', *, *, #23073, .T. ) ;
#3163=( BOUNDED_CURVE ( )  B_SPLINE_CURVE ( 3, ( #15631, #38274, #35075, #45457 ),
 .UNSPECIFIED., .F., .F. ) 
 B_SPLINE_CURVE_WITH_KNOTS ( ( 4, 4 ),
 ( 0.5000000000000000000, 0.9074455897393711723 ),
 .UNSPECIFIED. ) 
 CURVE ( )  GEOMETRIC_REPRESENTATION_ITEM ( )  RATIONAL_B_SPLINE_CURVE ( ( 0.9999999999999897859, 0.4567392136813225867, 0.3561768502900338751, 0.6983129098261126044 ) ) 
 REPRESENTATION_ITEM ( '' )  );
#3165=CARTESIAN_POINT ( 'NONE',  ( -17.65301634040397261, -7.362555908020970818, 63.69023642131870133 ) ) ;
#3166=VERTEX_POINT ( 'NONE', #1429 ) ;
#3168=CARTESIAN_POINT ( 'NONE',  ( -20.29576906775320921, -8.423958474866362067, 70.32270528577072355 ) ) ;
#3171=FACE_OUTER_BOUND ( 'NONE', #29667, .T. ) ;
#3174=CARTESIAN_POINT ( 'NONE',  ( -10.72552571836178181, -12.61109718544098612, 60.79853568372239891 ) ) ;
#3175=ORIENTED_EDGE ( 'NONE', *, *, #14116, .T. ) ;
#3176=CARTESIAN_POINT ( 'NONE',  ( -10.48067321144888808, -16.03043919553437036, 68.12767830706636119 ) ) ;
#3177=CARTESIAN_POINT ( 'NONE',  ( -11.36226365097591184, -11.30848497612717374, 60.69388164123920859 ) ) ;
#3178=CARTESIAN_POINT ( 'NONE',  ( -21.34582186320181307, -20.66775149956831115, 72.82446429489806405 ) ) ;
#3179=VERTEX_POINT ( 'NONE', #46745 ) ;
#3181=CARTESIAN_POINT ( 'NONE',  ( -14.07539661982785262, -8.605278201040592378, 74.34954655214895070 ) ) ;
#3182=LINE ( 'NONE', #44093, #3752 ) ;
#3183=CARTESIAN_POINT ( 'NONE',  ( -20.77185612116493374, -8.153571591454063849, 63.47268022219622452 ) ) ;
#3185=CARTESIAN_POINT ( 'NONE',  ( -15.87557486115803052, -7.931373420853707223, 67.44007279014866185 ) ) ;
#3186=CARTESIAN_POINT ( 'NONE',  ( -13.83248983650026709, -21.33638410845934885, 72.18253639678975730 ) ) ;
#3187=FACE_OUTER_BOUND ( 'NONE', #37840, .T. ) ;
#3189=ORIENTED_EDGE ( 'NONE', *, *, #40961, .T. ) ;
#3192=EDGE_CURVE ( 'NONE', #45223, #28690, #9572, .T. ) ;
#3194=AXIS2_PLACEMENT_3D ( 'NONE', #30568, #11591, #37930 ) ;
#3196=CARTESIAN_POINT ( 'NONE',  ( -13.57788044043476461, -8.959030902765807269, 60.66780251997597873 ) ) ;
#3200=ORIENTED_EDGE ( 'NONE', *, *, #45025, .F. ) ;
#3201=CARTESIAN_POINT ( 'NONE',  ( -11.46044050272623416, -11.04924139602722200, 57.20903212151935691 ) ) ;
#3203=ADVANCED_FACE ( 'NONE', ( #43297 ), #18051, .T. ) ;
#3207=ORIENTED_EDGE ( 'NONE', *, *, #41461, .F. ) ;
#3209=CARTESIAN_POINT ( 'NONE',  ( -23.79049241923990721, -17.71949969818489379, 59.01880874247220987 ) ) ;
#3210=EDGE_CURVE ( 'NONE', #26240, #37436, #40721, .T. ) ;
#3211=ORIENTED_EDGE ( 'NONE', *, *, #39961, .T. ) ;
#3212=CARTESIAN_POINT ( 'NONE',  ( -22.38280345442485242, -20.36932031849321589, 62.27793240076999126 ) ) ;
#3213=CARTESIAN_POINT ( 'NONE',  ( -19.77436091090941517, -21.87886160397694368, 65.64981624214608757 ) ) ;
#3215=ORIENTED_EDGE ( 'NONE', *, *, #16956, .T. ) ;
#3216=DIRECTION ( 'NONE',  ( 0.8467008005855415353, -0.3141239757129648535, 0.4294460177601879258 ) ) ;
#3217=ORIENTED_EDGE ( 'NONE', *, *, #47720, .F. ) ;
#3218=CARTESIAN_POINT ( 'NONE',  ( -23.78282461406436710, -10.92707771475091150, 73.53910168191997343 ) ) ;
#3220=FACE_OUTER_BOUND ( 'NONE', #9750, .T. ) ;
#3221=B_SPLINE_CURVE_WITH_KNOTS ( 'NONE', 3,
 ( #32464, #3142, #36377, #33160, #2889, #2659, #48197, #17895, #32921, #40559 ),
 .UNSPECIFIED., .F., .F.,
 ( 4, 2, 2, 2, 4 ),
 ( 0.6272669072877943286, 0.7522669073073021684, 0.8772669073268100082, 1.002266907346317737, 1.127266907365825688 ),
 .UNSPECIFIED. ) ;
#3223=CARTESIAN_POINT ( 'NONE',  ( -16.26195973558533581, -21.76306465430365122, 58.57113428431811997 ) ) ;
#3224=CARTESIAN_POINT ( 'NONE',  ( -10.27391136003569905, -12.71670657087258327, 64.31190181376453552 ) ) ;
#3228=CARTESIAN_POINT ( 'NONE',  ( -23.74985771237617627, -17.93965049410213197, 62.61793715156320417 ) ) ;
#3233=CARTESIAN_POINT ( 'NONE',  ( -24.46146587544552276, -14.38248120490118609, 66.46820668217904426 ) ) ;
#3234=FACE_OUTER_BOUND ( 'NONE', #10450, .T. ) ;
#3236=CARTESIAN_POINT ( 'NONE',  ( -13.82836502510361854, -20.88256612802230450, 61.67213144371572042 ) ) ;
#3237=LINE ( 'NONE', #36236, #20365 ) ;
#3240=ORIENTED_EDGE ( 'NONE', *, *, #27152, .F. ) ;
#3242=CARTESIAN_POINT ( 'NONE',  ( -20.98579777188748707, -20.83533835786949950, 65.58453944793343737 ) ) ;
#3243=ORIENTED_EDGE ( 'NONE', *, *, #6757, .F. ) ;
#3244=CARTESIAN_POINT ( 'NONE',  ( -14.72778380697628187, -21.32322314059345558, 58.16617885012796307 ) ) ;
#3247=CARTESIAN_POINT ( 'NONE',  ( -24.17271927670314113, -12.95015993349377048, 66.30246741691458112 ) ) ;
#3248=CARTESIAN_POINT ( 'NONE',  ( -12.36648897341435749, -9.886239853951966694, 64.17347106801278755 ) ) ;
#3249=CARTESIAN_POINT ( 'NONE',  ( -14.53767063111817137, -21.24453063237525541, 58.58106478802027084 ) ) ;
#3250=( BOUNDED_CURVE ( )  B_SPLINE_CURVE ( 3, ( #46075, #8901, #31541, #22960 ),
 .UNSPECIFIED., .F., .F. ) 
 B_SPLINE_CURVE_WITH_KNOTS ( ( 4, 4 ),
 ( 0.9074455897393663983, 1.000000000000000000 ),
 .UNSPECIFIED. ) 
 CURVE ( )  GEOMETRIC_REPRESENTATION_ITEM ( )  RATIONAL_B_SPLINE_CURVE ( ( 0.6983129098261016132, 0.7760317562607056407, 0.8765941196520050660, 1.000000000000000000 ) ) 
 REPRESENTATION_ITEM ( '' )  );
#3251=CARTESIAN_POINT ( 'NONE',  ( -22.07016944540107062, -20.11663773636943731, 66.00421750868065374 ) ) ;
#3252=LINE ( 'NONE', #2534, #14451 ) ;
#3253=DIRECTION ( 'NONE',  ( 2.846534188916127659E-06, 1.189262794724463340E-05, 0.9999999999252312533 ) ) ;
#3254=CARTESIAN_POINT ( 'NONE',  ( -22.51726279860821833, -19.68384809141796765, 72.64400547081167758 ) ) ;
#3257=FACE_OUTER_BOUND ( 'NONE', #18674, .T. ) ;
#3259=CARTESIAN_POINT ( 'NONE',  ( -16.77411572588129118, -21.83219480353551134, 72.58031927177887610 ) ) ;
#3260=CARTESIAN_POINT ( 'NONE',  ( -11.16720114480400383, -11.56054632708127450, 67.61864607954859707 ) ) ;
#3261=CARTESIAN_POINT ( 'NONE',  ( -24.57849813159777597, -12.72878314728456850, 66.41591366067137869 ) ) ;
#3262=CARTESIAN_POINT ( 'NONE',  ( -13.71293330176565384, -21.26916511146244915, 68.64120417180296840 ) ) ;
#3263=( BOUNDED_CURVE ( )  B_SPLINE_CURVE ( 3, ( #11578, #25618, #3962, #15005 ),
 .UNSPECIFIED., .F., .F. ) 
 B_SPLINE_CURVE_WITH_KNOTS ( ( 4, 4 ),
 ( 0.000000000000000000, 0.4074455897393636783 ),
 .UNSPECIFIED. ) 
 CURVE ( )  GEOMETRIC_REPRESENTATION_ITEM ( )  RATIONAL_B_SPLINE_CURVE ( ( 1.000000000000000000, 0.4567392136813336889, 0.3561768502900309330, 0.6983129098260917322 ) ) 
 REPRESENTATION_ITEM ( '' )  );
#3264=CARTESIAN_POINT ( 'NONE',  ( -22.16605834473193326, -9.587270374048046051, 60.02171285714800320 ) ) ;
#3265=( BOUNDED_SURFACE ( )  B_SPLINE_SURFACE ( 3, 1, ( 
 ( #7759, #38241 ),
 ( #26451, #41466 ),
 ( #22775, #27420 ),
 ( #594, #4524 ),
 ( #37766, #34069 ),
 ( #15842, #1076 ),
 ( #20036, #362 ) ),
 .UNSPECIFIED., .T., .F., .F. ) 
 B_SPLINE_SURFACE_WITH_KNOTS ( ( 4, 3, 4 ),
 ( 2, 2 ),
 ( 0.000000000000000000, 0.5000000000000000000, 1.000000000000000000 ),
 ( 0.000000000000000000, 1.000000000000000000 ),
 .UNSPECIFIED. ) 
 GEOMETRIC_REPRESENTATION_ITEM ( )  RATIONAL_B_SPLINE_SURFACE ( (
 ( 1.000000000000000000, 1.000000000000000000),
 ( 0.3333333333333335369, 0.3333333333333330373),
 ( 0.3333333333333335369, 0.3333333333333330373),
 ( 1.000000000000000000, 1.000000000000000000),
 ( 0.3333333333333333703, 0.3333333333333333703),
 ( 0.3333333333333333703, 0.3333333333333333703),
 ( 1.000000000000000000, 1.000000000000000000) ) ) 
 REPRESENTATION_ITEM ( '' )  SURFACE ( )  );
#3269=ADVANCED_FACE ( 'NONE', ( #40795 ), #22091, .T. ) ;
#3271=ORIENTED_EDGE ( 'NONE', *, *, #8686, .T. ) ;
#3272=CARTESIAN_POINT ( 'NONE',  ( -23.54137353425661061, -19.06164953464739753, 65.94672567501233118 ) ) ;
#3274=CARTESIAN_POINT ( 'NONE',  ( -20.02766381537926677, -8.311286447040620473, 74.02096589762064127 ) ) ;
#3276=( BOUNDED_SURFACE ( )  B_SPLINE_SURFACE ( 3, 1, ( 
 ( #1403, #1657 ),
 ( #31210, #42553 ),
 ( #15935, #42056 ),
 ( #16664, #27033 ),
 ( #8570, #34896 ),
 ( #8823, #16420 ),
 ( #12965, #46488 ) ),
 .UNSPECIFIED., .T., .F., .F. ) 
 B_SPLINE_SURFACE_WITH_KNOTS ( ( 4, 3, 4 ),
 ( 2, 2 ),
 ( 0.000000000000000000, 0.5000000000000000000, 1.000000000000000000 ),
 ( 0.000000000000000000, 1.000000000000000000 ),
 .UNSPECIFIED. ) 
 GEOMETRIC_REPRESENTATION_ITEM ( )  RATIONAL_B_SPLINE_SURFACE ( (
 ( 1.000000000000000000, 1.000000000000000000),
 ( 0.3333333333333335369, 0.3333333333333330373),
 ( 0.3333333333333335369, 0.3333333333333330373),
 ( 1.000000000000000000, 1.000000000000000000),
 ( 0.3333333333333333703, 0.3333333333333333703),
 ( 0.3333333333333333703, 0.3333333333333333703),
 ( 1.000000000000000000, 1.000000000000000000) ) ) 
 REPRESENTATION_ITEM ( '' )  SURFACE ( )  );
#3277=CARTESIAN_POINT ( 'NONE',  ( -18.29367245688808552, -17.15309925898211674, 47.99999999999994316 ) ) ;
#3278=CARTESIAN_POINT ( 'NONE',  ( -10.37051006938303388, -14.56035623187037942, 74.94211941000891386 ) ) ;
#3279=ORIENTED_EDGE ( 'NONE', *, *, #9605, .F. ) ;
#3281=VECTOR ( 'NONE', #9714, 1000.000000000000227 ) ;
#3282=CARTESIAN_POINT ( 'NONE',  ( -22.48940708121607202, -20.36508298871479283, 53.76227901944322696 ) ) ;
#3283=VERTEX_POINT ( 'NONE', #3368 ) ;
#3284=CARTESIAN_POINT ( 'NONE',  ( -24.66730449611544529, -13.06573935865489844, 62.94768786448354092 ) ) ;
#3285=LINE ( 'NONE', #29626, #22008 ) ;
#3287=DIRECTION ( 'NONE',  ( -5.215802026392426595E-06, 6.671378403414619972E-06, 0.9999999999641440152 ) ) ;
#3288=CARTESIAN_POINT ( 'NONE',  ( -15.06268261486706983, -8.219072439155830523, 56.86616596445847449 ) ) ;
#3290=CARTESIAN_POINT ( 'NONE',  ( -11.96654139922548232, -19.88064104245263408, 58.04869629833985556 ) ) ;
#3292=CARTESIAN_POINT ( 'NONE',  ( -24.44055745662519641, -14.11932379769929113, 73.13743607903229815 ) ) ;
#3294=CARTESIAN_POINT ( 'NONE',  ( -21.89264518680100835, -20.26253109894388160, 58.77915004610762395 ) ) ;
#3295=ORIENTED_EDGE ( 'NONE', *, *, #21753, .F. ) ;
#3298=CARTESIAN_POINT ( 'NONE',  ( -16.68462913526379765, -22.29107483173095261, 53.76227901944321275 ) ) ;
#3300=ORIENTED_EDGE ( 'NONE', *, *, #22565, .T. ) ;
#3301=CARTESIAN_POINT ( 'NONE',  ( -24.25486363958986757, -13.06355980472538292, 63.11792038370487035 ) ) ;
#3304=DIRECTION ( 'NONE',  ( -0.3478314405900308492, -0.9375570856950864451, 0.000000000000000000 ) ) ;
#3306=FACE_OUTER_BOUND ( 'NONE', #44471, .T. ) ;
#3308=B_SPLINE_CURVE_WITH_KNOTS ( 'NONE', 3,
 ( #28783, #13506, #9609, #43575, #25572, #24621, #40577, #33181, #40350, #2674 ),
 .UNSPECIFIED., .F., .F.,
 ( 4, 2, 2, 2, 4 ),
 ( 0.000000000000000000, 0.2500000000000000000, 0.5000000000000000000, 0.7500000000000000000, 1.000000000000000000 ),
 .UNSPECIFIED. ) ;
#3309=EDGE_LOOP ( 'NONE', ( #41914, #13118, #27432, #24464, #23819 ) ) ;
#3310=CARTESIAN_POINT ( 'NONE',  ( -19.96994565995125015, -21.32983830779690848, 72.70478737306767414 ) ) ;
#3311=ORIENTED_EDGE ( 'NONE', *, *, #42007, .T. ) ;
#3313=EDGE_LOOP ( 'NONE', ( #7667, #1305, #8375, #45381 ) ) ;
#3315=CARTESIAN_POINT ( 'NONE',  ( -11.18734459328334907, -11.50497870355291319, 60.83452645039198359 ) ) ;
#3316=DIRECTION ( 'NONE',  ( 1.011289380940303784E-05, -7.260693215641691253E-06, 0.9999999999225058778 ) ) ;
#3318=CARTESIAN_POINT ( 'NONE',  ( -13.24261710015883864, -8.643249176123326549, 60.55454998173587455 ) ) ;
#3319=ORIENTED_EDGE ( 'NONE', *, *, #26112, .F. ) ;
#3320=ORIENTED_EDGE ( 'NONE', *, *, #42961, .T. ) ;
#3322=EDGE_CURVE ( 'NONE', #1165, #33555, #19666, .T. ) ;
#3325=EDGE_CURVE ( 'NONE', #6697, #24590, #11429, .T. ) ;
#3329=CARTESIAN_POINT ( 'NONE',  ( -10.80526167902494805, -12.38110965600595215, 57.33417096153107195 ) ) ;
#3331=CARTESIAN_POINT ( 'NONE',  ( -11.56806251476610115, -18.73522173559940995, 65.03234934376791898 ) ) ;
#3333=VERTEX_POINT ( 'NONE', #40076 ) ;
#3336=ORIENTED_EDGE ( 'NONE', *, *, #16877, .F. ) ;
#3337=CARTESIAN_POINT ( 'NONE',  ( -13.22529448846758804, -9.145569705956512863, 64.19474388871357462 ) ) ;
#3338=CARTESIAN_POINT ( 'NONE',  ( -10.12334741456209208, -16.29302180943733802, 71.64761590623798782 ) ) ;
#3340=CARTESIAN_POINT ( 'NONE',  ( -13.65110067086344792, -21.23324738024127356, 68.57129742521463811 ) ) ;
#3341=VERTEX_POINT ( 'NONE', #3615 ) ;
#3342=CARTESIAN_POINT ( 'NONE',  ( -18.94833981748636376, -7.977060738621439384, 66.90071832655067396 ) ) ;
#3343=CARTESIAN_POINT ( 'NONE',  ( -24.20884359724224311, -11.73171579724705005, 59.59740298356196320 ) ) ;
#3344=( BOUNDED_CURVE ( )  B_SPLINE_CURVE ( 3, ( #20334, #31896, #17588, #9506 ),
 .UNSPECIFIED., .F., .F. ) 
 B_SPLINE_CURVE_WITH_KNOTS ( ( 4, 4 ),
 ( 0.4074455897393596260, 0.5000000000000000000 ),
 .UNSPECIFIED. ) 
 CURVE ( )  GEOMETRIC_REPRESENTATION_ITEM ( )  RATIONAL_B_SPLINE_CURVE ( ( 0.6983129098260822953, 0.7760317562606835473, 0.8765941196519878575, 0.9999999999999914513 ) ) 
 REPRESENTATION_ITEM ( '' )  );
#3345=CARTESIAN_POINT ( 'NONE',  ( -12.18836193727821460, -19.53083876418623532, 57.94154444592973618 ) ) ;
#3346=CARTESIAN_POINT ( 'NONE',  ( -10.07807850977444097, -16.05059584699720432, 68.13914376727996114 ) ) ;
#3348=CARTESIAN_POINT ( 'NONE',  ( -10.37459419693011853, -14.72189344584419679, 71.62782694350063650 ) ) ;
#3350=CARTESIAN_POINT ( 'NONE',  ( -17.39742543611924930, -7.759256981132186759, 67.32039592192056432 ) ) ;
#3351=ORIENTED_EDGE ( 'NONE', *, *, #24060, .F. ) ;
#3352=DIRECTION ( 'NONE',  ( -1.653275063147722522E-06, 1.135554159962570470E-05, 0.9999999999341591117 ) ) ;
#3353=ORIENTED_EDGE ( 'NONE', *, *, #18963, .F. ) ;
#3355=CARTESIAN_POINT ( 'NONE',  ( -14.06084784944548716, -21.00867483325099982, 68.34136283933983691 ) ) ;
#3356=CARTESIAN_POINT ( 'NONE',  ( -24.47354778464749003, -12.39902454472287197, 73.42720984402279782 ) ) ;
#3357=CARTESIAN_POINT ( 'NONE',  ( -16.13263948075386978, -7.878200451182638453, 63.68483172840383588 ) ) ;
#3358=ORIENTED_EDGE ( 'NONE', *, *, #3901, .T. ) ;
#3360=EDGE_LOOP ( 'NONE', ( #8963, #14168, #24898, #43631, #46606 ) ) ;
#3361=CARTESIAN_POINT ( 'NONE',  ( -17.79084088774826000, -7.768752266068899459, 60.08060768310445354 ) ) ;
#3364=CARTESIAN_POINT ( 'NONE',  ( -10.76785811675247118, -12.48515291162924434, 57.61385273545094066 ) ) ;
#3365=CARTESIAN_POINT ( 'NONE',  ( -13.47672066442975236, -20.59013050379473952, 58.06152457431510072 ) ) ;
#3368=CARTESIAN_POINT ( 'NONE',  ( -16.78341213209640159, -22.23169296657789928, 68.88056055876903372 ) ) ;
#3369=CARTESIAN_POINT ( 'NONE',  ( -18.31357888663954725, -21.80286911112441572, 69.11514702303101387 ) ) ;
#3370=CARTESIAN_POINT ( 'NONE',  ( -23.43824811396329011, -19.20609618851374023, 62.45432639691269117 ) ) ;
#3371=FACE_OUTER_BOUND ( 'NONE', #34261, .T. ) ;
#3372=CARTESIAN_POINT ( 'NONE',  ( -23.73684003905821527, -18.76684476618103403, 72.95023626440647035 ) ) ;
#3373=CARTESIAN_POINT ( 'NONE',  ( -14.06695675121984301, -8.606427752881131710, 70.61468953885895417 ) ) ;
#3374=ADVANCED_FACE ( 'NONE', ( #2644 ), #11452, .T. ) ;
#3375=CARTESIAN_POINT ( 'NONE',  ( -14.81397530905920235, -21.78719282451566386, 61.79633834696925732 ) ) ;
#3376=VERTEX_POINT ( 'NONE', #37831 ) ;
#3377=ORIENTED_EDGE ( 'NONE', *, *, #39188, .T. ) ;
#3379=B_SPLINE_CURVE_WITH_KNOTS ( 'NONE', 3,
 ( #36277, #39738, #9717, #29139, #28892, #43448, #2560, #13127, #43941, #44190 ),
 .UNSPECIFIED., .F., .F.,
 ( 4, 2, 2, 2, 4 ),
 ( 0.1272669073658177219, 0.2522669073463039702, 0.3772669073267902462, 0.5022669073072765222, 0.6272669072877627983 ),
 .UNSPECIFIED. ) ;
#3382=DIRECTION ( 'NONE',  ( -0.3722980621098836984, -0.2477784351981131006, 0.8944271909999157444 ) ) ;
#3385=VERTEX_POINT ( 'NONE', #33630 ) ;
#3386=EDGE_CURVE ( 'NONE', #21212, #29021, #3761, .T. ) ;
#3387=CARTESIAN_POINT ( 'NONE',  ( -24.34625376782045336, -15.85315735139701587, 69.54924175052593682 ) ) ;
#3388=CARTESIAN_POINT ( 'NONE',  ( -12.27604185553471616, -19.62628656662749549, 58.21210303282668264 ) ) ;
#3393=( BOUNDED_CURVE ( )  B_SPLINE_CURVE ( 3, ( #6132, #32479, #2903, #6618 ),
 .UNSPECIFIED., .F., .F. ) 
 B_SPLINE_CURVE_WITH_KNOTS ( ( 4, 4 ),
 ( 0.000000000000000000, 0.4074455897393625126 ),
 .UNSPECIFIED. ) 
 CURVE ( )  GEOMETRIC_REPRESENTATION_ITEM ( )  RATIONAL_B_SPLINE_CURVE ( ( 1.000000000000000000, 0.4567392136813230863, 0.3561768502900269917, 0.6983129098261117162 ) ) 
 REPRESENTATION_ITEM ( '' )  );
#3395=CARTESIAN_POINT ( 'NONE',  ( -21.62175721279969665, -9.207301523296434809, 66.96149954034976304 ) ) ;
#3396=EDGE_LOOP ( 'NONE', ( #6813, #12285, #24784, #12192, #34139 ) ) ;
#3397=CARTESIAN_POINT ( 'NONE',  ( -10.40888626530166405, -14.10966241957602207, 60.91821293886854249 ) ) ;
#3399=CARTESIAN_POINT ( 'NONE',  ( -10.40035142239662669, -15.50347837920617167, 64.65204674534754758 ) ) ;
#3400=VERTEX_POINT ( 'NONE', #33895 ) ;
#3402=( BOUNDED_CURVE ( )  B_SPLINE_CURVE ( 3, ( #44978, #48155, #28955, #48639 ),
 .UNSPECIFIED., .F., .F. ) 
 B_SPLINE_CURVE_WITH_KNOTS ( ( 4, 4 ),
 ( 0.000000000000000000, 0.4074455897393629566 ),
 .UNSPECIFIED. ) 
 CURVE ( )  GEOMETRIC_REPRESENTATION_ITEM ( )  RATIONAL_B_SPLINE_CURVE ( ( 1.000000000000000000, 0.4567392136813334114, 0.3561768502900308775, 0.6983129098260923984 ) ) 
 REPRESENTATION_ITEM ( '' )  );
#3403=EDGE_CURVE ( 'NONE', #25120, #17121, #41534, .T. ) ;
#3404=ORIENTED_EDGE ( 'NONE', *, *, #37848, .F. ) ;
#3405=CARTESIAN_POINT ( 'NONE',  ( -24.47423110178408479, -14.79660573996179451, 59.53740478059303598 ) ) ;
#3406=CARTESIAN_POINT ( 'NONE',  ( -24.87123160714014958, -14.59964084223042491, 62.89791924484052998 ) ) ;
#3407=ORIENTED_EDGE ( 'NONE', *, *, #35110, .T. ) ;
#3408=ADVANCED_FACE ( 'NONE', ( #7821 ), #24709, .T. ) ;
#3409=EDGE_CURVE ( 'NONE', #47072, #26020, #12954, .T. ) ;
#3412=B_SPLINE_CURVE_WITH_KNOTS ( 'NONE', 1,
 ( #40751, #33100 ),
 .UNSPECIFIED., .F., .F.,
 ( 2, 2 ),
 ( 0.000000000000000000, 1.000000000000000000 ),
 .UNSPECIFIED. ) ;
#3413=ORIENTED_EDGE ( 'NONE', *, *, #39062, .F. ) ;
#3415=CARTESIAN_POINT ( 'NONE',  ( -19.29727288544221864, -21.61407024248036635, 65.60919142207177401 ) ) ;
#3416=FACE_OUTER_BOUND ( 'NONE', #40906, .T. ) ;
#3418=CARTESIAN_POINT ( 'NONE',  ( -13.52677154722849906, -21.15855052895092214, 65.17903009207861942 ) ) ;
#3419=CARTESIAN_POINT ( 'NONE',  ( -10.78978129071826686, -12.42417052737943095, 57.32857332104951098 ) ) ;
#3422=ORIENTED_EDGE ( 'NONE', *, *, #45348, .F. ) ;
#3424=CARTESIAN_POINT ( 'NONE',  ( -22.93742361178516731, -14.77499336254049922, 53.69233794759168887 ) ) ;
#3425=DIRECTION ( 'NONE',  ( -0.003782665018460030538, -0.9999928456970870183, -9.532993539451315208E-09 ) ) ;
#3426=CARTESIAN_POINT ( 'NONE',  ( -23.48344415125163565, -18.41350569598871090, 73.04896097104848707 ) ) ;
#3428=DIRECTION ( 'NONE',  ( -0.7150252244155714809, 0.6990986543038555379, -2.983336731533474947E-17 ) ) ;
#3430=B_SPLINE_CURVE_WITH_KNOTS ( 'NONE', 3,
 ( #37914, #14999, #10603, #44580, #48258, #14496, #10840, #29552, #3446, #25860 ),
 .UNSPECIFIED., .F., .F.,
 ( 4, 2, 2, 2, 4 ),
 ( 0.6272669072877681273, 0.7522669073072665302, 0.8772669073267648221, 1.002266907346263114, 1.127266907365761517 ),
 .UNSPECIFIED. ) ;
#3432=CARTESIAN_POINT ( 'NONE',  ( -14.62687775177895766, -8.392386291203132842, 63.78978840643812021 ) ) ;
#3433=ORIENTED_EDGE ( 'NONE', *, *, #41305, .F. ) ;
#3434=DIRECTION ( 'NONE',  ( 0.9640890753730593232, -0.2655790932026004803, 6.310348465037888425E-08 ) ) ;
#3437=CARTESIAN_POINT ( 'NONE',  ( -12.10599200002982556, -20.02663609087960239, 61.58174067880212021 ) ) ;
#3440=EDGE_CURVE ( 'NONE', #14812, #9213, #20235, .T. ) ;
#3441=DIRECTION ( 'NONE',  ( -0.9345716196833626643, 0.3557750520798445559, 2.412542607589989711E-09 ) ) ;
#3442=CARTESIAN_POINT ( 'NONE',  ( -24.45422819554991278, -14.24171526414585287, 66.06804100909725719 ) ) ;
#3444=CARTESIAN_POINT ( 'NONE',  ( -11.68391713028079515, -10.70246380009546527, 71.12460117624890188 ) ) ;
#3445=EDGE_LOOP ( 'NONE', ( #42413, #47423 ) ) ;
#3446=CARTESIAN_POINT ( 'NONE',  ( -24.49392389907278655, -12.45956950672031738, 73.34951415186112911 ) ) ;
#3448=B_SPLINE_CURVE_WITH_KNOTS ( 'NONE', 1,
 ( #48618, #26461 ),
 .UNSPECIFIED., .F., .F.,
 ( 2, 2 ),
 ( 0.000000000000000000, 1.000000000000000000 ),
 .UNSPECIFIED. ) ;
#3450=VERTEX_POINT ( 'NONE', #23583 ) ;
#3451=CARTESIAN_POINT ( 'NONE',  ( -16.16748626245079379, -22.20318634978239203, 47.99999999999994316 ) ) ;
#3452=CARTESIAN_POINT ( 'NONE',  ( -13.60236376389480384, -20.73382277062339085, 61.80174179654961364 ) ) ;
#3453=CARTESIAN_POINT ( 'NONE',  ( -10.82872618853034119, -17.15944597561106377, 64.81666377234489573 ) ) ;
#3454=VERTEX_POINT ( 'NONE', #16886 ) ;
#3455=CARTESIAN_POINT ( 'NONE',  ( -12.20309502476489882, -20.12380431889209831, 64.98179558605960437 ) ) ;
#3457=CARTESIAN_POINT ( 'NONE',  ( -23.78315586890771982, -10.92762747184599625, 73.48380518477267742 ) ) ;
#3458=ORIENTED_EDGE ( 'NONE', *, *, #39803, .F. ) ;
#3459=LINE ( 'NONE', #28842, #27022 ) ;
#3460=ADVANCED_FACE ( 'NONE', ( #16158 ), #24557, .T. ) ;
#3461=EDGE_CURVE ( 'NONE', #15544, #20590, #26704, .T. ) ;
#3462=DIRECTION ( 'NONE',  ( 0.9904243694481097426, 0.1380563957348939774, 6.973877024228147881E-08 ) ) ;
#3464=CARTESIAN_POINT ( 'NONE',  ( -14.44809130310161471, -8.473323905341505480, 67.25975083863336579 ) ) ;
#3465=CARTESIAN_POINT ( 'NONE',  ( -24.46146587544552276, -14.38248120490118787, 66.46820668217904426 ) ) ;
#3466=CARTESIAN_POINT ( 'NONE',  ( -16.98027701540031487, -7.372437998827603423, 74.11018272214712965 ) ) ;
#3467=CARTESIAN_POINT ( 'NONE',  ( -21.94239094699587511, -20.22099839777041907, 58.91442899523080001 ) ) ;
#3469=CARTESIAN_POINT ( 'NONE',  ( -16.98991614605047218, -22.24663000551990777, 72.35038637723081933 ) ) ;
#3470=CARTESIAN_POINT ( 'NONE',  ( -18.71756812234623979, -7.929749856837892352, 70.67068030594712980 ) ) ;
#3471=CARTESIAN_POINT ( 'NONE',  ( -22.93140599106849464, -9.791786736557840598, 70.15032017024104505 ) ) ;
#3473=ADVANCED_FACE ( 'NONE', ( #12730 ), #31201, .T. ) ;
#3475=CARTESIAN_POINT ( 'NONE',  ( -16.40075914357782949, -21.78757426832101274, 58.17096681542334835 ) ) ;
#3477=VERTEX_POINT ( 'NONE', #39065 ) ;
#3478=ORIENTED_EDGE ( 'NONE', *, *, #38491, .T. ) ;
#3479=CARTESIAN_POINT ( 'NONE',  ( -15.03427660820159772, -21.44211488324610571, 65.12068745241758450 ) ) ;
#3480=CARTESIAN_POINT ( 'NONE',  ( -14.84921296472849583, -8.299983211734243582, 56.95852036331775281 ) ) ;
#3481=ORIENTED_EDGE ( 'NONE', *, *, #10775, .F. ) ;
#3482=CARTESIAN_POINT ( 'NONE',  ( -14.66790711817407278, -21.29843871104708342, 58.18089935161520287 ) ) ;
#3484=CYLINDRICAL_SURFACE ( 'NONE', #46347, 0.1500000000000049349 ) ;
#3485=CARTESIAN_POINT ( 'NONE',  ( -14.09463846823036981, -8.088735815341543400, 47.99999999999994316 ) ) ;
#3486=CARTESIAN_POINT ( 'NONE',  ( -24.38391081516821401, -14.06024225110868464, 73.12271507915593816 ) ) ;
#3487=CARTESIAN_POINT ( 'NONE',  ( -11.41081668282658157, -19.20748171390168579, 71.86498669792840133 ) ) ;
#3488=CARTESIAN_POINT ( 'NONE',  ( -24.45670955521185164, -12.20012290887857098, 53.49999999999995026 ) ) ;
#3490=CARTESIAN_POINT ( 'NONE',  ( -16.71068108117115969, -21.77319771387776726, 68.97944111337483264 ) ) ;
#3491=EDGE_CURVE ( 'NONE', #7972, #33406, #40361, .T. ) ;
#3492=ORIENTED_EDGE ( 'NONE', *, *, #16356, .T. ) ;
#3493=VECTOR ( 'NONE', #31047, 1000.000000000000227 ) ;
#3495=CARTESIAN_POINT ( 'NONE',  ( -11.49054114279358885, -18.52332417048542013, 61.57710786629046140 ) ) ;
#3497=CARTESIAN_POINT ( 'NONE',  ( -24.26595263201846109, -13.32969024507516309, 59.66267925069213618 ) ) ;
#3498=CARTESIAN_POINT ( 'NONE',  ( -12.10131192688100477, -10.18592936015514638, 64.31442259820508411 ) ) ;
#3499=PLANE ( 'NONE',  #36194 ) ;
#3500=CARTESIAN_POINT ( 'NONE',  ( -18.19230087906959170, -22.21957251972233749, 65.38886231616686473 ) ) ;
#3501=VERTEX_POINT ( 'NONE', #16656 ) ;
#3502=VERTEX_POINT ( 'NONE', #34885 ) ;
#3504=ORIENTED_EDGE ( 'NONE', *, *, #33188, .F. ) ;
#3505=CARTESIAN_POINT ( 'NONE',  ( -23.53756504580003650, -19.06719683152477174, 65.96356102755147788 ) ) ;
#3506=CARTESIAN_POINT ( 'NONE',  ( -10.42302287260171312, -13.97751933429587012, 57.73352905910142852 ) ) ;
#3507=CARTESIAN_POINT ( 'NONE',  ( -15.70814931713893792, -7.971180294065260519, 70.60989868072361730 ) ) ;
#3508=CARTESIAN_POINT ( 'NONE',  ( -15.56003183875577278, -7.596127455810019136, 70.71651511567537796 ) ) ;
#3509=ORIENTED_EDGE ( 'NONE', *, *, #24161, .T. ) ;
#3510=B_SPLINE_CURVE_WITH_KNOTS ( 'NONE', 1,
 ( #9490, #39513 ),
 .UNSPECIFIED., .F., .F.,
 ( 2, 2 ),
 ( 0.000000000000000000, 1.000000000000000000 ),
 .UNSPECIFIED. ) ;
#3511=CARTESIAN_POINT ( 'NONE',  ( -23.13029420580725315, -10.01925251292537489, 66.66465368338731423 ) ) ;
#3512=DIRECTION ( 'NONE',  ( -0.1847813031241906379, 0.9827796650397889744, -7.910442904995767160E-08 ) ) ;
#3515=B_SPLINE_CURVE_WITH_KNOTS ( 'NONE', 1,
 ( #11785, #3653 ),
 .UNSPECIFIED., .F., .F.,
 ( 2, 2 ),
 ( 0.000000000000000000, 1.000000000000000000 ),
 .UNSPECIFIED. ) ;
#3516=CARTESIAN_POINT ( 'NONE',  ( -24.35706328060247827, -15.77560928887050373, 69.53307488759497801 ) ) ;
#3517=AXIS2_PLACEMENT_3D ( 'NONE', #32216, #35882, #2163 ) ;
#3518=ORIENTED_EDGE ( 'NONE', *, *, #22100, .T. ) ;
#3519=CARTESIAN_POINT ( 'NONE',  ( -10.98611580423108336, -17.68970554115635352, 67.98233349607527032 ) ) ;
#3521=CARTESIAN_POINT ( 'NONE',  ( -23.24618082141521214, -10.81943526098172548, 59.74636554153219237 ) ) ;
#3523=CARTESIAN_POINT ( 'NONE',  ( -10.73343087151675590, -11.53221169192942597, 71.34506790255136366 ) ) ;
#3524=EDGE_CURVE ( 'NONE', #29406, #22557, #4370, .T. ) ;
#3527=( BOUNDED_CURVE ( )  B_SPLINE_CURVE ( 3, ( #12326, #31772, #5912, #23911 ),
 .UNSPECIFIED., .F., .F. ) 
 B_SPLINE_CURVE_WITH_KNOTS ( ( 4, 4 ),
 ( 0.9074455897393642889, 1.000000000000000000 ),
 .UNSPECIFIED. ) 
 CURVE ( )  GEOMETRIC_REPRESENTATION_ITEM ( )  RATIONAL_B_SPLINE_CURVE ( ( 0.6983129098260905110, 0.7760317562606959818, 0.8765941196519991818, 1.000000000000000000 ) ) 
 REPRESENTATION_ITEM ( '' )  );
#3529=CARTESIAN_POINT ( 'NONE',  ( -23.96395177782270380, -17.30542690858300503, 66.17030669039861834 ) ) ;
#3530=EDGE_LOOP ( 'NONE', ( #38837, #3924, #30214, #38755, #4332 ) ) ;
#3531=CARTESIAN_POINT ( 'NONE',  ( -9.979603215878100286, -14.52052451035377345, 68.04295550616701860 ) ) ;
#3534=CARTESIAN_POINT ( 'NONE',  ( -17.91839958824308709, -21.79173199888728263, 61.87535923606637311 ) ) ;
#3535=EDGE_CURVE ( 'NONE', #5056, #6304, #31687, .T. ) ;
#3540=CYLINDRICAL_SURFACE ( 'NONE', #7843, 2.500000000000001332 ) ;
#3545=CARTESIAN_POINT ( 'NONE',  ( -22.55199052693725648, -10.04362092364324255, 73.76544497664282574 ) ) ;
#3547=( BOUNDED_CURVE ( )  B_SPLINE_CURVE ( 3, ( #14512, #6925, #21945, #7924 ),
 .UNSPECIFIED., .F., .F. ) 
 B_SPLINE_CURVE_WITH_KNOTS ( ( 4, 4 ),
 ( 0.5000000000000000000, 0.9074455897393648440 ),
 .UNSPECIFIED. ) 
 CURVE ( )  GEOMETRIC_REPRESENTATION_ITEM ( )  RATIONAL_B_SPLINE_CURVE ( ( 1.000000000000029310, 0.4567392136813408499, 0.3561768502900130584, 0.6983129098260774104 ) ) 
 REPRESENTATION_ITEM ( '' )  );
#3548=VERTEX_POINT ( 'NONE', #29200 ) ;
#3549=( BOUNDED_CURVE ( )  B_SPLINE_CURVE ( 3, ( #23117, #4388, #38345, #15942 ),
 .UNSPECIFIED., .F., .F. ) 
 B_SPLINE_CURVE_WITH_KNOTS ( ( 4, 4 ),
 ( 0.9074455897393562953, 1.000000000000000000 ),
 .UNSPECIFIED. ) 
 CURVE ( )  GEOMETRIC_REPRESENTATION_ITEM ( )  RATIONAL_B_SPLINE_CURVE ( ( 0.6983129098260636436, 0.7760317562606728892, 0.8765941196519849710, 1.000000000000000000 ) ) 
 REPRESENTATION_ITEM ( '' )  );
#3551=CARTESIAN_POINT ( 'NONE',  ( -23.42858231244642297, -18.40751668988569634, 73.06368185858580944 ) ) ;
#3552=VERTEX_POINT ( 'NONE', #44240 ) ;
#3553=ADVANCED_FACE ( 'NONE', ( #18093 ), #36799, .T. ) ;
#3554=EDGE_LOOP ( 'NONE', ( #39142, #3633, #2694, #16363, #24608 ) ) ;
#3556=LINE ( 'NONE', #18073, #26339 ) ;
#3557=FACE_OUTER_BOUND ( 'NONE', #125, .T. ) ;
#3558=CARTESIAN_POINT ( 'NONE',  ( -24.85470879995478199, -14.26980839996429040, 69.81421776232033949 ) ) ;
#3559=CARTESIAN_POINT ( 'NONE',  ( -13.18362886651731358, -8.683667069837246899, 60.62445550483372614 ) ) ;
#3560=( BOUNDED_SURFACE ( )  B_SPLINE_SURFACE ( 3, 1, ( 
 ( #23002, #37746 ),
 ( #15088, #15327 ),
 ( #3787, #44927 ),
 ( #36347, #22254 ),
 ( #32663, #44672 ),
 ( #30387, #22755 ),
 ( #18797, #11655 ) ),
 .UNSPECIFIED., .T., .F., .F. ) 
 B_SPLINE_SURFACE_WITH_KNOTS ( ( 4, 3, 4 ),
 ( 2, 2 ),
 ( 0.000000000000000000, 0.5000000000000000000, 1.000000000000000000 ),
 ( 0.000000000000000000, 1.000000000000000000 ),
 .UNSPECIFIED. ) 
 GEOMETRIC_REPRESENTATION_ITEM ( )  RATIONAL_B_SPLINE_SURFACE ( (
 ( 1.000000000000000000, 1.000000000000000000),
 ( 0.3333333333333335369, 0.3333333333333330373),
 ( 0.3333333333333335369, 0.3333333333333330373),
 ( 1.000000000000000000, 1.000000000000000000),
 ( 0.3333333333333333703, 0.3333333333333333703),
 ( 0.3333333333333333703, 0.3333333333333333703),
 ( 1.000000000000000000, 1.000000000000000000) ) ) 
 REPRESENTATION_ITEM ( '' )  SURFACE ( )  );
#3562=VERTEX_POINT ( 'NONE', #10493 ) ;
#3568=ORIENTED_EDGE ( 'NONE', *, *, #41520, .F. ) ;
#3569=FACE_OUTER_BOUND ( 'NONE', #12241, .T. ) ;
#3570=CARTESIAN_POINT ( 'NONE',  ( -10.12326195556307695, -13.32541703369907893, 74.86313051124790263 ) ) ;
#3571=EDGE_CURVE ( 'NONE', #29274, #42743, #35490, .T. ) ;
#3572=ORIENTED_EDGE ( 'NONE', *, *, #36367, .T. ) ;
#3574=ORIENTED_EDGE ( 'NONE', *, *, #42354, .F. ) ;
#3575=B_SPLINE_CURVE_WITH_KNOTS ( 'NONE', 3,
 ( #5186, #40588, #17932, #21888, #25347, #2454, #47993, #36888, #7129, #11060 ),
 .UNSPECIFIED., .F., .F.,
 ( 4, 2, 2, 2, 4 ),
 ( 0.6272669072877600227, 0.7522669073072842938, 0.8772669073268084539, 1.002266907346332836, 1.127266907365856996 ),
 .UNSPECIFIED. ) ;
#3576=CARTESIAN_POINT ( 'NONE',  ( -22.27817835350360909, -9.157512823226451104, 59.83675901011532261 ) ) ;
#3577=CARTESIAN_POINT ( 'NONE',  ( -18.15846757210552553, -21.77219414362900807, 68.92587836579659211 ) ) ;
#3578=CARTESIAN_POINT ( 'NONE',  ( -17.42409385541300892, -14.80920654474439324, 54.49999999999995026 ) ) ;
#3579=CARTESIAN_POINT ( 'NONE',  ( -21.53281191010185935, -21.02392799970474258, 72.70259218005269020 ) ) ;
#3581=ORIENTED_EDGE ( 'NONE', *, *, #44647, .F. ) ;
#3582=CARTESIAN_POINT ( 'NONE',  ( -17.98657259272421172, -21.83703102787368167, 62.16063850355641307 ) ) ;
#3583=CARTESIAN_POINT ( 'NONE',  ( -24.18913222791875484, -11.68880796321081661, 59.68224518730406203 ) ) ;
#3585=CARTESIAN_POINT ( 'NONE',  ( -10.09291391017891115, -16.13494330055838333, 68.16263215882007387 ) ) ;
#3586=EDGE_LOOP ( 'NONE', ( #36254, #16648, #13382, #36993, #35217 ) ) ;
#3588=CARTESIAN_POINT ( 'NONE',  ( -17.13698961087219175, -7.364572068746518596, 70.65069232833010915 ) ) ;
#3591=FACE_BOUND ( 'NONE', #14029, .T. ) ;
#3592=B_SPLINE_CURVE_WITH_KNOTS ( 'NONE', 3,
 ( #8653, #1488, #774, #30825, #23185, #30342, #19970, #11604, #41649, #12332 ),
 .UNSPECIFIED., .F., .F.,
 ( 4, 2, 2, 2, 4 ),
 ( 0.000000000000000000, 0.2500000000000000000, 0.5000000000000000000, 0.7500000000000000000, 1.000000000000000000 ),
 .UNSPECIFIED. ) ;
#3593=ORIENTED_EDGE ( 'NONE', *, *, #39131, .F. ) ;
#3594=CARTESIAN_POINT ( 'NONE',  ( -18.31357764725860093, -21.80286926110680668, 68.96514702303620936 ) ) ;
#3596=CARTESIAN_POINT ( 'NONE',  ( -16.95565408849980216, -21.84366694028823730, 72.16543230909471163 ) ) ;
#3597=ADVANCED_FACE ( 'NONE', ( #32871 ), #36555, .T. ) ;
#3599=B_SPLINE_CURVE_WITH_KNOTS ( 'NONE', 1,
 ( #15858, #30906 ),
 .UNSPECIFIED., .F., .F.,
 ( 2, 2 ),
 ( 0.000000000000000000, 1.000000000000000000 ),
 .UNSPECIFIED. ) ;
#3600=CARTESIAN_POINT ( 'NONE',  ( -15.86712703025682103, -7.930203392541469221, 63.55522141739008646 ) ) ;
#3602=CARTESIAN_POINT ( 'NONE',  ( -10.45160174785924312, -14.17496227992596580, 64.61633729656794856 ) ) ;
#3605=CARTESIAN_POINT ( 'NONE',  ( -12.20772386052854408, -10.14112062039578532, 64.02914330961903033 ) ) ;
#3606=CARTESIAN_POINT ( 'NONE',  ( -10.98437665993992596, -18.55522755060170681, 58.00703366852174980 ) ) ;
#3608=EDGE_LOOP ( 'NONE', ( #25055, #15354, #3279, #37136, #40266 ) ) ;
#3609=CARTESIAN_POINT ( 'NONE',  ( -21.59804090337381410, -20.98026344205569771, 72.70941702861115630 ) ) ;
#3611=CARTESIAN_POINT ( 'NONE',  ( -18.35379419424621972, -22.20097654771712570, 69.01525906027519852 ) ) ;
#3613=ORIENTED_EDGE ( 'NONE', *, *, #16880, .T. ) ;
#3614=ORIENTED_EDGE ( 'NONE', *, *, #43918, .F. ) ;
#3615=CARTESIAN_POINT ( 'NONE',  ( -14.92764478915313653, -21.34891159457319532, 61.63600440564275829 ) ) ;
#3616=CARTESIAN_POINT ( 'NONE',  ( -20.57278596605185683, -8.057205637650621810, 66.89608763938375091 ) ) ;
#3617=CARTESIAN_POINT ( 'NONE',  ( -19.36518065869528726, -8.031383756764064685, 59.97565108339750850 ) ) ;
#3618=CARTESIAN_POINT ( 'NONE',  ( -20.85039448910245241, -8.638677133180788559, 63.45554403117525055 ) ) ;
#3620=LINE ( 'NONE', #23082, #37748 ) ;
#3621=CARTESIAN_POINT ( 'NONE',  ( -14.43441977789444763, -8.421195553735145722, 71.14446303425738449 ) ) ;
#3622=CARTESIAN_POINT ( 'NONE',  ( -14.74088078129247137, -21.75928990931933527, 61.74326270667029348 ) ) ;
#3624=ORIENTED_EDGE ( 'NONE', *, *, #27377, .T. ) ;
#3625=B_SPLINE_CURVE_WITH_KNOTS ( 'NONE', 3,
 ( #16092, #8255, #14435, #27439, #34574, #33170, #4081, #46156, #30183, #45201 ),
 .UNSPECIFIED., .F., .F.,
 ( 4, 2, 2, 2, 4 ),
 ( 0.000000000000000000, 0.2500000000000000000, 0.5000000000000000000, 0.7500000000000000000, 1.000000000000000000 ),
 .UNSPECIFIED. ) ;
#3626=CARTESIAN_POINT ( 'NONE',  ( -16.32575768948312600, -7.844986739114469643, 60.21500614002425777 ) ) ;
#3627=DIRECTION ( 'NONE',  ( 0.2393306345705741855, 0.3777841279832264143, 0.8944271909999157444 ) ) ;
#3628=CARTESIAN_POINT ( 'NONE',  ( -14.90981263331598328, -21.39562362703504306, 61.93600440604522817 ) ) ;
#3629=PLANE ( 'NONE',  #44132 ) ;
#3633=ORIENTED_EDGE ( 'NONE', *, *, #20792, .T. ) ;
#3634=CARTESIAN_POINT ( 'NONE',  ( -24.35164231460261064, -15.81449975624289728, 69.83307533819942137 ) ) ;
#3635=CARTESIAN_POINT ( 'NONE',  ( -13.35550429318260512, -8.568184490765622385, 57.15463139269148485 ) ) ;
#3636=LINE ( 'NONE', #14938, #15779 ) ;
#3637=( BOUNDED_SURFACE ( )  B_SPLINE_SURFACE ( 3, 1, ( 
 ( #23451, #38446 ),
 ( #34763, #47311 ),
 ( #43865, #16521 ),
 ( #13297, #20717 ),
 ( #13545, #24662 ),
 ( #31557, #1763 ),
 ( #6178, #2482 ) ),
 .UNSPECIFIED., .T., .F., .F. ) 
 B_SPLINE_SURFACE_WITH_KNOTS ( ( 4, 3, 4 ),
 ( 2, 2 ),
 ( 0.000000000000000000, 0.5000000000000000000, 1.000000000000000000 ),
 ( 0.000000000000000000, 1.000000000000000000 ),
 .UNSPECIFIED. ) 
 GEOMETRIC_REPRESENTATION_ITEM ( )  RATIONAL_B_SPLINE_SURFACE ( (
 ( 1.000000000000000000, 1.000000000000000000),
 ( 0.3333333333333335369, 0.3333333333333330373),
 ( 0.3333333333333335369, 0.3333333333333330373),
 ( 1.000000000000000000, 1.000000000000000000),
 ( 0.3333333333333333703, 0.3333333333333333703),
 ( 0.3333333333333333703, 0.3333333333333333703),
 ( 1.000000000000000000, 1.000000000000000000) ) ) 
 REPRESENTATION_ITEM ( '' )  SURFACE ( )  );
#3639=ORIENTED_EDGE ( 'NONE', *, *, #23925, .T. ) ;
#3640=CARTESIAN_POINT ( 'NONE',  ( -20.38226146016681994, -7.971588334861294811, 70.36604906519886526 ) ) ;
#3642=CARTESIAN_POINT ( 'NONE',  ( -13.41327373486474883, -20.54621981236622830, 58.04650078084816300 ) ) ;
#3643=ORIENTED_EDGE ( 'NONE', *, *, #27487, .F. ) ;
#3644=LINE ( 'NONE', #26542, #30478 ) ;
#3645=CARTESIAN_POINT ( 'NONE',  ( -10.03804196927290882, -15.78895246822652076, 64.69426957934942379 ) ) ;
#3646=PLANE ( 'NONE',  #15794 ) ;
#3648=PLANE ( 'NONE',  #35390 ) ;
#3651=CARTESIAN_POINT ( 'NONE',  ( -12.36756753426621813, -9.896138138887707214, 57.37463480816234096 ) ) ;
#3653=CARTESIAN_POINT ( 'NONE',  ( -24.77723895724858494, -16.00713575449774595, 66.24820309305337673 ) ) ;
#3654=DIRECTION ( 'NONE',  ( -0.9990515194385544140, -0.04354378839186318073, 1.103613758316041049E-08 ) ) ;
#3655=EDGE_CURVE ( 'NONE', #44694, #12297, #28439, .T. ) ;
#3656=ORIENTED_EDGE ( 'NONE', *, *, #33432, .T. ) ;
#3657=CARTESIAN_POINT ( 'NONE',  ( -22.06352374043166265, -8.980015506435984562, 63.37649162950052784 ) ) ;
#3658=CARTESIAN_POINT ( 'NONE',  ( -16.41802950720715160, -7.880257431743621588, 60.38955644688196855 ) ) ;
#3659=CARTESIAN_POINT ( 'NONE',  ( -24.32752796592761158, -15.96791130369872391, 66.06324927019940674 ) ) ;
#3660=ORIENTED_EDGE ( 'NONE', *, *, #4163, .T. ) ;
#3664=ADVANCED_FACE ( 'NONE', ( #25024 ), #2126, .T. ) ;
#3665=CARTESIAN_POINT ( 'NONE',  ( -20.95545100651803594, -20.91135505560678354, 65.59926067308570907 ) ) ;
#3668=ORIENTED_EDGE ( 'NONE', *, *, #35060, .T. ) ;
#3669=CARTESIAN_POINT ( 'NONE',  ( -22.30326020397728115, -9.709333660337318150, 73.63728338005337548 ) ) ;
#3670=FACE_OUTER_BOUND ( 'NONE', #8068, .T. ) ;
#3671=CARTESIAN_POINT ( 'NONE',  ( -23.32045150837215175, -18.68837265512984303, 62.50973769122266788 ) ) ;
#3673=EDGE_CURVE ( 'NONE', #10295, #4829, #43506, .T. ) ;
#3674=AXIS2_PLACEMENT_3D ( 'NONE', #39586, #35875, #24592 ) ;
#3676=CARTESIAN_POINT ( 'NONE',  ( -20.13271805750754595, -8.299978134201072777, 70.53628287813307907 ) ) ;
#3677=CARTESIAN_POINT ( 'NONE',  ( -24.10584550580110985, -12.56049697540380095, 73.54225570139644219 ) ) ;
#3678=CARTESIAN_POINT ( 'NONE',  ( -24.29205067375949056, -17.69794899492463713, 66.13012485676826202 ) ) ;
#3679=CARTESIAN_POINT ( 'NONE',  ( -14.69865266434688955, -8.361098232125304008, 63.80595424419050232 ) ) ;
#3680=EDGE_LOOP ( 'NONE', ( #23347, #40733 ) ) ;
#3681=B_SPLINE_CURVE_WITH_KNOTS ( 'NONE', 3,
 ( #41374, #34723, #3713, #18716, #4689, #30561, #34222, #7669, #41880, #11346 ),
 .UNSPECIFIED., .F., .F.,
 ( 4, 2, 2, 2, 4 ),
 ( 0.000000000000000000, 0.2500000000000000000, 0.5000000000000000000, 0.7500000000000000000, 1.000000000000000000 ),
 .UNSPECIFIED. ) ;
#3682=FACE_OUTER_BOUND ( 'NONE', #6869, .T. ) ;
#3684=CYLINDRICAL_SURFACE ( 'NONE', #7549, 0.1500000000000005218 ) ;
#3685=CARTESIAN_POINT ( 'NONE',  ( -14.66790711817407278, -21.29843871104708342, 58.18089935161520287 ) ) ;
#3687=EDGE_CURVE ( 'NONE', #19987, #31666, #40285, .T. ) ;
#3688=ORIENTED_EDGE ( 'NONE', *, *, #19369, .F. ) ;
#3689=EDGE_CURVE ( 'NONE', #18786, #26541, #33115, .T. ) ;
#3690=B_SPLINE_CURVE_WITH_KNOTS ( 'NONE', 3,
 ( #42909, #31822, #35263, #47339, #20980, #35982, #28125, #2510, #28613, #39931 ),
 .UNSPECIFIED., .F., .F.,
 ( 4, 2, 2, 2, 4 ),
 ( 0.000000000000000000, 0.2500000000000000000, 0.5000000000000000000, 0.7500000000000000000, 1.000000000000000000 ),
 .UNSPECIFIED. ) ;
#3691=ORIENTED_EDGE ( 'NONE', *, *, #20048, .F. ) ;
#3693=FACE_OUTER_BOUND ( 'NONE', #45163, .T. ) ;
#3694=CARTESIAN_POINT ( 'NONE',  ( -10.63166622156590790, -13.11537716526513186, 71.22445270976328402 ) ) ;
#3695=B_SPLINE_CURVE_WITH_KNOTS ( 'NONE', 3,
 ( #2707, #5704, #14007, #16750, #13057, #47052, #28088, #13292, #43373, #24888 ),
 .UNSPECIFIED., .F., .F.,
 ( 4, 2, 2, 2, 4 ),
 ( 0.000000000000000000, 0.2500000000000000000, 0.5000000000000000000, 0.7500000000000000000, 1.000000000000000000 ),
 .UNSPECIFIED. ) ;
#3697=CARTESIAN_POINT ( 'NONE',  ( -10.18562964238619806, -13.04598147208188053, 71.38641367950162930 ) ) ;
#3699=( BOUNDED_SURFACE ( )  B_SPLINE_SURFACE ( 3, 1, ( 
 ( #35061, #1324 ),
 ( #45202, #26471 ),
 ( #45442, #41486 ),
 ( #7777, #22795 ),
 ( #37789, #378 ),
 ( #26723, #15361 ),
 ( #30427, #23039 ) ),
 .UNSPECIFIED., .T., .F., .F. ) 
 B_SPLINE_SURFACE_WITH_KNOTS ( ( 4, 3, 4 ),
 ( 2, 2 ),
 ( 0.000000000000000000, 0.5000000000000000000, 1.000000000000000000 ),
 ( 0.000000000000000000, 1.000000000000000000 ),
 .UNSPECIFIED. ) 
 GEOMETRIC_REPRESENTATION_ITEM ( )  RATIONAL_B_SPLINE_SURFACE ( (
 ( 1.000000000000000000, 1.000000000000000000),
 ( 0.3333333333333335369, 0.3333333333333330373),
 ( 0.3333333333333335369, 0.3333333333333330373),
 ( 1.000000000000000000, 1.000000000000000000),
 ( 0.3333333333333333703, 0.3333333333333333703),
 ( 0.3333333333333333703, 0.3333333333333333703),
 ( 1.000000000000000000, 1.000000000000000000) ) ) 
 REPRESENTATION_ITEM ( '' )  SURFACE ( )  );
#3702=CARTESIAN_POINT ( 'NONE',  ( -14.36817892824948650, -8.455618309860652104, 67.54503025475185041 ) ) ;
#3703=ORIENTED_EDGE ( 'NONE', *, *, #8514, .T. ) ;
#3706=CARTESIAN_POINT ( 'NONE',  ( -10.99582063857411995, -11.91441743271276366, 74.55840195587596497 ) ) ;
#3707=CARTESIAN_POINT ( 'NONE',  ( -14.05440619237976385, -8.616608212056021898, 74.49954658714564459 ) ) ;
#3709=B_SPLINE_CURVE_WITH_KNOTS ( 'NONE', 3,
 ( #35428, #741, #15739, #13015, #44468, #9349, #44716, #18334, #48148, #48381 ),
 .UNSPECIFIED., .F., .F.,
 ( 4, 2, 2, 2, 4 ),
 ( 0.000000000000000000, 0.2500000000000000000, 0.5000000000000000000, 0.7500000000000000000, 1.000000000000000000 ),
 .UNSPECIFIED. ) ;
#3710=CARTESIAN_POINT ( 'NONE',  ( -12.25319814409069252, -20.17255476956438542, 64.91028984507975963 ) ) ;
#3713=CARTESIAN_POINT ( 'NONE',  ( -20.45830450918359489, -8.500926063925801301, 63.32623952627614017 ) ) ;
#3714=EDGE_LOOP ( 'NONE', ( #37591, #22018, #30444, #11654, #6115 ) ) ;
#3719=CARTESIAN_POINT ( 'NONE',  ( -24.29299122354570883, -17.69571185755203757, 62.58705726155704951 ) ) ;
#3722=ORIENTED_EDGE ( 'NONE', *, *, #11329, .F. ) ;
#3723=CARTESIAN_POINT ( 'NONE',  ( -10.43906310151734651, -14.34979072177226911, 64.68803843020796762 ) ) ;
#3724=CARTESIAN_POINT ( 'NONE',  ( -15.68503317936312236, -7.977064329016500643, 70.60989839961001735 ) ) ;
#3725=CARTESIAN_POINT ( 'NONE',  ( -18.11396590982544197, -21.77512906430638040, 65.64532159443497505 ) ) ;
#3726=CARTESIAN_POINT ( 'NONE',  ( -10.70566809389435647, -16.94585225683366048, 57.68760548748759476 ) ) ;
#3729=CARTESIAN_POINT ( 'NONE',  ( -13.12613380977788147, -20.89454282643029259, 58.16154686733092660 ) ) ;
#3730=ORIENTED_EDGE ( 'NONE', *, *, #43738, .T. ) ;
#3731=ORIENTED_EDGE ( 'NONE', *, *, #8386, .F. ) ;
#3732=CARTESIAN_POINT ( 'NONE',  ( -21.68499379980493558, -9.192514338196573931, 66.96149992326067490 ) ) ;
#3734=CARTESIAN_POINT ( 'NONE',  ( -15.37275756075460365, -7.647176670682967803, 74.17962025520618852 ) ) ;
#3735=CARTESIAN_POINT ( 'NONE',  ( -21.02603828283602283, -21.33060232236718434, 62.31482603073411042 ) ) ;
#3736=CARTESIAN_POINT ( 'NONE',  ( -15.30563816890515660, -21.53343246974097625, 68.87592909656478923 ) ) ;
#3737=CARTESIAN_POINT ( 'NONE',  ( -11.59700437785899574, -18.68821983113924645, 64.74707024157237356 ) ) ;
#3738=FACE_OUTER_BOUND ( 'NONE', #37025, .T. ) ;
#3739=FACE_BOUND ( 'NONE', #25058, .T. ) ;
#3740=CARTESIAN_POINT ( 'NONE',  ( -11.42008220035761923, -19.21999808210960836, 71.88024208098950396 ) ) ;
#3741=DIRECTION ( 'NONE',  ( 0.7029450532227031756, 0.7112441579020041260, -7.405715380709556396E-09 ) ) ;
#3743=EDGE_LOOP ( 'NONE', ( #21317, #36870, #18935, #3927, #36844 ) ) ;
#3744=CARTESIAN_POINT ( 'NONE',  ( -17.52853272358826686, -7.759682304905023642, 63.83584969886392457 ) ) ;
#3747=AXIS2_PLACEMENT_3D ( 'NONE', #36224, #47336, #10618 ) ;
#3749=CARTESIAN_POINT ( 'NONE',  ( -24.20371252810814866, -12.87440185077122834, 66.58774614429587757 ) ) ;
#3750=CARTESIAN_POINT ( 'NONE',  ( -14.78766009005058812, -21.34800739930362568, 58.45145834864037937 ) ) ;
#3751=CARTESIAN_POINT ( 'NONE',  ( -18.18338144371267617, -21.81849904615365432, 65.63060065626805795 ) ) ;
#3752=VECTOR ( 'NONE', #25357, 1000.000000000000114 ) ;
#3754=ORIENTED_EDGE ( 'NONE', *, *, #47592, .T. ) ;
#3755=ORIENTED_EDGE ( 'NONE', *, *, #3524, .F. ) ;
#3757=EDGE_LOOP ( 'NONE', ( #22338, #9402, #2962, #36549 ) ) ;
#3758=ADVANCED_FACE ( 'NONE', ( #14620 ), #8260, .T. ) ;
#3759=EDGE_CURVE ( 'NONE', #32800, #37610, #44835, .T. ) ;
#3760=CARTESIAN_POINT ( 'NONE',  ( -17.36874312174564139, -7.359362613910461093, 67.12701303326514335 ) ) ;
#3761=B_SPLINE_CURVE_WITH_KNOTS ( 'NONE', 1,
 ( #15404, #45249 ),
 .UNSPECIFIED., .F., .F.,
 ( 2, 2 ),
 ( 0.000000000000000000, 1.000000000000000000 ),
 .UNSPECIFIED. ) ;
#3763=B_SPLINE_CURVE_WITH_KNOTS ( 'NONE', 3,
 ( #3981, #45835, #12090, #18993, #33996, #27103, #8397, #38417, #4703, #35933 ),
 .UNSPECIFIED., .F., .F.,
 ( 4, 2, 2, 2, 4 ),
 ( 0.000000000000000000, 0.2500000000000000000, 0.5000000000000000000, 0.7500000000000000000, 1.000000000000000000 ),
 .UNSPECIFIED. ) ;
#3765=CARTESIAN_POINT ( 'NONE',  ( -18.12574864353739201, -7.786197982121914052, 60.22493603095571046 ) ) ;
#3767=CARTESIAN_POINT ( 'NONE',  ( -20.49170831689750472, -8.461258797198503601, 63.59649424907593129 ) ) ;
#3768=VECTOR ( 'NONE', #41992, 1000.000000000000114 ) ;
#3771=CARTESIAN_POINT ( 'NONE',  ( -14.90981300391231024, -21.39562377109201208, 61.63600440604547970 ) ) ;
#3772=CARTESIAN_POINT ( 'NONE',  ( -10.37141135217074961, -14.92372438906622811, 71.53602713937311819 ) ) ;
#3775=ORIENTED_EDGE ( 'NONE', *, *, #30141, .T. ) ;
#3776=CARTESIAN_POINT ( 'NONE',  ( -19.50844099596679371, -21.96177777289817357, 62.11008350414853396 ) ) ;
#3777=CARTESIAN_POINT ( 'NONE',  ( -15.48424059001683339, -21.53504990492328375, 72.04575460974366763 ) ) ;
#3778=CARTESIAN_POINT ( 'NONE',  ( -9.979977042000861331, -14.51194761097949382, 67.96461827199280492 ) ) ;
#3779=ORIENTED_EDGE ( 'NONE', *, *, #21152, .T. ) ;
#3780=CARTESIAN_POINT ( 'NONE',  ( -10.68551981713787136, -12.73596763222149164, 64.28308208171728211 ) ) ;
#3782=CARTESIAN_POINT ( 'NONE',  ( -24.34138212120913991, -16.17068457824029792, 62.74328676669021831 ) ) ;
#3784=CARTESIAN_POINT ( 'NONE',  ( -24.68345461824787890, -13.13130818398968103, 59.47612521039077649 ) ) ;
#3785=CARTESIAN_POINT ( 'NONE',  ( -10.93232766038821424, -17.55941949638709687, 68.38249893951126523 ) ) ;
#3786=ORIENTED_EDGE ( 'NONE', *, *, #13151, .T. ) ;
#3787=CARTESIAN_POINT ( 'NONE',  ( -24.34586551078590233, -16.16342498662110572, 59.00843562520186936 ) ) ;
#3788=DIRECTION ( 'NONE',  ( 0.9997277805376392212, -0.02333162706040292633, -9.101776391673708383E-09 ) ) ;
#3789=VECTOR ( 'NONE', #2751, 999.9999999999998863 ) ;
#3791=CARTESIAN_POINT ( 'NONE',  ( -19.45281838860202228, -9.697037067072807659, 53.49999999999995026 ) ) ;
#3792=CARTESIAN_POINT ( 'NONE',  ( -23.51785832295892931, -11.36449550514380036, 69.89210750611785272 ) ) ;
#3793=CARTESIAN_POINT ( 'NONE',  ( -10.49291259435924673, -15.78913940232298785, 64.50771630042218874 ) ) ;
#3795=EDGE_LOOP ( 'NONE', ( #28513, #48162, #21774, #2345, #32422 ) ) ;
#3796=EDGE_CURVE ( 'NONE', #18177, #21199, #14871, .T. ) ;
#3797=DIRECTION ( 'NONE',  ( -0.3688590060343601151, 0.9294853595766551235, -9.484706316669577488E-17 ) ) ;
#3798=CARTESIAN_POINT ( 'NONE',  ( -24.69856829750257177, -13.20119948815759159, 59.40621968628075678 ) ) ;
#3799=ORIENTED_EDGE ( 'NONE', *, *, #1828, .F. ) ;
#3802=DIRECTION ( 'NONE',  ( 3.549360974554993999E-17, -6.371834667797928663E-18, -1.000000000000000000 ) ) ;
#3804=CARTESIAN_POINT ( 'NONE',  ( -18.10946867608448940, -21.82882885753907942, 69.23003497527133732 ) ) ;
#3805=CARTESIAN_POINT ( 'NONE',  ( -18.41353416428395917, -22.19337852133874023, 68.95368170273926012 ) ) ;
#3808=AXIS2_PLACEMENT_3D ( 'NONE', #10988, #18354, #10507 ) ;
#3809=CARTESIAN_POINT ( 'NONE',  ( -12.83571665415373708, -8.939642480694315552, 67.51796240912459268 ) ) ;
#3811=CARTESIAN_POINT ( 'NONE',  ( -24.79781836340079337, -15.87314503134675014, 69.64812095075065201 ) ) ;
#3812=CARTESIAN_POINT ( 'NONE',  ( -18.92057448382017881, -7.919863665830077615, 67.20071783788056052 ) ) ;
#3816=ORIENTED_EDGE ( 'NONE', *, *, #47032, .T. ) ;
#3819=EDGE_CURVE ( 'NONE', #18099, #25345, #36597, .T. ) ;
#3820=ADVANCED_FACE ( 'NONE', ( #30674 ), #45697, .T. ) ;
#3821=CARTESIAN_POINT ( 'NONE',  ( -23.41977899678227004, -11.19648470850049904, 73.36193302072521760 ) ) ;
#3825=EDGE_CURVE ( 'NONE', #41834, #27306, #21987, .T. ) ;
#3827=ORIENTED_EDGE ( 'NONE', *, *, #29669, .T. ) ;
#3829=EDGE_CURVE ( 'NONE', #8929, #31196, #38989, .T. ) ;
#3830=CARTESIAN_POINT ( 'NONE',  ( -12.44869033171645611, -9.885248809711741913, 57.38935532200543577 ) ) ;
#3832=CARTESIAN_POINT ( 'NONE',  ( -24.43235039625237803, -15.64544980915412431, 66.21891754810816622 ) ) ;
#3833=( BOUNDED_SURFACE ( )  B_SPLINE_SURFACE ( 3, 1, ( 
 ( #30779, #19429 ),
 ( #38369, #34435 ),
 ( #729, #15722 ),
 ( #45800, #34692 ),
 ( #26099, #16693 ),
 ( #42593, #31008 ),
 ( #46028, #24350 ) ),
 .UNSPECIFIED., .T., .F., .F. ) 
 B_SPLINE_SURFACE_WITH_KNOTS ( ( 4, 3, 4 ),
 ( 2, 2 ),
 ( 0.000000000000000000, 0.5000000000000000000, 1.000000000000000000 ),
 ( 0.000000000000000000, 1.000000000000000000 ),
 .UNSPECIFIED. ) 
 GEOMETRIC_REPRESENTATION_ITEM ( )  RATIONAL_B_SPLINE_SURFACE ( (
 ( 1.000000000000000000, 1.000000000000000000),
 ( 0.3333333333333335369, 0.3333333333333330373),
 ( 0.3333333333333335369, 0.3333333333333330373),
 ( 1.000000000000000000, 1.000000000000000000),
 ( 0.3333333333333333703, 0.3333333333333333703),
 ( 0.3333333333333333703, 0.3333333333333333703),
 ( 1.000000000000000000, 1.000000000000000000) ) ) 
 REPRESENTATION_ITEM ( '' )  SURFACE ( )  );
#3834=ORIENTED_EDGE ( 'NONE', *, *, #35709, .T. ) ;
#3835=B_SPLINE_CURVE_WITH_KNOTS ( 'NONE', 3,
 ( #45782, #19408, #7865, #30271, #18665, #29768, #15211, #22886, #7373, #4392 ),
 .UNSPECIFIED., .F., .F.,
 ( 4, 2, 2, 2, 4 ),
 ( 0.000000000000000000, 0.2500000000000000000, 0.5000000000000000000, 0.7500000000000000000, 1.000000000000000000 ),
 .UNSPECIFIED. ) ;
#3836=ORIENTED_EDGE ( 'NONE', *, *, #34330, .F. ) ;
#3837=DIRECTION ( 'NONE',  ( -8.719004481856245202E-07, 8.513143972389065227E-07, -0.9999999999992574828 ) ) ;
#3838=CARTESIAN_POINT ( 'NONE',  ( -18.30727046116018286, -21.75326869042403288, 69.11514702556002021 ) ) ;
#3839=CARTESIAN_POINT ( 'NONE',  ( -24.42163167104895294, -17.36632341347029751, 69.59056710591525530 ) ) ;
#3840=CARTESIAN_POINT ( 'NONE',  ( -16.92014803599858652, -22.24222107688192196, 72.42189142509964483 ) ) ;
#3841=ADVANCED_FACE ( 'NONE', ( #37532 ), #45208, .T. ) ;
#3845=CARTESIAN_POINT ( 'NONE',  ( -15.38656303155622673, -21.97522069389735222, 72.23849606682514946 ) ) ;
#3846=AXIS2_PLACEMENT_3D ( 'NONE', #37091, #10528, #33148 ) ;
#3847=CARTESIAN_POINT ( 'NONE',  ( -12.84690951644825851, -8.931012861620404308, 67.56438176077992352 ) ) ;
#3848=CARTESIAN_POINT ( 'NONE',  ( -19.80301260837064703, -21.44571507605098404, 69.23482476707422961 ) ) ;
#3849=ORIENTED_EDGE ( 'NONE', *, *, #40961, .F. ) ;
#3850=CARTESIAN_POINT ( 'NONE',  ( -19.50112608350124788, -21.96394757316516433, 62.11786765711682534 ) ) ;
#3852=( BOUNDED_CURVE ( )  B_SPLINE_CURVE ( 3, ( #17480, #17710, #10585, #32279 ),
 .UNSPECIFIED., .F., .F. ) 
 B_SPLINE_CURVE_WITH_KNOTS ( ( 4, 4 ),
 ( 0.5000000000000000000, 0.9074455897393656212 ),
 .UNSPECIFIED. ) 
 CURVE ( )  GEOMETRIC_REPRESENTATION_ITEM ( )  RATIONAL_B_SPLINE_CURVE ( ( 0.9999999999999958922, 0.4567392136813264170, 0.3561768502900310995, 0.6983129098261053880 ) ) 
 REPRESENTATION_ITEM ( '' )  );
#3855=LINE ( 'NONE', #3350, #37224 ) ;
#3856=FACE_BOUND ( 'NONE', #24866, .T. ) ;
#3858=CARTESIAN_POINT ( 'NONE',  ( -13.13317054870913125, -20.89946229583447135, 58.23988401356517386 ) ) ;
#3862=ORIENTED_EDGE ( 'NONE', *, *, #39003, .T. ) ;
#3863=CARTESIAN_POINT ( 'NONE',  ( -10.13258914451759019, -16.33817228489381179, 71.63245656337019796 ) ) ;
#3865=VERTEX_POINT ( 'NONE', #34826 ) ;
#3866=DIRECTION ( 'NONE',  ( 0.7150252244155669290, -0.6990986543038600898, 2.983336731533460772E-17 ) ) ;
#3867=CARTESIAN_POINT ( 'NONE',  ( -10.99273270719357498, -18.56964325624270273, 57.99988733456820000 ) ) ;
#3868=VERTEX_POINT ( 'NONE', #45925 ) ;
#3869=CARTESIAN_POINT ( 'NONE',  ( -21.62450594022013206, -20.48119921038467695, 72.68013252948732372 ) ) ;
#3870=( BOUNDED_CURVE ( )  B_SPLINE_CURVE ( 3, ( #33231, #14275, #41138, #21465 ),
 .UNSPECIFIED., .F., .F. ) 
 B_SPLINE_CURVE_WITH_KNOTS ( ( 4, 4 ),
 ( 0.9074455897393656212, 1.000000000000000000 ),
 .UNSPECIFIED. ) 
 CURVE ( )  GEOMETRIC_REPRESENTATION_ITEM ( )  RATIONAL_B_SPLINE_CURVE ( ( 0.6983129098261039447, 0.7760317562607076392, 0.8765941196520062872, 1.000000000000000000 ) ) 
 REPRESENTATION_ITEM ( '' )  );
#3873=VERTEX_POINT ( 'NONE', #23523 ) ;
#3874=ORIENTED_EDGE ( 'NONE', *, *, #39353, .T. ) ;
#3875=CARTESIAN_POINT ( 'NONE',  ( -15.32518410995109193, -21.95751795911967008, 72.16080160551160816 ) ) ;
#3876=CARTESIAN_POINT ( 'NONE',  ( -20.43185948505062299, -8.432683554863363184, 66.79576150497511833 ) ) ;
#3877=CARTESIAN_POINT ( 'NONE',  ( -21.15336504700141163, -20.73310185707507713, 69.05450185101547333 ) ) ;
#3878=CARTESIAN_POINT ( 'NONE',  ( -10.03993391926675116, -13.82001047774868496, 57.62637814497484356 ) ) ;
#3879=ADVANCED_FACE ( 'NONE', ( #1100 ), #13301, .T. ) ;
#3881=CARTESIAN_POINT ( 'NONE',  ( -14.16804786125913118, -8.612086647834459541, 74.48338047236791226 ) ) ;
#3884=EDGE_LOOP ( 'NONE', ( #33436, #19522, #7565, #28926, #14538 ) ) ;
#3885=CARTESIAN_POINT ( 'NONE',  ( -16.16063142123006813, -7.467037929575190525, 60.38523757159160965 ) ) ;
#3887=CARTESIAN_POINT ( 'NONE',  ( -13.62460154206902807, -8.321601493802987193, 53.76227901944321985 ) ) ;
#3888=CARTESIAN_POINT ( 'NONE',  ( -10.90759844528708911, -17.49952021360972765, 68.24721944423116327 ) ) ;
#3889=CARTESIAN_POINT ( 'NONE',  ( -21.56413130975026959, -4.978830828776663608, 54.49999999999995026 ) ) ;
#3893=AXIS2_PLACEMENT_3D ( 'NONE', #2047, #25194, #32093 ) ;
#3896=CARTESIAN_POINT ( 'NONE',  ( -10.63004074901718532, -12.92571453866564823, 67.75304464120749515 ) ) ;
#3897=CARTESIAN_POINT ( 'NONE',  ( -12.45907596150898300, -19.82553632194446180, 58.08249573729000304 ) ) ;
#3898=EDGE_CURVE ( 'NONE', #2764, #21586, #14880, .T. ) ;
#3899=CARTESIAN_POINT ( 'NONE',  ( -10.42302287260171312, -13.97751933429587012, 57.73352905910142852 ) ) ;
#3901=EDGE_CURVE ( 'NONE', #16737, #11137, #43713, .T. ) ;
#3902=ORIENTED_EDGE ( 'NONE', *, *, #13741, .F. ) ;
#3903=CARTESIAN_POINT ( 'NONE',  ( -20.38927765283500904, -7.974583868351674099, 70.37383423426267370 ) ) ;
#3904=B_SPLINE_CURVE_WITH_KNOTS ( 'NONE', 3,
 ( #17533, #43907, #10160, #33257, #29590, #25181, #40428, #29351, #44621, #6471 ),
 .UNSPECIFIED., .F., .F.,
 ( 4, 2, 2, 2, 4 ),
 ( 0.000000000000000000, 0.2500000000000000000, 0.5000000000000000000, 0.7500000000000000000, 1.000000000000000000 ),
 .UNSPECIFIED. ) ;
#3905=CARTESIAN_POINT ( 'NONE',  ( -14.56495137627929637, -8.364837042462607286, 64.08419083274510797 ) ) ;
#3907=ADVANCED_FACE ( 'NONE', ( #39258 ), #38492, .T. ) ;
#3908=CARTESIAN_POINT ( 'NONE',  ( -19.30128557755455532, -21.60500301973953086, 58.81035253397666196 ) ) ;
#3911=CARTESIAN_POINT ( 'NONE',  ( -24.43362360091611052, -14.05489060867666495, 73.42271507725004653 ) ) ;
#3914=CARTESIAN_POINT ( 'NONE',  ( -24.87140955007623333, -14.60726545267721121, 62.90570658404245563 ) ) ;
#3915=EDGE_LOOP ( 'NONE', ( #39075, #32708, #30699, #40497, #32037 ) ) ;
#3916=CARTESIAN_POINT ( 'NONE',  ( -13.28240554951661245, -9.100331501070346718, 67.79431631125400770 ) ) ;
#3917=CARTESIAN_POINT ( 'NONE',  ( -24.18470913683765389, -12.80901137141652768, 69.78715111652664405 ) ) ;
#3918=PLANE ( 'NONE',  #11620 ) ;
#3920=VERTEX_POINT ( 'NONE', #23279 ) ;
#3922=DIRECTION ( 'NONE',  ( 3.549360974554993999E-17, -6.371834667797928663E-18, -1.000000000000000000 ) ) ;
#3923=CARTESIAN_POINT ( 'NONE',  ( -19.80301260837064703, -21.44571507605098404, 69.23482476707422961 ) ) ;
#3924=ORIENTED_EDGE ( 'NONE', *, *, #12671, .F. ) ;
#3925=CARTESIAN_POINT ( 'NONE',  ( -12.50776634899986384, -20.40684016789016297, 71.92158251742569064 ) ) ;
#3926=CARTESIAN_POINT ( 'NONE',  ( -23.56138519289638822, -11.33989039198723248, 69.89210750373884196 ) ) ;
#3927=ORIENTED_EDGE ( 'NONE', *, *, #6598, .T. ) ;
#3928=EDGE_LOOP ( 'NONE', ( #9167, #36625, #48192, #24682, #2797, #15200, #46207, #43881, #1183, #45781, #28563, #23263 ) ) ;
#3929=FACE_OUTER_BOUND ( 'NONE', #11304, .T. ) ;
#3930=CARTESIAN_POINT ( 'NONE',  ( -19.24190894175819366, -7.584296403803404196, 63.54593838833191910 ) ) ;
#3931=DIRECTION ( 'NONE',  ( 0.8788484374452892878, -0.3260506722428099247, -0.3483050145059431446 ) ) ;
#3934=CARTESIAN_POINT ( 'NONE',  ( -24.39774143530919304, -13.72145442755526545, 73.27838554735291154 ) ) ;
#3935=EDGE_CURVE ( 'NONE', #42856, #25718, #36605, .T. ) ;
#3937=CARTESIAN_POINT ( 'NONE',  ( -16.93047781583662470, -7.375409967019452395, 74.09871763077661910 ) ) ;
#3938=CARTESIAN_POINT ( 'NONE',  ( -17.13503149044196761, -7.764836982087094164, 70.77563787455143540 ) ) ;
#3939=ORIENTED_EDGE ( 'NONE', *, *, #14171, .F. ) ;
#3940=CARTESIAN_POINT ( 'NONE',  ( -20.52762743779272014, -8.534807845156915818, 63.31121513079826713 ) ) ;
#3943=VERTEX_POINT ( 'NONE', #10200 ) ;
#3946=CARTESIAN_POINT ( 'NONE',  ( -10.62264639038924408, -13.15335193860895302, 71.50828630683409415 ) ) ;
#3949=CARTESIAN_POINT ( 'NONE',  ( -13.85341075922988985, -21.34777127333467561, 72.12618907608873542 ) ) ;
#3951=EDGE_CURVE ( 'NONE', #12784, #31348, #23131, .T. ) ;
#3954=DIRECTION ( 'NONE',  ( -0.3303050442826436783, 0.9438742382973703826, 3.829623549872328964E-09 ) ) ;
#3956=CARTESIAN_POINT ( 'NONE',  ( -22.23733827145997566, -19.96043728507621395, 65.70421731380814379 ) ) ;
#3958=CARTESIAN_POINT ( 'NONE',  ( -24.65023647254185590, -12.99629722456026393, 63.01759562046499497 ) ) ;
#3962=CARTESIAN_POINT ( 'NONE',  ( -22.90552330334707420, -10.36975038659888249, 59.60203168817258046 ) ) ;
#3963=ORIENTED_EDGE ( 'NONE', *, *, #11242, .F. ) ;
#3964=CARTESIAN_POINT ( 'NONE',  ( -17.43688419659117983, -7.809108078509128248, 67.32039585984551877 ) ) ;
#3966=FACE_OUTER_BOUND ( 'NONE', #11525, .T. ) ;
#3968=B_SPLINE_CURVE_WITH_KNOTS ( 'NONE', 3,
 ( #7784, #7534, #45211, #22541, #18583, #37796, #26968, #4092, #33855, #15620 ),
 .UNSPECIFIED., .F., .F.,
 ( 4, 2, 2, 2, 4 ),
 ( 0.1272669073658358463, 0.2522669073463222333, 0.3772669073268086759, 0.5022669073072950630, 0.6272669072877814500 ),
 .UNSPECIFIED. ) ;
#3969=ORIENTED_EDGE ( 'NONE', *, *, #32677, .F. ) ;
#3970=CARTESIAN_POINT ( 'NONE',  ( -13.42948644998191732, -8.996466925491649391, 56.85478874482843992 ) ) ;
#3973=CARTESIAN_POINT ( 'NONE',  ( -10.52030486862438430, -16.25576698781496887, 67.97767553346105274 ) ) ;
#3974=CARTESIAN_POINT ( 'NONE',  ( -18.92057809895272058, -7.919864474132485732, 66.90071783790342863 ) ) ;
#3975=ORIENTED_EDGE ( 'NONE', *, *, #4504, .T. ) ;
#3978=CARTESIAN_POINT ( 'NONE',  ( -20.72450927900464634, -21.03929139025763106, 58.93003081252663833 ) ) ;
#3979=CARTESIAN_POINT ( 'NONE',  ( -18.15520726479059022, -21.77104471536384267, 65.64532137700102510 ) ) ;
#3980=CARTESIAN_POINT ( 'NONE',  ( -22.39459439135063334, -20.35890138417862261, 62.37292654065244335 ) ) ;
#3981=CARTESIAN_POINT ( 'NONE',  ( -18.30726797983150789, -21.75326897020822514, 68.81514702557041119 ) ) ;
#3982=CARTESIAN_POINT ( 'NONE',  ( -23.76567461856301122, -18.71936826787876740, 72.90334907938832032 ) ) ;
#3985=CARTESIAN_POINT ( 'NONE',  ( -11.10470733248389230, -18.75498039752055490, 61.46206112672981448 ) ) ;
#3986=CARTESIAN_POINT ( 'NONE',  ( -14.91739522418961350, -8.273357693606131491, 57.13534681401838355 ) ) ;
#3988=CARTESIAN_POINT ( 'NONE',  ( -21.06635048418738165, -21.30826373965517817, 62.29966805574095901 ) ) ;
#3990=CARTESIAN_POINT ( 'NONE',  ( -11.64964760867527538, -18.76605229218658621, 64.97380311690855592 ) ) ;
#3992=( BOUNDED_SURFACE ( )  B_SPLINE_SURFACE ( 3, 1, ( 
 ( #25291, #1666 ),
 ( #32666, #44021 ),
 ( #43768, #16908 ),
 ( #6080, #21361 ),
 ( #5368, #46958 ),
 ( #13205, #20386 ),
 ( #39814, #24806 ) ),
 .UNSPECIFIED., .T., .F., .F. ) 
 B_SPLINE_SURFACE_WITH_KNOTS ( ( 4, 3, 4 ),
 ( 2, 2 ),
 ( 0.000000000000000000, 0.5000000000000000000, 1.000000000000000000 ),
 ( 0.000000000000000000, 1.000000000000000000 ),
 .UNSPECIFIED. ) 
 GEOMETRIC_REPRESENTATION_ITEM ( )  RATIONAL_B_SPLINE_SURFACE ( (
 ( 1.000000000000000000, 1.000000000000000000),
 ( 0.3333333333333335369, 0.3333333333333330373),
 ( 0.3333333333333335369, 0.3333333333333330373),
 ( 1.000000000000000000, 1.000000000000000000),
 ( 0.3333333333333333703, 0.3333333333333333703),
 ( 0.3333333333333333703, 0.3333333333333333703),
 ( 1.000000000000000000, 1.000000000000000000) ) ) 
 REPRESENTATION_ITEM ( '' )  SURFACE ( )  );
#3993=EDGE_CURVE ( 'NONE', #14949, #28015, #31881, .T. ) ;
#3994=CARTESIAN_POINT ( 'NONE',  ( -21.59804182614902146, -20.98026282434625500, 72.70941811628220819 ) ) ;
#3995=LINE ( 'NONE', #37447, #34141 ) ;
#3997=CARTESIAN_POINT ( 'NONE',  ( -14.03142060029363236, -8.686249327000295395, 74.21457139832153871 ) ) ;
#3999=CARTESIAN_POINT ( 'NONE',  ( -16.06050865347321732, -9.480920197610746669, 54.07175714974878389 ) ) ;
#4000=CARTESIAN_POINT ( 'NONE',  ( -24.38954374850577267, -15.50445147885005071, 73.28838359349398957 ) ) ;
#4007=EDGE_CURVE ( 'NONE', #4227, #5788, #2788, .T. ) ;
#4008=( BOUNDED_CURVE ( )  B_SPLINE_CURVE ( 3, ( #26581, #1193, #34193, #16198 ),
 .UNSPECIFIED., .F., .F. ) 
 B_SPLINE_CURVE_WITH_KNOTS ( ( 4, 4 ),
 ( 0.9074455897393631787, 1.000000000000000000 ),
 .UNSPECIFIED. ) 
 CURVE ( )  GEOMETRIC_REPRESENTATION_ITEM ( )  RATIONAL_B_SPLINE_CURVE ( ( 0.6983129098260822953, 0.7760317562606889874, 0.8765941196519948519, 1.000000000000000000 ) ) 
 REPRESENTATION_ITEM ( '' )  );
#4009=ORIENTED_EDGE ( 'NONE', *, *, #16489, .F. ) ;
#4014=AXIS2_PLACEMENT_3D ( 'NONE', #18043, #18787, #3287 ) ;
#4015=CARTESIAN_POINT ( 'NONE',  ( -22.07022430586338402, -11.86582892075562157, 53.49999999999995026 ) ) ;
#4016=EDGE_CURVE ( 'NONE', #21230, #40125, #21752, .T. ) ;
#4017=AXIS2_PLACEMENT_3D ( 'NONE', #38633, #5155, #16458 ) ;
#4018=PLANE ( 'NONE',  #38680 ) ;
#4019=CARTESIAN_POINT ( 'NONE',  ( -17.72612443559818018, -7.765381109175947927, 60.36588690973874094 ) ) ;
#4020=ORIENTED_EDGE ( 'NONE', *, *, #39997, .T. ) ;
#4021=ADVANCED_FACE ( 'NONE', ( #24502 ), #20788, .T. ) ;
#4022=AXIS2_PLACEMENT_3D ( 'NONE', #42502, #4830, #12924 ) ;
#4023=CARTESIAN_POINT ( 'NONE',  ( -24.36668204746468902, -15.71385111637027165, 73.07474071338100430 ) ) ;
#4025=ORIENTED_EDGE ( 'NONE', *, *, #11707, .F. ) ;
#4026=DIRECTION ( 'NONE',  ( 7.623677598973384647E-06, 4.209792897500673425E-06, -0.9999999999620786673 ) ) ;
#4028=DIRECTION ( 'NONE',  ( -1.053901171479178877E-05, 6.708308826365502595E-06, -0.9999999999219638669 ) ) ;
#4031=DIRECTION ( 'NONE',  ( 0.02843338833657542419, -0.4463087971659328024, 0.8944271909999157444 ) ) ;
#4032=CARTESIAN_POINT ( 'NONE',  ( -12.23160957677214178, -12.95553921741658243, 53.88362224778187226 ) ) ;
#4033=ORIENTED_EDGE ( 'NONE', *, *, #591, .F. ) ;
#4034=CARTESIAN_POINT ( 'NONE',  ( -19.74917416150487171, -21.41189869944521362, 69.23482485975905831 ) ) ;
#4036=AXIS2_PLACEMENT_3D ( 'NONE', #41677, #15065, #45146 ) ;
#4037=EDGE_CURVE ( 'NONE', #22481, #28514, #6504, .T. ) ;
#4042=CARTESIAN_POINT ( 'NONE',  ( -17.42409385541300892, -14.80920654474439679, 47.99999999999994316 ) ) ;
#4043=CARTESIAN_POINT ( 'NONE',  ( -16.13263948075386978, -7.878200451182638453, 63.68483172840383588 ) ) ;
#4044=ADVANCED_FACE ( 'NONE', ( #33054 ), #5781, .T. ) ;
#4046=CARTESIAN_POINT ( 'NONE',  ( -17.65810221059773610, -7.762793303104816189, 63.56529088875731759 ) ) ;
#4047=CARTESIAN_POINT ( 'NONE',  ( -22.63674339536608926, -20.13198319316658313, 69.43063894133570102 ) ) ;
#4049=ADVANCED_FACE ( 'NONE', ( #9478 ), #13379, .T. ) ;
#4051=EDGE_CURVE ( 'NONE', #34971, #27190, #42486, .T. ) ;
#4054=B_SPLINE_CURVE_WITH_KNOTS ( 'NONE', 1,
 ( #34100, #5057 ),
 .UNSPECIFIED., .F., .F.,
 ( 2, 2 ),
 ( 0.000000000000000000, 1.000000000000000000 ),
 .UNSPECIFIED. ) ;
#4055=CARTESIAN_POINT ( 'NONE',  ( -24.35037712455101655, -13.45216126592925754, 62.97697330661279835 ) ) ;
#4057=VERTEX_POINT ( 'NONE', #3284 ) ;
#4058=CARTESIAN_POINT ( 'NONE',  ( -11.33476867595667770, -19.10151316506851416, 68.40185013497388411 ) ) ;
#4059=CARTESIAN_POINT ( 'NONE',  ( -24.47507746028116671, -14.61665733240941378, 59.45120272392967564 ) ) ;
#4060=CARTESIAN_POINT ( 'NONE',  ( -14.71062180296534017, -21.26200528251204247, 58.46617879205846435 ) ) ;
#4061=ORIENTED_EDGE ( 'NONE', *, *, #37204, .T. ) ;
#4063=CARTESIAN_POINT ( 'NONE',  ( -24.42340909951234096, -14.70711335020210520, 59.31588370434493385 ) ) ;
#4066=VERTEX_POINT ( 'NONE', #29879 ) ;
#4071=FACE_OUTER_BOUND ( 'NONE', #19356, .T. ) ;
#4072=CARTESIAN_POINT ( 'NONE',  ( -13.62949042321701398, -8.926946430974666669, 56.96967755885751217 ) ) ;
#4075=VERTEX_POINT ( 'NONE', #11638 ) ;
#4077=EDGE_CURVE ( 'NONE', #41843, #9176, #45417, .T. ) ;
#4078=CARTESIAN_POINT ( 'NONE',  ( -10.44532783130100562, -14.26439015257133924, 61.10924436523676917 ) ) ;
#4081=CARTESIAN_POINT ( 'NONE',  ( -10.77075480930259133, -16.98888344060621947, 61.38572962699099378 ) ) ;
#4082=CARTESIAN_POINT ( 'NONE',  ( -15.25801600794807555, -21.93814553200309092, 72.23230793488828283 ) ) ;
#4084=B_SPLINE_CURVE_WITH_KNOTS ( 'NONE', 3,
 ( #40145, #18198, #33205, #2222, #13769, #20945, #32508, #9638, #17233, #43850 ),
 .UNSPECIFIED., .F., .F.,
 ( 4, 2, 2, 2, 4 ),
 ( 0.000000000000000000, 0.2500000000000000000, 0.5000000000000000000, 0.7500000000000000000, 1.000000000000000000 ),
 .UNSPECIFIED. ) ;
#4085=CARTESIAN_POINT ( 'NONE',  ( -15.62222905942471840, -7.993050613273783966, 70.89517703929612935 ) ) ;
#4086=CARTESIAN_POINT ( 'NONE',  ( -13.73677046600794149, -20.82228291470529058, 61.72466036792861388 ) ) ;
#4088=DIRECTION ( 'NONE',  ( 2.584300424743464895E-08, 1.497441459180121760E-06, -0.9999999999988785637 ) ) ;
#4089=B_SPLINE_CURVE_WITH_KNOTS ( 'NONE', 3,
 ( #46272, #47240, #13000, #5880, #9817, #1442, #16456, #24833, #1931, #43556 ),
 .UNSPECIFIED., .F., .F.,
 ( 4, 2, 2, 2, 4 ),
 ( 0.000000000000000000, 0.2500000000000000000, 0.5000000000000000000, 0.7500000000000000000, 1.000000000000000000 ),
 .UNSPECIFIED. ) ;
#4092=CARTESIAN_POINT ( 'NONE',  ( -12.54429422870864741, -9.179802802619546398, 74.51911777589955932 ) ) ;
#4093=CARTESIAN_POINT ( 'NONE',  ( -20.28216670725803894, -8.419192670066959039, 67.06638753379743889 ) ) ;
#4097=ORIENTED_EDGE ( 'NONE', *, *, #44078, .F. ) ;
#4098=CARTESIAN_POINT ( 'NONE',  ( -10.35611353805053980, -12.45393147150008772, 61.05499485166044593 ) ) ;
#4099=DIRECTION ( 'NONE',  ( 0.7971031148784507581, -0.6038432116460915600, 6.916509187980650173E-08 ) ) ;
#4101=ORIENTED_EDGE ( 'NONE', *, *, #3409, .F. ) ;
#4102=CARTESIAN_POINT ( 'NONE',  ( -19.56968442187927693, -21.94361132924262492, 62.18777784925811147 ) ) ;
#4103=LINE ( 'NONE', #41508, #10098 ) ;
#4105=FACE_OUTER_BOUND ( 'NONE', #3928, .T. ) ;
#4107=ORIENTED_EDGE ( 'NONE', *, *, #1319, .F. ) ;
#4110=DIRECTION ( 'NONE',  ( 0.9087012777736581670, -0.4174469879787382487, -4.853707507795077342E-09 ) ) ;
#4112=CARTESIAN_POINT ( 'NONE',  ( -15.20275948037936864, -21.92046911484317917, 68.75309815756419596 ) ) ;
#4117=LINE ( 'NONE', #30703, #47847 ) ;
#4118=CARTESIAN_POINT ( 'NONE',  ( -12.26752988409003287, -16.72227946798956211, 53.49899999999994549 ) ) ;
#4119=CARTESIAN_POINT ( 'NONE',  ( -10.61330258792943226, -12.98832159324076052, 68.03832347271725212 ) ) ;
#4120=EDGE_LOOP ( 'NONE', ( #808, #33790, #24335, #44301 ) ) ;
#4123=ORIENTED_EDGE ( 'NONE', *, *, #20671, .T. ) ;
#4124=ORIENTED_EDGE ( 'NONE', *, *, #37879, .T. ) ;
#4127=CARTESIAN_POINT ( 'NONE',  ( -23.34481640033245853, -18.63641755246779752, 69.59371984262205046 ) ) ;
#4128=CARTESIAN_POINT ( 'NONE',  ( -12.95250271175661183, -20.26353575427058828, 71.69165012371371404 ) ) ;
#4129=CYLINDRICAL_SURFACE ( 'NONE', #8288, 0.1500000000000031586 ) ;
#4131=CARTESIAN_POINT ( 'NONE',  ( -14.04013919049901560, -8.171999524408169790, 70.77311711151845941 ) ) ;
#4132=CARTESIAN_POINT ( 'NONE',  ( -12.51424385636291170, -20.41247444060362071, 71.99991975137920974 ) ) ;
#4133=ORIENTED_EDGE ( 'NONE', *, *, #28391, .T. ) ;
#4134=ORIENTED_EDGE ( 'NONE', *, *, #41325, .F. ) ;
#4135=CARTESIAN_POINT ( 'NONE',  ( -17.52853272358826686, -7.759682304905023642, 63.83584969886392457 ) ) ;
#4137=CARTESIAN_POINT ( 'NONE',  ( -22.54704564128305222, -20.21849264563443782, 65.86455114034160374 ) ) ;
#4138=CARTESIAN_POINT ( 'NONE',  ( -10.51635384603322976, -15.94466201910895897, 67.99384522443050116 ) ) ;
#4139=CARTESIAN_POINT ( 'NONE',  ( -23.37999588001404661, -18.58199455739222827, 69.57899840282863124 ) ) ;
#4141=( BOUNDED_CURVE ( )  B_SPLINE_CURVE ( 3, ( #32381, #47401, #13637, #28677 ),
 .UNSPECIFIED., .F., .F. ) 
 B_SPLINE_CURVE_WITH_KNOTS ( ( 4, 4 ),
 ( 0.4074455897393696180, 0.5000000000000000000 ),
 .UNSPECIFIED. ) 
 CURVE ( )  GEOMETRIC_REPRESENTATION_ITEM ( )  RATIONAL_B_SPLINE_CURVE ( ( 0.6983129098261098289, 0.7760317562606982023, 0.8765941196519907441, 0.9999999999999770184 ) ) 
 REPRESENTATION_ITEM ( '' )  );
#4143=EDGE_LOOP ( 'NONE', ( #30258, #16228, #22628, #21162, #7820 ) ) ;
#4145=CARTESIAN_POINT ( 'NONE',  ( -10.47141612868932192, -15.99879407189726699, 71.74750680274701153 ) ) ;
#4148=CARTESIAN_POINT ( 'NONE',  ( -20.31649657898477912, -7.943510300654241796, 70.43595776394847974 ) ) ;
#4152=ORIENTED_EDGE ( 'NONE', *, *, #35530, .T. ) ;
#4153=DIRECTION ( 'NONE',  ( -0.6172023957221239865, -0.7799807200343535918, 0.1033986416233890343 ) ) ;
#4156=ORIENTED_EDGE ( 'NONE', *, *, #27277, .T. ) ;
#4157=CARTESIAN_POINT ( 'NONE',  ( -10.49862840407593367, -15.82799419795606966, 64.80771590052736997 ) ) ;
#4158=( BOUNDED_CURVE ( )  B_SPLINE_CURVE ( 3, ( #9233, #12428, #12190, #27697 ),
 .UNSPECIFIED., .F., .F. ) 
 B_SPLINE_CURVE_WITH_KNOTS ( ( 4, 4 ),
 ( 0.9074455897393693959, 1.000000000000000000 ),
 .UNSPECIFIED. ) 
 CURVE ( )  GEOMETRIC_REPRESENTATION_ITEM ( )  RATIONAL_B_SPLINE_CURVE ( ( 0.6983129098261139367, 0.7760317562607162989, 0.8765941196520116163, 1.000000000000000000 ) ) 
 REPRESENTATION_ITEM ( '' )  );
#4159=EDGE_LOOP ( 'NONE', ( #37727, #16692 ) ) ;
#4160=CARTESIAN_POINT ( 'NONE',  ( -10.54994933093899867, -13.24305344519376959, 71.49356453765415154 ) ) ;
#4161=CARTESIAN_POINT ( 'NONE',  ( -23.84743916260113039, -11.89450597454958114, 63.25218314574954093 ) ) ;
#4162=VERTEX_POINT ( 'NONE', #21998 ) ;
#4163=EDGE_CURVE ( 'NONE', #15682, #37990, #15414, .T. ) ;
#4165=CARTESIAN_POINT ( 'NONE',  ( -23.78500256881436314, -11.88707711785523635, 59.48235732566631384 ) ) ;
#4166=CARTESIAN_POINT ( 'NONE',  ( -12.45873566688477929, -9.804017486950373339, 57.10407583662104258 ) ) ;
#4167=VERTEX_POINT ( 'NONE', #19271 ) ;
#4168=CARTESIAN_POINT ( 'NONE',  ( -11.29134393598116937, -11.33126488396075260, 64.16354160640879911 ) ) ;
#4169=CARTESIAN_POINT ( 'NONE',  ( -22.79960237261627398, -9.650942640399760464, 73.66656521964461035 ) ) ;
#4170=CARTESIAN_POINT ( 'NONE',  ( -11.96671518932367029, -9.737692337828448785, 60.66579796421850546 ) ) ;
#4171=VERTEX_POINT ( 'NONE', #34276 ) ;
#4172=CARTESIAN_POINT ( 'NONE',  ( -19.22943344864035353, -8.044691675300194689, 63.65919177093534387 ) ) ;
#4173=EDGE_CURVE ( 'NONE', #43582, #4699, #23122, .T. ) ;
#4174=CARTESIAN_POINT ( 'NONE',  ( -23.57312343282865896, -11.36065554106722786, 69.89210769048611382 ) ) ;
#4175=EDGE_LOOP ( 'NONE', ( #41006, #28427 ) ) ;
#4176=ORIENTED_EDGE ( 'NONE', *, *, #43070, .T. ) ;
#4177=EDGE_CURVE ( 'NONE', #12172, #20147, #46980, .T. ) ;
#4178=CARTESIAN_POINT ( 'NONE',  ( -24.84861529636215849, -14.19299288461673747, 69.75936971009964793 ) ) ;
#4179=CARTESIAN_POINT ( 'NONE',  ( -19.17437844398820701, -7.979623566120205957, 63.44561363416070776 ) ) ;
#4180=CARTESIAN_POINT ( 'NONE',  ( -14.07761608144266674, -20.95746532167037302, 71.92607703845176559 ) ) ;
#4181=VERTEX_POINT ( 'NONE', #14813 ) ;
#4183=EDGE_CURVE ( 'NONE', #28650, #44593, #38358, .T. ) ;
#4184=CARTESIAN_POINT ( 'NONE',  ( -10.40257400440372315, -14.13711964566031654, 57.65644799979391166 ) ) ;
#4186=DIRECTION ( 'NONE',  ( -0.7150252244155669290, 0.6990986543038602008, -7.133781456731120165E-17 ) ) ;
#4190=CARTESIAN_POINT ( 'NONE',  ( -10.57550014152487705, -13.13548074022098433, 71.21388402457256461 ) ) ;
#4193=ORIENTED_EDGE ( 'NONE', *, *, #20444, .F. ) ;
#4194=DIRECTION ( 'NONE',  ( 3.913797943140854342E-06, 1.965591624649253694E-06, 0.9999999999904093384 ) ) ;
#4195=FACE_OUTER_BOUND ( 'NONE', #36114, .T. ) ;
#4196=CARTESIAN_POINT ( 'NONE',  ( -22.56207008003183745, -19.63703213565221617, 72.92928497383269359 ) ) ;
#4197=CARTESIAN_POINT ( 'NONE',  ( -20.03282965983824226, -21.84088468745754597, 47.99999999999994316 ) ) ;
#4198=VERTEX_POINT ( 'NONE', #806 ) ;
#4199=CARTESIAN_POINT ( 'NONE',  ( -23.54066400932483205, -11.40515459557274447, 66.53100539013419734 ) ) ;
#4200=CARTESIAN_POINT ( 'NONE',  ( -14.24059955017480306, -8.515543114936868108, 67.14486463900426827 ) ) ;
#4202=CARTESIAN_POINT ( 'NONE',  ( -22.67603917253425294, -10.10156321767594179, 73.89649722025401957 ) ) ;
#4203=CARTESIAN_POINT ( 'NONE',  ( -21.29196722032537537, -20.70380199363842877, 72.53918572867779346 ) ) ;
#4204=CARTESIAN_POINT ( 'NONE',  ( -13.85534475943383370, -8.269504983759647487, 74.24308752109034515 ) ) ;
#4207=CARTESIAN_POINT ( 'NONE',  ( -21.76140000860026191, -9.313236413093783028, 66.88979917059124602 ) ) ;
#4210=B_SPLINE_CURVE_WITH_KNOTS ( 'NONE', 3,
 ( #22145, #10571, #6873, #41092, #28794, #47747, #44317, #2921, #25824, #29033 ),
 .UNSPECIFIED., .F., .F.,
 ( 4, 2, 2, 2, 4 ),
 ( 0.1272669073658634353, 0.2522669073463360001, 0.3772669073268085649, 0.5022669073072811852, 0.6272669072877536944 ),
 .UNSPECIFIED. ) ;
#4211=CARTESIAN_POINT ( 'NONE',  ( -19.22579631480732587, -21.57336711704104104, 58.82507384991394872 ) ) ;
#4212=EDGE_LOOP ( 'NONE', ( #44413, #23588, #26598, #14037, #39097 ) ) ;
#4213=FACE_OUTER_BOUND ( 'NONE', #7648, .T. ) ;
#4217=CARTESIAN_POINT ( 'NONE',  ( -17.59048613883335932, -21.80850830400060403, 58.63383171954600215 ) ) ;
#4218=LINE ( 'NONE', #45596, #10366 ) ;
#4220=ORIENTED_EDGE ( 'NONE', *, *, #37408, .F. ) ;
#4221=CARTESIAN_POINT ( 'NONE',  ( -23.19916440516392697, -19.59445054535707698, 47.99999999999994316 ) ) ;
#4222=CARTESIAN_POINT ( 'NONE',  ( -13.18473975798692877, -20.93551490194142062, 58.23145353898504339 ) ) ;
#4226=ORIENTED_EDGE ( 'NONE', *, *, #31002, .F. ) ;
#4227=VERTEX_POINT ( 'NONE', #38951 ) ;
#4228=ADVANCED_FACE ( 'NONE', ( #12131 ), #6130, .T. ) ;
#4229=CARTESIAN_POINT ( 'NONE',  ( -24.48129518141919903, -12.42204491826083590, 73.44214348908371903 ) ) ;
#4230=CARTESIAN_POINT ( 'NONE',  ( -14.72744631621160494, -8.295007313424175521, 60.60524229057013201 ) ) ;
#4233=CARTESIAN_POINT ( 'NONE',  ( -15.19548991633585011, -21.91815178685365595, 68.76088227238139439 ) ) ;
#4237=CARTESIAN_POINT ( 'NONE',  ( -24.39823031370633544, -14.19330659245935422, 73.35101391479588528 ) ) ;
#4238=CARTESIAN_POINT ( 'NONE',  ( -23.59011972508282895, -18.99064774873246009, 65.94576636911624234 ) ) ;
#4239=CARTESIAN_POINT ( 'NONE',  ( -14.06269433208033171, -8.668953365929850108, 74.19954661247773231 ) ) ;
#4241=CARTESIAN_POINT ( 'NONE',  ( -22.75539019595754908, -10.19575032747719412, 66.82710158566565894 ) ) ;
#4243=CARTESIAN_POINT ( 'NONE',  ( -24.12651600458584511, -12.62191667979047338, 73.25697658996379857 ) ) ;
#4244=DIRECTION ( 'NONE',  ( 6.059369597461991776E-06, -3.309764069070163182E-06, -0.9999999999761647329 ) ) ;
#4245=CARTESIAN_POINT ( 'NONE',  ( -11.92202137443377907, -10.38855435516889081, 64.18481546414660954 ) ) ;
#4247=CARTESIAN_POINT ( 'NONE',  ( -23.78676244964941233, -10.93361294341921131, 73.54688584860882372 ) ) ;
#4248=ORIENTED_EDGE ( 'NONE', *, *, #38402, .F. ) ;
#4250=CARTESIAN_POINT ( 'NONE',  ( -12.12884284833700299, -9.568708778729794417, 57.23935532548082961 ) ) ;
#4251=B_SPLINE_CURVE_WITH_KNOTS ( 'NONE', 3,
 ( #46765, #4673, #27800, #8621, #19935, #13009, #42828, #9101, #5162, #31253 ),
 .UNSPECIFIED., .F., .F.,
 ( 4, 2, 2, 2, 4 ),
 ( 0.000000000000000000, 0.2500000000000000000, 0.5000000000000000000, 0.7500000000000000000, 1.000000000000000000 ),
 .UNSPECIFIED. ) ;
#4252=ORIENTED_EDGE ( 'NONE', *, *, #4988, .F. ) ;
#4255=CARTESIAN_POINT ( 'NONE',  ( -13.67313477037754232, -20.71991182390168618, 65.27012384153809421 ) ) ;
#4256=CARTESIAN_POINT ( 'NONE',  ( -16.64476583608805882, -21.82402065185451079, 72.30976097999173646 ) ) ;
#4258=B_SPLINE_CURVE_WITH_KNOTS ( 'NONE', 3,
 ( #31204, #19151, #26792, #46227, #12488, #5109, #41817, #8093, #23103, #38095 ),
 .UNSPECIFIED., .F., .F.,
 ( 4, 2, 2, 2, 4 ),
 ( 0.6272669072877604668, 0.7522669073072876245, 0.8772669073268148932, 1.002266907346342162, 1.127266907365869208 ),
 .UNSPECIFIED. ) ;
#4259=PLANE ( 'NONE',  #38308 ) ;
#4261=CARTESIAN_POINT ( 'NONE',  ( -11.46044050272623416, -11.04924139602722200, 57.20903212151936401 ) ) ;
#4263=CARTESIAN_POINT ( 'NONE',  ( -10.37394849890712401, -14.76283852923608286, 71.61310637325181006 ) ) ;
#4264=ORIENTED_EDGE ( 'NONE', *, *, #22170, .F. ) ;
#4266=CARTESIAN_POINT ( 'NONE',  ( -11.09636497276514966, -11.81291589161553901, 74.63010272337737661 ) ) ;
#4267=CARTESIAN_POINT ( 'NONE',  ( -10.41569439578338496, -15.57669382292980131, 61.05261153187079515 ) ) ;
#4268=EDGE_LOOP ( 'NONE', ( #25808, #7829 ) ) ;
#4269=CARTESIAN_POINT ( 'NONE',  ( -22.28468842640967651, -19.91619389767071269, 65.98949666203347419 ) ) ;
#4272=CARTESIAN_POINT ( 'NONE',  ( -16.20999260610575377, -7.914000153054798758, 63.74181402343131708 ) ) ;
#4274=ORIENTED_EDGE ( 'NONE', *, *, #38727, .T. ) ;
#4275=FACE_OUTER_BOUND ( 'NONE', #16659, .T. ) ;
#4276=CARTESIAN_POINT ( 'NONE',  ( -24.37529183752970141, -13.98356525902160463, 73.13773933009861139 ) ) ;
#4279=CARTESIAN_POINT ( 'NONE',  ( -10.41569439578338496, -15.57669382292980131, 61.05261153187079515 ) ) ;
#4284=EDGE_LOOP ( 'NONE', ( #9682, #1703, #13145, #5546, #20447 ) ) ;
#4285=EDGE_CURVE ( 'NONE', #1012, #34613, #38463, .T. ) ;
#4287=CARTESIAN_POINT ( 'NONE',  ( -11.00824494338232284, -11.02245153356902030, 60.87874549475150587 ) ) ;
#4290=CARTESIAN_POINT ( 'NONE',  ( -15.30848412986786578, -21.53807271814892843, 65.31416673886597835 ) ) ;
#4291=CARTESIAN_POINT ( 'NONE',  ( -18.46801905451614090, -7.836623195388690455, 74.12592262855558545 ) ) ;
#4292=EDGE_LOOP ( 'NONE', ( #14622, #26408, #44641, #1898, #23574 ) ) ;
#4293=DIRECTION ( 'NONE',  ( 0.8705373987491421550, -0.4921022631314296292, 4.758021987246392057E-08 ) ) ;
#4294=( BOUNDED_CURVE ( )  B_SPLINE_CURVE ( 3, ( #31601, #27412, #38233, #11923 ),
 .UNSPECIFIED., .F., .F. ) 
 B_SPLINE_CURVE_WITH_KNOTS ( ( 4, 4 ),
 ( 0.9074455897393672865, 1.000000000000000000 ),
 .UNSPECIFIED. ) 
 CURVE ( )  GEOMETRIC_REPRESENTATION_ITEM ( )  RATIONAL_B_SPLINE_CURVE ( ( 0.6983129098260997258, 0.7760317562607039754, 0.8765941196520040668, 1.000000000000000000 ) ) 
 REPRESENTATION_ITEM ( '' )  );
#4295=EDGE_CURVE ( 'NONE', #43099, #7039, #47188, .T. ) ;
#4296=DIRECTION ( 'NONE',  ( -8.339041841313433703E-07, -7.401745998521586792E-06, 0.9999999999722594124 ) ) ;
#4297=EDGE_LOOP ( 'NONE', ( #26550, #23859, #20775, #40130, #44836 ) ) ;
#4301=CARTESIAN_POINT ( 'NONE',  ( -24.79583619959666763, -15.88736519870960784, 69.67274155994940088 ) ) ;
#4302=CARTESIAN_POINT ( 'NONE',  ( -10.52991759648590531, -16.02177972226642311, 68.27767831073917648 ) ) ;
#4303=B_SPLINE_CURVE_WITH_KNOTS ( 'NONE', 3,
 ( #24637, #38669, #16966, #16493, #32010, #47024, #31527, #20196, #35208, #31769 ),
 .UNSPECIFIED., .F., .F.,
 ( 4, 2, 2, 2, 4 ),
 ( 0.000000000000000000, 0.2500000000000000000, 0.5000000000000000000, 0.7500000000000000000, 1.000000000000000000 ),
 .UNSPECIFIED. ) ;
#4305=ORIENTED_EDGE ( 'NONE', *, *, #44467, .F. ) ;
#4306=EDGE_LOOP ( 'NONE', ( #26160, #28478, #28027, #38915, #13793 ) ) ;
#4308=CARTESIAN_POINT ( 'NONE',  ( -22.98865756656685022, -9.855479763439479512, 70.12683098403445570 ) ) ;
#4313=EDGE_CURVE ( 'NONE', #26935, #35691, #7257, .T. ) ;
#4315=CARTESIAN_POINT ( 'NONE',  ( -23.00441852451001523, -19.11762575345012749, 58.88410642058938294 ) ) ;
#4316=EDGE_CURVE ( 'NONE', #44852, #37303, #41665, .T. ) ;
#4317=CARTESIAN_POINT ( 'NONE',  ( -20.94465692579565896, -8.243430592510261334, 59.95629952546280350 ) ) ;
#4318=CARTESIAN_POINT ( 'NONE',  ( -18.86948588052436904, -7.959932294928454333, 66.90071733017600764 ) ) ;
#4320=ORIENTED_EDGE ( 'NONE', *, *, #37251, .T. ) ;
#4323=CARTESIAN_POINT ( 'NONE',  ( -22.33142775017075010, -9.202805011845722305, 59.90826508960974195 ) ) ;
#4324=CARTESIAN_POINT ( 'NONE',  ( -20.21484531253453198, -8.389572098386633314, 66.97207325640498254 ) ) ;
#4326=PLANE ( 'NONE',  #35612 ) ;
#4327=ORIENTED_EDGE ( 'NONE', *, *, #4641, .T. ) ;
#4328=CARTESIAN_POINT ( 'NONE',  ( -20.21944967009625671, -8.333140613769380423, 73.81276534411087198 ) ) ;
#4329=CARTESIAN_POINT ( 'NONE',  ( -21.36489355414517988, -8.963473290115421932, 73.90128753234840531 ) ) ;
#4332=ORIENTED_EDGE ( 'NONE', *, *, #29601, .F. ) ;
#4333=CYLINDRICAL_SURFACE ( 'NONE', #17356, 0.1500000000000015488 ) ;
#4334=CARTESIAN_POINT ( 'NONE',  ( -24.22092332596094977, -12.93687947476191269, 66.45246741375130739 ) ) ;
#4335=PLANE ( 'NONE',  #23098 ) ;
#4336=PLANE ( 'NONE',  #10065 ) ;
#4338=ORIENTED_EDGE ( 'NONE', *, *, #44462, .T. ) ;
#4339=CARTESIAN_POINT ( 'NONE',  ( -11.38873422713818684, -18.35549357326604891, 58.10714557467345998 ) ) ;
#4340=CARTESIAN_POINT ( 'NONE',  ( -15.20214831426356739, -21.92027429138432026, 68.69780165605466493 ) ) ;
#4341=CARTESIAN_POINT ( 'NONE',  ( -21.67609690912980014, -8.690862426448951794, 73.78784151156415305 ) ) ;
#4342=ORIENTED_EDGE ( 'NONE', *, *, #21348, .T. ) ;
#4343=LINE ( 'NONE', #44746, #22909 ) ;
#4345=CARTESIAN_POINT ( 'NONE',  ( -12.73481051501216044, -9.020086340885832499, 70.95651207417664352 ) ) ;
#4346=CARTESIAN_POINT ( 'NONE',  ( -13.21199854220980718, -9.217750189091946211, 67.39559466746432292 ) ) ;
#4348=CARTESIAN_POINT ( 'NONE',  ( -9.939267784769082681, -14.33236412611010913, 53.49999999999994316 ) ) ;
#4349=EDGE_CURVE ( 'NONE', #36615, #14276, #199, .T. ) ;
#4350=EDGE_LOOP ( 'NONE', ( #31517, #13786 ) ) ;
#4351=ORIENTED_EDGE ( 'NONE', *, *, #26350, .F. ) ;
#4353=CARTESIAN_POINT ( 'NONE',  ( -22.28902083190231309, -19.84295425696266335, 69.19034576393465841 ) ) ;
#4354=CARTESIAN_POINT ( 'NONE',  ( -19.38292004262868673, -21.99720527105973744, 58.64694598308297202 ) ) ;
#4356=CARTESIAN_POINT ( 'NONE',  ( -12.65491851050466288, -19.93331706820960747, 68.63657436096360698 ) ) ;
#4357=CYLINDRICAL_SURFACE ( 'NONE', #14961, 0.1500000000000038802 ) ;
#4358=VERTEX_POINT ( 'NONE', #17500 ) ;
#4361=CARTESIAN_POINT ( 'NONE',  ( -10.38752013045322009, -14.36951432065623635, 64.67331771650336236 ) ) ;
#4363=ORIENTED_EDGE ( 'NONE', *, *, #26234, .T. ) ;
#4365=EDGE_CURVE ( 'NONE', #34898, #40354, #8997, .T. ) ;
#4367=ADVANCED_FACE ( 'NONE', ( #31811 ), #40399, .T. ) ;
#4369=CARTESIAN_POINT ( 'NONE',  ( -12.41310947992116098, -19.76871611099698001, 61.68206578716802113 ) ) ;
#4370=B_SPLINE_CURVE_WITH_KNOTS ( 'NONE', 1,
 ( #27746, #42776 ),
 .UNSPECIFIED., .F., .F.,
 ( 2, 2 ),
 ( 0.000000000000000000, 1.000000000000000000 ),
 .UNSPECIFIED. ) ;
#4371=CARTESIAN_POINT ( 'NONE',  ( -15.22349782163815490, -21.45476955923737705, 68.85976349797824980 ) ) ;
#4372=ORIENTED_EDGE ( 'NONE', *, *, #6608, .T. ) ;
#4373=CARTESIAN_POINT ( 'NONE',  ( -10.00117625416208433, -15.44487358686203571, 57.68297391752145842 ) ) ;
#4375=CARTESIAN_POINT ( 'NONE',  ( -10.42581515057458930, -14.65397996935263336, 67.96686193206075188 ) ) ;
#4378=CARTESIAN_POINT ( 'NONE',  ( -10.56492483649129710, -13.18000429128331596, 71.50828586225091499 ) ) ;
#4380=CARTESIAN_POINT ( 'NONE',  ( -20.18232088801011415, -7.888550879367295821, 73.82822426864265708 ) ) ;
#4382=CARTESIAN_POINT ( 'NONE',  ( -10.49862800246030936, -15.82799116930659622, 64.50771590054291948 ) ) ;
#4384=CARTESIAN_POINT ( 'NONE',  ( -10.61247293337548214, -12.97981955831074075, 71.62317441356958625 ) ) ;
#4385=CARTESIAN_POINT ( 'NONE',  ( -11.03124136535102373, -17.66077402989073875, 71.56718193465405875 ) ) ;
#4386=ORIENTED_EDGE ( 'NONE', *, *, #31017, .T. ) ;
#4387=CARTESIAN_POINT ( 'NONE',  ( -23.96075626263749214, -17.45014286185010732, 66.24357239682277054 ) ) ;
#4388=CARTESIAN_POINT ( 'NONE',  ( -17.94572468556024702, -21.83992273462958877, 62.17535918563021369 ) ) ;
#4389=EDGE_CURVE ( 'NONE', #32914, #15992, #39732, .T. ) ;
#4390=CARTESIAN_POINT ( 'NONE',  ( -14.28913879486226435, -8.050816564744696535, 67.37479651646088996 ) ) ;
#4391=ORIENTED_EDGE ( 'NONE', *, *, #33343, .F. ) ;
#4392=CARTESIAN_POINT ( 'NONE',  ( -21.31800817620502286, -20.62620158190326336, 72.82446429882371319 ) ) ;
#4394=CARTESIAN_POINT ( 'NONE',  ( -11.48063109083140354, -11.11096805901812878, 57.50903159540615661 ) ) ;
#4396=CARTESIAN_POINT ( 'NONE',  ( -12.36756753426621813, -9.896138138887707214, 57.37463480816234096 ) ) ;
#4397=CARTESIAN_POINT ( 'NONE',  ( -23.34288396506439867, -19.33377296368179543, 59.06906041190286771 ) ) ;
#4398=ORIENTED_EDGE ( 'NONE', *, *, #1526, .T. ) ;
#4399=VERTEX_POINT ( 'NONE', #5950 ) ;
#4400=CARTESIAN_POINT ( 'NONE',  ( -22.84587727614884756, -10.37951393556890523, 66.77012138597072521 ) ) ;
#4401=CARTESIAN_POINT ( 'NONE',  ( -10.61247293337548214, -12.97981955831074075, 71.62317441356958625 ) ) ;
#4404=CARTESIAN_POINT ( 'NONE',  ( -24.46950595589296285, -14.38832865607273703, 73.26704460715303924 ) ) ;
#4405=( BOUNDED_CURVE ( )  B_SPLINE_CURVE ( 3, ( #46823, #20490, #46350, #16527 ),
 .UNSPECIFIED., .F., .F. ) 
 B_SPLINE_CURVE_WITH_KNOTS ( ( 4, 4 ),
 ( 0.9074455897393649551, 1.000000000000000000 ),
 .UNSPECIFIED. ) 
 CURVE ( )  GEOMETRIC_REPRESENTATION_ITEM ( )  RATIONAL_B_SPLINE_CURVE ( ( 0.6983129098260905110, 0.7760317562606959818, 0.8765941196519991818, 1.000000000000000000 ) ) 
 REPRESENTATION_ITEM ( '' )  );
#4406=CARTESIAN_POINT ( 'NONE',  ( -12.40538917401127961, -20.31523793222865493, 68.52152763170285255 ) ) ;
#4408=CARTESIAN_POINT ( 'NONE',  ( -11.07238894598444112, -11.74315414212633080, 67.50375847841529264 ) ) ;
#4410=ORIENTED_EDGE ( 'NONE', *, *, #33600, .T. ) ;
#4411=DIRECTION ( 'NONE',  ( -0.1648596854219665231, -0.9863170302304251624, 7.074492695208254125E-08 ) ) ;
#4412=( NAMED_UNIT ( * ) SI_UNIT ( $, .STERADIAN. ) SOLID_ANGLE_UNIT ( ) );
#4413=CARTESIAN_POINT ( 'NONE',  ( -24.53360078033622216, -12.58211837844622849, 69.93276349028228367 ) ) ;
#4414=CARTESIAN_POINT ( 'NONE',  ( -23.89370412103122021, -17.61049410758369760, 62.77360985931112225 ) ) ;
#4415=( BOUNDED_CURVE ( )  B_SPLINE_CURVE ( 3, ( #5809, #43234, #9508, #12700 ),
 .UNSPECIFIED., .F., .F. ) 
 B_SPLINE_CURVE_WITH_KNOTS ( ( 4, 4 ),
 ( 0.5000000000000000000, 0.9074455897393668424 ),
 .UNSPECIFIED. ) 
 CURVE ( )  GEOMETRIC_REPRESENTATION_ITEM ( )  RATIONAL_B_SPLINE_CURVE ( ( 1.000000000000026423, 0.4567392136813426817, 0.3561768502900156674, 0.6983129098260740797 ) ) 
 REPRESENTATION_ITEM ( '' )  );
#4416=ORIENTED_EDGE ( 'NONE', *, *, #25102, .F. ) ;
#4418=EDGE_CURVE ( 'NONE', #5705, #18740, #37350, .T. ) ;
#4419=CARTESIAN_POINT ( 'NONE',  ( -19.92732520184441825, -21.34631850905071815, 69.05907916208967379 ) ) ;
#4420=CARTESIAN_POINT ( 'NONE',  ( -23.85974590284097374, -11.05473623917629844, 73.54848671873985211 ) ) ;
#4421=CARTESIAN_POINT ( 'NONE',  ( -15.40747091633432575, -21.98125088338273514, 72.18428936984274458 ) ) ;
#4422=CARTESIAN_POINT ( 'NONE',  ( -15.93879930885702656, -7.917138641544857691, 67.15479422225767792 ) ) ;
#4424=CARTESIAN_POINT ( 'NONE',  ( -20.19231683483797113, -8.325423577284544407, 70.55100341277886855 ) ) ;
#4425=( BOUNDED_SURFACE ( )  B_SPLINE_SURFACE ( 3, 1, ( 
 ( #3750, #15967 ),
 ( #14316, #29609 ),
 ( #29367, #44638 ),
 ( #44399, #31010 ),
 ( #8359, #18765 ),
 ( #14792, #38372 ),
 ( #4666, #46031 ) ),
 .UNSPECIFIED., .T., .F., .F. ) 
 B_SPLINE_SURFACE_WITH_KNOTS ( ( 4, 3, 4 ),
 ( 2, 2 ),
 ( 0.000000000000000000, 0.5000000000000000000, 1.000000000000000000 ),
 ( 0.000000000000000000, 1.000000000000000000 ),
 .UNSPECIFIED. ) 
 GEOMETRIC_REPRESENTATION_ITEM ( )  RATIONAL_B_SPLINE_SURFACE ( (
 ( 1.000000000000000000, 1.000000000000000000),
 ( 0.3333333333333335369, 0.3333333333333330373),
 ( 0.3333333333333335369, 0.3333333333333330373),
 ( 1.000000000000000000, 1.000000000000000000),
 ( 0.3333333333333333703, 0.3333333333333333703),
 ( 0.3333333333333333703, 0.3333333333333333703),
 ( 1.000000000000000000, 1.000000000000000000) ) ) 
 REPRESENTATION_ITEM ( '' )  SURFACE ( )  );
#4426=ADVANCED_FACE ( 'NONE', ( #29077 ), #11759, .T. ) ;
#4428=CARTESIAN_POINT ( 'NONE',  ( -24.47217469005601131, -14.64471752244405067, 62.71296487297676947 ) ) ;
#4429=ORIENTED_EDGE ( 'NONE', *, *, #14551, .F. ) ;
#4430=EDGE_CURVE ( 'NONE', #28690, #25694, #17986, .T. ) ;
#4431=CARTESIAN_POINT ( 'NONE',  ( -24.46146587544552276, -14.38248120490118609, 66.46820668217904426 ) ) ;
#4432=EDGE_CURVE ( 'NONE', #27722, #16942, #46702, .T. ) ;
#4434=VERTEX_POINT ( 'NONE', #14501 ) ;
#4435=CARTESIAN_POINT ( 'NONE',  ( -12.46122051107220408, -19.81685944811288991, 64.88146935704573082 ) ) ;
#4436=AXIS2_PLACEMENT_3D ( 'NONE', #16822, #21682, #36665 ) ;
#4439=CARTESIAN_POINT ( 'NONE',  ( -10.81170448216924740, -12.36318809540519048, 57.34329390664808557 ) ) ;
#4440=CARTESIAN_POINT ( 'NONE',  ( -11.42587710518540334, -11.10406226247761019, 57.49431069621225276 ) ) ;
#4441=EDGE_LOOP ( 'NONE', ( #14485, #43355, #48668, #359, #4634 ) ) ;
#4444=EDGE_CURVE ( 'NONE', #29219, #3179, #22183, .T. ) ;
#4446=CARTESIAN_POINT ( 'NONE',  ( -17.57433509196185994, -21.80920136703782575, 58.51626380509593162 ) ) ;
#4447=CARTESIAN_POINT ( 'NONE',  ( -10.54860170345752302, -17.67816087046063700, 68.28996115284763846 ) ) ;
#4450=CARTESIAN_POINT ( 'NONE',  ( -19.22579631480732587, -21.57336711704104104, 58.82507384991394872 ) ) ;
#4452=CARTESIAN_POINT ( 'NONE',  ( -23.56856754720352853, -18.27334893135431315, 72.76367955138505295 ) ) ;
#4455=ORIENTED_EDGE ( 'NONE', *, *, #14484, .T. ) ;
#4456=ORIENTED_EDGE ( 'NONE', *, *, #45821, .F. ) ;
#4457=CARTESIAN_POINT ( 'NONE',  ( -18.69922557824643761, -7.468382084482742655, 74.02719791125277027 ) ) ;
#4460=CARTESIAN_POINT ( 'NONE',  ( -24.00225419842380603, -17.20718624873268254, 73.07263044545001662 ) ) ;
#4461=DIRECTION ( 'NONE',  ( -1.352396026799963059E-06, -5.694414568552746141E-07, -0.9999999999989234167 ) ) ;
#4464=CARTESIAN_POINT ( 'NONE',  ( -14.24059955017480306, -8.515543114936868108, 67.14486463900426827 ) ) ;
#4465=CARTESIAN_POINT ( 'NONE',  ( -19.55458118857802319, -21.94809134954223140, 62.09480011547082512 ) ) ;
#4466=FACE_OUTER_BOUND ( 'NONE', #27960, .T. ) ;
#4467=ORIENTED_EDGE ( 'NONE', *, *, #16075, .T. ) ;
#4468=CARTESIAN_POINT ( 'NONE',  ( -24.38957690932039313, -15.50410419900979342, 73.01806150963400910 ) ) ;
#4470=CARTESIAN_POINT ( 'NONE',  ( -15.50784526261009511, -8.076599967007890513, 74.37985659287807039 ) ) ;
#4471=CARTESIAN_POINT ( 'NONE',  ( -14.84764829735760827, -8.246537290690364230, 60.33468334944129197 ) ) ;
#4472=CARTESIAN_POINT ( 'NONE',  ( -14.07539642552819359, -8.605278304397881328, 74.19954655214911554 ) ) ;
#4473=EDGE_CURVE ( 'NONE', #8895, #36030, #40082, .T. ) ;
#4474=B_SPLINE_CURVE_WITH_KNOTS ( 'NONE', 3,
 ( #1023, #4239, #3997, #38431, #33763, #783, #15044, #15780, #30104, #16019 ),
 .UNSPECIFIED., .F., .F.,
 ( 4, 2, 2, 2, 4 ),
 ( 0.000000000000000000, 0.2500000000000000000, 0.5000000000000000000, 0.7500000000000000000, 1.000000000000000000 ),
 .UNSPECIFIED. ) ;
#4476=VERTEX_POINT ( 'NONE', #15252 ) ;
#4482=EDGE_CURVE ( 'NONE', #7468, #45657, #3263, .T. ) ;
#4483=CARTESIAN_POINT ( 'NONE',  ( -11.25622321624083355, -18.98904307544693282, 64.86051675911045322 ) ) ;
#4486=CARTESIAN_POINT ( 'NONE',  ( -21.84256997353123353, -8.809979007422205299, 66.77494628644626573 ) ) ;
#4488=CARTESIAN_POINT ( 'NONE',  ( -17.72612443559818018, -7.765381109175947927, 60.36588690973874094 ) ) ;
#4489=ORIENTED_EDGE ( 'NONE', *, *, #18256, .T. ) ;
#4490=ADVANCED_FACE ( 'NONE', ( #29558 ), #31606, .T. ) ;
#4492=CARTESIAN_POINT ( 'NONE',  ( -18.53202070066404517, -7.846807721809618386, 73.84064401782792686 ) ) ;
#4493=EDGE_CURVE ( 'NONE', #14, #21561, #37165, .T. ) ;
#4494=EDGE_LOOP ( 'NONE', ( #28604, #33133 ) ) ;
#4495=CARTESIAN_POINT ( 'NONE',  ( -11.32266926000110985, -11.37785695497957228, 64.44882076993899034 ) ) ;
#4496=CARTESIAN_POINT ( 'NONE',  ( -12.23758870452319236, -20.15736674837955889, 64.96651269001253581 ) ) ;
#4497=ORIENTED_EDGE ( 'NONE', *, *, #6866, .F. ) ;
#4498=EDGE_CURVE ( 'NONE', #15877, #30899, #41625, .T. ) ;
#4499=CARTESIAN_POINT ( 'NONE',  ( -24.87417961795293664, -14.80849281899037884, 59.42795564617806292 ) ) ;
#4503=CARTESIAN_POINT ( 'NONE',  ( -14.54176566789882585, -21.67913831930545854, 58.28122448549703449 ) ) ;
#4504=EDGE_CURVE ( 'NONE', #42067, #44829, #21517, .T. ) ;
#4505=CARTESIAN_POINT ( 'NONE',  ( -16.11718879935913407, -7.932176570520619308, 63.97011080779262215 ) ) ;
#4507=LINE ( 'NONE', #47570, #14025 ) ;
#4508=CARTESIAN_POINT ( 'NONE',  ( -20.00946503018472811, -8.250368534377352958, 73.72096600125087207 ) ) ;
#4511=CARTESIAN_POINT ( 'NONE',  ( -23.36251582567715701, -10.31057965045351388, 59.75203426425787256 ) ) ;
#4513=CARTESIAN_POINT ( 'NONE',  ( -22.63560595208270954, -20.13310736574185000, 69.28922662766110818 ) ) ;
#4515=ORIENTED_EDGE ( 'NONE', *, *, #19938, .F. ) ;
#4517=CYLINDRICAL_SURFACE ( 'NONE', #39958, 0.1499999999999955536 ) ;
#4518=ORIENTED_EDGE ( 'NONE', *, *, #16829, .T. ) ;
#4519=CARTESIAN_POINT ( 'NONE',  ( -10.37394849890712401, -14.76283852923608464, 71.61310637325181006 ) ) ;
#4522=CARTESIAN_POINT ( 'NONE',  ( -20.75354924259569245, -21.52967727414722532, 54.27966884056655061 ) ) ;
#4523=VERTEX_POINT ( 'NONE', #19944 ) ;
#4524=CARTESIAN_POINT ( 'NONE',  ( -10.04821616988549593, -15.85811384580076933, 64.62276300976363075 ) ) ;
#4525=CARTESIAN_POINT ( 'NONE',  ( -19.05924993160927983, -8.002740344303022724, 63.73089191517998842 ) ) ;
#4526=EDGE_LOOP ( 'NONE', ( #10187, #32784, #38881, #37367, #48200 ) ) ;
#4527=CARTESIAN_POINT ( 'NONE',  ( -12.81603496567665879, -20.14954717766431003, 68.54477457630689230 ) ) ;
#4528=CARTESIAN_POINT ( 'NONE',  ( -12.85370899154983526, -8.925770522350823910, 67.48604460341357481 ) ) ;
#4530=DIRECTION ( 'NONE',  ( 0.9345716196833626643, -0.3557750520798446114, -2.412542649833449708E-09 ) ) ;
#4531=CARTESIAN_POINT ( 'NONE',  ( -23.16108440525936274, -18.82016358243141241, 62.42694848944771024 ) ) ;
#4532=ORIENTED_EDGE ( 'NONE', *, *, #31788, .F. ) ;
#4538=CARTESIAN_POINT ( 'NONE',  ( -24.15236833420705764, -12.70328255177875754, 70.06683202284229139 ) ) ;
#4539=( BOUNDED_CURVE ( )  B_SPLINE_CURVE ( 3, ( #8903, #24404, #13532, #17232 ),
 .UNSPECIFIED., .F., .F. ) 
 B_SPLINE_CURVE_WITH_KNOTS ( ( 4, 4 ),
 ( 0.5000000000000000000, 0.9074455897393604031 ),
 .UNSPECIFIED. ) 
 CURVE ( )  GEOMETRIC_REPRESENTATION_ITEM ( )  RATIONAL_B_SPLINE_CURVE ( ( 0.9999999999999921174, 0.4567392136813352987, 0.3561768502900369282, 0.6983129098260885126 ) ) 
 REPRESENTATION_ITEM ( '' )  );
#4540=VECTOR ( 'NONE', #1439, 1000.000000000000114 ) ;
#4542=CARTESIAN_POINT ( 'NONE',  ( -17.77761167241057549, -22.25089262147902147, 58.44907471483963946 ) ) ;
#4543=CARTESIAN_POINT ( 'NONE',  ( -20.38775243360237965, -8.467418945486670623, 67.08104087472003130 ) ) ;
#4545=CARTESIAN_POINT ( 'NONE',  ( -10.37795889460693033, -14.56696403379599403, 68.14328054657653411 ) ) ;
#4547=CARTESIAN_POINT ( 'NONE',  ( -24.36611147337434957, -16.04009697885371111, 66.07797069094537790 ) ) ;
#4548=EDGE_CURVE ( 'NONE', #37558, #24279, #45137, .T. ) ;
#4550=( BOUNDED_SURFACE ( )  B_SPLINE_SURFACE ( 3, 1, ( 
 ( #1798, #28395 ),
 ( #16797, #13818 ),
 ( #46858, #43419 ),
 ( #13099, #9685 ),
 ( #28859, #24701 ),
 ( #39706, #2277 ),
 ( #13581, #43903 ) ),
 .UNSPECIFIED., .T., .F., .F. ) 
 B_SPLINE_SURFACE_WITH_KNOTS ( ( 4, 3, 4 ),
 ( 2, 2 ),
 ( 0.000000000000000000, 0.5000000000000000000, 1.000000000000000000 ),
 ( 0.000000000000000000, 1.000000000000000000 ),
 .UNSPECIFIED. ) 
 GEOMETRIC_REPRESENTATION_ITEM ( )  RATIONAL_B_SPLINE_SURFACE ( (
 ( 1.000000000000000000, 1.000000000000000000),
 ( 0.3333333333333335369, 0.3333333333333330373),
 ( 0.3333333333333335369, 0.3333333333333330373),
 ( 1.000000000000000000, 1.000000000000000000),
 ( 0.3333333333333333703, 0.3333333333333333703),
 ( 0.3333333333333333703, 0.3333333333333333703),
 ( 1.000000000000000000, 1.000000000000000000) ) ) 
 REPRESENTATION_ITEM ( '' )  SURFACE ( )  );
#4551=CARTESIAN_POINT ( 'NONE',  ( -21.28537167527045071, -20.64804852447636918, 72.52446480616642077 ) ) ;
#4553=CARTESIAN_POINT ( 'NONE',  ( -24.30112618867181240, -13.25578303422174997, 59.64795780745660636 ) ) ;
#4554=VERTEX_POINT ( 'NONE', #34716 ) ;
#4557=FACE_OUTER_BOUND ( 'NONE', #43608, .T. ) ;
#4558=CARTESIAN_POINT ( 'NONE',  ( -10.93232766038821424, -17.55941949638709687, 68.38249893951126523 ) ) ;
#4559=FACE_OUTER_BOUND ( 'NONE', #10018, .T. ) ;
#4561=CARTESIAN_POINT ( 'NONE',  ( -10.37462440636232053, -14.89569459299594456, 75.09778901493891112 ) ) ;
#4562=EDGE_CURVE ( 'NONE', #45761, #10902, #15648, .T. ) ;
#4564=CARTESIAN_POINT ( 'NONE',  ( -20.87530219893326588, -8.206670134541473871, 59.96312479527349382 ) ) ;
#4566=CARTESIAN_POINT ( 'NONE',  ( -10.33762933896429637, -17.10842426733604782, 57.86477433150147931 ) ) ;
#4568=CARTESIAN_POINT ( 'NONE',  ( -23.55661029900229053, -18.29303667177271464, 72.64879359478229048 ) ) ;
#4569=( BOUNDED_SURFACE ( )  B_SPLINE_SURFACE ( 3, 1, ( 
 ( #42352, #9351 ),
 ( #12068, #12785 ),
 ( #5411, #42107 ),
 ( #16709, #4676 ),
 ( #1213, #38390 ),
 ( #35186, #31750 ),
 ( #8370, #15980 ) ),
 .UNSPECIFIED., .T., .F., .F. ) 
 B_SPLINE_SURFACE_WITH_KNOTS ( ( 4, 3, 4 ),
 ( 2, 2 ),
 ( 0.000000000000000000, 0.5000000000000000000, 1.000000000000000000 ),
 ( 0.000000000000000000, 1.000000000000000000 ),
 .UNSPECIFIED. ) 
 GEOMETRIC_REPRESENTATION_ITEM ( )  RATIONAL_B_SPLINE_SURFACE ( (
 ( 1.000000000000000000, 1.000000000000000000),
 ( 0.3333333333333335369, 0.3333333333333330373),
 ( 0.3333333333333335369, 0.3333333333333330373),
 ( 1.000000000000000000, 1.000000000000000000),
 ( 0.3333333333333333703, 0.3333333333333333703),
 ( 0.3333333333333333703, 0.3333333333333333703),
 ( 1.000000000000000000, 1.000000000000000000) ) ) 
 REPRESENTATION_ITEM ( '' )  SURFACE ( )  );
#4570=CARTESIAN_POINT ( 'NONE',  ( -21.18000274887674905, -20.77541536365158592, 69.05450184741354747 ) ) ;
#4572=DIRECTION ( 'NONE',  ( -0.8651630202045380580, 0.5014907262059380422, 5.433021001366389699E-08 ) ) ;
#4573=CYLINDRICAL_SURFACE ( 'NONE', #41282, 0.1500000000000043243 ) ;
#4574=CARTESIAN_POINT ( 'NONE',  ( -14.66790711817407278, -21.29843871104708342, 58.18089935161520287 ) ) ;
#4575=VERTEX_POINT ( 'NONE', #38893 ) ;
#4576=CARTESIAN_POINT ( 'NONE',  ( -19.77436091090941517, -21.87886160397694368, 65.64981624214608757 ) ) ;
#4577=ORIENTED_EDGE ( 'NONE', *, *, #29192, .F. ) ;
#4578=VECTOR ( 'NONE', #39651, 1000.000000000000114 ) ;
#4579=CARTESIAN_POINT ( 'NONE',  ( -21.47456293661849713, -9.038556783377254433, 70.41660404402310292 ) ) ;
#4580=CARTESIAN_POINT ( 'NONE',  ( -16.79100947509958175, -22.23238548518695268, 68.87277532904636246 ) ) ;
#4581=EDGE_CURVE ( 'NONE', #47078, #1710, #15082, .T. ) ;
#4582=EDGE_LOOP ( 'NONE', ( #39174, #33852, #6507, #13289, #22448 ) ) ;
#4584=AXIS2_PLACEMENT_3D ( 'NONE', #24922, #46848, #2741 ) ;
#4586=ADVANCED_FACE ( 'NONE', ( #5171 ), #26561, .T. ) ;
#4587=FACE_BOUND ( 'NONE', #6456, .T. ) ;
#4588=ORIENTED_EDGE ( 'NONE', *, *, #22141, .F. ) ;
#4589=ORIENTED_EDGE ( 'NONE', *, *, #47198, .F. ) ;
#4591=FACE_OUTER_BOUND ( 'NONE', #26406, .T. ) ;
#4592=B_SPLINE_CURVE_WITH_KNOTS ( 'NONE', 3,
 ( #38436, #22463, #4727, #19749, #15052, #45132, #11377, #26399, #41411, #4470 ),
 .UNSPECIFIED., .F., .F.,
 ( 4, 2, 2, 2, 4 ),
 ( 0.000000000000000000, 0.2499999999999981126, 0.4999999999999962252, 0.7499999999999943379, 1.000000000000000000 ),
 .UNSPECIFIED. ) ;
#4594=FACE_OUTER_BOUND ( 'NONE', #3915, .T. ) ;
#4596=CARTESIAN_POINT ( 'NONE',  ( -10.37352921641884684, -17.21638894027030986, 61.31889622878785673 ) ) ;
#4597=CARTESIAN_POINT ( 'NONE',  ( -20.17268378225416825, -8.371407738384645469, 70.25100341248858626 ) ) ;
#4598=CARTESIAN_POINT ( 'NONE',  ( -19.32724692393761146, -8.072771991737997865, 59.96093028617590903 ) ) ;
#4599=ORIENTED_EDGE ( 'NONE', *, *, #3440, .T. ) ;
#4600=ORIENTED_EDGE ( 'NONE', *, *, #33947, .T. ) ;
#4601=B_SPLINE_CURVE_WITH_KNOTS ( 'NONE', 1,
 ( #5586, #38817 ),
 .UNSPECIFIED., .F., .F.,
 ( 2, 2 ),
 ( 0.000000000000000000, 1.000000000000000000 ),
 .UNSPECIFIED. ) ;
#4603=CARTESIAN_POINT ( 'NONE',  ( -22.54688186880658307, -20.21864567242280941, 65.84275238437966493 ) ) ;
#4604=LINE ( 'NONE', #19624, #27610 ) ;
#4605=CARTESIAN_POINT ( 'NONE',  ( -20.75486715718922781, -8.591426074064321128, 63.61121613145932940 ) ) ;
#4606=ORIENTED_EDGE ( 'NONE', *, *, #16234, .T. ) ;
#4608=ORIENTED_EDGE ( 'NONE', *, *, #13516, .T. ) ;
#4609=CARTESIAN_POINT ( 'NONE',  ( -23.04367355717579713, -10.55211556811382856, 59.90203429191419815 ) ) ;
#4610=CARTESIAN_POINT ( 'NONE',  ( -12.51133688094842888, -19.86980477907010822, 61.28190024782882972 ) ) ;
#4612=CARTESIAN_POINT ( 'NONE',  ( -24.46281123712706673, -17.25067832759902942, 73.06148774291726511 ) ) ;
#4614=ORIENTED_EDGE ( 'NONE', *, *, #22545, .F. ) ;
#4615=CARTESIAN_POINT ( 'NONE',  ( -10.43972881942000086, -15.77115500203794873, 64.52243715390834211 ) ) ;
#4617=ADVANCED_FACE ( 'NONE', ( #45816 ), #16220, .T. ) ;
#4618=CARTESIAN_POINT ( 'NONE',  ( -11.33385179977767265, -19.10019906511433518, 68.26043675633501095 ) ) ;
#4620=EDGE_CURVE ( 'NONE', #46199, #23813, #46804, .T. ) ;
#4621=ORIENTED_EDGE ( 'NONE', *, *, #48585, .T. ) ;
#4622=AXIS2_PLACEMENT_3D ( 'NONE', #37545, #18855, #21815 ) ;
#4623=CARTESIAN_POINT ( 'NONE',  ( -24.64621740481133116, -16.83181165628401033, 47.99999999999994316 ) ) ;
#4624=CARTESIAN_POINT ( 'NONE',  ( -22.87317391125343846, -19.20579927338366133, 58.99483778520830413 ) ) ;
#4626=ORIENTED_EDGE ( 'NONE', *, *, #43652, .T. ) ;
#4627=CARTESIAN_POINT ( 'NONE',  ( -22.04378365035703879, -20.13510231884741231, 62.24911246861644543 ) ) ;
#4628=ORIENTED_EDGE ( 'NONE', *, *, #24534, .T. ) ;
#4629=CARTESIAN_POINT ( 'NONE',  ( -18.50196246566170899, -7.838335838159340874, 70.37067732408392828 ) ) ;
#4630=CARTESIAN_POINT ( 'NONE',  ( -22.00995465109835436, -9.454493699438653920, 59.72171220707129891 ) ) ;
#4632=CARTESIAN_POINT ( 'NONE',  ( -22.22619444978876757, -20.50513558618911958, 58.94938304221643222 ) ) ;
#4633=CARTESIAN_POINT ( 'NONE',  ( -24.47324232082262085, -14.69046401860230766, 62.71856245267908747 ) ) ;
#4634=ORIENTED_EDGE ( 'NONE', *, *, #29266, .F. ) ;
#4635=CARTESIAN_POINT ( 'NONE',  ( -10.66331429883175019, -17.94058386735023802, 71.68062945273115361 ) ) ;
#4637=CARTESIAN_POINT ( 'NONE',  ( -11.95118918738345748, -9.754277919233853567, 60.69771603915999947 ) ) ;
#4639=VERTEX_POINT ( 'NONE', #24374 ) ;
#4640=CARTESIAN_POINT ( 'NONE',  ( -12.15286730501820678, -9.544433317881530598, 57.34581436681493471 ) ) ;
#4641=EDGE_CURVE ( 'NONE', #29512, #45877, #46190, .T. ) ;
#4642=B_SPLINE_CURVE_WITH_KNOTS ( 'NONE', 3,
 ( #48215, #220, #14445, #33663, #26300, #44788, #11040, #7852, #29504, #37115 ),
 .UNSPECIFIED., .F., .F.,
 ( 4, 2, 2, 2, 4 ),
 ( 0.6272669072877827823, 0.7522669073072977275, 0.8772669073268126727, 1.002266907346327507, 1.127266907365842563 ),
 .UNSPECIFIED. ) ;
#4643=CARTESIAN_POINT ( 'NONE',  ( -21.73099075187129614, -8.730192115828774746, 70.31627817507801126 ) ) ;
#4644=EDGE_CURVE ( 'NONE', #43113, #26442, #6848, .T. ) ;
#4645=EDGE_CURVE ( 'NONE', #46252, #9124, #35615, .T. ) ;
#4646=EDGE_CURVE ( 'NONE', #6597, #31450, #22740, .T. ) ;
#4648=ORIENTED_EDGE ( 'NONE', *, *, #39017, .T. ) ;
#4649=LINE ( 'NONE', #476, #24386 ) ;
#4651=B_SPLINE_CURVE_WITH_KNOTS ( 'NONE', 3,
 ( #2847, #25505, #22060, #37058, #17854, #47919, #18345, #48390, #14626, #15372 ),
 .UNSPECIFIED., .F., .F.,
 ( 4, 2, 2, 2, 4 ),
 ( 0.6272669072877907759, 0.7522669073073098289, 0.8772669073268288820, 1.002266907346347935, 1.127266907365866988 ),
 .UNSPECIFIED. ) ;
#4653=CARTESIAN_POINT ( 'NONE',  ( -11.49287318421094817, -18.63485491799402993, 57.96281551145487043 ) ) ;
#4654=( BOUNDED_CURVE ( )  B_SPLINE_CURVE ( 3, ( #36923, #18705, #33712, #6905 ),
 .UNSPECIFIED., .F., .F. ) 
 B_SPLINE_CURVE_WITH_KNOTS ( ( 4, 4 ),
 ( 0.9074455897393653991, 1.000000000000000000 ),
 .UNSPECIFIED. ) 
 CURVE ( )  GEOMETRIC_REPRESENTATION_ITEM ( )  RATIONAL_B_SPLINE_CURVE ( ( 0.6983129098261023904, 0.7760317562607063069, 0.8765941196520055101, 1.000000000000000000 ) ) 
 REPRESENTATION_ITEM ( '' )  );
#4657=CARTESIAN_POINT ( 'NONE',  ( -12.09966231065201825, -10.17612992894743229, 71.11326093460978370 ) ) ;
#4662=EDGE_LOOP ( 'NONE', ( #47175, #30766 ) ) ;
#4665=B_SPLINE_CURVE_WITH_KNOTS ( 'NONE', 1,
 ( #17271, #32317 ),
 .UNSPECIFIED., .F., .F.,
 ( 2, 2 ),
 ( 0.000000000000000000, 1.000000000000000000 ),
 .UNSPECIFIED. ) ;
#4666=CARTESIAN_POINT ( 'NONE',  ( -14.78766009005058812, -21.34800739930362568, 58.45145834864037937 ) ) ;
#4667=CARTESIAN_POINT ( 'NONE',  ( -10.03904597514415009, -13.82694077737217242, 57.56329639008353638 ) ) ;
#4668=ORIENTED_EDGE ( 'NONE', *, *, #26947, .F. ) ;
#4669=VERTEX_POINT ( 'NONE', #47264 ) ;
#4670=EDGE_CURVE ( 'NONE', #29749, #38378, #42094, .T. ) ;
#4671=FACE_OUTER_BOUND ( 'NONE', #364, .T. ) ;
#4672=LINE ( 'NONE', #42602, #38628 ) ;
#4673=CARTESIAN_POINT ( 'NONE',  ( -15.52404113052931223, -21.54652912111637164, 72.04575433027748943 ) ) ;
#4674=VERTEX_POINT ( 'NONE', #40519 ) ;
#4675=CARTESIAN_POINT ( 'NONE',  ( -24.43574572327428740, -14.04659777256190623, 69.53786587444344036 ) ) ;
#4676=CARTESIAN_POINT ( 'NONE',  ( -24.79781851656146330, -15.87314393256401424, 69.64812203948034153 ) ) ;
#4677=ORIENTED_EDGE ( 'NONE', *, *, #40052, .T. ) ;
#4678=ADVANCED_FACE ( 'NONE', ( #6796 ), #18336, .T. ) ;
#4679=VECTOR ( 'NONE', #20307, 999.9999999999998863 ) ;
#4680=B_SPLINE_CURVE_WITH_KNOTS ( 'NONE', 3,
 ( #44821, #18683, #25107, #3937, #11073, #33691, #26096, #22904, #483, #26579 ),
 .UNSPECIFIED., .F., .F.,
 ( 4, 2, 2, 2, 4 ),
 ( 0.6272669072878297447, 0.7522669073073277035, 0.8772669073268255513, 1.002266907346323510, 1.127266907365821469 ),
 .UNSPECIFIED. ) ;
#4681=CARTESIAN_POINT ( 'NONE',  ( -11.10386160987148862, -10.86480171160796893, 57.25257256893876701 ) ) ;
#4682=CARTESIAN_POINT ( 'NONE',  ( -14.13242279744181751, -8.574497162196566435, 74.21426705364891063 ) ) ;
#4683=EDGE_LOOP ( 'NONE', ( #6582, #30249 ) ) ;
#4684=CARTESIAN_POINT ( 'NONE',  ( -20.38226146016681994, -7.971588334861294811, 70.36604906519886526 ) ) ;
#4685=AXIS2_PLACEMENT_3D ( 'NONE', #33503, #36706, #36480 ) ;
#4689=CARTESIAN_POINT ( 'NONE',  ( -20.39277704316526751, -8.469891104483282973, 63.42007541787698699 ) ) ;
#4691=CARTESIAN_POINT ( 'NONE',  ( -13.33151401730585306, -20.55006798877650454, 58.06122216312902395 ) ) ;
#4692=CARTESIAN_POINT ( 'NONE',  ( -24.36611147337434957, -16.04009697885371111, 66.07797069094537790 ) ) ;
#4694=PLANE ( 'NONE',  #3194 ) ;
#4696=( BOUNDED_SURFACE ( )  B_SPLINE_SURFACE ( 3, 1, ( 
 ( #9335, #36376 ),
 ( #43557, #34757 ),
 ( #1698, #24604 ),
 ( #9818, #42156 ),
 ( #16698, #28032 ),
 ( #2170, #31737 ),
 ( #5649, #20657 ) ),
 .UNSPECIFIED., .T., .F., .F. ) 
 B_SPLINE_SURFACE_WITH_KNOTS ( ( 4, 3, 4 ),
 ( 2, 2 ),
 ( 0.000000000000000000, 0.5000000000000000000, 1.000000000000000000 ),
 ( 0.000000000000000000, 1.000000000000000000 ),
 .UNSPECIFIED. ) 
 GEOMETRIC_REPRESENTATION_ITEM ( )  RATIONAL_B_SPLINE_SURFACE ( (
 ( 1.000000000000000000, 1.000000000000000000),
 ( 0.3333333333333335369, 0.3333333333333330373),
 ( 0.3333333333333335369, 0.3333333333333330373),
 ( 1.000000000000000000, 1.000000000000000000),
 ( 0.3333333333333333703, 0.3333333333333333703),
 ( 0.3333333333333333703, 0.3333333333333333703),
 ( 1.000000000000000000, 1.000000000000000000) ) ) 
 REPRESENTATION_ITEM ( '' )  SURFACE ( )  );
#4698=CARTESIAN_POINT ( 'NONE',  ( -17.04413539470110095, -21.84925844046378174, 72.45071136019464575 ) ) ;
#4699=VERTEX_POINT ( 'NONE', #4561 ) ;
#4700=CARTESIAN_POINT ( 'NONE',  ( -19.08084801036773825, -21.61197561877568063, 58.63580559908311329 ) ) ;
#4701=CARTESIAN_POINT ( 'NONE',  ( -13.43773910423563400, -20.62433115109003268, 58.33177939114180788 ) ) ;
#4702=CYLINDRICAL_SURFACE ( 'NONE', #27367, 0.1500000000000020206 ) ;
#4703=CARTESIAN_POINT ( 'NONE',  ( -18.34838239305179641, -21.74803989268259130, 69.11514668064288003 ) ) ;
#4704=CARTESIAN_POINT ( 'NONE',  ( -20.74847848266319161, -20.96993682883388743, 62.39854858292977724 ) ) ;
#4706=ADVANCED_FACE ( 'NONE', ( #41501 ), #6718, .T. ) ;
#4708=ORIENTED_EDGE ( 'NONE', *, *, #6512, .F. ) ;
#4710=CARTESIAN_POINT ( 'NONE',  ( -18.56115164150112662, -7.446410555819776178, 73.88418448558978469 ) ) ;
#4711=LINE ( 'NONE', #527, #12425 ) ;
#4712=ORIENTED_EDGE ( 'NONE', *, *, #38371, .T. ) ;
#4713=CARTESIAN_POINT ( 'NONE',  ( -9.994877497295997060, -15.37525289974553289, 57.75448116320448833 ) ) ;
#4714=DIRECTION ( 'NONE',  ( 0.3824554607245534421, -0.9239739285077093189, 8.917814433895553251E-09 ) ) ;
#4716=DIRECTION ( 'NONE',  ( -0.1648596854219664953, -0.9863170302304249404, 7.074492695208252801E-08 ) ) ;
#4717=CARTESIAN_POINT ( 'NONE',  ( -11.16720114480626336, -11.56054632707691709, 67.61864607954859707 ) ) ;
#4718=CARTESIAN_POINT ( 'NONE',  ( -12.31380156693488992, -10.02538874655004442, 60.85918086676540639 ) ) ;
#4719=( BOUNDED_CURVE ( )  B_SPLINE_CURVE ( 3, ( #47351, #25173, #40190, #6463 ),
 .UNSPECIFIED., .F., .F. ) 
 B_SPLINE_CURVE_WITH_KNOTS ( ( 4, 4 ),
 ( 0.9074455897393634007, 1.000000000000000000 ),
 .UNSPECIFIED. ) 
 CURVE ( )  GEOMETRIC_REPRESENTATION_ITEM ( )  RATIONAL_B_SPLINE_CURVE ( ( 0.6983129098260865142, 0.7760317562606925401, 0.8765941196519970724, 1.000000000000000000 ) ) 
 REPRESENTATION_ITEM ( '' )  );
#4720=CARTESIAN_POINT ( 'NONE',  ( -24.14679772577363437, -12.68507108172156705, 70.05770892828130059 ) ) ;
#4721=VERTEX_POINT ( 'NONE', #7301 ) ;
#4722=EDGE_CURVE ( 'NONE', #25942, #43778, #33427, .T. ) ;
#4723=ADVANCED_FACE ( 'NONE', ( #26484 ), #48561, .T. ) ;
#4727=CARTESIAN_POINT ( 'NONE',  ( -15.58315477633296631, -8.055165212349223225, 74.09602325307160697 ) ) ;
#4728=CARTESIAN_POINT ( 'NONE',  ( -13.84034573514469457, -20.82276458638829553, 68.74008628059695525 ) ) ;
#4729=CARTESIAN_POINT ( 'NONE',  ( -21.38764993922222146, -9.039365983805389249, 70.20420499562830230 ) ) ;
#4730=CARTESIAN_POINT ( 'NONE',  ( -15.92487197799934506, -7.971525956357276677, 67.14007330039670762 ) ) ;
#4731=ORIENTED_EDGE ( 'NONE', *, *, #5334, .F. ) ;
#4736=CARTESIAN_POINT ( 'NONE',  ( -12.01493067177793606, -9.686186367714711309, 60.68201168315654570 ) ) ;
#4737=LINE ( 'NONE', #46343, #21365 ) ;
#4739=VERTEX_POINT ( 'NONE', #34590 ) ;
#4742=CARTESIAN_POINT ( 'NONE',  ( -17.58536440216138885, -7.758048768718602162, 59.96572088198239214 ) ) ;
#4744=CARTESIAN_POINT ( 'NONE',  ( -16.00570185478497010, -7.495462356776134705, 63.77036791188361775 ) ) ;
#4745=CARTESIAN_POINT ( 'NONE',  ( -10.48085305489969521, -13.91959585118948617, 57.74825035244229809 ) ) ;
#4746=ORIENTED_EDGE ( 'NONE', *, *, #24002, .F. ) ;
#4748=CARTESIAN_POINT ( 'NONE',  ( -12.25981284559622075, -20.17899088736047730, 65.04391808465086910 ) ) ;
#4749=ORIENTED_EDGE ( 'NONE', *, *, #17341, .T. ) ;
#4751=CARTESIAN_POINT ( 'NONE',  ( -22.53098214739562621, -20.23350217257768691, 65.89695895308028639 ) ) ;
#4752=CARTESIAN_POINT ( 'NONE',  ( -24.03350017844798003, -12.50343444556183847, 73.25728008851183404 ) ) ;
#4753=ORIENTED_EDGE ( 'NONE', *, *, #8939, .F. ) ;
#4754=CARTESIAN_POINT ( 'NONE',  ( -10.93447185890128992, -11.14999657484283446, 64.28848697573772597 ) ) ;
#4755=CARTESIAN_POINT ( 'NONE',  ( -17.80091866675434886, -21.79911790395781424, 58.69088063202684680 ) ) ;
#4759=CARTESIAN_POINT ( 'NONE',  ( -21.30572535954460633, -21.16897061578360351, 65.69798576082847319 ) ) ;
#4762=CARTESIAN_POINT ( 'NONE',  ( -14.78766009005058635, -21.34800739930362568, 58.45145834864037937 ) ) ;
#4763=PLANE ( 'NONE',  #16337 ) ;
#4764=CARTESIAN_POINT ( 'NONE',  ( -23.92719435707370224, -11.17417392741853988, 70.00715344888816105 ) ) ;
#4765=CARTESIAN_POINT ( 'NONE',  ( -10.47679690896004701, -15.67958946752583138, 64.61844751979357682 ) ) ;
#4767=ADVANCED_FACE ( 'NONE', ( #876 ), #18852, .F. ) ;
#4769=CARTESIAN_POINT ( 'NONE',  ( -14.05371270701021302, -21.00138147690670820, 71.92607703580544865 ) ) ;
#4770=CARTESIAN_POINT ( 'NONE',  ( -10.45662601068241848, -17.44683468735947685, 64.72765127533203611 ) ) ;
#4771=VERTEX_POINT ( 'NONE', #39511 ) ;
#4772=CARTESIAN_POINT ( 'NONE',  ( -15.62222905942471840, -7.993050613273783966, 70.89517703929612935 ) ) ;
#4774=CARTESIAN_POINT ( 'NONE',  ( -21.59671027634132656, -20.98115415594247324, 72.56800473755950520 ) ) ;
#4775=CARTESIAN_POINT ( 'NONE',  ( -22.78195790197552384, -10.22153446486525219, 63.28005797477638339 ) ) ;
#4776=CARTESIAN_POINT ( 'NONE',  ( -22.72031779163844334, -16.29245029320677673, 53.49899999999994549 ) ) ;
#4777=ORIENTED_EDGE ( 'NONE', *, *, #15308, .F. ) ;
#4778=FACE_OUTER_BOUND ( 'NONE', #47645, .T. ) ;
#4779=EDGE_CURVE ( 'NONE', #27411, #23020, #20373, .T. ) ;
#4780=CARTESIAN_POINT ( 'NONE',  ( -24.02655296236175175, -11.35792967378293916, 66.53719098615387395 ) ) ;
#4781=ORIENTED_EDGE ( 'NONE', *, *, #38218, .F. ) ;
#4782=DIRECTION ( 'NONE',  ( 0.05202058437830281434, -0.9986460127597465153, 1.657953767687799911E-08 ) ) ;
#4783=EDGE_CURVE ( 'NONE', #29219, #1317, #16762, .T. ) ;
#4785=LINE ( 'NONE', #366, #21668 ) ;
#4786=CARTESIAN_POINT ( 'NONE',  ( -10.02134419679888211, -13.96483583313674615, 61.10476640098193002 ) ) ;
#4787=CARTESIAN_POINT ( 'NONE',  ( -21.71931446036287028, -8.721835193296540112, 70.29165865351603770 ) ) ;
#4789=ORIENTED_EDGE ( 'NONE', *, *, #40163, .T. ) ;
#4790=ORIENTED_EDGE ( 'NONE', *, *, #47039, .F. ) ;
#4793=CARTESIAN_POINT ( 'NONE',  ( -13.43921731646364925, -8.993429882417945720, 60.43950277494440115 ) ) ;
#4795=CARTESIAN_POINT ( 'NONE',  ( -23.39838849549200717, -11.16098491156533257, 73.66193259096606027 ) ) ;
#4796=VECTOR ( 'NONE', #30248, 1000.000000000000227 ) ;
#4798=CARTESIAN_POINT ( 'NONE',  ( -17.70936732686351789, -22.25382107568847800, 58.66199285276312025 ) ) ;
#4799=CARTESIAN_POINT ( 'NONE',  ( -20.66848101912799862, -8.549761622307151754, 60.12653141481577990 ) ) ;
#4800=CARTESIAN_POINT ( 'NONE',  ( -14.37051197998799523, -8.445983692038035784, 74.34387349308116200 ) ) ;
#4801=VECTOR ( 'NONE', #38315, 1000.000000000000114 ) ;
#4802=CARTESIAN_POINT ( 'NONE',  ( -18.18338144371267617, -21.81849904615365432, 65.63060065626805795 ) ) ;
#4803=B_SPLINE_CURVE_WITH_KNOTS ( 'NONE', 1,
 ( #23074, #41781 ),
 .UNSPECIFIED., .F., .F.,
 ( 2, 2 ),
 ( 0.000000000000000000, 1.000000000000000000 ),
 .UNSPECIFIED. ) ;
#4804=VERTEX_POINT ( 'NONE', #9487 ) ;
#4805=CARTESIAN_POINT ( 'NONE',  ( -21.41781370759021641, -8.989828079956971862, 66.81716936885602820 ) ) ;
#4809=CARTESIAN_POINT ( 'NONE',  ( -15.09544287645192462, -21.46351977604527761, 65.10596681500476279 ) ) ;
#4810=EDGE_LOOP ( 'NONE', ( #17739, #8246, #7110, #6499, #19607 ) ) ;
#4811=DIRECTION ( 'NONE',  ( 0.04287186434519785205, 0.9990805789562556827, -2.806673972535358096E-09 ) ) ;
#4814=EDGE_CURVE ( 'NONE', #3385, #38648, #7737, .T. ) ;
#4815=B_SPLINE_CURVE_WITH_KNOTS ( 'NONE', 1,
 ( #472, #41839 ),
 .UNSPECIFIED., .F., .F.,
 ( 2, 2 ),
 ( 0.000000000000000000, 1.000000000000000000 ),
 .UNSPECIFIED. ) ;
#4816=CARTESIAN_POINT ( 'NONE',  ( -21.35994700726987006, -8.956524206332462157, 70.01643677269403554 ) ) ;
#4817=CARTESIAN_POINT ( 'NONE',  ( -24.49273639735834607, -17.16277907914581036, 73.04369411581572535 ) ) ;
#4819=CARTESIAN_POINT ( 'NONE',  ( -13.99679447977218061, -20.97040113148658591, 71.94079819673058296 ) ) ;
#4822=FACE_BOUND ( 'NONE', #34508, .T. ) ;
#4825=CARTESIAN_POINT ( 'NONE',  ( -22.82696774913247495, -10.28001814127269320, 66.54742050011650178 ) ) ;
#4828=CARTESIAN_POINT ( 'NONE',  ( -11.07857809310684516, -11.73724795245126096, 71.38860870961248395 ) ) ;
#4829=VERTEX_POINT ( 'NONE', #27216 ) ;
#4830=DIRECTION ( 'NONE',  ( -5.731567514496413899E-31, -1.020425574103664789E-16, -1.000000000000000000 ) ) ;
#4831=ORIENTED_EDGE ( 'NONE', *, *, #46898, .F. ) ;
#4832=CARTESIAN_POINT ( 'NONE',  ( -20.10030204730919223, -21.76202525863913451, 72.51983304728076973 ) ) ;
#4833=ORIENTED_EDGE ( 'NONE', *, *, #11798, .T. ) ;
#4836=CARTESIAN_POINT ( 'NONE',  ( -20.16798188746241394, -8.311166627122801742, 66.98924058670168336 ) ) ;
#4837=B_SPLINE_CURVE_WITH_KNOTS ( 'NONE', 3,
 ( #26926, #30384, #38721, #1058, #46366, #19283, #23000, #19782, #16055, #31096 ),
 .UNSPECIFIED., .F., .F.,
 ( 4, 2, 2, 2, 4 ),
 ( 0.6272669072877714580, 0.7522669073072920654, 0.8772669073268126727, 1.002266907346333280, 1.127266907365853887 ),
 .UNSPECIFIED. ) ;
#4838=ORIENTED_EDGE ( 'NONE', *, *, #42891, .F. ) ;
#4840=ORIENTED_EDGE ( 'NONE', *, *, #15217, .F. ) ;
#4842=LINE ( 'NONE', #35352, #6051 ) ;
#4843=B_SPLINE_CURVE_WITH_KNOTS ( 'NONE', 3,
 ( #10362, #36192, #32514, #25372, #43858, #40383, #10112, #26102, #11081, #32971 ),
 .UNSPECIFIED., .F., .F.,
 ( 4, 2, 2, 2, 4 ),
 ( 0.6272669072782827149, 0.7522669073001686524, 0.8772669073220544789, 1.002266907343940527, 1.127266907365826354 ),
 .UNSPECIFIED. ) ;
#4846=CARTESIAN_POINT ( 'NONE',  ( -24.43617598160173543, -14.07860879870782966, 73.12271522640413934 ) ) ;
#4847=( BOUNDED_CURVE ( )  B_SPLINE_CURVE ( 3, ( #20285, #42457, #23499, #35047 ),
 .UNSPECIFIED., .F., .F. ) 
 B_SPLINE_CURVE_WITH_KNOTS ( ( 4, 4 ),
 ( 0.5000000000000000000, 0.9074455897393657322 ),
 .UNSPECIFIED. ) 
 CURVE ( )  GEOMETRIC_REPRESENTATION_ITEM ( )  RATIONAL_B_SPLINE_CURVE ( ( 1.000000000000004663, 0.4567392136813346326, 0.3561768502900279909, 0.6983129098260896228 ) ) 
 REPRESENTATION_ITEM ( '' )  );
#4848=CARTESIAN_POINT ( 'NONE',  ( -14.56922799437018057, -8.416425268799397230, 67.33145281372107149 ) ) ;
#4849=CARTESIAN_POINT ( 'NONE',  ( -10.68551981713787136, -12.73596763222149519, 64.28308208171728211 ) ) ;
#4850=CARTESIAN_POINT ( 'NONE',  ( -10.50429924535250414, -16.15944446069506668, 71.46222527016213633 ) ) ;
#4851=ORIENTED_EDGE ( 'NONE', *, *, #29922, .F. ) ;
#4852=ORIENTED_EDGE ( 'NONE', *, *, #23913, .F. ) ;
#4853=EDGE_CURVE ( 'NONE', #9098, #6412, #12695, .T. ) ;
#4856=CARTESIAN_POINT ( 'NONE',  ( -21.62450594022013206, -20.48119921038467695, 72.68013252948732372 ) ) ;
#4857=CARTESIAN_POINT ( 'NONE',  ( -10.52311447087272178, -15.98309989773700046, 67.97767878683296772 ) ) ;
#4858=FACE_BOUND ( 'NONE', #7355, .T. ) ;
#4861=( BOUNDED_CURVE ( )  B_SPLINE_CURVE ( 3, ( #45353, #34741, #4962, #15277 ),
 .UNSPECIFIED., .F., .F. ) 
 B_SPLINE_CURVE_WITH_KNOTS ( ( 4, 4 ),
 ( 0.5000000000000000000, 0.9074455897393634007 ),
 .UNSPECIFIED. ) 
 CURVE ( )  GEOMETRIC_REPRESENTATION_ITEM ( )  RATIONAL_B_SPLINE_CURVE ( ( 1.000000000000004663, 0.4567392136813371861, 0.3561768502900288791, 0.6983129098260848489 ) ) 
 REPRESENTATION_ITEM ( '' )  );
#4863=( BOUNDED_CURVE ( )  B_SPLINE_CURVE ( 3, ( #22118, #32696, #48203, #37106 ),
 .UNSPECIFIED., .F., .F. ) 
 B_SPLINE_CURVE_WITH_KNOTS ( ( 4, 4 ),
 ( 0.5000000000000000000, 0.9074455897393647330 ),
 .UNSPECIFIED. ) 
 CURVE ( )  GEOMETRIC_REPRESENTATION_ITEM ( )  RATIONAL_B_SPLINE_CURVE ( ( 0.9999999999999874545, 0.4567392136813364645, 0.3561768502900406475, 0.6983129098260862921 ) ) 
 REPRESENTATION_ITEM ( '' )  );
#4864=ORIENTED_EDGE ( 'NONE', *, *, #8322, .T. ) ;
#4865=AXIS2_PLACEMENT_3D ( 'NONE', #43262, #9529, #5829 ) ;
#4866=DIRECTION ( 'NONE',  ( -2.671295504230222649E-06, -1.272698190446629743E-05, -0.9999999999154440822 ) ) ;
#4868=VECTOR ( 'NONE', #4186, 1000.000000000000114 ) ;
#4869=CARTESIAN_POINT ( 'NONE',  ( -12.51438871980625045, -19.79882953766492193, 65.16674880260835323 ) ) ;
#4870=VERTEX_POINT ( 'NONE', #24020 ) ;
#4871=CARTESIAN_POINT ( 'NONE',  ( -12.27729936708703384, -9.991218733798060470, 60.70918086709614414 ) ) ;
#4872=( BOUNDED_SURFACE ( )  B_SPLINE_SURFACE ( 3, 1, ( 
 ( #11249, #26260 ),
 ( #45475, #11484 ),
 ( #18873, #33885 ),
 ( #31351, #16561 ),
 ( #44750, #7815 ),
 ( #20030, #38737 ),
 ( #23744, #5021 ) ),
 .UNSPECIFIED., .T., .F., .F. ) 
 B_SPLINE_SURFACE_WITH_KNOTS ( ( 4, 3, 4 ),
 ( 2, 2 ),
 ( 0.000000000000000000, 0.5000000000000000000, 1.000000000000000000 ),
 ( 0.000000000000000000, 1.000000000000000000 ),
 .UNSPECIFIED. ) 
 GEOMETRIC_REPRESENTATION_ITEM ( )  RATIONAL_B_SPLINE_SURFACE ( (
 ( 1.000000000000000000, 1.000000000000000000),
 ( 0.3333333333333335369, 0.3333333333333330373),
 ( 0.3333333333333335369, 0.3333333333333330373),
 ( 1.000000000000000000, 1.000000000000000000),
 ( 0.3333333333333333703, 0.3333333333333333703),
 ( 0.3333333333333333703, 0.3333333333333333703),
 ( 1.000000000000000000, 1.000000000000000000) ) ) 
 REPRESENTATION_ITEM ( '' )  SURFACE ( )  );
#4873=CARTESIAN_POINT ( 'NONE',  ( -10.42394424466950476, -17.36098423042032124, 64.81394647623933736 ) ) ;
#4874=CARTESIAN_POINT ( 'NONE',  ( -12.10369346210734243, -9.594120923840563364, 57.27430859790474926 ) ) ;
#4877=CARTESIAN_POINT ( 'NONE',  ( -10.44050839523226060, -15.30664602827292775, 57.79622666356080174 ) ) ;
#4878=ADVANCED_FACE ( 'NONE', ( #8998 ), #19838, .T. ) ;
#4879=CARTESIAN_POINT ( 'NONE',  ( -24.82398108165943285, -15.67291706594333611, 73.18116521566574306 ) ) ;
#4881=ORIENTED_EDGE ( 'NONE', *, *, #5603, .F. ) ;
#4882=CARTESIAN_POINT ( 'NONE',  ( -15.95707209241614422, -7.504986913482371236, 63.85506412386598640 ) ) ;
#4883=ORIENTED_EDGE ( 'NONE', *, *, #32459, .F. ) ;
#4884=CARTESIAN_POINT ( 'NONE',  ( -9.974335981654279593, -14.73511362144080294, 71.50499609704121440 ) ) ;
#4885=CARTESIAN_POINT ( 'NONE',  ( -24.32886716615087153, -16.23426984194678724, 62.60800820172418923 ) ) ;
#4886=VERTEX_POINT ( 'NONE', #5296 ) ;
#4887=CARTESIAN_POINT ( 'NONE',  ( -20.54979551517892489, -8.489990701729437816, 63.31121512946744190 ) ) ;
#4889=CARTESIAN_POINT ( 'NONE',  ( -23.80338573481879294, -11.80731802715296297, 59.76763678108634537 ) ) ;
#4892=CARTESIAN_POINT ( 'NONE',  ( -10.63483670088760924, -17.87674068094334245, 71.75213521449022380 ) ) ;
#4893=CARTESIAN_POINT ( 'NONE',  ( -15.19549097431359463, -21.91815212410659086, 68.76088336006283441 ) ) ;
#4894=DIRECTION ( 'NONE',  ( -0.7621627669932626858, 0.6473854467078884456, -3.680865981908973010E-08 ) ) ;
#4896=ORIENTED_EDGE ( 'NONE', *, *, #11648, .T. ) ;
#4897=ADVANCED_FACE ( 'NONE', ( #31390 ), #1595, .T. ) ;
#4899=CARTESIAN_POINT ( 'NONE',  ( -11.10470733248389230, -18.75498039752055490, 61.46206112672981448 ) ) ;
#4900=EDGE_LOOP ( 'NONE', ( #46167, #32168 ) ) ;
#4901=ORIENTED_EDGE ( 'NONE', *, *, #28234, .T. ) ;
#4903=FACE_OUTER_BOUND ( 'NONE', #23086, .T. ) ;
#4904=CARTESIAN_POINT ( 'NONE',  ( -10.20016939456313843, -12.98476690782802834, 71.39483965270750332 ) ) ;
#4905=FACE_OUTER_BOUND ( 'NONE', #41395, .T. ) ;
#4909=CARTESIAN_POINT ( 'NONE',  ( -12.36152504943391506, -19.64358911433177823, 58.15355758026139199 ) ) ;
#4910=CARTESIAN_POINT ( 'NONE',  ( -10.71953686386422788, -16.98946087901043001, 57.98200754419831782 ) ) ;
#4911=CARTESIAN_POINT ( 'NONE',  ( -9.975178868143471433, -14.94333879318065428, 74.91966125157830447 ) ) ;
#4914=ADVANCED_FACE ( 'NONE', ( #42962 ), #9238, .T. ) ;
#4915=CARTESIAN_POINT ( 'NONE',  ( -21.55883939963115026, -8.611815437115641458, 73.78624134823098757 ) ) ;
#4917=ADVANCED_FACE ( 'NONE', ( #47629 ), #37912, .T. ) ;
#4918=CARTESIAN_POINT ( 'NONE',  ( -11.90143264907557707, -10.50540407141871668, 74.54958359901495157 ) ) ;
#4919=CARTESIAN_POINT ( 'NONE',  ( -13.65684165595416921, -8.849801312179289781, 56.98439896120441261 ) ) ;
#4920=EDGE_CURVE ( 'NONE', #18177, #16383, #2735, .T. ) ;
#4921=CARTESIAN_POINT ( 'NONE',  ( -21.92783717115298359, -9.450287623791650660, 59.72171200097150745 ) ) ;
#4922=B_SPLINE_CURVE_WITH_KNOTS ( 'NONE', 3,
 ( #36168, #17696, #13754, #32723, #18423, #14235, #47750, #44319, #3418, #10338 ),
 .UNSPECIFIED., .F., .F.,
 ( 4, 2, 2, 2, 4 ),
 ( 0.1272669073658479755, 0.2522669073439446352, 0.3772669073220412672, 0.5022669073001380102, 0.6272669072782346422 ),
 .UNSPECIFIED. ) ;
#4923=EDGE_LOOP ( 'NONE', ( #30848, #1354, #7789, #30467, #1364 ) ) ;
#4924=B_SPLINE_CURVE_WITH_KNOTS ( 'NONE', 3,
 ( #2844, #33348, #17853, #29204, #25503, #29686, #32875, #41015, #10976, #26236 ),
 .UNSPECIFIED., .F., .F.,
 ( 4, 2, 2, 2, 4 ),
 ( 0.000000000000000000, 0.2500000000000000000, 0.5000000000000000000, 0.7500000000000000000, 1.000000000000000000 ),
 .UNSPECIFIED. ) ;
#4926=CARTESIAN_POINT ( 'NONE',  ( -24.47535868512742496, -14.65268306083313199, 66.59781357586173556 ) ) ;
#4928=CARTESIAN_POINT ( 'NONE',  ( -11.05969852021412869, -18.68212028911960232, 61.43857375368525453 ) ) ;
#4930=ORIENTED_EDGE ( 'NONE', *, *, #43440, .T. ) ;
#4932=CARTESIAN_POINT ( 'NONE',  ( -12.99758330771203951, -9.386476247090117297, 70.84925353123610137 ) ) ;
#4935=EDGE_CURVE ( 'NONE', #41932, #891, #6297, .T. ) ;
#4936=ORIENTED_EDGE ( 'NONE', *, *, #23398, .F. ) ;
#4938=CARTESIAN_POINT ( 'NONE',  ( -22.10541328151775886, -20.01527608457440266, 65.93251542687603717 ) ) ;
#4939=ORIENTED_EDGE ( 'NONE', *, *, #1843, .F. ) ;
#4940=CARTESIAN_POINT ( 'NONE',  ( -11.75774308769439003, -19.00384223356172697, 71.98685884781657762 ) ) ;
#4942=CARTESIAN_POINT ( 'NONE',  ( -18.53201889041905659, -7.846807422456379300, 73.99064401781672018 ) ) ;
#4943=CARTESIAN_POINT ( 'NONE',  ( -21.61680475328812889, -8.650891705389904374, 73.85774703147257014 ) ) ;
#4944=ORIENTED_EDGE ( 'NONE', *, *, #32394, .T. ) ;
#4945=CARTESIAN_POINT ( 'NONE',  ( -24.84806299871600643, -14.18603056061780343, 69.69629353939886585 ) ) ;
#4949=( BOUNDED_CURVE ( )  B_SPLINE_CURVE ( 3, ( #5563, #20579, #35574, #1852 ),
 .UNSPECIFIED., .F., .F. ) 
 B_SPLINE_CURVE_WITH_KNOTS ( ( 4, 4 ),
 ( 1.570796326794896558, 1.780235837034217505 ),
 .UNSPECIFIED. ) 
 CURVE ( )  GEOMETRIC_REPRESENTATION_ITEM ( )  RATIONAL_B_SPLINE_CURVE ( ( 1.000000000000000000, 0.9963479302455154896, 0.9963479302455154896, 1.000000000000000000 ) ) 
 REPRESENTATION_ITEM ( '' )  );
#4950=CARTESIAN_POINT ( 'NONE',  ( -10.53392471227544114, -17.64261015482012596, 68.29733140449641837 ) ) ;
#4951=CARTESIAN_POINT ( 'NONE',  ( -16.97945985512182787, -21.84517132341290591, 72.16543221430227106 ) ) ;
#4952=ORIENTED_EDGE ( 'NONE', *, *, #45619, .F. ) ;
#4955=DIRECTION ( 'NONE',  ( -6.516572651863732626E-06, 8.834921937557814562E-06, 0.9999999999397393147 ) ) ;
#4957=FACE_OUTER_BOUND ( 'NONE', #45369, .T. ) ;
#4958=ADVANCED_FACE ( 'NONE', ( #47867 ), #26274, .T. ) ;
#4959=EDGE_LOOP ( 'NONE', ( #1996, #27566 ) ) ;
#4960=ORIENTED_EDGE ( 'NONE', *, *, #3403, .T. ) ;
#4962=CARTESIAN_POINT ( 'NONE',  ( -12.03360233570622739, -10.25976192134970866, 71.26893272426330839 ) ) ;
#4963=ORIENTED_EDGE ( 'NONE', *, *, #16541, .T. ) ;
#4964=CARTESIAN_POINT ( 'NONE',  ( -22.43322805121811214, -20.32484237088842249, 65.89077003248591780 ) ) ;
#4966=CARTESIAN_POINT ( 'NONE',  ( -10.46764514157213455, -15.58883556682774874, 57.67678839390069356 ) ) ;
#4967=CARTESIAN_POINT ( 'NONE',  ( -10.63483670088760924, -17.87674068094334245, 71.75213521449022380 ) ) ;
#4969=CARTESIAN_POINT ( 'NONE',  ( -19.39825701701550287, -7.625522893467396202, 60.16081771123726440 ) ) ;
#4970=ORIENTED_EDGE ( 'NONE', *, *, #40500, .F. ) ;
#4972=CARTESIAN_POINT ( 'NONE',  ( -22.63560595208270954, -20.13310736574185000, 69.28922662766110818 ) ) ;
#4973=CARTESIAN_POINT ( 'NONE',  ( -19.17604249790256077, -21.63836284480991878, 58.53979515915469278 ) ) ;
#4974=CARTESIAN_POINT ( 'NONE',  ( -22.62394951084894146, -10.04809318868971424, 70.29706442286226320 ) ) ;
#4976=CARTESIAN_POINT ( 'NONE',  ( -12.72909403660860228, -20.00294204248303132, 72.03483503000991561 ) ) ;
#4977=B_SPLINE_CURVE_WITH_KNOTS ( 'NONE', 3,
 ( #45594, #11845, #26872, #42853, #16723, #1961, #5906, #46558, #12799, #19957 ),
 .UNSPECIFIED., .F., .F.,
 ( 4, 2, 2, 2, 4 ),
 ( 0.000000000000000000, 0.2500000000000000000, 0.5000000000000000000, 0.7500000000000000000, 1.000000000000000000 ),
 .UNSPECIFIED. ) ;
#4978=EDGE_LOOP ( 'NONE', ( #25522, #46717, #10806, #4901, #36560 ) ) ;
#4979=ORIENTED_EDGE ( 'NONE', *, *, #48622, .F. ) ;
#4981=VERTEX_POINT ( 'NONE', #14101 ) ;
#4982=FACE_OUTER_BOUND ( 'NONE', #27478, .T. ) ;
#4983=DIRECTION ( 'NONE',  ( -9.632611953450936153E-07, 3.816342149705755051E-07, 0.9999999999994632072 ) ) ;
#4987=CARTESIAN_POINT ( 'NONE',  ( -11.22844613476422460, -11.44458948612160043, 64.43409918096024569 ) ) ;
#4988=EDGE_CURVE ( 'NONE', #40480, #18094, #817, .T. ) ;
#4992=CARTESIAN_POINT ( 'NONE',  ( -18.09515488393238414, -21.82723660550677636, 65.34532171799240530 ) ) ;
#4993=DIRECTION ( 'NONE',  ( -0.2393306345705715765, -0.3777841279832278021, 0.8944271909999157444 ) ) ;
#4994=ORIENTED_EDGE ( 'NONE', *, *, #43497, .F. ) ;
#4996=DIRECTION ( 'NONE',  ( 3.549360974554993999E-17, -6.371834667797928663E-18, -1.000000000000000000 ) ) ;
#4997=ORIENTED_EDGE ( 'NONE', *, *, #39785, .F. ) ;
#4998=EDGE_CURVE ( 'NONE', #2922, #41672, #42951, .T. ) ;
#4999=EDGE_CURVE ( 'NONE', #33324, #46845, #34286, .T. ) ;
#5000=CARTESIAN_POINT ( 'NONE',  ( -23.00190342510993347, -19.12578814502481350, 62.76895730438863552 ) ) ;
#5001=CARTESIAN_POINT ( 'NONE',  ( -22.23721589179859492, -20.49593378876094718, 58.92476249817150347 ) ) ;
#5003=VERTEX_POINT ( 'NONE', #45652 ) ;
#5005=CARTESIAN_POINT ( 'NONE',  ( -21.68495691188242702, -20.43592993620880804, 58.90875877921045145 ) ) ;
#5006=CARTESIAN_POINT ( 'NONE',  ( -14.81535805098777736, -7.777528402031248511, 47.99999999999994316 ) ) ;
#5007=CARTESIAN_POINT ( 'NONE',  ( -20.72253465480533308, -21.04901898548487793, 65.72887014617839441 ) ) ;
#5008=B_SPLINE_CURVE_WITH_KNOTS ( 'NONE', 3,
 ( #24232, #13597, #39969, #17300, #1811, #9209, #16574, #6239, #5764, #2051 ),
 .UNSPECIFIED., .F., .F.,
 ( 4, 2, 2, 2, 4 ),
 ( 0.1272669073658179995, 0.2522669073463016942, 0.3772669073267853612, 0.5022669073072690837, 0.6272669072877528063 ),
 .UNSPECIFIED. ) ;
#5009=CARTESIAN_POINT ( 'NONE',  ( -10.96921284960095377, -11.97350354382807680, 74.84368195529052059 ) ) ;
#5011=( BOUNDED_CURVE ( )  B_SPLINE_CURVE ( 3, ( #22749, #8441, #37488, #19523 ),
 .UNSPECIFIED., .F., .F. ) 
 B_SPLINE_CURVE_WITH_KNOTS ( ( 4, 4 ),
 ( 0.4074455897393670090, 0.5000000000000000000 ),
 .UNSPECIFIED. ) 
 CURVE ( )  GEOMETRIC_REPRESENTATION_ITEM ( )  RATIONAL_B_SPLINE_CURVE ( ( 0.6983129098260917322, 0.7760317562606943165, 0.8765941196519962952, 0.9999999999999956701 ) ) 
 REPRESENTATION_ITEM ( '' )  );
#5012=CARTESIAN_POINT ( 'NONE',  ( -10.39634573379212767, -15.41385649924959544, 61.33789215671617967 ) ) ;
#5013=CARTESIAN_POINT ( 'NONE',  ( -20.16691314815865255, -21.73601827195274794, 72.58974169946205279 ) ) ;
#5016=EDGE_LOOP ( 'NONE', ( #16870, #20143, #8141, #34815, #36800 ) ) ;
#5017=CARTESIAN_POINT ( 'NONE',  ( -21.84079957929829874, -9.314189696129256291, 63.19153755727188582 ) ) ;
#5018=CARTESIAN_POINT ( 'NONE',  ( -12.50776634899986384, -20.40684016789016297, 71.92158251742569064 ) ) ;
#5019=EDGE_LOOP ( 'NONE', ( #15002, #37109, #24074, #47920, #12714 ) ) ;
#5020=FACE_OUTER_BOUND ( 'NONE', #48369, .T. ) ;
#5021=CARTESIAN_POINT ( 'NONE',  ( -14.41428275390769365, -7.994163218335415877, 63.97474169571218283 ) ) ;
#5023=CARTESIAN_POINT ( 'NONE',  ( -12.27729925481933471, -9.991218852276041673, 60.55918086709623083 ) ) ;
#5024=CYLINDRICAL_SURFACE ( 'NONE', #48616, 0.1499999999999971634 ) ;
#5025=ORIENTED_EDGE ( 'NONE', *, *, #44136, .F. ) ;
#5027=CARTESIAN_POINT ( 'NONE',  ( -24.42421134999058552, -14.80068637069104653, 59.54300242294779366 ) ) ;
#5028=CARTESIAN_POINT ( 'NONE',  ( -10.09536215149225491, -16.14886288462728459, 68.11621278793219858 ) ) ;
#5029=VERTEX_POINT ( 'NONE', #37986 ) ;
#5032=CARTESIAN_POINT ( 'NONE',  ( -12.76547314785493192, -9.517330534081262172, 74.60450883341005124 ) ) ;
#5036=ORIENTED_EDGE ( 'NONE', *, *, #47835, .T. ) ;
#5038=CARTESIAN_POINT ( 'NONE',  ( -10.74573065459234478, -12.54952415110468422, 60.81325645027152405 ) ) ;
#5039=CARTESIAN_POINT ( 'NONE',  ( -14.11538500997439627, -8.134069317748153338, 70.86924253296322718 ) ) ;
#5040=CARTESIAN_POINT ( 'NONE',  ( -17.04413539470110095, -21.84925844046378174, 72.45071136019464575 ) ) ;
#5041=ADVANCED_FACE ( 'NONE', ( #45165 ), #41203, .T. ) ;
#5042=CARTESIAN_POINT ( 'NONE',  ( -15.53265176333180619, -21.60105060138385369, 72.33103357390284316 ) ) ;
#5044=CARTESIAN_POINT ( 'NONE',  ( -14.01837044221388595, -8.636059239884618322, 74.48482605064899076 ) ) ;
#5045=FACE_OUTER_BOUND ( 'NONE', #44134, .T. ) ;
#5047=CARTESIAN_POINT ( 'NONE',  ( -22.43986228125061544, -19.69212616369310354, 69.24706122172230494 ) ) ;
#5049=AXIS2_PLACEMENT_3D ( 'NONE', #15588, #11927, #29910 ) ;
#5050=( BOUNDED_CURVE ( )  B_SPLINE_CURVE ( 3, ( #37382, #14061, #15224, #32562 ),
 .UNSPECIFIED., .F., .F. ) 
 B_SPLINE_CURVE_WITH_KNOTS ( ( 4, 4 ),
 ( 1.570796326794896558, 1.780235837034217505 ),
 .UNSPECIFIED. ) 
 CURVE ( )  GEOMETRIC_REPRESENTATION_ITEM ( )  RATIONAL_B_SPLINE_CURVE ( ( 1.000000000000000000, 0.9963479302455154896, 0.9963479302455154896, 1.000000000000000000 ) ) 
 REPRESENTATION_ITEM ( '' )  );
#5051=ORIENTED_EDGE ( 'NONE', *, *, #2452, .F. ) ;
#5054=CARTESIAN_POINT ( 'NONE',  ( -10.80730693270912468, -17.26544268483686650, 57.84327589213576459 ) ) ;
#5055=CARTESIAN_POINT ( 'NONE',  ( -20.31443949084103906, -8.433657969208125493, 67.08104076698165841 ) ) ;
#5056=VERTEX_POINT ( 'NONE', #19281 ) ;
#5057=CARTESIAN_POINT ( 'NONE',  ( -14.03870967672415304, -8.172720116890397790, 70.91453050697840865 ) ) ;
#5060=CARTESIAN_POINT ( 'NONE',  ( -10.00761947527410634, -15.51609109068450465, 57.75288224187332276 ) ) ;
#5061=ADVANCED_FACE ( 'NONE', ( #30629 ), #18290, .T. ) ;
#5062=CARTESIAN_POINT ( 'NONE',  ( -21.78913871579879569, -8.771809629715434653, 70.24637254705723421 ) ) ;
#5063=CARTESIAN_POINT ( 'NONE',  ( -24.46683668533210110, -14.41599144169055258, 62.71296521563537141 ) ) ;
#5066=CARTESIAN_POINT ( 'NONE',  ( -22.96375064570672819, -10.44813988596692589, 63.08658113699938497 ) ) ;
#5067=CARTESIAN_POINT ( 'NONE',  ( -10.90414816633800399, -11.20463157964466205, 64.24858404949443980 ) ) ;
#5071=DIRECTION ( 'NONE',  ( 0.6478992145799702396, -0.7617260713318518839, 1.927832152310587483E-08 ) ) ;
#5072=EDGE_CURVE ( 'NONE', #10114, #18224, #21251, .T. ) ;
#5073=CARTESIAN_POINT ( 'NONE',  ( -24.40658499505740053, -15.78250870199476630, 69.83307488408829045 ) ) ;
#5075=CARTESIAN_POINT ( 'NONE',  ( -10.71495605983455590, -12.81234157828920850, 64.26836111193937029 ) ) ;
#5076=EDGE_LOOP ( 'NONE', ( #34521, #6510 ) ) ;
#5077=CARTESIAN_POINT ( 'NONE',  ( -19.85891393954322837, -21.37210614461000446, 47.99999999999994316 ) ) ;
#5078=CARTESIAN_POINT ( 'NONE',  ( -14.65765131015531253, -21.78034674156931061, 47.99999999999994316 ) ) ;
#5079=ORIENTED_EDGE ( 'NONE', *, *, #21021, .T. ) ;
#5080=DIRECTION ( 'NONE',  ( 0.9862050927915948506, 0.1655279884246635136, 7.765682856207885122E-08 ) ) ;
#5081=FACE_BOUND ( 'NONE', #1218, .T. ) ;
#5083=VERTEX_POINT ( 'NONE', #14821 ) ;
#5085=CARTESIAN_POINT ( 'NONE',  ( -10.02191638112385697, -15.65273889608829982, 61.15293747381159761 ) ) ;
#5086=B_SPLINE_CURVE_WITH_KNOTS ( 'NONE', 3,
 ( #20985, #2269, #13808, #24456, #31827, #43157, #39459, #5742, #2026, #17021 ),
 .UNSPECIFIED., .F., .F.,
 ( 4, 2, 2, 2, 4 ),
 ( 0.1272669073657571592, 0.2522669073462757705, 0.3772669073267943540, 0.5022669073073130486, 0.6272669072878316321 ),
 .UNSPECIFIED. ) ;
#5089=CARTESIAN_POINT ( 'NONE',  ( -24.83263378688676326, -15.59489965655864374, 73.18799144572807336 ) ) ;
#5092=VECTOR ( 'NONE', #20650, 1000.000000000000114 ) ;
#5095=CARTESIAN_POINT ( 'NONE',  ( -22.68646401470678953, -20.08284273627726435, 69.35913316877790180 ) ) ;
#5096=CYLINDRICAL_SURFACE ( 'NONE', #7952, 0.1500000000000072387 ) ;
#5097=CARTESIAN_POINT ( 'NONE',  ( -28.05565061734489873, -15.48652051201079516, 54.60745305979834541 ) ) ;
#5098=ORIENTED_EDGE ( 'NONE', *, *, #4295, .T. ) ;
#5099=EDGE_CURVE ( 'NONE', #28201, #20914, #7492, .T. ) ;
#5101=ORIENTED_EDGE ( 'NONE', *, *, #16858, .F. ) ;
#5102=CARTESIAN_POINT ( 'NONE',  ( -23.08463473158306556, -10.68898933584892674, 59.67373781969178737 ) ) ;
#5103=ADVANCED_FACE ( 'NONE', ( #34046 ), #37489, .T. ) ;
#5105=CARTESIAN_POINT ( 'NONE',  ( -24.48028110873323726, -17.19936403064268760, 73.08324815060153412 ) ) ;
#5106=EDGE_LOOP ( 'NONE', ( #6737, #10786, #43845, #44023 ) ) ;
#5107=CARTESIAN_POINT ( 'NONE',  ( -10.87811525140410929, -17.44835992831754368, 61.31310265544169624 ) ) ;
#5108=DIRECTION ( 'NONE',  ( 5.224165695523869193E-06, -4.853366963026260877E-07, -0.9999999999862362321 ) ) ;
#5109=CARTESIAN_POINT ( 'NONE',  ( -22.82502255886352671, -19.94079571721461264, 72.75062258121896264 ) ) ;
#5111=ORIENTED_EDGE ( 'NONE', *, *, #45957, .T. ) ;
#5114=CARTESIAN_POINT ( 'NONE',  ( -22.72031779163844334, -16.29245029320677673, 54.07175714974878389 ) ) ;
#5115=CARTESIAN_POINT ( 'NONE',  ( -20.69509153224808173, -8.115601224564374050, 63.49616927690831858 ) ) ;
#5116=ORIENTED_EDGE ( 'NONE', *, *, #9768, .F. ) ;
#5117=DIRECTION ( 'NONE',  ( 6.258914665795302800E-07, -5.777405081385165423E-07, -0.9999999999996371791 ) ) ;
#5119=VECTOR ( 'NONE', #36482, 1000.000000000000114 ) ;
#5120=CARTESIAN_POINT ( 'NONE',  ( -19.61601346313181082, -21.50980264518277707, 65.46486213821819433 ) ) ;
#5121=CARTESIAN_POINT ( 'NONE',  ( -23.74619244455238487, -11.68933966055485030, 63.25218278636740621 ) ) ;
#5122=EDGE_CURVE ( 'NONE', #24550, #14223, #45032, .T. ) ;
#5123=EDGE_LOOP ( 'NONE', ( #28183, #13041, #41794, #32534, #30987 ) ) ;
#5125=CARTESIAN_POINT ( 'NONE',  ( -10.42546172544805039, -12.25520447285018122, 57.44362008841285672 ) ) ;
#5129=ORIENTED_EDGE ( 'NONE', *, *, #14743, .F. ) ;
#5130=CARTESIAN_POINT ( 'NONE',  ( -10.60570763719787735, -17.81143699334987218, 71.68222866232767387 ) ) ;
#5131=EDGE_CURVE ( 'NONE', #24042, #19458, #22682, .T. ) ;
#5132=( BOUNDED_CURVE ( )  B_SPLINE_CURVE ( 3, ( #39965, #28155, #36256, #21728 ),
 .UNSPECIFIED., .F., .F. ) 
 B_SPLINE_CURVE_WITH_KNOTS ( ( 4, 4 ),
 ( 1.570796326794896780, 1.780235837034217727 ),
 .UNSPECIFIED. ) 
 CURVE ( )  GEOMETRIC_REPRESENTATION_ITEM ( )  RATIONAL_B_SPLINE_CURVE ( ( 1.000000000000000000, 0.9963479302455154896, 0.9963479302455154896, 1.000000000000000000 ) ) 
 REPRESENTATION_ITEM ( '' )  );
#5133=DIRECTION ( 'NONE',  ( 5.297746385098606630E-06, 8.914243324979344743E-06, 0.9999999999462350075 ) ) ;
#5134=CARTESIAN_POINT ( 'NONE',  ( -22.28911595143133439, -9.166815984689403507, 59.86137841136315529 ) ) ;
#5135=ORIENTED_EDGE ( 'NONE', *, *, #20935, .T. ) ;
#5136=CARTESIAN_POINT ( 'NONE',  ( -15.89079584495563502, -7.517933547575396780, 67.32662675182959333 ) ) ;
#5137=CARTESIAN_POINT ( 'NONE',  ( -11.24997143734453076, -18.22902874506724302, 61.42143955951387113 ) ) ;
#5141=CARTESIAN_POINT ( 'NONE',  ( -13.22529448846758804, -9.145569705956512863, 64.19474388871357462 ) ) ;
#5142=CARTESIAN_POINT ( 'NONE',  ( -11.42787535746950667, -18.52272177604094239, 57.69225786326394001 ) ) ;
#5145=CARTESIAN_POINT ( 'NONE',  ( -23.84653597794508784, -18.58622903642730151, 72.87712840465626130 ) ) ;
#5146=CARTESIAN_POINT ( 'NONE',  ( -19.71364512540636582, -21.89872317270189939, 65.57212061471852849 ) ) ;
#5147=( BOUNDED_CURVE ( )  B_SPLINE_CURVE ( 3, ( #15423, #38321, #30491, #34388 ),
 .UNSPECIFIED., .F., .F. ) 
 B_SPLINE_CURVE_WITH_KNOTS ( ( 4, 4 ),
 ( 0.5000000000000000000, 0.9074455897393605142 ),
 .UNSPECIFIED. ) 
 CURVE ( )  GEOMETRIC_REPRESENTATION_ITEM ( )  RATIONAL_B_SPLINE_CURVE ( ( 1.000000000000018430, 0.4567392136813420711, 0.3561768502900211075, 0.6983129098260754120 ) ) 
 REPRESENTATION_ITEM ( '' )  );
#5148=CARTESIAN_POINT ( 'NONE',  ( -22.96481576609224717, -19.16891988936071556, 58.89882756593014790 ) ) ;
#5149=EDGE_LOOP ( 'NONE', ( #9774, #44002 ) ) ;
#5151=CARTESIAN_POINT ( 'NONE',  ( -10.96921284960095555, -11.97350354382807680, 74.84368195529052059 ) ) ;
#5154=CARTESIAN_POINT ( 'NONE',  ( -23.21283044961208830, -10.11939778159179859, 63.25681392212788268 ) ) ;
#5155=DIRECTION ( 'NONE',  ( 0.05202058437830281434, -0.9986460127597465153, 1.657953767687799911E-08 ) ) ;
#5156=EDGE_CURVE ( 'NONE', #31006, #17131, #42045, .T. ) ;
#5157=( BOUNDED_CURVE ( )  B_SPLINE_CURVE ( 3, ( #19038, #37982, #23726, #46112 ),
 .UNSPECIFIED., .F., .F. ) 
 B_SPLINE_CURVE_WITH_KNOTS ( ( 4, 4 ),
 ( 0.5000000000000000000, 0.9074455897393653991 ),
 .UNSPECIFIED. ) 
 CURVE ( )  GEOMETRIC_REPRESENTATION_ITEM ( )  RATIONAL_B_SPLINE_CURVE ( ( 1.000000000000033973, 0.4567392136813364090, 0.3561768502900080069, 0.6983129098260858481 ) ) 
 REPRESENTATION_ITEM ( '' )  );
#5160=CARTESIAN_POINT ( 'NONE',  ( -15.06868085595426621, -21.40102190336860488, 61.82703723969883924 ) ) ;
#5161=CARTESIAN_POINT ( 'NONE',  ( -23.28952267755650851, -10.88343168269180339, 73.51760210707182353 ) ) ;
#5162=CARTESIAN_POINT ( 'NONE',  ( -15.52406250999510817, -21.54653527486415854, 72.34575433013422696 ) ) ;
#5163=CARTESIAN_POINT ( 'NONE',  ( -15.82941474652824176, -7.531753325696857182, 67.31820067426403398 ) ) ;
#5164=ORIENTED_EDGE ( 'NONE', *, *, #40278, .T. ) ;
#5165=CARTESIAN_POINT ( 'NONE',  ( -24.84793648988037518, -14.18443574041886457, 69.83770584630335065 ) ) ;
#5166=B_SPLINE_CURVE_WITH_KNOTS ( 'NONE', 3,
 ( #15601, #45680, #26954, #4531, #41973, #23262, #19556, #850, #15851, #16577 ),
 .UNSPECIFIED., .F., .F.,
 ( 4, 2, 2, 2, 4 ),
 ( 0.000000000000000000, 0.2500000000000000000, 0.5000000000000000000, 0.7500000000000000000, 1.000000000000000000 ),
 .UNSPECIFIED. ) ;
#5168=ORIENTED_EDGE ( 'NONE', *, *, #40405, .T. ) ;
#5170=CARTESIAN_POINT ( 'NONE',  ( -22.63017914794042085, -20.13847084750349836, 69.29701070597593571 ) ) ;
#5171=FACE_OUTER_BOUND ( 'NONE', #12667, .T. ) ;
#5172=ORIENTED_EDGE ( 'NONE', *, *, #2601, .F. ) ;
#5174=ORIENTED_EDGE ( 'NONE', *, *, #33588, .F. ) ;
#5175=LINE ( 'NONE', #38656, #11508 ) ;
#5177=CARTESIAN_POINT ( 'NONE',  ( -10.42411308964128480, -14.77563531838571009, 71.61317379136900740 ) ) ;
#5180=CARTESIAN_POINT ( 'NONE',  ( -18.37786432726835883, -21.79469297182707521, 69.10042588711679912 ) ) ;
#5183=CARTESIAN_POINT ( 'NONE',  ( -24.42668993457695592, -13.99045928592870780, 73.40799407547365263 ) ) ;
#5184=EDGE_CURVE ( 'NONE', #34569, #545, #27851, .T. ) ;
#5185=CARTESIAN_POINT ( 'NONE',  ( -14.73368791995220839, -7.861157911666011522, 56.96344736924808672 ) ) ;
#5186=CARTESIAN_POINT ( 'NONE',  ( -24.86242983737997747, -14.39095285025967286, 66.36788159907001727 ) ) ;
#5187=ORIENTED_EDGE ( 'NONE', *, *, #31505, .T. ) ;
#5189=CARTESIAN_POINT ( 'NONE',  ( -11.38784684563249527, -10.44144024994987774, 74.55229573521346254 ) ) ;
#5192=CARTESIAN_POINT ( 'NONE',  ( -20.50783493979771421, -8.027295371342848540, 66.96599508560271374 ) ) ;
#5193=CARTESIAN_POINT ( 'NONE',  ( -12.25434429315920859, -20.17366997322574562, 65.05170215947674706 ) ) ;
#5194=VERTEX_POINT ( 'NONE', #12374 ) ;
#5196=CARTESIAN_POINT ( 'NONE',  ( -24.48824824621826224, -12.44270503963961438, 73.44236770847334128 ) ) ;
#5197=CARTESIAN_POINT ( 'NONE',  ( -21.65914559189701194, -18.31838547852702348, 53.49999999999995026 ) ) ;
#5198=VERTEX_POINT ( 'NONE', #16542 ) ;
#5203=ADVANCED_FACE ( 'NONE', ( #27396 ), #47979, .T. ) ;
#5205=CARTESIAN_POINT ( 'NONE',  ( -15.77324217985454347, -8.006205760197399712, 70.89373336146486793 ) ) ;
#5206=EDGE_CURVE ( 'NONE', #30992, #10658, #33833, .T. ) ;
#5207=ORIENTED_EDGE ( 'NONE', *, *, #35300, .T. ) ;
#5212=B_SPLINE_CURVE_WITH_KNOTS ( 'NONE', 3,
 ( #8599, #12993, #38625, #27304, #19921, #35411, #31241, #46517, #5146, #34926 ),
 .UNSPECIFIED., .F., .F.,
 ( 4, 2, 2, 2, 4 ),
 ( 0.6272669072877862240, 0.7522669073072955070, 0.8772669073268049011, 1.002266907346314184, 1.127266907365823467 ),
 .UNSPECIFIED. ) ;
#5213=CARTESIAN_POINT ( 'NONE',  ( -24.42401643431037073, -14.84212902100172293, 59.54300237020546405 ) ) ;
#5214=CARTESIAN_POINT ( 'NONE',  ( -19.81321178474628653, -21.38894381613673090, 68.93482470043255717 ) ) ;
#5215=EDGE_LOOP ( 'NONE', ( #28186, #32722, #30945, #1047, #41429 ) ) ;
#5217=ORIENTED_EDGE ( 'NONE', *, *, #48585, .F. ) ;
#5218=CARTESIAN_POINT ( 'NONE',  ( -11.17855950479832927, -18.87086615690261482, 64.86211796126700335 ) ) ;
#5219=CARTESIAN_POINT ( 'NONE',  ( -24.07726096719255438, -12.63292432398402454, 69.84531015058388448 ) ) ;
#5221=CARTESIAN_POINT ( 'NONE',  ( -10.43414267264621209, -14.42617504702240616, 67.87416736802629202 ) ) ;
#5225=( BOUNDED_CURVE ( )  B_SPLINE_CURVE ( 3, ( #36104, #44019, #32194, #39571 ),
 .UNSPECIFIED., .F., .F. ) 
 B_SPLINE_CURVE_WITH_KNOTS ( ( 4, 4 ),
 ( 1.570796326794897002, 1.780235837034217283 ),
 .UNSPECIFIED. ) 
 CURVE ( )  GEOMETRIC_REPRESENTATION_ITEM ( )  RATIONAL_B_SPLINE_CURVE ( ( 1.000000000000000000, 0.9963479302455154896, 0.9963479302455154896, 1.000000000000000000 ) ) 
 REPRESENTATION_ITEM ( '' )  );
#5226=CARTESIAN_POINT ( 'NONE',  ( -10.47558616449645719, -13.96070292038791294, 57.74824990892705756 ) ) ;
#5227=ORIENTED_EDGE ( 'NONE', *, *, #10485, .T. ) ;
#5230=CARTESIAN_POINT ( 'NONE',  ( -14.25068793291388225, -8.513811817964199946, 71.02957628655769895 ) ) ;
#5232=EDGE_CURVE ( 'NONE', #25942, #12218, #27386, .T. ) ;
#5236=CARTESIAN_POINT ( 'NONE',  ( -24.46812100523181144, -14.51191712007779699, 66.19764790277996269 ) ) ;
#5237=CARTESIAN_POINT ( 'NONE',  ( -15.39389095703113952, -21.97733419268598709, 72.23070866474378704 ) ) ;
#5238=ADVANCED_FACE ( 'NONE', ( #20740 ), #35980, .T. ) ;
#5240=CARTESIAN_POINT ( 'NONE',  ( -20.83411228044830210, -20.98307166581800587, 65.99942768993690834 ) ) ;
#5241=CARTESIAN_POINT ( 'NONE',  ( -20.60909959404585479, -21.04276736930940572, 58.64475179565906160 ) ) ;
#5243=DIRECTION ( 'NONE',  ( -0.8565259173193582320, 0.5161040137028852781, -6.301967848571462020E-08 ) ) ;
#5244=CARTESIAN_POINT ( 'NONE',  ( -13.49145512112739276, -18.65424914341562967, 53.49999999999995026 ) ) ;
#5245=CARTESIAN_POINT ( 'NONE',  ( -24.86683893566021908, -14.47670559543334612, 66.32259343128521323 ) ) ;
#5246=DIRECTION ( 'NONE',  ( 3.549360974554993999E-17, -6.371834667797928663E-18, -1.000000000000000000 ) ) ;
#5247=CARTESIAN_POINT ( 'NONE',  ( -14.21044241041869682, -21.02792381686613155, 72.11710836390169277 ) ) ;
#5251=CARTESIAN_POINT ( 'NONE',  ( -24.26837845117148618, -16.27774503625218827, 59.13834813487091679 ) ) ;
#5252=ORIENTED_EDGE ( 'NONE', *, *, #31379, .F. ) ;
#5253=CYLINDRICAL_SURFACE ( 'NONE', #35491, 0.1499999999999994116 ) ;
#5254=CARTESIAN_POINT ( 'NONE',  ( -14.97500087744905706, -21.84515684796887314, 65.20573060225068218 ) ) ;
#5255=CARTESIAN_POINT ( 'NONE',  ( -17.90754188454616980, -22.24362682123764401, 62.05348668397390099 ) ) ;
#5256=CARTESIAN_POINT ( 'NONE',  ( -22.89412281574421471, -9.750308782327882895, 70.12523226502652562 ) ) ;
#5257=LINE ( 'NONE', #21250, #40848 ) ;
#5258=ORIENTED_EDGE ( 'NONE', *, *, #12418, .T. ) ;
#5259=CARTESIAN_POINT ( 'NONE',  ( -24.41485939984550058, -14.44976655980182834, 66.48292729254383460 ) ) ;
#5260=EDGE_CURVE ( 'NONE', #16415, #40297, #13940, .T. ) ;
#5261=AXIS2_PLACEMENT_3D ( 'NONE', #26827, #7388, #37892 ) ;
#5262=CARTESIAN_POINT ( 'NONE',  ( -16.93941734680483080, -7.775588144984237005, 74.24546186738449194 ) ) ;
#5264=CARTESIAN_POINT ( 'NONE',  ( -10.09540101917376198, -16.14908387813135349, 68.13801154137269123 ) ) ;
#5265=EDGE_CURVE ( 'NONE', #46590, #27904, #43800, .T. ) ;
#5268=ORIENTED_EDGE ( 'NONE', *, *, #7866, .F. ) ;
#5269=CARTESIAN_POINT ( 'NONE',  ( -14.97188219925329378, -8.199429090594037461, 56.84999999999994458 ) ) ;
#5271=CARTESIAN_POINT ( 'NONE',  ( -23.41977742916776251, -11.19648202114625235, 73.66193302070908544 ) ) ;
#5273=CARTESIAN_POINT ( 'NONE',  ( -10.59656512619885227, -13.05092609425065397, 68.02360230423870746 ) ) ;
#5274=LINE ( 'NONE', #23506, #30724 ) ;
#5275=ORIENTED_EDGE ( 'NONE', *, *, #25593, .T. ) ;
#5278=CARTESIAN_POINT ( 'NONE',  ( -24.05059673655033947, -17.06518960458298650, 73.18336032079744768 ) ) ;
#5279=CARTESIAN_POINT ( 'NONE',  ( -20.11563925035808253, -8.345964739383660458, 73.79266765117813520 ) ) ;
#5280=( BOUNDED_SURFACE ( )  B_SPLINE_SURFACE ( 3, 1, ( 
 ( #43962, #17091 ),
 ( #36526, #10462 ),
 ( #6760, #43476 ),
 ( #24757, #39759 ),
 ( #113, #15098 ),
 ( #18301, #14837 ),
 ( #48351, #33311 ) ),
 .UNSPECIFIED., .T., .F., .F. ) 
 B_SPLINE_SURFACE_WITH_KNOTS ( ( 4, 3, 4 ),
 ( 2, 2 ),
 ( 0.000000000000000000, 0.5000000000000000000, 1.000000000000000000 ),
 ( 0.000000000000000000, 1.000000000000000000 ),
 .UNSPECIFIED. ) 
 GEOMETRIC_REPRESENTATION_ITEM ( )  RATIONAL_B_SPLINE_SURFACE ( (
 ( 1.000000000000000000, 1.000000000000000000),
 ( 0.3333333333333335369, 0.3333333333333330373),
 ( 0.3333333333333335369, 0.3333333333333330373),
 ( 1.000000000000000000, 1.000000000000000000),
 ( 0.3333333333333333703, 0.3333333333333333703),
 ( 0.3333333333333333703, 0.3333333333333333703),
 ( 1.000000000000000000, 1.000000000000000000) ) ) 
 REPRESENTATION_ITEM ( '' )  SURFACE ( )  );
#5281=CARTESIAN_POINT ( 'NONE',  ( -17.36015840614627592, -7.359395087992972151, 67.20535029649403214 ) ) ;
#5282=ADVANCED_FACE ( 'NONE', ( #9902 ), #17511, .T. ) ;
#5283=CARTESIAN_POINT ( 'NONE',  ( -24.33592553122863578, -17.58935301986056032, 66.14346027011359297 ) ) ;
#5284=CARTESIAN_POINT ( 'NONE',  ( -20.12289122552838094, -7.865124802246414859, 73.90591932823114973 ) ) ;
#5286=EDGE_LOOP ( 'NONE', ( #11314, #27625, #24910, #40535, #19946 ) ) ;
#5287=CARTESIAN_POINT ( 'NONE',  ( -21.89826351590202336, -8.852228842849337198, 66.84645279485334868 ) ) ;
#5288=( BOUNDED_CURVE ( )  B_SPLINE_CURVE ( 3, ( #35122, #8315, #12725, #447 ),
 .UNSPECIFIED., .F., .F. ) 
 B_SPLINE_CURVE_WITH_KNOTS ( ( 4, 4 ),
 ( 0.5000000000000000000, 0.9074455897393635118 ),
 .UNSPECIFIED. ) 
 CURVE ( )  GEOMETRIC_REPRESENTATION_ITEM ( )  RATIONAL_B_SPLINE_CURVE ( ( 0.9999999999999961142, 0.4567392136813367420, 0.3561768502900346522, 0.6983129098260856260 ) ) 
 REPRESENTATION_ITEM ( '' )  );
#5289=CARTESIAN_POINT ( 'NONE',  ( -17.14068154504527186, -7.813665858854684565, 74.03188528864532714 ) ) ;
#5292=ORIENTED_EDGE ( 'NONE', *, *, #8679, .T. ) ;
#5293=CARTESIAN_POINT ( 'NONE',  ( -10.76802635004704989, -17.14192985119425572, 57.57271792098855201 ) ) ;
#5294=ORIENTED_EDGE ( 'NONE', *, *, #23814, .T. ) ;
#5295=CARTESIAN_POINT ( 'NONE',  ( -10.51728758832436661, -13.39531270954807063, 74.97817630058322891 ) ) ;
#5296=CARTESIAN_POINT ( 'NONE',  ( -10.49189908542464522, -16.09426454567519116, 68.26295692486267797 ) ) ;
#5297=EDGE_CURVE ( 'NONE', #12385, #24381, #22064, .T. ) ;
#5299=CARTESIAN_POINT ( 'NONE',  ( -13.60236376389480384, -20.73382277062339085, 61.80174179654961364 ) ) ;
#5300=CARTESIAN_POINT ( 'NONE',  ( -19.32571124525177098, -8.020471753322730990, 59.96093016115477070 ) ) ;
#5302=CARTESIAN_POINT ( 'NONE',  ( -24.10489316104180801, -11.51232611631470348, 63.10218278254900781 ) ) ;
#5303=CARTESIAN_POINT ( 'NONE',  ( -10.96693745925601959, -17.63935232738105796, 71.57277952047664371 ) ) ;
#5304=CARTESIAN_POINT ( 'NONE',  ( -24.57916482434842820, -12.73107666121563142, 69.95898344571149607 ) ) ;
#5305=CARTESIAN_POINT ( 'NONE',  ( -19.86569447268030686, -19.73755174630646536, 54.07175714974878389 ) ) ;
#5307=B_SPLINE_CURVE_WITH_KNOTS ( 'NONE', 1,
 ( #22097, #13712 ),
 .UNSPECIFIED., .F., .F.,
 ( 2, 2 ),
 ( 0.000000000000000000, 1.000000000000000000 ),
 .UNSPECIFIED. ) ;
#5308=CARTESIAN_POINT ( 'NONE',  ( -11.43673139740920597, -18.43582035383210993, 57.88002590065035946 ) ) ;
#5310=CARTESIAN_POINT ( 'NONE',  ( -22.84886471163500588, -9.702775354051940582, 73.59665661135821324 ) ) ;
#5311=VERTEX_POINT ( 'NONE', #28844 ) ;
#5312=CARTESIAN_POINT ( 'NONE',  ( -23.64630840998975359, -11.48693468987944577, 63.16038249791161263 ) ) ;
#5314=CARTESIAN_POINT ( 'NONE',  ( -21.34121592312026650, -8.943118034117361503, 70.13132274644620168 ) ) ;
#5317=CARTESIAN_POINT ( 'NONE',  ( -24.37683887807358474, -15.97618392648307584, 66.36324926629207255 ) ) ;
#5318=FACE_BOUND ( 'NONE', #48512, .T. ) ;
#5319=ORIENTED_EDGE ( 'NONE', *, *, #3210, .T. ) ;
#5320=ADVANCED_FACE ( 'NONE', ( #35736 ), #25162, .F. ) ;
#5323=ORIENTED_EDGE ( 'NONE', *, *, #37392, .T. ) ;
#5324=CARTESIAN_POINT ( 'NONE',  ( -17.85728874018075985, -21.84618329174708151, 61.89007996730683203 ) ) ;
#5326=CARTESIAN_POINT ( 'NONE',  ( -11.53247046633659423, -18.68106308600668441, 64.74707076449911369 ) ) ;
#5327=CARTESIAN_POINT ( 'NONE',  ( -12.57344175313163781, -19.85833261874117284, 68.44730439049486392 ) ) ;
#5328=CARTESIAN_POINT ( 'NONE',  ( -14.72778380697628187, -21.32322314059345558, 58.16617885012795597 ) ) ;
#5330=AXIS2_PLACEMENT_3D ( 'NONE', #2902, #14214, #43332 ) ;
#5331=ORIENTED_EDGE ( 'NONE', *, *, #10422, .T. ) ;
#5334=EDGE_CURVE ( 'NONE', #15747, #39502, #42666, .T. ) ;
#5337=FACE_OUTER_BOUND ( 'NONE', #20791, .T. ) ;
#5343=B_SPLINE_CURVE_WITH_KNOTS ( 'NONE', 1,
 ( #10336, #40362 ),
 .UNSPECIFIED., .F., .F.,
 ( 2, 2 ),
 ( 0.000000000000000000, 1.000000000000000000 ),
 .UNSPECIFIED. ) ;
#5344=DIRECTION ( 'NONE',  ( -5.731567514496413899E-31, -1.020425574103664789E-16, -1.000000000000000000 ) ) ;
#5345=EDGE_CURVE ( 'NONE', #18572, #24808, #48042, .T. ) ;
#5347=CARTESIAN_POINT ( 'NONE',  ( -12.54253442593986456, -19.82621537833410841, 64.86674886820043184 ) ) ;
#5348=VERTEX_POINT ( 'NONE', #10140 ) ;
#5349=DIRECTION ( 'NONE',  ( 0.9774082387306983755, -0.2113602016968848529, 7.903122840289807171E-08 ) ) ;
#5350=CARTESIAN_POINT ( 'NONE',  ( -22.57893663749957369, -9.999394138389963160, 73.49633153340955971 ) ) ;
#5351=CARTESIAN_POINT ( 'NONE',  ( -22.10214723240122225, -9.011059706093044852, 63.29179509575568119 ) ) ;
#5352=CARTESIAN_POINT ( 'NONE',  ( -19.12163971562669218, -7.963538243666484107, 67.31560661829935555 ) ) ;
#5353=VERTEX_POINT ( 'NONE', #32999 ) ;
#5354=AXIS2_PLACEMENT_3D ( 'NONE', #36680, #10614, #17979 ) ;
#5355=CARTESIAN_POINT ( 'NONE',  ( -11.77169535943213319, -10.59578862612641714, 74.73885051658086809 ) ) ;
#5357=CARTESIAN_POINT ( 'NONE',  ( -11.38992678570165396, -18.36044987817664875, 61.38784012437933768 ) ) ;
#5361=VECTOR ( 'NONE', #37421, 999.9999999999998863 ) ;
#5364=CARTESIAN_POINT ( 'NONE',  ( -14.67111564601650997, -7.886426081561471513, 60.43500846974642116 ) ) ;
#5365=EDGE_LOOP ( 'NONE', ( #44682, #15278 ) ) ;
#5367=DIRECTION ( 'NONE',  ( 0.9986807914369957295, -0.05134858142905001505, 1.286972170232539807E-09 ) ) ;
#5368=CARTESIAN_POINT ( 'NONE',  ( -13.71586683582447819, -8.803873544643577631, 60.58383457371648717 ) ) ;
#5369=CARTESIAN_POINT ( 'NONE',  ( -26.66312147401635713, -19.64855152110175140, 54.58422952202462142 ) ) ;
#5371=DIRECTION ( 'NONE',  ( -5.731567514496413899E-31, -1.020425574103664789E-16, -1.000000000000000000 ) ) ;
#5372=VECTOR ( 'NONE', #24458, 1000.000000000000000 ) ;
#5373=LINE ( 'NONE', #43287, #41562 ) ;
#5374=ADVANCED_FACE ( 'NONE', ( #39929 ), #32540, .T. ) ;
#5375=CARTESIAN_POINT ( 'NONE',  ( -10.49189908542464700, -16.09426454567519116, 68.26295692486267797 ) ) ;
#5376=ORIENTED_EDGE ( 'NONE', *, *, #45361, .T. ) ;
#5377=B_SPLINE_CURVE_WITH_KNOTS ( 'NONE', 3,
 ( #30077, #46302, #1225, #42850, #47017, #23409, #15994, #12315, #13261, #23900 ),
 .UNSPECIFIED., .F., .F.,
 ( 4, 2, 2, 2, 4 ),
 ( 0.1272669073657988481, 0.2522669073439235410, 0.3772669073220482616, 0.5022669073001729823, 0.6272669072782977029 ),
 .UNSPECIFIED. ) ;
#5378=CARTESIAN_POINT ( 'NONE',  ( -15.81235419205221859, -7.945607373518419614, 67.42535135806457447 ) ) ;
#5379=CARTESIAN_POINT ( 'NONE',  ( -24.72417498505505051, -16.29709994844161969, 62.73295351231081440 ) ) ;
#5382=ORIENTED_EDGE ( 'NONE', *, *, #13750, .T. ) ;
#5383=CARTESIAN_POINT ( 'NONE',  ( -24.45601047785835647, -15.36200925639139037, 73.21123547652044294 ) ) ;
#5385=CARTESIAN_POINT ( 'NONE',  ( -10.42619868690400153, -14.62054347036657909, 71.34399284208600989 ) ) ;
#5387=CARTESIAN_POINT ( 'NONE',  ( -11.75188473902813335, -10.61641672623718158, 71.17712947513925315 ) ) ;
#5389=CARTESIAN_POINT ( 'NONE',  ( -12.19762647230555075, -20.11848340473563468, 64.98957966092764593 ) ) ;
#5390=CARTESIAN_POINT ( 'NONE',  ( -13.87335526996593948, -21.35862697870957660, 72.02584070344211398 ) ) ;
#5391=ORIENTED_EDGE ( 'NONE', *, *, #48107, .F. ) ;
#5392=ORIENTED_EDGE ( 'NONE', *, *, #18547, .T. ) ;
#5393=ADVANCED_FACE ( 'NONE', ( #39870 ), #9312, .T. ) ;
#5394=EDGE_CURVE ( 'NONE', #38583, #40137, #31492, .T. ) ;
#5396=CARTESIAN_POINT ( 'NONE',  ( -24.07704370891654122, -17.14264987453632827, 72.89808101046213551 ) ) ;
#5397=LINE ( 'NONE', #28289, #12657 ) ;
#5398=EDGE_CURVE ( 'NONE', #45248, #39530, #12753, .T. ) ;
#5404=CARTESIAN_POINT ( 'NONE',  ( -10.20197030601470090, -12.78660143320473175, 54.27966884056655061 ) ) ;
#5405=CARTESIAN_POINT ( 'NONE',  ( -19.09948850906665285, -8.012659424734943414, 63.73089235424028942 ) ) ;
#5406=CARTESIAN_POINT ( 'NONE',  ( -10.51729421260818320, -16.22293138110306643, 71.44750383217574097 ) ) ;
#5408=EDGE_CURVE ( 'NONE', #38712, #28574, #11516, .T. ) ;
#5410=CARTESIAN_POINT ( 'NONE',  ( -15.87557486115803052, -7.931373420853708112, 67.44007279014866185 ) ) ;
#5411=CARTESIAN_POINT ( 'NONE',  ( -24.43499015649444317, -15.57872826220114781, 69.41818628325123086 ) ) ;
#5413=CARTESIAN_POINT ( 'NONE',  ( -22.84886471163500588, -9.702775354051940582, 73.59665661135821324 ) ) ;
#5414=( BOUNDED_CURVE ( )  B_SPLINE_CURVE ( 3, ( #11501, #11753, #26777, #41796 ),
 .UNSPECIFIED., .F., .F. ) 
 B_SPLINE_CURVE_WITH_KNOTS ( ( 4, 4 ),
 ( 4.712388980384690562, 4.921828490624004182 ),
 .UNSPECIFIED. ) 
 CURVE ( )  GEOMETRIC_REPRESENTATION_ITEM ( )  RATIONAL_B_SPLINE_CURVE ( ( 1.000000000000000000, 0.9963479302455156006, 0.9963479302455156006, 1.000000000000000000 ) ) 
 REPRESENTATION_ITEM ( '' )  );
#5417=CARTESIAN_POINT ( 'NONE',  ( -21.63336539757928634, -9.153348366551478321, 66.94677872351418557 ) ) ;
#5418=ORIENTED_EDGE ( 'NONE', *, *, #41499, .T. ) ;
#5419=CARTESIAN_POINT ( 'NONE',  ( -10.00731240618708462, -14.10555136595099945, 61.10316694600977172 ) ) ;
#5421=VERTEX_POINT ( 'NONE', #14958 ) ;
#5422=CARTESIAN_POINT ( 'NONE',  ( -24.84240844029834250, -14.11474841844398043, 69.76619977786306492 ) ) ;
#5423=DIRECTION ( 'NONE',  ( -0.5022914217388750879, 0.8646984027090224290, 6.766381827299039861E-08 ) ) ;
#5425=AXIS2_PLACEMENT_3D ( 'NONE', #36, #14513, #44605 ) ;
#5427=CARTESIAN_POINT ( 'NONE',  ( -15.26209398273251772, -21.93938324809698770, 68.68937616499954402 ) ) ;
#5429=EDGE_CURVE ( 'NONE', #3502, #44359, #30895, .T. ) ;
#5430=CARTESIAN_POINT ( 'NONE',  ( -10.65158109870909442, -11.70468408355161216, 74.71986640429058468 ) ) ;
#5431=( BOUNDED_CURVE ( )  B_SPLINE_CURVE ( 3, ( #12434, #5300, #20316, #631 ),
 .UNSPECIFIED., .F., .F. ) 
 B_SPLINE_CURVE_WITH_KNOTS ( ( 4, 4 ),
 ( 0.4074455897393606252, 0.5000000000000000000 ),
 .UNSPECIFIED. ) 
 CURVE ( )  GEOMETRIC_REPRESENTATION_ITEM ( )  RATIONAL_B_SPLINE_CURVE ( ( 0.6983129098260884016, 0.7760317562607006447, 0.8765941196520063983, 1.000000000000010214 ) ) 
 REPRESENTATION_ITEM ( '' )  );
#5432=CARTESIAN_POINT ( 'NONE',  ( -16.22845603143158755, -22.16339683637704638, 61.94223519165076652 ) ) ;
#5433=ORIENTED_EDGE ( 'NONE', *, *, #3052, .F. ) ;
#5434=( BOUNDED_CURVE ( )  B_SPLINE_CURVE ( 3, ( #12658, #15607, #34571, #38511 ),
 .UNSPECIFIED., .F., .F. ) 
 B_SPLINE_CURVE_WITH_KNOTS ( ( 4, 4 ),
 ( 0.4074455897393636228, 0.5000000000000000000 ),
 .UNSPECIFIED. ) 
 CURVE ( )  GEOMETRIC_REPRESENTATION_ITEM ( )  RATIONAL_B_SPLINE_CURVE ( ( 0.6983129098260854040, 0.7760317562606773301, 0.8765941196519780876, 0.9999999999999773515 ) ) 
 REPRESENTATION_ITEM ( '' )  );
#5435=FACE_OUTER_BOUND ( 'NONE', #8403, .T. ) ;
#5437=PLANE ( 'NONE',  #11763 ) ;
#5438=FACE_OUTER_BOUND ( 'NONE', #22345, .T. ) ;
#5439=B_SPLINE_CURVE_WITH_KNOTS ( 'NONE', 3,
 ( #34109, #44732, #3588, #14635, #30204, #29952, #37301, #18596, #37549, #44987 ),
 .UNSPECIFIED., .F., .F.,
 ( 4, 2, 2, 2, 4 ),
 ( 0.6272669072783160216, 0.7522669073002095086, 0.8772669073221031066, 1.002266907343996483, 1.127266907365890081 ),
 .UNSPECIFIED. ) ;
#5443=VERTEX_POINT ( 'NONE', #18176 ) ;
#5445=ORIENTED_EDGE ( 'NONE', *, *, #29619, .F. ) ;
#5446=CARTESIAN_POINT ( 'NONE',  ( -15.81235419205221859, -7.945607373518419614, 67.42535135806457447 ) ) ;
#5450=CARTESIAN_POINT ( 'NONE',  ( -23.79929752752725847, -10.95441614946243725, 73.56182072376812187 ) ) ;
#5452=CARTESIAN_POINT ( 'NONE',  ( -10.72552546848295485, -12.61109793159036485, 61.09853568372136579 ) ) ;
#5453=( BOUNDED_CURVE ( )  B_SPLINE_CURVE ( 3, ( #3651, #32939, #33419, #45048 ),
 .UNSPECIFIED., .F., .F. ) 
 B_SPLINE_CURVE_WITH_KNOTS ( ( 4, 4 ),
 ( 0.000000000000000000, 0.4074455897393692849 ),
 .UNSPECIFIED. ) 
 CURVE ( )  GEOMETRIC_REPRESENTATION_ITEM ( )  RATIONAL_B_SPLINE_CURVE ( ( 1.000000000000000000, 0.4567392136813255288, 0.3561768502900278799, 0.6983129098261070533 ) ) 
 REPRESENTATION_ITEM ( '' )  );
#5454=ORIENTED_EDGE ( 'NONE', *, *, #46523, .F. ) ;
#5455=CARTESIAN_POINT ( 'NONE',  ( -22.79734409636068904, -10.24514240368273477, 66.54182257473807738 ) ) ;
#5456=CARTESIAN_POINT ( 'NONE',  ( -14.84927081153347039, -21.37251255130113137, 61.65072491673618771 ) ) ;
#5457=EDGE_CURVE ( 'NONE', #17138, #7495, #37619, .T. ) ;
#5458=CARTESIAN_POINT ( 'NONE',  ( -23.25657551529890554, -10.17392617991681192, 63.32831932546986309 ) ) ;
#5460=EDGE_CURVE ( 'NONE', #28748, #27648, #27565, .T. ) ;
#5461=VERTEX_POINT ( 'NONE', #14456 ) ;
#5462=ORIENTED_EDGE ( 'NONE', *, *, #19094, .F. ) ;
#5468=EDGE_CURVE ( 'NONE', #1538, #20590, #29134, .T. ) ;
#5470=EDGE_CURVE ( 'NONE', #23831, #34081, #41328, .T. ) ;
#5473=CARTESIAN_POINT ( 'NONE',  ( -10.83219059380440541, -11.33772365494832535, 67.74147721111465614 ) ) ;
#5474=CARTESIAN_POINT ( 'NONE',  ( -10.79572390357762046, -11.40795830647630282, 67.80360014157953685 ) ) ;
#5475=VERTEX_POINT ( 'NONE', #26077 ) ;
#5476=CARTESIAN_POINT ( 'NONE',  ( -11.15651104234136781, -18.05456883900698983, 57.95147637344698666 ) ) ;
#5477=LINE ( 'NONE', #43134, #24203 ) ;
#5478=ORIENTED_EDGE ( 'NONE', *, *, #46226, .T. ) ;
#5479=CARTESIAN_POINT ( 'NONE',  ( -11.34160916837339883, -11.34373242234389778, 64.43265517655409269 ) ) ;
#5480=VERTEX_POINT ( 'NONE', #41088 ) ;
#5481=CARTESIAN_POINT ( 'NONE',  ( -10.12802834128535245, -13.30252786720044078, 74.77794016282906853 ) ) ;
#5484=CARTESIAN_POINT ( 'NONE',  ( -12.98761351705371503, -9.325367763573320090, 74.61923228824977627 ) ) ;
#5485=CYLINDRICAL_SURFACE ( 'NONE', #20294, 0.1500000000000032696 ) ;
#5488=CARTESIAN_POINT ( 'NONE',  ( -10.37795889460693033, -14.56696403379599225, 68.14328054657653411 ) ) ;
#5492=CARTESIAN_POINT ( 'NONE',  ( -11.19706266256277694, -11.50303319689152737, 67.63336710488009373 ) ) ;
#5494=CARTESIAN_POINT ( 'NONE',  ( -19.28939461086542906, -8.062307027802660286, 60.26092997386343342 ) ) ;
#5496=CARTESIAN_POINT ( 'NONE',  ( -17.44246871614987526, -7.809230653018538248, 63.65943123996323294 ) ) ;
#5497=CARTESIAN_POINT ( 'NONE',  ( -17.01195873393923463, -21.85086728866913219, 68.69560488337936022 ) ) ;
#5498=DIRECTION ( 'NONE',  ( -1.061592179903616477E-06, -3.103086884670442514E-06, 0.9999999999946218576 ) ) ;
#5499=CARTESIAN_POINT ( 'NONE',  ( -15.18731133007365663, -21.91554468673477629, 68.68254614095756949 ) ) ;
#5500=CARTESIAN_POINT ( 'NONE',  ( -18.19389434033494268, -22.21941471489327569, 65.53027570717884487 ) ) ;
#5502=ORIENTED_EDGE ( 'NONE', *, *, #46653, .T. ) ;
#5507=CARTESIAN_POINT ( 'NONE',  ( -23.17061082369141900, -10.06671700699632233, 66.72837583070179335 ) ) ;
#5509=CARTESIAN_POINT ( 'NONE',  ( -10.76785811675246940, -12.48515291162924434, 57.61385273545094066 ) ) ;
#5511=EDGE_CURVE ( 'NONE', #29328, #43190, #48715, .T. ) ;
#5512=CARTESIAN_POINT ( 'NONE',  ( -12.09832633641969402, -9.599544124683230706, 57.26652452003035876 ) ) ;
#5514=FACE_OUTER_BOUND ( 'NONE', #30377, .T. ) ;
#5516=CARTESIAN_POINT ( 'NONE',  ( -12.81830071990639475, -20.15163239091832992, 68.33657451194982002 ) ) ;
#5518=CARTESIAN_POINT ( 'NONE',  ( -23.44004635400542114, -11.23012040261692590, 73.36193342793328043 ) ) ;
#5519=CARTESIAN_POINT ( 'NONE',  ( -24.53780051168580911, -12.59584816521350348, 69.95738404390658616 ) ) ;
#5520=B_SPLINE_CURVE_WITH_KNOTS ( 'NONE', 3,
 ( #20454, #46317, #34968, #20932, #31281, #24392, #32012, #12571, #38912, #27831 ),
 .UNSPECIFIED., .F., .F.,
 ( 4, 2, 2, 2, 4 ),
 ( 0.6272669072877306018, 0.7522669073072547619, 0.8772669073267790329, 1.002266907346303304, 1.127266907365827464 ),
 .UNSPECIFIED. ) ;
#5521=LINE ( 'NONE', #27188, #42522 ) ;
#5524=ORIENTED_EDGE ( 'NONE', *, *, #19039, .F. ) ;
#5526=ADVANCED_FACE ( 'NONE', ( #11298 ), #3918, .T. ) ;
#5527=CARTESIAN_POINT ( 'NONE',  ( -13.19836015843563182, -9.228522675521540819, 64.13619768069759175 ) ) ;
#5529=ADVANCED_FACE ( 'NONE', ( #40583 ), #42563, .F. ) ;
#5530=CARTESIAN_POINT ( 'NONE',  ( -15.41904641700715217, -7.634001813009263060, 74.19490365927923392 ) ) ;
#5531=EDGE_CURVE ( 'NONE', #17249, #46845, #46760, .T. ) ;
#5532=CARTESIAN_POINT ( 'NONE',  ( -11.64339224431418529, -10.10844562305556771, 71.15548443915361077 ) ) ;
#5533=CARTESIAN_POINT ( 'NONE',  ( -22.97879330524300912, -10.54927326435941026, 59.90203382372271790 ) ) ;
#5534=FACE_OUTER_BOUND ( 'NONE', #11489, .T. ) ;
#5539=CARTESIAN_POINT ( 'NONE',  ( -24.41897112398753933, -17.37347453850100720, 69.59835118672229726 ) ) ;
#5540=VERTEX_POINT ( 'NONE', #4889 ) ;
#5541=CARTESIAN_POINT ( 'NONE',  ( -24.18037252889021005, -17.94870914462638822, 59.18873732074431615 ) ) ;
#5544=CARTESIAN_POINT ( 'NONE',  ( -10.52215041504658188, -13.37196039468857833, 74.97817647370040106 ) ) ;
#5545=EDGE_CURVE ( 'NONE', #13075, #21204, #34410, .T. ) ;
#5546=ORIENTED_EDGE ( 'NONE', *, *, #8535, .F. ) ;
#5547=DIRECTION ( 'NONE',  ( 0.09855345062332551698, 0.9951317587989213509, 3.188559572831062401E-08 ) ) ;
#5548=CARTESIAN_POINT ( 'NONE',  ( -12.21605471856059921, -19.48707561184010117, 57.94298983722725183 ) ) ;
#5550=ORIENTED_EDGE ( 'NONE', *, *, #48609, .T. ) ;
#5551=EDGE_CURVE ( 'NONE', #45668, #42703, #35581, .T. ) ;
#5552=DIRECTION ( 'NONE',  ( 0.9048399035850772654, 0.4257519804770707461, 1.330923649722295902E-08 ) ) ;
#5554=CARTESIAN_POINT ( 'NONE',  ( -12.00117731135775578, -10.30420433458623819, 67.79896860124506475 ) ) ;
#5555=CARTESIAN_POINT ( 'NONE',  ( -10.76763551407085373, -17.13171859787639661, 61.45743118825841833 ) ) ;
#5557=ORIENTED_EDGE ( 'NONE', *, *, #12595, .T. ) ;
#5558=CARTESIAN_POINT ( 'NONE',  ( -10.70532053225239366, -12.67267096592666675, 61.08381491717225487 ) ) ;
#5559=CARTESIAN_POINT ( 'NONE',  ( -10.39693166811831304, -15.37990016280386740, 57.58264896457095006 ) ) ;
#5560=CARTESIAN_POINT ( 'NONE',  ( -23.19948571119275726, -18.85291137746750323, 65.83861571032234394 ) ) ;
#5561=DIRECTION ( 'NONE',  ( 0.4332512900281770274, -0.1108752438054627226, 0.8944271909999157444 ) ) ;
#5563=CARTESIAN_POINT ( 'NONE',  ( -17.73224099643095286, -22.30287356026373047, 53.49999999999994316 ) ) ;
#5566=ORIENTED_EDGE ( 'NONE', *, *, #44339, .F. ) ;
#5568=CARTESIAN_POINT ( 'NONE',  ( -10.52422430310768320, -17.61911375464911700, 68.21226508126260057 ) ) ;
#5569=CARTESIAN_POINT ( 'NONE',  ( -21.08780618903275439, -10.68911097779236385, 53.69233794759168887 ) ) ;
#5570=ORIENTED_EDGE ( 'NONE', *, *, #30786, .T. ) ;
#5571=CARTESIAN_POINT ( 'NONE',  ( -19.90433039125390025, -21.83431899736824988, 69.04987161812600505 ) ) ;
#5574=VERTEX_POINT ( 'NONE', #20136 ) ;
#5575=ORIENTED_EDGE ( 'NONE', *, *, #40257, .T. ) ;
#5576=AXIS2_PLACEMENT_3D ( 'NONE', #22680, #12084, #41381 ) ;
#5578=DIRECTION ( 'NONE',  ( -0.3566357048164924270, 0.9342435303763380050, -8.054691247152028744E-09 ) ) ;
#5579=( BOUNDED_CURVE ( )  B_SPLINE_CURVE ( 3, ( #23790, #8281, #24032, #5073 ),
 .UNSPECIFIED., .F., .F. ) 
 B_SPLINE_CURVE_WITH_KNOTS ( ( 4, 4 ),
 ( 0.5000000000000000000, 0.9074455897393697290 ),
 .UNSPECIFIED. ) 
 CURVE ( )  GEOMETRIC_REPRESENTATION_ITEM ( )  RATIONAL_B_SPLINE_CURVE ( ( 1.000000000000022649, 0.4567392136813365200, 0.3561768502900160560, 0.6983129098260858481 ) ) 
 REPRESENTATION_ITEM ( '' )  );
#5581=CARTESIAN_POINT ( 'NONE',  ( -24.70797074432933371, -13.24467984323328551, 59.56279132098635642 ) ) ;
#5582=CARTESIAN_POINT ( 'NONE',  ( -16.29069520099238133, -22.17261162040731648, 61.93380917110247452 ) ) ;
#5584=EDGE_LOOP ( 'NONE', ( #4840, #36723, #14127, #35441, #39123 ) ) ;
#5586=CARTESIAN_POINT ( 'NONE',  ( -17.66159697976433307, -21.85550285805611637, 58.42025434932890704 ) ) ;
#5589=CARTESIAN_POINT ( 'NONE',  ( -19.80301227694363675, -21.44571519258606074, 69.08482476707463604 ) ) ;
#5592=ORIENTED_EDGE ( 'NONE', *, *, #36859, .F. ) ;
#5593=DIRECTION ( 'NONE',  ( -0.9999247414263408018, 0.01226831216845469807, 5.367905339378915168E-08 ) ) ;
#5594=DIRECTION ( 'NONE',  ( 0.8603613874411346618, -0.3191920208248670288, -0.3973597071195111852 ) ) ;
#5595=AXIS2_PLACEMENT_3D ( 'NONE', #32535, #18652, #30257 ) ;
#5596=DIRECTION ( 'NONE',  ( -0.7364384864160969935, 0.6765045127160409510, 1.031360481960658298E-08 ) ) ;
#5597=B_SPLINE_CURVE_WITH_KNOTS ( 'NONE', 1,
 ( #38285, #27891 ),
 .UNSPECIFIED., .F., .F.,
 ( 2, 2 ),
 ( 0.000000000000000000, 1.000000000000000000 ),
 .UNSPECIFIED. ) ;
#5598=EDGE_LOOP ( 'NONE', ( #4107, #24962, #46171, #1514 ) ) ;
#5599=CARTESIAN_POINT ( 'NONE',  ( -11.60677440104695890, -18.70493592551879658, 68.28860005670347277 ) ) ;
#5601=CARTESIAN_POINT ( 'NONE',  ( -10.38025826595154477, -14.36272272558099772, 71.47215414551031643 ) ) ;
#5602=CARTESIAN_POINT ( 'NONE',  ( -24.46479344177693349, -14.44719919422189491, 66.18292729247950490 ) ) ;
#5603=EDGE_CURVE ( 'NONE', #5635, #21906, #14304, .T. ) ;
#5604=ADVANCED_FACE ( 'NONE', ( #30516 ), #45532, .T. ) ;
#5605=CARTESIAN_POINT ( 'NONE',  ( -22.58763249286555208, -20.18056880150341215, 65.81766459098905386 ) ) ;
#5606=AXIS2_PLACEMENT_3D ( 'NONE', #31947, #5371, #43030 ) ;
#5609=CARTESIAN_POINT ( 'NONE',  ( -24.82569768056232107, -15.65743930089875668, 73.19642064348015253 ) ) ;
#5610=DIRECTION ( 'NONE',  ( -6.516572651863732626E-06, 8.834921937557814562E-06, 0.9999999999397393147 ) ) ;
#5611=ORIENTED_EDGE ( 'NONE', *, *, #33591, .T. ) ;
#5612=DIRECTION ( 'NONE',  ( 0.9968684284758858594, -0.07907803935364897396, 1.831731161803828584E-08 ) ) ;
#5613=VERTEX_POINT ( 'NONE', #11787 ) ;
#5614=CARTESIAN_POINT ( 'NONE',  ( -22.63560516303400050, -20.13310814558360917, 69.28922553891734992 ) ) ;
#5615=EDGE_CURVE ( 'NONE', #30692, #6106, #47379, .T. ) ;
#5617=CARTESIAN_POINT ( 'NONE',  ( -9.983049145142542713, -14.44146248316089753, 67.98083219581930337 ) ) ;
#5618=ORIENTED_EDGE ( 'NONE', *, *, #24122, .F. ) ;
#5619=CARTESIAN_POINT ( 'NONE',  ( -22.17789279454246554, -20.54546261288653852, 58.95781210373504422 ) ) ;
#5621=CARTESIAN_POINT ( 'NONE',  ( -24.21458799606873669, -12.91388130977151327, 66.60246716606879147 ) ) ;
#5622=DIRECTION ( 'NONE',  ( 0.6205284308219133349, 0.7841839494287637935, 1.702810348471058466E-17 ) ) ;
#5623=VERTEX_POINT ( 'NONE', #23601 ) ;
#5624=CARTESIAN_POINT ( 'NONE',  ( -11.46043843694620179, -11.04924462883820802, 57.50903212149482613 ) ) ;
#5626=CARTESIAN_POINT ( 'NONE',  ( -20.52762743779272014, -8.534807845156915818, 63.31121513079826713 ) ) ;
#5627=CARTESIAN_POINT ( 'NONE',  ( -22.22370946352282672, -9.111183370010303761, 59.90666632495347699 ) ) ;
#5629=CARTESIAN_POINT ( 'NONE',  ( -17.46222794319647775, -7.759011850482251837, 67.03511641684839617 ) ) ;
#5631=B_SPLINE_CURVE_WITH_KNOTS ( 'NONE', 3,
 ( #22542, #6558, #37537, #30192, #3577, #14624, #21580, #36803, #44976, #3838 ),
 .UNSPECIFIED., .F., .F.,
 ( 4, 2, 2, 2, 4 ),
 ( 0.000000000000000000, 0.2500000000000000000, 0.5000000000000000000, 0.7500000000000000000, 1.000000000000000000 ),
 .UNSPECIFIED. ) ;
#5632=EDGE_CURVE ( 'NONE', #29649, #34219, #2396, .T. ) ;
#5633=AXIS2_PLACEMENT_3D ( 'NONE', #33864, #41023, #7053 ) ;
#5634=EDGE_LOOP ( 'NONE', ( #15445, #3816 ) ) ;
#5635=VERTEX_POINT ( 'NONE', #28972 ) ;
#5636=CARTESIAN_POINT ( 'NONE',  ( -23.71751471349159601, -11.63122711669449316, 63.23746208799618529 ) ) ;
#5638=CARTESIAN_POINT ( 'NONE',  ( -10.96149970135419061, -18.51576062833312974, 58.06360531077050524 ) ) ;
#5640=CARTESIAN_POINT ( 'NONE',  ( -20.47136568995129480, -10.23054578351414001, 53.49999999999995026 ) ) ;
#5642=CARTESIAN_POINT ( 'NONE',  ( -17.72612443559818018, -7.765381109175947927, 60.36588690973874094 ) ) ;
#5643=ORIENTED_EDGE ( 'NONE', *, *, #11819, .F. ) ;
#5645=VECTOR ( 'NONE', #14132, 1000.000000000000000 ) ;
#5646=CARTESIAN_POINT ( 'NONE',  ( -12.34715986329718085, -20.26164850408625284, 68.45940522080938706 ) ) ;
#5649=CARTESIAN_POINT ( 'NONE',  ( -19.67760665824181388, -21.48965406232008490, 65.75014118398131302 ) ) ;
#5650=CARTESIAN_POINT ( 'NONE',  ( -13.35685073114381716, -8.567315923767541364, 57.01321801328607108 ) ) ;
#5652=ORIENTED_EDGE ( 'NONE', *, *, #10613, .T. ) ;
#5653=CARTESIAN_POINT ( 'NONE',  ( -20.54979551517892489, -8.489990701729437816, 63.31121512946744190 ) ) ;
#5654=CARTESIAN_POINT ( 'NONE',  ( -23.99312268326606201, -11.29471679256767125, 66.60709928216182618 ) ) ;
#5655=CARTESIAN_POINT ( 'NONE',  ( -11.06712629860931152, -18.69414434431124761, 61.39215439313597500 ) ) ;
#5658=CARTESIAN_POINT ( 'NONE',  ( -10.12481675042743667, -13.31795058064993853, 74.87091791722596668 ) ) ;
#5659=CARTESIAN_POINT ( 'NONE',  ( -24.01565389239745585, -17.31039229478603048, 69.41899553355973751 ) ) ;
#5662=( BOUNDED_CURVE ( )  B_SPLINE_CURVE ( 3, ( #16686, #1433, #35878, #46748 ),
 .UNSPECIFIED., .F., .F. ) 
 B_SPLINE_CURVE_WITH_KNOTS ( ( 4, 4 ),
 ( 0.4074455897393622350, 0.5000000000000000000 ),
 .UNSPECIFIED. ) 
 CURVE ( )  GEOMETRIC_REPRESENTATION_ITEM ( )  RATIONAL_B_SPLINE_CURVE ( ( 0.6983129098260739687, 0.7760317562606696695, 0.8765941196519746459, 0.9999999999999807931 ) ) 
 REPRESENTATION_ITEM ( '' )  );
#5663=CARTESIAN_POINT ( 'NONE',  ( -24.03160975973305824, -17.26750547207224784, 69.56339792588553905 ) ) ;
#5664=CARTESIAN_POINT ( 'NONE',  ( -23.47957010007013778, -11.29750547940444427, 69.90713163543374264 ) ) ;
#5666=CARTESIAN_POINT ( 'NONE',  ( -23.65366066840426029, -18.89546231072650784, 69.45518534502666341 ) ) ;
#5668=ADVANCED_FACE ( 'NONE', ( #9306 ), #10590, .T. ) ;
#5670=AXIS2_PLACEMENT_3D ( 'NONE', #45030, #33917, #18398 ) ;
#5671=CARTESIAN_POINT ( 'NONE',  ( -21.50087588749055811, -8.572740410265922151, 73.71473348964758543 ) ) ;
#5672=ORIENTED_EDGE ( 'NONE', *, *, #13871, .F. ) ;
#5674=ADVANCED_FACE ( 'NONE', ( #13926 ), #3992, .T. ) ;
#5676=VECTOR ( 'NONE', #13776, 1000.000000000000227 ) ;
#5678=CARTESIAN_POINT ( 'NONE',  ( -15.34465393633500696, -21.54586957516256263, 68.86120835375241711 ) ) ;
#5679=ADVANCED_FACE ( 'NONE', ( #28256 ), #15611, .T. ) ;
#5680=CARTESIAN_POINT ( 'NONE',  ( -19.79661600260421750, -8.166467367689241641, 73.72096660036417859 ) ) ;
#5681=CARTESIAN_POINT ( 'NONE',  ( -16.36675962830097930, -22.18387328577503581, 61.79922180027413958 ) ) ;
#5682=EDGE_LOOP ( 'NONE', ( #10343, #23727, #16566, #9906, #18384 ) ) ;
#5683=CARTESIAN_POINT ( 'NONE',  ( -23.86876348378221024, -17.54180441657964096, 62.75895669395315224 ) ) ;
#5684=CARTESIAN_POINT ( 'NONE',  ( -10.90856645720024254, -17.50971350489534828, 64.51250748301919202 ) ) ;
#5685=DIRECTION ( 'NONE',  ( 7.130145686591618268E-06, -1.088473442731139027E-05, -0.9999999999153417196 ) ) ;
#5689=ORIENTED_EDGE ( 'NONE', *, *, #612, .T. ) ;
#5690=CARTESIAN_POINT ( 'NONE',  ( -22.51726279860821478, -19.68384809141796765, 72.64400547081167758 ) ) ;
#5691=CARTESIAN_POINT ( 'NONE',  ( -21.35412623182586955, -20.66579906811421452, 68.93961316870652922 ) ) ;
#5692=ORIENTED_EDGE ( 'NONE', *, *, #17278, .T. ) ;
#5694=CARTESIAN_POINT ( 'NONE',  ( -19.27094009026993859, -21.56284704995934831, 62.10576782500217519 ) ) ;
#5696=CARTESIAN_POINT ( 'NONE',  ( -10.42751908256963311, -15.03006480610451234, 74.87066898757765898 ) ) ;
#5698=CARTESIAN_POINT ( 'NONE',  ( -12.26133756782281203, -10.08196798276019557, 60.57420568413689210 ) ) ;
#5699=ORIENTED_EDGE ( 'NONE', *, *, #40554, .T. ) ;
#5702=FACE_OUTER_BOUND ( 'NONE', #42984, .T. ) ;
#5703=CARTESIAN_POINT ( 'NONE',  ( -22.81633530706992019, -9.668548653678303850, 73.68149876278019406 ) ) ;
#5704=CARTESIAN_POINT ( 'NONE',  ( -13.54291469596969577, -20.63483873347275122, 61.51646374974303200 ) ) ;
#5705=VERTEX_POINT ( 'NONE', #40063 ) ;
#5711=( BOUNDED_SURFACE ( )  B_SPLINE_SURFACE ( 3, 1, ( 
 ( #1622, #657 ),
 ( #16134, #19610 ),
 ( #38557, #38806 ),
 ( #5324, #31178 ),
 ( #23310, #27724 ),
 ( #45960, #12706 ),
 ( #46200, #30948 ) ),
 .UNSPECIFIED., .T., .F., .F. ) 
 B_SPLINE_SURFACE_WITH_KNOTS ( ( 4, 3, 4 ),
 ( 2, 2 ),
 ( 0.000000000000000000, 0.5000000000000000000, 1.000000000000000000 ),
 ( 0.000000000000000000, 1.000000000000000000 ),
 .UNSPECIFIED. ) 
 GEOMETRIC_REPRESENTATION_ITEM ( )  RATIONAL_B_SPLINE_SURFACE ( (
 ( 1.000000000000000000, 1.000000000000000000),
 ( 0.3333333333333335369, 0.3333333333333330373),
 ( 0.3333333333333335369, 0.3333333333333330373),
 ( 1.000000000000000000, 1.000000000000000000),
 ( 0.3333333333333333703, 0.3333333333333333703),
 ( 0.3333333333333333703, 0.3333333333333333703),
 ( 1.000000000000000000, 1.000000000000000000) ) ) 
 REPRESENTATION_ITEM ( '' )  SURFACE ( )  );
#5714=B_SPLINE_CURVE_WITH_KNOTS ( 'NONE', 1,
 ( #31304, #31549 ),
 .UNSPECIFIED., .F., .F.,
 ( 2, 2 ),
 ( 0.000000000000000000, 1.000000000000000000 ),
 .UNSPECIFIED. ) ;
#5715=CARTESIAN_POINT ( 'NONE',  ( -16.23805205469483681, -7.454097322849217555, 60.37841262270664089 ) ) ;
#5716=CARTESIAN_POINT ( 'NONE',  ( -10.01086014178825323, -14.06997349321342483, 61.06821291928545747 ) ) ;
#5717=EDGE_CURVE ( 'NONE', #12076, #21448, #8555, .T. ) ;
#5718=ORIENTED_EDGE ( 'NONE', *, *, #26514, .T. ) ;
#5719=CARTESIAN_POINT ( 'NONE',  ( -13.43773910423563400, -20.62433115109003268, 58.33177939114180788 ) ) ;
#5722=CARTESIAN_POINT ( 'NONE',  ( -23.34092575347512266, -10.28207967581048088, 59.78698817202694471 ) ) ;
#5723=ORIENTED_EDGE ( 'NONE', *, *, #42481, .F. ) ;
#5724=( BOUNDED_CURVE ( )  B_SPLINE_CURVE ( 3, ( #1623, #4846, #35353, #16136 ),
 .UNSPECIFIED., .F., .F. ) 
 B_SPLINE_CURVE_WITH_KNOTS ( ( 4, 4 ),
 ( 0.4074455897393660098, 0.5000000000000000000 ),
 .UNSPECIFIED. ) 
 CURVE ( )  GEOMETRIC_REPRESENTATION_ITEM ( )  RATIONAL_B_SPLINE_CURVE ( ( 0.6983129098260920653, 0.7760317562606868780, 0.8765941196519864143, 0.9999999999999834577 ) ) 
 REPRESENTATION_ITEM ( '' )  );
#5725=CARTESIAN_POINT ( 'NONE',  ( -10.59609684676525276, -13.26671058769154676, 71.22330973224352135 ) ) ;
#5726=ORIENTED_EDGE ( 'NONE', *, *, #16020, .T. ) ;
#5727=CARTESIAN_POINT ( 'NONE',  ( -11.91343869374197695, -19.82283377674160718, 58.04186948019505365 ) ) ;
#5728=CARTESIAN_POINT ( 'NONE',  ( -12.27729947935473476, -9.991218615320079266, 60.85918086709605745 ) ) ;
#5729=CARTESIAN_POINT ( 'NONE',  ( -19.44371787714632305, -21.98101111209947334, 58.63852002154196441 ) ) ;
#5730=ORIENTED_EDGE ( 'NONE', *, *, #1319, .T. ) ;
#5732=CARTESIAN_POINT ( 'NONE',  ( -24.69852204723760281, -16.41745771733451775, 59.30827817708741634 ) ) ;
#5733=EDGE_CURVE ( 'NONE', #32337, #21832, #24435, .T. ) ;
#5735=EDGE_CURVE ( 'NONE', #10202, #34559, #19364, .T. ) ;
#5736=CARTESIAN_POINT ( 'NONE',  ( -19.86401518824997581, -21.42384811948916479, 69.22010401872219632 ) ) ;
#5737=FACE_OUTER_BOUND ( 'NONE', #13058, .T. ) ;
#5738=CARTESIAN_POINT ( 'NONE',  ( -10.38069781390674251, -17.23693455343903480, 61.26468960721474843 ) ) ;
#5739=ORIENTED_EDGE ( 'NONE', *, *, #20014, .F. ) ;
#5741=( BOUNDED_SURFACE ( )  B_SPLINE_SURFACE ( 3, 1, ( 
 ( #47666, #14140 ),
 ( #21798, #17119 ),
 ( #28232, #32172 ),
 ( #43263, #29197 ),
 ( #28948, #40042 ),
 ( #47190, #21574 ),
 ( #13434, #6055 ) ),
 .UNSPECIFIED., .T., .F., .F. ) 
 B_SPLINE_SURFACE_WITH_KNOTS ( ( 4, 3, 4 ),
 ( 2, 2 ),
 ( 0.000000000000000000, 0.5000000000000000000, 1.000000000000000000 ),
 ( 0.000000000000000000, 1.000000000000000000 ),
 .UNSPECIFIED. ) 
 GEOMETRIC_REPRESENTATION_ITEM ( )  RATIONAL_B_SPLINE_SURFACE ( (
 ( 1.000000000000000000, 1.000000000000000000),
 ( 0.3333333333333335369, 0.3333333333333330373),
 ( 0.3333333333333335369, 0.3333333333333330373),
 ( 1.000000000000000000, 1.000000000000000000),
 ( 0.3333333333333333703, 0.3333333333333333703),
 ( 0.3333333333333333703, 0.3333333333333333703),
 ( 1.000000000000000000, 1.000000000000000000) ) ) 
 REPRESENTATION_ITEM ( '' )  SURFACE ( )  );
#5742=CARTESIAN_POINT ( 'NONE',  ( -24.65603385937463088, -13.01988417981330315, 63.03252945310004662 ) ) ;
#5743=B_SPLINE_CURVE_WITH_KNOTS ( 'NONE', 3,
 ( #8607, #5646, #16930, #35415, #20416, #38874, #23632, #42819, #31244, #38629 ),
 .UNSPECIFIED., .F., .F.,
 ( 4, 2, 2, 2, 4 ),
 ( 0.1272669073658327099, 0.2522669073488013614, 0.3772669073317700406, 0.5022669073147386642, 0.6272669072977072879 ),
 .UNSPECIFIED. ) ;
#5744=CARTESIAN_POINT ( 'NONE',  ( -21.35673258969864818, -10.96416394607318701, 53.49899999999994549 ) ) ;
#5745=EDGE_CURVE ( 'NONE', #10314, #1656, #28535, .T. ) ;
#5746=CARTESIAN_POINT ( 'NONE',  ( -19.98494827787780181, -21.80542074767473437, 69.07335975967473018 ) ) ;
#5748=ORIENTED_EDGE ( 'NONE', *, *, #10890, .F. ) ;
#5749=CARTESIAN_POINT ( 'NONE',  ( -21.68499379980493558, -9.192514338196573931, 66.96149992326067490 ) ) ;
#5750=LINE ( 'NONE', #36474, #45445 ) ;
#5752=FACE_OUTER_BOUND ( 'NONE', #10936, .T. ) ;
#5753=CARTESIAN_POINT ( 'NONE',  ( -10.53028993777715883, -16.28642212234895226, 71.73278239416407587 ) ) ;
#5754=CARTESIAN_POINT ( 'NONE',  ( -22.75539019595755263, -10.19575032747719590, 66.82710158566565894 ) ) ;
#5755=CARTESIAN_POINT ( 'NONE',  ( -19.37484727228654080, -7.619050864103940057, 60.14588289477547534 ) ) ;
#5756=EDGE_CURVE ( 'NONE', #24418, #47047, #25762, .T. ) ;
#5757=VERTEX_POINT ( 'NONE', #14642 ) ;
#5758=CARTESIAN_POINT ( 'NONE',  ( -23.70135487130767515, -11.71146637837649074, 63.25218278684473461 ) ) ;
#5761=CARTESIAN_POINT ( 'NONE',  ( -21.22358616875703063, -21.29681159568578153, 53.76227901944321275 ) ) ;
#5763=B_SPLINE_CURVE_WITH_KNOTS ( 'NONE', 3,
 ( #15805, #35244, #19268, #562, #23946, #46102, #23716, #45872, #46352, #8432 ),
 .UNSPECIFIED., .F., .F.,
 ( 4, 2, 2, 2, 4 ),
 ( 0.1272669073658498906, 0.2522669073463310041, 0.3772669073268121176, 0.5022669073072931756, 0.6272669072877743446 ),
 .UNSPECIFIED. ) ;
#5764=CARTESIAN_POINT ( 'NONE',  ( -13.18991935570955576, -8.679356915182284027, 60.63224404241364596 ) ) ;
#5765=CARTESIAN_POINT ( 'NONE',  ( -21.12013511752277495, -20.75402118300628018, 69.35450231647695318 ) ) ;
#5766=CARTESIAN_POINT ( 'NONE',  ( -10.76458884141051975, -11.46785096862322995, 71.27516169247240896 ) ) ;
#5767=CARTESIAN_POINT ( 'NONE',  ( -10.73729177923718758, -12.73729707409820122, 64.28452752943745452 ) ) ;
#5768=VERTEX_POINT ( 'NONE', #29703 ) ;
#5771=CARTESIAN_POINT ( 'NONE',  ( -10.37491704552005167, -14.91954605113452459, 75.09778880425432135 ) ) ;
#5773=CARTESIAN_POINT ( 'NONE',  ( -14.06039897761215762, -8.161786889575166626, 70.92946410255460421 ) ) ;
#5776=CARTESIAN_POINT ( 'NONE',  ( -24.79781836340079337, -15.87314503134675014, 69.64812095075065201 ) ) ;
#5777=ORIENTED_EDGE ( 'NONE', *, *, #29503, .F. ) ;
#5778=CARTESIAN_POINT ( 'NONE',  ( -20.98579777188748707, -20.83533835786949950, 65.58453944793343737 ) ) ;
#5779=CARTESIAN_POINT ( 'NONE',  ( -24.24654216478982960, -17.80199886438881762, 62.67372181833962230 ) ) ;
#5781=CYLINDRICAL_SURFACE ( 'NONE', #6057, 0.1499999999999962474 ) ;
#5785=B_SPLINE_CURVE_WITH_KNOTS ( 'NONE', 3,
 ( #23992, #24235, #5767, #39241, #2054, #13116, #38993, #1569, #17054, #28159 ),
 .UNSPECIFIED., .F., .F.,
 ( 4, 2, 2, 2, 4 ),
 ( 0.000000000000000000, 0.2500000000000000000, 0.5000000000000000000, 0.7500000000000000000, 1.000000000000000000 ),
 .UNSPECIFIED. ) ;
#5786=CARTESIAN_POINT ( 'NONE',  ( -24.48810908846319734, -17.17637088580320537, 73.06831457992643664 ) ) ;
#5787=CARTESIAN_POINT ( 'NONE',  ( -18.64993026675905341, -21.70103686862637105, 72.47614041008449703 ) ) ;
#5788=VERTEX_POINT ( 'NONE', #18602 ) ;
#5789=CARTESIAN_POINT ( 'NONE',  ( -23.80321465417087978, -17.81075909821204917, 59.15378417737379380 ) ) ;
#5791=CARTESIAN_POINT ( 'NONE',  ( -22.94085434386056832, -9.802298134861713308, 70.19673941016031904 ) ) ;
#5793=CARTESIAN_POINT ( 'NONE',  ( -16.93941734680482725, -7.775588144984237005, 74.24546186738449194 ) ) ;
#5797=CARTESIAN_POINT ( 'NONE',  ( -11.07857809310684338, -11.73724795245126451, 71.38860870961248395 ) ) ;
#5798=CARTESIAN_POINT ( 'NONE',  ( -12.18836193727821460, -19.53083876418623532, 57.94154444592973618 ) ) ;
#5800=CARTESIAN_POINT ( 'NONE',  ( -20.12437885760196110, -7.865711196993452781, 73.76450701231766516 ) ) ;
#5806=CARTESIAN_POINT ( 'NONE',  ( -14.23131808380166596, -8.077975302584915696, 67.45249250995216528 ) ) ;
#5807=CARTESIAN_POINT ( 'NONE',  ( -24.32886716615087153, -16.23426984194678724, 62.60800820172418923 ) ) ;
#5809=CARTESIAN_POINT ( 'NONE',  ( -15.22116837037893866, -21.50650591823945845, 68.59065000974109694 ) ) ;
#5810=VERTEX_POINT ( 'NONE', #174 ) ;
#5813=CARTESIAN_POINT ( 'NONE',  ( -24.93953149451673568, -10.04808947811604902, 53.49999999999995026 ) ) ;
#5814=FACE_OUTER_BOUND ( 'NONE', #31126, .T. ) ;
#5816=EDGE_CURVE ( 'NONE', #39922, #15615, #2672, .T. ) ;
#5817=CARTESIAN_POINT ( 'NONE',  ( -16.98831825750070479, -22.24652902502744922, 72.20897298418123000 ) ) ;
#5820=ORIENTED_EDGE ( 'NONE', *, *, #8265, .F. ) ;
#5823=CARTESIAN_POINT ( 'NONE',  ( -24.87388367747922757, -14.87141420204137710, 59.43638527419312823 ) ) ;
#5824=CARTESIAN_POINT ( 'NONE',  ( -24.05059659118241555, -17.06519001246171996, 72.88336032079776317 ) ) ;
#5826=VECTOR ( 'NONE', #15511, 1000.000000000000000 ) ;
#5827=VERTEX_POINT ( 'NONE', #40306 ) ;
#5828=CARTESIAN_POINT ( 'NONE',  ( -12.43365403769799826, -9.824193568099090612, 60.85918061814654578 ) ) ;
#5829=DIRECTION ( 'NONE',  ( 1.184681381641773627E-05, 1.827615834487727850E-06, -0.9999999999281563579 ) ) ;
#5830=AXIS2_PLACEMENT_3D ( 'NONE', #106, #48112, #25696 ) ;
#5831=FACE_OUTER_BOUND ( 'NONE', #36770, .T. ) ;
#5832=VERTEX_POINT ( 'NONE', #21595 ) ;
#5833=CARTESIAN_POINT ( 'NONE',  ( -14.98927377128279304, -8.246306944878790901, 47.99999999999994316 ) ) ;
#5834=DIRECTION ( 'NONE',  ( -0.4599824152910791941, -0.8879280250239794947, -2.250728351766169940E-08 ) ) ;
#5836=CARTESIAN_POINT ( 'NONE',  ( -14.41428173599358331, -7.994163662063686893, 63.97474278339937115 ) ) ;
#5838=CARTESIAN_POINT ( 'NONE',  ( -19.85890256509918572, -21.37233786973231275, 68.95612130754568625 ) ) ;
#5844=CARTESIAN_POINT ( 'NONE',  ( -11.78701489841286332, -10.65889831958446976, 74.73884969804157663 ) ) ;
#5848=CARTESIAN_POINT ( 'NONE',  ( -17.42409385541300892, -14.80920654474439679, 47.99999999999994316 ) ) ;
#5849=CARTESIAN_POINT ( 'NONE',  ( -10.40127108354264429, -12.32249413655887871, 57.51352655450988749 ) ) ;
#5850=CARTESIAN_POINT ( 'NONE',  ( -17.08574859075978480, -7.366143556642608559, 74.14673579026420214 ) ) ;
#5852=VERTEX_POINT ( 'NONE', #11977 ) ;
#5853=FACE_OUTER_BOUND ( 'NONE', #793, .T. ) ;
#5854=FACE_OUTER_BOUND ( 'NONE', #32632, .T. ) ;
#5855=( BOUNDED_SURFACE ( )  B_SPLINE_SURFACE ( 3, 1, ( 
 ( #46425, #34594 ),
 ( #39019, #878 ),
 ( #4816, #46177 ),
 ( #34839, #5062 ),
 ( #35326, #20070 ),
 ( #35074, #12680 ),
 ( #47869, #17571 ) ),
 .UNSPECIFIED., .T., .F., .F. ) 
 B_SPLINE_SURFACE_WITH_KNOTS ( ( 4, 3, 4 ),
 ( 2, 2 ),
 ( 0.000000000000000000, 0.5000000000000000000, 1.000000000000000000 ),
 ( 0.000000000000000000, 1.000000000000000000 ),
 .UNSPECIFIED. ) 
 GEOMETRIC_REPRESENTATION_ITEM ( )  RATIONAL_B_SPLINE_SURFACE ( (
 ( 1.000000000000000000, 1.000000000000000000),
 ( 0.3333333333333335369, 0.3333333333333330373),
 ( 0.3333333333333335369, 0.3333333333333330373),
 ( 1.000000000000000000, 1.000000000000000000),
 ( 0.3333333333333333703, 0.3333333333333333703),
 ( 0.3333333333333333703, 0.3333333333333333703),
 ( 1.000000000000000000, 1.000000000000000000) ) ) 
 REPRESENTATION_ITEM ( '' )  SURFACE ( )  );
#5857=CARTESIAN_POINT ( 'NONE',  ( -10.61052024580041930, -11.79586507274399310, 74.71873631039885311 ) ) ;
#5858=AXIS2_PLACEMENT_3D ( 'NONE', #41718, #122, #15105 ) ;
#5859=CARTESIAN_POINT ( 'NONE',  ( -12.13668540368383653, -10.14142895936130628, 60.44429485117178302 ) ) ;
#5861=VERTEX_POINT ( 'NONE', #9188 ) ;
#5862=EDGE_LOOP ( 'NONE', ( #13480, #12073, #1278, #12309 ) ) ;
#5863=CARTESIAN_POINT ( 'NONE',  ( -14.81833918149647822, -21.30619657749716112, 58.18120369631310496 ) ) ;
#5865=CARTESIAN_POINT ( 'NONE',  ( -19.96994565995125015, -21.32983830779690848, 72.70478737306767414 ) ) ;
#5867=CARTESIAN_POINT ( 'NONE',  ( -24.45390269921422188, -14.27548703327989621, 69.65275280629234089 ) ) ;
#5868=CARTESIAN_POINT ( 'NONE',  ( -19.55842747286782313, -21.47588638780701942, 62.18606779526226092 ) ) ;
#5869=CARTESIAN_POINT ( 'NONE',  ( -12.29704640786070158, -19.57524266776748334, 57.92682366959790130 ) ) ;
#5870=CARTESIAN_POINT ( 'NONE',  ( -11.14886767096676934, -11.58796814604482250, 64.14881821840825182 ) ) ;
#5871=( BOUNDED_SURFACE ( )  B_SPLINE_SURFACE ( 3, 1, ( 
 ( #31396, #35077 ),
 ( #16364, #12917 ),
 ( #16109, #26978 ),
 ( #8274, #42967 ),
 ( #23290, #16609 ),
 ( #633, #1601 ),
 ( #27940, #39022 ) ),
 .UNSPECIFIED., .T., .F., .F. ) 
 B_SPLINE_SURFACE_WITH_KNOTS ( ( 4, 3, 4 ),
 ( 2, 2 ),
 ( 0.000000000000000000, 0.5000000000000000000, 1.000000000000000000 ),
 ( 0.000000000000000000, 1.000000000000000000 ),
 .UNSPECIFIED. ) 
 GEOMETRIC_REPRESENTATION_ITEM ( )  RATIONAL_B_SPLINE_SURFACE ( (
 ( 1.000000000000000000, 1.000000000000000000),
 ( 0.3333333333333335369, 0.3333333333333330373),
 ( 0.3333333333333335369, 0.3333333333333330373),
 ( 1.000000000000000000, 1.000000000000000000),
 ( 0.3333333333333333703, 0.3333333333333333703),
 ( 0.3333333333333333703, 0.3333333333333333703),
 ( 1.000000000000000000, 1.000000000000000000) ) ) 
 REPRESENTATION_ITEM ( '' )  SURFACE ( )  );
#5872=EDGE_CURVE ( 'NONE', #44873, #34640, #34160, .T. ) ;
#5873=CARTESIAN_POINT ( 'NONE',  ( -16.70460144941857195, -22.22450915091796020, 68.81843766967561749 ) ) ;
#5874=VERTEX_POINT ( 'NONE', #24206 ) ;
#5876=CARTESIAN_POINT ( 'NONE',  ( -18.83586040784625126, -7.494106175837369044, 70.48572642001049360 ) ) ;
#5880=CARTESIAN_POINT ( 'NONE',  ( -22.01318819962695983, -20.09513598245419885, 58.83730921330041497 ) ) ;
#5882=CARTESIAN_POINT ( 'NONE',  ( -20.36919052476639180, -21.22336078664356407, 58.78908032405391992 ) ) ;
#5883=ORIENTED_EDGE ( 'NONE', *, *, #45298, .T. ) ;
#5884=CARTESIAN_POINT ( 'NONE',  ( -20.10030308072983374, -21.76202485516048668, 72.51983413602351902 ) ) ;
#5886=CARTESIAN_POINT ( 'NONE',  ( -16.39156059917436181, -21.78318494029796781, 62.05568132351888977 ) ) ;
#5887=CARTESIAN_POINT ( 'NONE',  ( -10.09291371782238045, -16.13494220690481384, 68.16263107114907882 ) ) ;
#5888=ORIENTED_EDGE ( 'NONE', *, *, #45159, .T. ) ;
#5889=CARTESIAN_POINT ( 'NONE',  ( -17.99631655628617466, -7.779455715877602984, 60.49549448422539655 ) ) ;
#5891=AXIS2_PLACEMENT_3D ( 'NONE', #11367, #45611, #22959 ) ;
#5893=CARTESIAN_POINT ( 'NONE',  ( -17.35166681046315773, -7.759430071869731549, 67.31479834546361474 ) ) ;
#5894=CARTESIAN_POINT ( 'NONE',  ( -11.13707727077725096, -10.81211843560235053, 57.31629078479772943 ) ) ;
#5895=CARTESIAN_POINT ( 'NONE',  ( -16.06904454444675778, -7.890656075740461795, 63.67011029959335389 ) ) ;
#5898=VERTEX_POINT ( 'NONE', #30452 ) ;
#5900=CARTESIAN_POINT ( 'NONE',  ( -10.23808006521456093, -12.84309671393774721, 67.86115469475366524 ) ) ;
#5902=CARTESIAN_POINT ( 'NONE',  ( -13.70551016122406018, -21.26485310498106429, 68.56286810530107800 ) ) ;
#5904=EDGE_CURVE ( 'NONE', #32131, #5574, #7347, .T. ) ;
#5906=CARTESIAN_POINT ( 'NONE',  ( -17.92189206272508883, -7.825646655266591090, 60.30890604785338382 ) ) ;
#5907=CARTESIAN_POINT ( 'NONE',  ( -16.72330486927764426, -21.83230113783351101, 61.91134987066439521 ) ) ;
#5908=ORIENTED_EDGE ( 'NONE', *, *, #48622, .T. ) ;
#5909=PLANE ( 'NONE',  #16064 ) ;
#5911=B_SPLINE_CURVE_WITH_KNOTS ( 'NONE', 3,
 ( #38560, #30951, #45963, #4848, #19867, #8792, #34865, #23809, #38810, #6537 ),
 .UNSPECIFIED., .F., .F.,
 ( 4, 2, 2, 2, 4 ),
 ( 0.000000000000000000, 0.2500000000000000000, 0.5000000000000000000, 0.7500000000000000000, 1.000000000000000000 ),
 .UNSPECIFIED. ) ;
#5912=CARTESIAN_POINT ( 'NONE',  ( -12.93051514224950260, -9.376680094107033625, 71.14365550519747217 ) ) ;
#5915=VERTEX_POINT ( 'NONE', #43159 ) ;
#5916=CYLINDRICAL_SURFACE ( 'NONE', #2339, 0.1500000000000065448 ) ;
#5917=CARTESIAN_POINT ( 'NONE',  ( -10.02995815481606634, -13.89786978184575794, 57.63320425522585566 ) ) ;
#5920=CARTESIAN_POINT ( 'NONE',  ( -21.99178500617274779, -9.439039195359631762, 59.72171213140594404 ) ) ;
#5922=CARTESIAN_POINT ( 'NONE',  ( -10.42805625848568596, -15.04470190113622685, 74.90664863841101351 ) ) ;
#5924=CARTESIAN_POINT ( 'NONE',  ( -15.88442554950127139, -7.926310505211968227, 71.02478706424572863 ) ) ;
#5925=AXIS2_PLACEMENT_3D ( 'NONE', #28273, #34981, #24596 ) ;
#5927=CARTESIAN_POINT ( 'NONE',  ( -11.77169895589660698, -10.59578386207264700, 74.43885051664024388 ) ) ;
#5928=ADVANCED_FACE ( 'NONE', ( #30696 ), #24116, .T. ) ;
#5929=AXIS2_PLACEMENT_3D ( 'NONE', #23912, #16731, #46067 ) ;
#5930=CARTESIAN_POINT ( 'NONE',  ( -24.87384330655416420, -14.87999779688033719, 59.35804910119406230 ) ) ;
#5931=CARTESIAN_POINT ( 'NONE',  ( -19.42896492416523913, -21.56812594671148275, 61.99503644571810668 ) ) ;
#5933=EDGE_CURVE ( 'NONE', #22219, #32319, #8280, .T. ) ;
#5934=EDGE_CURVE ( 'NONE', #8273, #13357, #5597, .T. ) ;
#5935=ORIENTED_EDGE ( 'NONE', *, *, #15590, .F. ) ;
#5941=EDGE_CURVE ( 'NONE', #6262, #23858, #38451, .T. ) ;
#5942=ORIENTED_EDGE ( 'NONE', *, *, #41610, .T. ) ;
#5944=CARTESIAN_POINT ( 'NONE',  ( -18.46801905451614445, -7.836623195388688679, 74.12592262855558545 ) ) ;
#5945=EDGE_CURVE ( 'NONE', #1365, #20228, #26985, .T. ) ;
#5946=ORIENTED_EDGE ( 'NONE', *, *, #47317, .F. ) ;
#5947=CARTESIAN_POINT ( 'NONE',  ( -10.92563986671175691, -18.45389586190763964, 57.99369949602996854 ) ) ;
#5948=CARTESIAN_POINT ( 'NONE',  ( -17.84029764213619984, -21.79726099838181597, 62.15919343507878381 ) ) ;
#5950=CARTESIAN_POINT ( 'NONE',  ( -22.33376602745314798, -19.86903051493498040, 69.18890041286789483 ) ) ;
#5951=ORIENTED_EDGE ( 'NONE', *, *, #40609, .F. ) ;
#5952=CARTESIAN_POINT ( 'NONE',  ( -13.47245400663725690, -21.12492667118925382, 65.10133491818508844 ) ) ;
#5956=CARTESIAN_POINT ( 'NONE',  ( -19.37616744185158879, -21.99900390342548206, 58.71002665166666645 ) ) ;
#5957=ORIENTED_EDGE ( 'NONE', *, *, #9103, .F. ) ;
#5960=DIRECTION ( 'NONE',  ( 0.8394943004421989707, -0.3114503813636536056, -0.4452504682462418151 ) ) ;
#5962=CARTESIAN_POINT ( 'NONE',  ( -21.06702863216100141, -20.84540773593991148, 65.86981821684420879 ) ) ;
#5963=ORIENTED_EDGE ( 'NONE', *, *, #21393, .T. ) ;
#5964=CARTESIAN_POINT ( 'NONE',  ( -11.68672781637937419, -10.05669048882576533, 67.68392176937598492 ) ) ;
#5965=DIRECTION ( 'NONE',  ( -0.9441784275685842776, 0.3294345108122634369, 1.993146885055995131E-08 ) ) ;
#5966=CARTESIAN_POINT ( 'NONE',  ( -13.16557854728010746, -20.92211907906095547, 58.14626439336120711 ) ) ;
#5971=CARTESIAN_POINT ( 'NONE',  ( -22.51726247777427758, -19.68384842258191370, 72.94400547081133368 ) ) ;
#5973=CARTESIAN_POINT ( 'NONE',  ( -10.37821464302998109, -14.49231327520767465, 71.74271303568544056 ) ) ;
#5974=LINE ( 'NONE', #13821, #8593 ) ;
#5976=CARTESIAN_POINT ( 'NONE',  ( -15.42641777070416609, -21.57041088783041971, 72.05135256464748750 ) ) ;
#5977=ADVANCED_FACE ( 'NONE', ( #20263 ), #35270, .T. ) ;
#5978=ORIENTED_EDGE ( 'NONE', *, *, #27278, .T. ) ;
#5979=CARTESIAN_POINT ( 'NONE',  ( -23.88506645939990847, -17.50400960575725406, 66.22740630230595116 ) ) ;
#5980=DIRECTION ( 'NONE',  ( 0.8839923186919886877, -0.4675014229855999348, 2.842058574697910628E-08 ) ) ;
#5981=CARTESIAN_POINT ( 'NONE',  ( -23.74125355947768767, -17.82500418272770659, 59.30378426403790115 ) ) ;
#5982=ADVANCED_FACE ( 'NONE', ( #17522 ), #40653, .T. ) ;
#5983=ORIENTED_EDGE ( 'NONE', *, *, #34771, .T. ) ;
#5985=DIRECTION ( 'NONE',  ( -2.662580024931131981E-06, 1.091441817331640981E-05, -0.9999999999368931469 ) ) ;
#5986=CARTESIAN_POINT ( 'NONE',  ( -23.44004476468150600, -11.23011772834392730, 73.66193342791716248 ) ) ;
#5987=CARTESIAN_POINT ( 'NONE',  ( -24.15927579118118373, -17.99354550443843692, 59.10404166857890829 ) ) ;
#5988=( BOUNDED_SURFACE ( )  B_SPLINE_SURFACE ( 3, 1, ( 
 ( #46746, #38865 ),
 ( #4653, #12517 ),
 ( #5142, #42809 ),
 ( #27780, #24095 ),
 ( #12989, #28017 ),
 ( #34922, #5638 ),
 ( #35640, #31959 ) ),
 .UNSPECIFIED., .T., .F., .F. ) 
 B_SPLINE_SURFACE_WITH_KNOTS ( ( 4, 3, 4 ),
 ( 2, 2 ),
 ( 0.000000000000000000, 0.5000000000000000000, 1.000000000000000000 ),
 ( 0.000000000000000000, 1.000000000000000000 ),
 .UNSPECIFIED. ) 
 GEOMETRIC_REPRESENTATION_ITEM ( )  RATIONAL_B_SPLINE_SURFACE ( (
 ( 1.000000000000000000, 1.000000000000000000),
 ( 0.3333333333333335369, 0.3333333333333330373),
 ( 0.3333333333333335369, 0.3333333333333330373),
 ( 1.000000000000000000, 1.000000000000000000),
 ( 0.3333333333333333703, 0.3333333333333333703),
 ( 0.3333333333333333703, 0.3333333333333333703),
 ( 1.000000000000000000, 1.000000000000000000) ) ) 
 REPRESENTATION_ITEM ( '' )  SURFACE ( )  );
#5989=FACE_OUTER_BOUND ( 'NONE', #14351, .T. ) ;
#5990=CARTESIAN_POINT ( 'NONE',  ( -17.42409385541300892, -14.80920654474439502, 75.49999999999994316 ) ) ;
#5991=VERTEX_POINT ( 'NONE', #25638 ) ;
#5996=CARTESIAN_POINT ( 'NONE',  ( -13.27361356051800456, -9.172254427053855963, 63.90946478016504528 ) ) ;
#5997=ADVANCED_FACE ( 'NONE', ( #28620 ), #43414, .T. ) ;
#5998=CARTESIAN_POINT ( 'NONE',  ( -14.10256395084115866, -8.140532207465255965, 70.84462205307964666 ) ) ;
#6000=( BOUNDED_CURVE ( )  B_SPLINE_CURVE ( 3, ( #34237, #15028, #11854, #22697 ),
 .UNSPECIFIED., .F., .F. ) 
 B_SPLINE_CURVE_WITH_KNOTS ( ( 4, 4 ),
 ( 0.9074455897393707282, 1.000000000000000000 ),
 .UNSPECIFIED. ) 
 CURVE ( )  GEOMETRIC_REPRESENTATION_ITEM ( )  RATIONAL_B_SPLINE_CURVE ( ( 0.6983129098261133816, 0.7760317562607157438, 0.8765941196520112833, 1.000000000000000000 ) ) 
 REPRESENTATION_ITEM ( '' )  );
#6002=ORIENTED_EDGE ( 'NONE', *, *, #38018, .T. ) ;
#6003=CARTESIAN_POINT ( 'NONE',  ( -21.10139403845883876, -20.76557291098659164, 65.65741929463816007 ) ) ;
#6006=ORIENTED_EDGE ( 'NONE', *, *, #9217, .T. ) ;
#6007=CARTESIAN_POINT ( 'NONE',  ( -24.41887989321793739, -14.52796132729743839, 66.19909327358298867 ) ) ;
#6009=( BOUNDED_SURFACE ( )  B_SPLINE_SURFACE ( 3, 1, ( 
 ( #20104, #5095 ),
 ( #35111, #1378 ),
 ( #16397, #31425 ),
 ( #30637, #4513 ),
 ( #1064, #15575 ),
 ( #12383, #4047 ),
 ( #27406, #38228 ) ),
 .UNSPECIFIED., .T., .F., .F. ) 
 B_SPLINE_SURFACE_WITH_KNOTS ( ( 4, 3, 4 ),
 ( 2, 2 ),
 ( 0.000000000000000000, 0.5000000000000000000, 1.000000000000000000 ),
 ( 0.000000000000000000, 1.000000000000000000 ),
 .UNSPECIFIED. ) 
 GEOMETRIC_REPRESENTATION_ITEM ( )  RATIONAL_B_SPLINE_SURFACE ( (
 ( 1.000000000000000000, 1.000000000000000000),
 ( 0.3333333333333335369, 0.3333333333333330373),
 ( 0.3333333333333335369, 0.3333333333333330373),
 ( 1.000000000000000000, 1.000000000000000000),
 ( 0.3333333333333333703, 0.3333333333333333703),
 ( 0.3333333333333333703, 0.3333333333333333703),
 ( 1.000000000000000000, 1.000000000000000000) ) ) 
 REPRESENTATION_ITEM ( '' )  SURFACE ( )  );
#6010=ORIENTED_EDGE ( 'NONE', *, *, #961, .F. ) ;
#6012=FACE_OUTER_BOUND ( 'NONE', #47417, .T. ) ;
#6013=ORIENTED_EDGE ( 'NONE', *, *, #12947, .F. ) ;
#6017=CARTESIAN_POINT ( 'NONE',  ( -24.70004435018021383, -13.20802528152527877, 59.46929592674912612 ) ) ;
#6019=CARTESIAN_POINT ( 'NONE',  ( -14.41058011727219501, -8.490943137660508455, 67.55975084671482023 ) ) ;
#6021=DIRECTION ( 'NONE',  ( 0.6771828760946864145, -0.7358147540815750398, 3.419290845356542170E-09 ) ) ;
#6023=VECTOR ( 'NONE', #5344, 1000.000000000000000 ) ;
#6024=PLANE ( 'NONE',  #6929 ) ;
#6025=CARTESIAN_POINT ( 'NONE',  ( -20.12289122552838094, -7.865124802246414859, 73.90591932823114973 ) ) ;
#6026=CYLINDRICAL_SURFACE ( 'NONE', #9766, 0.1499999999999963862 ) ;
#6029=ORIENTED_EDGE ( 'NONE', *, *, #22622, .F. ) ;
#6030=FACE_OUTER_BOUND ( 'NONE', #41333, .T. ) ;
#6031=CARTESIAN_POINT ( 'NONE',  ( -16.55451525393793233, -12.46531383050667863, 77.49999999999994316 ) ) ;
#6032=CARTESIAN_POINT ( 'NONE',  ( -13.34910288913403065, -20.50135726297604677, 58.06266769909647962 ) ) ;
#6035=CARTESIAN_POINT ( 'NONE',  ( -19.48731947536727915, -21.55887828695198039, 69.07915298548451233 ) ) ;
#6036=ORIENTED_EDGE ( 'NONE', *, *, #23706, .T. ) ;
#6038=ORIENTED_EDGE ( 'NONE', *, *, #824, .F. ) ;
#6039=CARTESIAN_POINT ( 'NONE',  ( -10.03202132150386383, -15.73778161007442833, 61.17642517804716817 ) ) ;
#6040=CARTESIAN_POINT ( 'NONE',  ( -23.11919578175225354, -18.88151874835563859, 66.05219398271668751 ) ) ;
#6041=CARTESIAN_POINT ( 'NONE',  ( -15.94639903137639791, -7.966892978607620357, 63.74298973210061803 ) ) ;
#6043=VERTEX_POINT ( 'NONE', #43651 ) ;
#6047=CARTESIAN_POINT ( 'NONE',  ( -20.66122932390920752, -21.07544863110783950, 62.52960166509647166 ) ) ;
#6048=CARTESIAN_POINT ( 'NONE',  ( -24.09731288006578609, -16.92300596032393045, 72.99222104724324822 ) ) ;
#6049=ADVANCED_FACE ( 'NONE', ( #36467 ), #46116, .T. ) ;
#6051=VECTOR ( 'NONE', #19863, 1000.000000000000000 ) ;
#6053=ORIENTED_EDGE ( 'NONE', *, *, #10371, .T. ) ;
#6055=CARTESIAN_POINT ( 'NONE',  ( -24.80769047312930553, -15.80232199467591947, 69.71802767292497549 ) ) ;
#6056=EDGE_CURVE ( 'NONE', #35176, #14422, #2271, .T. ) ;
#6057=AXIS2_PLACEMENT_3D ( 'NONE', #40460, #21526, #36506 ) ;
#6059=CARTESIAN_POINT ( 'NONE',  ( -11.27324661094954550, -11.46480969376360726, 67.84694496584526746 ) ) ;
#6060=B_SPLINE_CURVE_WITH_KNOTS ( 'NONE', 3,
 ( #8433, #23461, #16281, #38461, #9411, #19768, #31321, #35245, #5226, #4745 ),
 .UNSPECIFIED., .F., .F.,
 ( 4, 2, 2, 2, 4 ),
 ( 0.000000000000000000, 0.2500000000000000000, 0.5000000000000000000, 0.7500000000000000000, 1.000000000000000000 ),
 .UNSPECIFIED. ) ;
#6062=B_SPLINE_CURVE_WITH_KNOTS ( 'NONE', 3,
 ( #40157, #21681, #6900, #36664, #20958, #2949, #25607, #17961, #32980, #48023 ),
 .UNSPECIFIED., .F., .F.,
 ( 4, 2, 2, 2, 4 ),
 ( 0.6272669072976775340, 0.7522669073147194574, 0.8772669073317613808, 1.002266907348803304, 1.127266907365845228 ),
 .UNSPECIFIED. ) ;
#6064=CARTESIAN_POINT ( 'NONE',  ( -22.07805708657739885, -20.69058616546009333, 47.99999999999994316 ) ) ;
#6065=CARTESIAN_POINT ( 'NONE',  ( -14.47983227664519212, -7.965588925009814858, 63.90483403727078837 ) ) ;
#6066=ORIENTED_EDGE ( 'NONE', *, *, #18573, .T. ) ;
#6067=LINE ( 'NONE', #44008, #30542 ) ;
#6068=EDGE_CURVE ( 'NONE', #26756, #32237, #30286, .T. ) ;
#6070=DIRECTION ( 'NONE',  ( -0.8459089628457129306, -0.5333273165489313961, 7.771812504399799980E-08 ) ) ;
#6072=FACE_OUTER_BOUND ( 'NONE', #18946, .T. ) ;
#6073=ADVANCED_FACE ( 'NONE', ( #2985 ), #17994, .T. ) ;
#6074=ORIENTED_EDGE ( 'NONE', *, *, #14584, .F. ) ;
#6075=CARTESIAN_POINT ( 'NONE',  ( -24.40658474706614101, -15.78251040532600769, 69.68307488409816131 ) ) ;
#6076=CARTESIAN_POINT ( 'NONE',  ( -16.25049871934676204, -21.71175505818405682, 61.86641321701562646 ) ) ;
#6077=ORIENTED_EDGE ( 'NONE', *, *, #6521, .T. ) ;
#6078=CARTESIAN_POINT ( 'NONE',  ( -13.17786431350945797, -8.687616865786688791, 60.56137482248813342 ) ) ;
#6079=CARTESIAN_POINT ( 'NONE',  ( -24.11881394502254849, -17.01995806294775448, 73.16863963025599560 ) ) ;
#6080=CARTESIAN_POINT ( 'NONE',  ( -13.49267557974227394, -8.956801037788498121, 60.45422421514565059 ) ) ;
#6081=CYLINDRICAL_SURFACE ( 'NONE', #45558, 0.1500000000000007716 ) ;
#6082=EDGE_LOOP ( 'NONE', ( #4939, #15803 ) ) ;
#6085=CARTESIAN_POINT ( 'NONE',  ( -23.80338573481879294, -11.80731802715296119, 59.76763678108634537 ) ) ;
#6086=B_SPLINE_CURVE_WITH_KNOTS ( 'NONE', 3,
 ( #40261, #21546, #36529, #26206, #23017, #33314, #11420, #34064, #48354, #40979 ),
 .UNSPECIFIED., .F., .F.,
 ( 4, 2, 2, 2, 4 ),
 ( 0.000000000000000000, 0.2500000000000000000, 0.5000000000000000000, 0.7500000000000000000, 1.000000000000000000 ),
 .UNSPECIFIED. ) ;
#6088=CARTESIAN_POINT ( 'NONE',  ( -16.54207536886490004, -21.80396438979022022, 65.23124200709338538 ) ) ;
#6090=CARTESIAN_POINT ( 'NONE',  ( -11.18274741528775884, -18.87723868614961731, 64.85432942596317218 ) ) ;
#6091=AXIS2_PLACEMENT_3D ( 'NONE', #22162, #17713, #48013 ) ;
#6092=CARTESIAN_POINT ( 'NONE',  ( -12.23301264461619553, -10.03852782535897958, 60.84446034103241630 ) ) ;
#6093=VERTEX_POINT ( 'NONE', #22949 ) ;
#6094=VERTEX_POINT ( 'NONE', #45601 ) ;
#6095=CARTESIAN_POINT ( 'NONE',  ( -24.43112999227502513, -15.58634490091466951, 73.00303748142292193 ) ) ;
#6101=CARTESIAN_POINT ( 'NONE',  ( -10.40689392953442294, -15.49001398589273393, 57.86233024654485035 ) ) ;
#6102=CARTESIAN_POINT ( 'NONE',  ( -12.40380818233537141, -19.68739593843253033, 61.69678633575567517 ) ) ;
#6104=CARTESIAN_POINT ( 'NONE',  ( -13.90002763284361365, -21.37314463245085250, 72.04794927803091298 ) ) ;
#6105=EDGE_LOOP ( 'NONE', ( #42446, #33619, #41323, #21958, #39428 ) ) ;
#6106=VERTEX_POINT ( 'NONE', #25889 ) ;
#6107=CARTESIAN_POINT ( 'NONE',  ( -24.35094580881710513, -16.14095786638556973, 59.12332159045481461 ) ) ;
#6108=B_SPLINE_CURVE_WITH_KNOTS ( 'NONE', 1,
 ( #43125, #24421 ),
 .UNSPECIFIED., .F., .F.,
 ( 2, 2 ),
 ( 0.000000000000000000, 1.000000000000000000 ),
 .UNSPECIFIED. ) ;
#6112=DIRECTION ( 'NONE',  ( 0.07061531369766044230, 0.9975036227860933913, 1.268851335910971019E-08 ) ) ;
#6113=B_SPLINE_CURVE_WITH_KNOTS ( 'NONE', 3,
 ( #27177, #16071, #19800, #35280, #31114, #35035, #34551, #38234, #12875, #12159 ),
 .UNSPECIFIED., .F., .F.,
 ( 4, 2, 2, 2, 4 ),
 ( 0.1272669073658370675, 0.2522669073488581493, 0.3772669073318791755, 0.5022669073149002017, 0.6272669072979213389 ),
 .UNSPECIFIED. ) ;
#6115=ORIENTED_EDGE ( 'NONE', *, *, #27796, .F. ) ;
#6117=CARTESIAN_POINT ( 'NONE',  ( -23.58616520728616806, -18.99640775243969060, 66.00884813586510802 ) ) ;
#6123=ORIENTED_EDGE ( 'NONE', *, *, #1705, .T. ) ;
#6126=CYLINDRICAL_SURFACE ( 'NONE', #42444, 0.1499999999999948874 ) ;
#6127=CARTESIAN_POINT ( 'NONE',  ( -12.74585782473854145, -9.602005322742989790, 74.39210991189573008 ) ) ;
#6129=CARTESIAN_POINT ( 'NONE',  ( -24.59706333651279664, -12.79617740830267891, 66.48742133194130588 ) ) ;
#6130=( BOUNDED_SURFACE ( )  B_SPLINE_SURFACE ( 3, 1, ( 
 ( #42424, #27388 ),
 ( #1048, #31324 ),
 ( #24185, #27868 ),
 ( #38210, #42668 ),
 ( #20006, #8693 ),
 ( #16044, #46355 ),
 ( #35248, #46105 ) ),
 .UNSPECIFIED., .T., .F., .F. ) 
 B_SPLINE_SURFACE_WITH_KNOTS ( ( 4, 3, 4 ),
 ( 2, 2 ),
 ( 0.000000000000000000, 0.5000000000000000000, 1.000000000000000000 ),
 ( 0.000000000000000000, 1.000000000000000000 ),
 .UNSPECIFIED. ) 
 GEOMETRIC_REPRESENTATION_ITEM ( )  RATIONAL_B_SPLINE_SURFACE ( (
 ( 1.000000000000000000, 1.000000000000000000),
 ( 0.3333333333333335369, 0.3333333333333330373),
 ( 0.3333333333333335369, 0.3333333333333330373),
 ( 1.000000000000000000, 1.000000000000000000),
 ( 0.3333333333333333703, 0.3333333333333333703),
 ( 0.3333333333333333703, 0.3333333333333333703),
 ( 1.000000000000000000, 1.000000000000000000) ) ) 
 REPRESENTATION_ITEM ( '' )  SURFACE ( )  );
#6132=CARTESIAN_POINT ( 'NONE',  ( -16.19792114999740562, -7.866354181730329742, 60.48556343814865954 ) ) ;
#6133=VERTEX_POINT ( 'NONE', #3726 ) ;
#6135=AXIS2_PLACEMENT_3D ( 'NONE', #12096, #8897, #16010 ) ;
#6136=EDGE_CURVE ( 'NONE', #13199, #20304, #36031, .T. ) ;
#6137=ORIENTED_EDGE ( 'NONE', *, *, #7030, .T. ) ;
#6138=CARTESIAN_POINT ( 'NONE',  ( -23.83043763270304183, -11.86620476845630101, 59.48235732590898550 ) ) ;
#6139=CARTESIAN_POINT ( 'NONE',  ( -10.21961014573118121, -12.91218125089532265, 67.93106486834143709 ) ) ;
#6140=VERTEX_POINT ( 'NONE', #7433 ) ;
#6141=ADVANCED_FACE ( 'NONE', ( #521, #14519 ), #22440, .T. ) ;
#6142=ADVANCED_FACE ( 'NONE', ( #37431 ), #37938, .T. ) ;
#6143=EDGE_CURVE ( 'NONE', #39245, #46590, #31309, .T. ) ;
#6144=PLANE ( 'NONE',  #28171 ) ;
#6145=CARTESIAN_POINT ( 'NONE',  ( -12.74836358285320159, -20.08597126951521261, 71.82125749157572159 ) ) ;
#6148=FACE_OUTER_BOUND ( 'NONE', #14736, .T. ) ;
#6149=CARTESIAN_POINT ( 'NONE',  ( -14.97035482569482312, -21.41873484682592377, 61.92128389535452015 ) ) ;
#6151=CARTESIAN_POINT ( 'NONE',  ( -18.16355857556227349, -7.327338257757846307, 53.76227901944321985 ) ) ;
#6152=( BOUNDED_CURVE ( )  B_SPLINE_CURVE ( 3, ( #43395, #1778, #24439, #20733 ),
 .UNSPECIFIED., .F., .F. ) 
 B_SPLINE_CURVE_WITH_KNOTS ( ( 4, 4 ),
 ( 0.9074455897393637338, 1.000000000000000000 ),
 .UNSPECIFIED. ) 
 CURVE ( )  GEOMETRIC_REPRESENTATION_ITEM ( )  RATIONAL_B_SPLINE_CURVE ( ( 0.6983129098260837386, 0.7760317562606902086, 0.8765941196519956291, 1.000000000000000000 ) ) 
 REPRESENTATION_ITEM ( '' )  );
#6153=CARTESIAN_POINT ( 'NONE',  ( -10.96500202619968256, -18.52180277100054795, 58.00052909868417572 ) ) ;
#6154=CARTESIAN_POINT ( 'NONE',  ( -12.00560918470589122, -10.37740546741846615, 67.51399311695257666 ) ) ;
#6156=EDGE_LOOP ( 'NONE', ( #35115, #39314, #34346, #11811, #10661 ) ) ;
#6157=ORIENTED_EDGE ( 'NONE', *, *, #31153, .F. ) ;
#6158=DIRECTION ( 'NONE',  ( 2.117869074558178593E-07, 2.255668799892331646E-07, 0.9999999999999520384 ) ) ;
#6159=CARTESIAN_POINT ( 'NONE',  ( -24.30032712313099807, -16.12036388816417798, 62.89328623440644606 ) ) ;
#6161=CARTESIAN_POINT ( 'NONE',  ( -17.00410623003636346, -7.771727578618798482, 74.11018273220987851 ) ) ;
#6163=CARTESIAN_POINT ( 'NONE',  ( -15.85230412793554144, -7.936612759385449856, 67.44007248260970755 ) ) ;
#6166=CARTESIAN_POINT ( 'NONE',  ( -20.58582848812473642, -8.063211782720200560, 66.92070701425123502 ) ) ;
#6167=AXIS2_PLACEMENT_3D ( 'NONE', #27403, #42438, #8708 ) ;
#6168=VECTOR ( 'NONE', #7061, 1000.000000000000114 ) ;
#6169=ORIENTED_EDGE ( 'NONE', *, *, #11792, .T. ) ;
#6170=CARTESIAN_POINT ( 'NONE',  ( -11.89386644692969597, -19.18772505311030230, 71.68685609106418610 ) ) ;
#6171=EDGE_CURVE ( 'NONE', #1629, #26191, #9027, .T. ) ;
#6172=CARTESIAN_POINT ( 'NONE',  ( -13.01353307917097268, -8.804980454159759162, 64.09441913135431435 ) ) ;
#6174=LINE ( 'NONE', #38933, #1234 ) ;
#6176=ORIENTED_EDGE ( 'NONE', *, *, #18895, .T. ) ;
#6177=ORIENTED_EDGE ( 'NONE', *, *, #16020, .F. ) ;
#6178=CARTESIAN_POINT ( 'NONE',  ( -17.52853272358826686, -7.759682304905023642, 63.83584969886392457 ) ) ;
#6179=CARTESIAN_POINT ( 'NONE',  ( -13.93897074462874919, -20.93787812888889377, 68.74153005185598886 ) ) ;
#6180=CARTESIAN_POINT ( 'NONE',  ( -10.00588775665706898, -14.11983824440616075, 61.07854638698739791 ) ) ;
#6182=CARTESIAN_POINT ( 'NONE',  ( -23.95182099924141994, -17.47225880813607901, 65.94357235735444078 ) ) ;
#6183=CARTESIAN_POINT ( 'NONE',  ( -12.65882755920527458, -9.609488432089360543, 74.20434181795738482 ) ) ;
#6185=PLANE ( 'NONE',  #36271 ) ;
#6186=VECTOR ( 'NONE', #44368, 1000.000000000000000 ) ;
#6187=CARTESIAN_POINT ( 'NONE',  ( -12.88213326721828089, -9.482801177541238857, 71.04028493289825974 ) ) ;
#6189=CARTESIAN_POINT ( 'NONE',  ( -23.13015969901951863, -18.95476373626217281, 58.76921843841908810 ) ) ;
#6190=ORIENTED_EDGE ( 'NONE', *, *, #46226, .F. ) ;
#6191=CARTESIAN_POINT ( 'NONE',  ( -14.72778340125292651, -21.32322296975913289, 58.46617885012761917 ) ) ;
#6194=CARTESIAN_POINT ( 'NONE',  ( -24.87384330655416420, -14.87999779688033719, 59.35804910119406230 ) ) ;
#6195=CARTESIAN_POINT ( 'NONE',  ( -13.51000599947710690, -20.67303722014981204, 61.52206147836523087 ) ) ;
#6198=FACE_OUTER_BOUND ( 'NONE', #37888, .T. ) ;
#6201=CARTESIAN_POINT ( 'NONE',  ( -20.15891617451884699, -21.73914053226047827, 72.51140444708435950 ) ) ;
#6202=CARTESIAN_POINT ( 'NONE',  ( -12.74071866071660075, -9.015263582886822391, 70.96429948631303830 ) ) ;
#6203=AXIS2_PLACEMENT_3D ( 'NONE', #38287, #12691, #30936 ) ;
#6204=FACE_OUTER_BOUND ( 'NONE', #28060, .T. ) ;
#6206=CARTESIAN_POINT ( 'NONE',  ( -20.64396943983181743, -21.02470340508176250, 58.94475165022391394 ) ) ;
#6207=VERTEX_POINT ( 'NONE', #7682 ) ;
#6208=DIRECTION ( 'NONE',  ( -5.297746385676333075E-06, -8.914243328957358747E-06, -0.9999999999462351186 ) ) ;
#6209=CARTESIAN_POINT ( 'NONE',  ( -11.87947861617434064, -19.08215629584865525, 71.91359129046459486 ) ) ;
#6210=CARTESIAN_POINT ( 'NONE',  ( -22.68035891289124351, -20.08887660193805047, 69.28079699623869203 ) ) ;
#6211=EDGE_CURVE ( 'NONE', #37990, #15682, #23215, .T. ) ;
#6212=ADVANCED_FACE ( 'NONE', ( #38671 ), #4702, .T. ) ;
#6217=VERTEX_POINT ( 'NONE', #24146 ) ;
#6218=DIRECTION ( 'NONE',  ( -0.9848822020395751053, 0.1732254256905498280, 7.367703375004543066E-08 ) ) ;
#6219=VERTEX_POINT ( 'NONE', #8396 ) ;
#6220=CARTESIAN_POINT ( 'NONE',  ( -11.67943375510494697, -18.89645239624664441, 68.50217487844219022 ) ) ;
#6223=CARTESIAN_POINT ( 'NONE',  ( -22.58023486647882550, -9.989541079992143580, 66.69749311060769514 ) ) ;
#6225=CARTESIAN_POINT ( 'NONE',  ( -16.96658279966119309, -22.24515547448776331, 72.26519595204030111 ) ) ;
#6227=B_SPLINE_CURVE_WITH_KNOTS ( 'NONE', 3,
 ( #16741, #16508, #19976, #46576, #31783, #39162, #35695, #13048, #27841, #8902 ),
 .UNSPECIFIED., .F., .F.,
 ( 4, 2, 2, 2, 4 ),
 ( 0.1272669073658277972, 0.2522669073439269827, 0.3772669073220261127, 0.5022669073001252427, 0.6272669072782244282 ),
 .UNSPECIFIED. ) ;
#6228=CARTESIAN_POINT ( 'NONE',  ( -12.74613139958686503, -9.010845216743291530, 71.02738122373636998 ) ) ;
#6230=CARTESIAN_POINT ( 'NONE',  ( -20.88122380307280324, -20.95354100073119241, 62.40911604053530226 ) ) ;
#6231=CARTESIAN_POINT ( 'NONE',  ( -20.24919536711601964, -8.341303680600599790, 63.46688622775676691 ) ) ;
#6232=B_SPLINE_CURVE_WITH_KNOTS ( 'NONE', 3,
 ( #17686, #16953, #47270, #17456, #47509, #13509, #43338, #28553, #9611, #20682 ),
 .UNSPECIFIED., .F., .F.,
 ( 4, 2, 2, 2, 4 ),
 ( 0.1272669073657963779, 0.2522669073462850964, 0.3772669073267738149, 0.5022669073072625334, 0.6272669072877512519 ),
 .UNSPECIFIED. ) ;
#6234=ORIENTED_EDGE ( 'NONE', *, *, #10241, .T. ) ;
#6239=CARTESIAN_POINT ( 'NONE',  ( -13.20366469342568294, -8.669938804193677129, 60.63939044432547831 ) ) ;
#6241=CARTESIAN_POINT ( 'NONE',  ( -24.59706363142188934, -12.79617847886399140, 66.48742024426742603 ) ) ;
#6242=CARTESIAN_POINT ( 'NONE',  ( -13.86839427437450745, -20.83888320357228352, 65.17731955186617654 ) ) ;
#6243=CARTESIAN_POINT ( 'NONE',  ( -16.39155882215229099, -21.78318466615559146, 61.90568132352964881 ) ) ;
#6245=VECTOR ( 'NONE', #6528, 1000.000000000000114 ) ;
#6249=PLANE ( 'NONE',  #43748 ) ;
#6250=CARTESIAN_POINT ( 'NONE',  ( -19.99112977906324318, -8.296885409642934306, 74.02096600045412345 ) ) ;
#6251=VECTOR ( 'NONE', #44934, 1000.000000000000227 ) ;
#6252=CARTESIAN_POINT ( 'NONE',  ( -15.68503317936312413, -7.977064329016499755, 70.60989839961001735 ) ) ;
#6253=CARTESIAN_POINT ( 'NONE',  ( -13.94386542258548189, -20.88289783676623657, 68.45625091214465385 ) ) ;
#6254=ORIENTED_EDGE ( 'NONE', *, *, #23073, .F. ) ;
#6255=CARTESIAN_POINT ( 'NONE',  ( -11.00024241808776004, -11.03596260037739007, 60.78547452563873321 ) ) ;
#6257=EDGE_LOOP ( 'NONE', ( #33567, #38090, #44823, #45476, #28498 ) ) ;
#6261=FACE_OUTER_BOUND ( 'NONE', #22854, .T. ) ;
#6262=VERTEX_POINT ( 'NONE', #39150 ) ;
#6263=CARTESIAN_POINT ( 'NONE',  ( -11.71918404020638427, -18.95175453447548009, 71.70158022526054253 ) ) ;
#6264=EDGE_CURVE ( 'NONE', #27202, #7586, #27912, .T. ) ;
#6265=VECTOR ( 'NONE', #43453, 1000.000000000000114 ) ;
#6266=CARTESIAN_POINT ( 'NONE',  ( -16.66975460573832635, -21.76850464344978420, 65.51098995538828262 ) ) ;
#6267=CARTESIAN_POINT ( 'NONE',  ( -10.77500719466768686, -17.16388024452267302, 57.68760401228323076 ) ) ;
#6268=VERTEX_POINT ( 'NONE', #12805 ) ;
#6270=AXIS2_PLACEMENT_3D ( 'NONE', #28983, #21838, #39582 ) ;
#6271=CARTESIAN_POINT ( 'NONE',  ( -23.23616624490289695, -18.79948399208958776, 66.12389430041484673 ) ) ;
#6273=ADVANCED_FACE ( 'NONE', ( #5438 ), #27830, .T. ) ;
#6274=CARTESIAN_POINT ( 'NONE',  ( -20.12289122552838094, -7.865124802246414859, 73.90591932823114973 ) ) ;
#6276=CARTESIAN_POINT ( 'NONE',  ( -13.29845767883066543, -21.01266560759323809, 61.63150935275904629 ) ) ;
#6277=CARTESIAN_POINT ( 'NONE',  ( -22.04378365035703879, -20.13510231884741231, 62.24911246861644543 ) ) ;
#6281=EDGE_CURVE ( 'NONE', #17592, #30297, #22842, .T. ) ;
#6284=( BOUNDED_SURFACE ( )  B_SPLINE_SURFACE ( 3, 1, ( 
 ( #46324, #39648 ),
 ( #42639, #8899 ),
 ( #39411, #38920 ),
 ( #20206, #35218 ),
 ( #24400, #24154 ),
 ( #16505, #39159 ),
 ( #5446, #16738 ) ),
 .UNSPECIFIED., .T., .F., .F. ) 
 B_SPLINE_SURFACE_WITH_KNOTS ( ( 4, 3, 4 ),
 ( 2, 2 ),
 ( 0.000000000000000000, 0.5000000000000000000, 1.000000000000000000 ),
 ( 0.000000000000000000, 1.000000000000000000 ),
 .UNSPECIFIED. ) 
 GEOMETRIC_REPRESENTATION_ITEM ( )  RATIONAL_B_SPLINE_SURFACE ( (
 ( 1.000000000000000000, 1.000000000000000000),
 ( 0.3333333333333335369, 0.3333333333333330373),
 ( 0.3333333333333335369, 0.3333333333333330373),
 ( 1.000000000000000000, 1.000000000000000000),
 ( 0.3333333333333333703, 0.3333333333333333703),
 ( 0.3333333333333333703, 0.3333333333333333703),
 ( 1.000000000000000000, 1.000000000000000000) ) ) 
 REPRESENTATION_ITEM ( '' )  SURFACE ( )  );
#6286=DIRECTION ( 'NONE',  ( -0.7300417127692488961, -0.6834025882427879894, -6.612978995310452690E-09 ) ) ;
#6288=ORIENTED_EDGE ( 'NONE', *, *, #21154, .F. ) ;
#6289=ORIENTED_EDGE ( 'NONE', *, *, #7217, .T. ) ;
#6291=DIRECTION ( 'NONE',  ( 1.896855589267346620E-06, 2.136244919385519396E-06, 0.9999999999959191532 ) ) ;
#6292=CARTESIAN_POINT ( 'NONE',  ( -12.86353962931362283, -9.432586330540292607, 74.33395128836551180 ) ) ;
#6293=( BOUNDED_CURVE ( )  B_SPLINE_CURVE ( 3, ( #27843, #42873, #9142, #5452 ),
 .UNSPECIFIED., .F., .F. ) 
 B_SPLINE_CURVE_WITH_KNOTS ( ( 4, 4 ),
 ( 0.5000000000000000000, 0.9074455897393632897 ),
 .UNSPECIFIED. ) 
 CURVE ( )  GEOMETRIC_REPRESENTATION_ITEM ( )  RATIONAL_B_SPLINE_CURVE ( ( 1.000000000000006217, 0.4567392136813389625, 0.3561768502900283240, 0.6983129098260811851 ) ) 
 REPRESENTATION_ITEM ( '' )  );
#6294=EDGE_LOOP ( 'NONE', ( #40544, #15403 ) ) ;
#6297=B_SPLINE_CURVE_WITH_KNOTS ( 'NONE', 3,
 ( #9958, #18048, #22007, #43704, #10453, #6513, #47147, #25691, #2800, #39996 ),
 .UNSPECIFIED., .F., .F.,
 ( 4, 2, 2, 2, 4 ),
 ( 0.000000000000000000, 0.2500000000000000000, 0.5000000000000000000, 0.7500000000000000000, 1.000000000000000000 ),
 .UNSPECIFIED. ) ;
#6298=AXIS2_PLACEMENT_3D ( 'NONE', #14950, #30010, #11526 ) ;
#6299=CARTESIAN_POINT ( 'NONE',  ( -14.32933440466380048, -7.972462762251764978, 54.15157107980258644 ) ) ;
#6300=CARTESIAN_POINT ( 'NONE',  ( -23.19494370299929287, -18.77118727246694263, 65.82389430425217824 ) ) ;
#6301=B_SPLINE_CURVE_WITH_KNOTS ( 'NONE', 1,
 ( #31454, #8826 ),
 .UNSPECIFIED., .F., .F.,
 ( 2, 2 ),
 ( 0.000000000000000000, 1.000000000000000000 ),
 .UNSPECIFIED. ) ;
#6304=VERTEX_POINT ( 'NONE', #12570 ) ;
#6305=DIRECTION ( 'NONE',  ( 0.2853368233144803479, -0.3443586753093368369, 0.8944271909999158554 ) ) ;
#6306=CYLINDRICAL_SURFACE ( 'NONE', #20510, 0.1499999999999981903 ) ;
#6307=AXIS2_PLACEMENT_3D ( 'NONE', #28310, #21871, #21159 ) ;
#6310=CARTESIAN_POINT ( 'NONE',  ( -11.21157534608376061, -11.58358818987947814, 67.91864608155252370 ) ) ;
#6311=ORIENTED_EDGE ( 'NONE', *, *, #33423, .T. ) ;
#6312=CARTESIAN_POINT ( 'NONE',  ( -14.63391651318349851, -8.330799758808863587, 67.55975079407809858 ) ) ;
#6313=B_SPLINE_CURVE_WITH_KNOTS ( 'NONE', 3,
 ( #17382, #40514, #6792, #32419, #2127, #36801, #13437, #9776, #32647, #10724 ),
 .UNSPECIFIED., .F., .F.,
 ( 4, 2, 2, 2, 4 ),
 ( 0.000000000000000000, 0.2500000000000000000, 0.5000000000000000000, 0.7500000000000000000, 1.000000000000000000 ),
 .UNSPECIFIED. ) ;
#6316=ORIENTED_EDGE ( 'NONE', *, *, #47059, .T. ) ;
#6317=CARTESIAN_POINT ( 'NONE',  ( -22.79851114622174180, -10.32406479491737983, 63.29859279992308529 ) ) ;
#6321=PLANE ( 'NONE',  #38009 ) ;
#6322=ORIENTED_EDGE ( 'NONE', *, *, #17688, .F. ) ;
#6323=CARTESIAN_POINT ( 'NONE',  ( -15.65034338963778460, -22.11529786783383145, 54.02312124697527906 ) ) ;
#6324=DIRECTION ( 'NONE',  ( -0.1555549491741979040, -0.4192882752801621038, 0.8944271909999157444 ) ) ;
#6325=ORIENTED_EDGE ( 'NONE', *, *, #37987, .T. ) ;
#6326=LINE ( 'NONE', #13203, #45515 ) ;
#6327=CARTESIAN_POINT ( 'NONE',  ( -24.65581703702211414, -13.01900205834191127, 62.93240538826285047 ) ) ;
#6330=B_SPLINE_CURVE_WITH_KNOTS ( 'NONE', 1,
 ( #8793, #16391 ),
 .UNSPECIFIED., .F., .F.,
 ( 2, 2 ),
 ( 0.000000000000000000, 1.000000000000000000 ),
 .UNSPECIFIED. ) ;
#6331=FACE_OUTER_BOUND ( 'NONE', #1599, .T. ) ;
#6333=DIRECTION ( 'NONE',  ( -0.05957303659011964347, -0.9982239494779874267, 2.515684304538401319E-08 ) ) ;
#6335=CARTESIAN_POINT ( 'NONE',  ( -10.89280251029460622, -11.22507333849785027, 64.33377325762776877 ) ) ;
#6338=CARTESIAN_POINT ( 'NONE',  ( -10.16947401241056248, -13.11399914557070190, 71.31490259464086989 ) ) ;
#6340=CARTESIAN_POINT ( 'NONE',  ( -24.77336880027706911, -16.03019386047689210, 66.16301287370103523 ) ) ;
#6342=ORIENTED_EDGE ( 'NONE', *, *, #9959, .F. ) ;
#6343=CARTESIAN_POINT ( 'NONE',  ( -14.60783717270099835, -21.70648693424663378, 58.35113322083577003 ) ) ;
#6344=CARTESIAN_POINT ( 'NONE',  ( -15.55206243756419404, -8.064171445415857065, 70.80092926608037374 ) ) ;
#6345=CARTESIAN_POINT ( 'NONE',  ( -13.82689732469268407, -20.87277619789260186, 68.47097268802275494 ) ) ;
#6347=CARTESIAN_POINT ( 'NONE',  ( -10.10901086070973420, -13.39385379864076242, 74.79162305847758319 ) ) ;
#6348=CARTESIAN_POINT ( 'NONE',  ( -19.43549419715917281, -7.635817758345905482, 60.15431310326993497 ) ) ;
#6350=CARTESIAN_POINT ( 'NONE',  ( -21.22541856475621103, -21.21643550156703384, 65.68430309725735583 ) ) ;
#6351=CARTESIAN_POINT ( 'NONE',  ( -20.03282965983824226, -21.84088468745754597, 75.49999999999994316 ) ) ;
#6352=CARTESIAN_POINT ( 'NONE',  ( -17.78355931627749698, -7.367830628488608369, 60.27334926503960588 ) ) ;
#6355=CARTESIAN_POINT ( 'NONE',  ( -24.83245720896766073, -15.59649170587275258, 73.04657806100746598 ) ) ;
#6357=CARTESIAN_POINT ( 'NONE',  ( -23.07412303265485320, -9.953122545109609476, 66.71899143667852172 ) ) ;
#6358=CARTESIAN_POINT ( 'NONE',  ( -14.85449503969317497, -21.32098759628606643, 61.91983833741223719 ) ) ;
#6359=LINE ( 'NONE', #21855, #27224 ) ;
#6360=CARTESIAN_POINT ( 'NONE',  ( -24.41897151118743636, -17.37347349776957017, 69.59835227440868266 ) ) ;
#6364=CARTESIAN_POINT ( 'NONE',  ( -14.79906637807316550, -21.78150152883456059, 61.67954536979805624 ) ) ;
#6366=AXIS2_PLACEMENT_3D ( 'NONE', #43771, #18118, #6579 ) ;
#6367=CARTESIAN_POINT ( 'NONE',  ( -23.54569140518488624, -19.05536029250058050, 65.93894040291287695 ) ) ;
#6369=EDGE_CURVE ( 'NONE', #300, #25885, #24415, .T. ) ;
#6370=ORIENTED_EDGE ( 'NONE', *, *, #43862, .T. ) ;
#6371=AXIS2_PLACEMENT_3D ( 'NONE', #6975, #21995, #30372 ) ;
#6372=B_SPLINE_CURVE_WITH_KNOTS ( 'NONE', 1,
 ( #12367, #27389 ),
 .UNSPECIFIED., .F., .F.,
 ( 2, 2 ),
 ( 0.000000000000000000, 1.000000000000000000 ),
 .UNSPECIFIED. ) ;
#6373=CARTESIAN_POINT ( 'NONE',  ( -10.59464835643876413, -16.34528333370979780, 71.67423614857023040 ) ) ;
#6374=CARTESIAN_POINT ( 'NONE',  ( -12.84719740098974583, -9.512790884556105553, 74.61923006383901225 ) ) ;
#6376=CARTESIAN_POINT ( 'NONE',  ( -15.62101046192594289, -7.580605815997546237, 70.72494447658496597 ) ) ;
#6377=CARTESIAN_POINT ( 'NONE',  ( -20.78299823145727387, -8.610459808214880439, 59.85597358678664648 ) ) ;
#6378=VERTEX_POINT ( 'NONE', #41561 ) ;
#6381=ORIENTED_EDGE ( 'NONE', *, *, #618, .T. ) ;
#6382=CARTESIAN_POINT ( 'NONE',  ( -22.23733845922741637, -19.96043711175405733, 66.00421731380804147 ) ) ;
#6383=B_SPLINE_CURVE_WITH_KNOTS ( 'NONE', 3,
 ( #23591, #42550, #1654, #20126, #4879, #5609, #46485, #39321, #35133, #27030 ),
 .UNSPECIFIED., .F., .F.,
 ( 4, 2, 2, 2, 4 ),
 ( 0.1272669073657147210, 0.2522669073438441600, 0.3772669073219735436, 0.5022669073001029272, 0.6272669072782521837 ),
 .UNSPECIFIED. ) ;
#6384=ORIENTED_EDGE ( 'NONE', *, *, #36266, .F. ) ;
#6385=FACE_OUTER_BOUND ( 'NONE', #13373, .T. ) ;
#6386=VECTOR ( 'NONE', #16843, 1000.000000000000114 ) ;
#6388=EDGE_LOOP ( 'NONE', ( #18972, #37630, #10838, #26324, #10534 ) ) ;
#6390=CARTESIAN_POINT ( 'NONE',  ( -20.78299823145727387, -8.610459808214880439, 59.85597358678664648 ) ) ;
#6393=CARTESIAN_POINT ( 'NONE',  ( -24.47217469780903443, -14.64471797168181411, 63.01296487297643267 ) ) ;
#6394=CARTESIAN_POINT ( 'NONE',  ( -17.22121256223034536, -7.361891212656819228, 70.74681744497029001 ) ) ;
#6395=EDGE_CURVE ( 'NONE', #27130, #28666, #44265, .T. ) ;
#6399=EDGE_LOOP ( 'NONE', ( #42901, #10915, #47342, #29244, #30626 ) ) ;
#6403=CARTESIAN_POINT ( 'NONE',  ( -24.69816866750256779, -16.41902046076232935, 59.16686479676427979 ) ) ;
#6404=VERTEX_POINT ( 'NONE', #4615 ) ;
#6408=FACE_OUTER_BOUND ( 'NONE', #35842, .T. ) ;
#6409=FACE_OUTER_BOUND ( 'NONE', #3743, .T. ) ;
#6410=CARTESIAN_POINT ( 'NONE',  ( -15.62222905942472018, -7.993050613273783966, 70.89517703929612935 ) ) ;
#6412=VERTEX_POINT ( 'NONE', #4373 ) ;
#6413=CARTESIAN_POINT ( 'NONE',  ( -20.54394416162392289, -8.483752705004535599, 59.72636470710568091 ) ) ;
#6414=CARTESIAN_POINT ( 'NONE',  ( -14.19282086353638839, -8.542981675383003903, 71.01485553001869278 ) ) ;
#6416=DIRECTION ( 'NONE',  ( -8.993561335472250294E-07, 8.977735684497376994E-07, 0.9999999999991925348 ) ) ;
#6418=( BOUNDED_CURVE ( )  B_SPLINE_CURVE ( 3, ( #38981, #19540, #16312, #46132 ),
 .UNSPECIFIED., .F., .F. ) 
 B_SPLINE_CURVE_WITH_KNOTS ( ( 4, 4 ),
 ( 0.4074455897393657322, 0.5000000000000000000 ),
 .UNSPECIFIED. ) 
 CURVE ( )  GEOMETRIC_REPRESENTATION_ITEM ( )  RATIONAL_B_SPLINE_CURVE ( ( 0.6983129098260999479, 0.7760317562606904307, 0.8765941196519864143, 0.9999999999999781286 ) ) 
 REPRESENTATION_ITEM ( '' )  );
#6420=EDGE_CURVE ( 'NONE', #30331, #45668, #39063, .T. ) ;
#6421=ORIENTED_EDGE ( 'NONE', *, *, #31859, .T. ) ;
#6423=ADVANCED_FACE ( 'NONE', ( #41309 ), #214, .T. ) ;
#6425=CARTESIAN_POINT ( 'NONE',  ( -20.56872696718735938, -8.555305145393857558, 60.03228400242546314 ) ) ;
#6427=CARTESIAN_POINT ( 'NONE',  ( -23.63369358133848053, -11.57797282307057607, 63.06104349419704391 ) ) ;
#6428=B_SPLINE_CURVE_WITH_KNOTS ( 'NONE', 3,
 ( #18008, #2761, #36251, #29356, #36481, #47826, #6709, #5979, #40668, #21001 ),
 .UNSPECIFIED., .F., .F.,
 ( 4, 2, 2, 2, 4 ),
 ( 0.000000000000000000, 0.2500000000000000000, 0.5000000000000000000, 0.7500000000000000000, 1.000000000000000000 ),
 .UNSPECIFIED. ) ;
#6430=CARTESIAN_POINT ( 'NONE',  ( -23.28921155407422106, -22.22116534042542213, 53.49999999999995026 ) ) ;
#6431=( BOUNDED_SURFACE ( )  B_SPLINE_SURFACE ( 3, 1, ( 
 ( #28919, #43963 ),
 ( #6523, #21544 ),
 ( #41215, #3798 ),
 ( #22262, #19055 ),
 ( #7000, #6761 ),
 ( #48119, #29904 ),
 ( #21773, #33558 ) ),
 .UNSPECIFIED., .T., .F., .F. ) 
 B_SPLINE_SURFACE_WITH_KNOTS ( ( 4, 3, 4 ),
 ( 2, 2 ),
 ( 0.000000000000000000, 0.5000000000000000000, 1.000000000000000000 ),
 ( 0.000000000000000000, 1.000000000000000000 ),
 .UNSPECIFIED. ) 
 GEOMETRIC_REPRESENTATION_ITEM ( )  RATIONAL_B_SPLINE_SURFACE ( (
 ( 1.000000000000000000, 1.000000000000000000),
 ( 0.3333333333333335369, 0.3333333333333330373),
 ( 0.3333333333333335369, 0.3333333333333330373),
 ( 1.000000000000000000, 1.000000000000000000),
 ( 0.3333333333333333703, 0.3333333333333333703),
 ( 0.3333333333333333703, 0.3333333333333333703),
 ( 1.000000000000000000, 1.000000000000000000) ) ) 
 REPRESENTATION_ITEM ( '' )  SURFACE ( )  );
#6433=( BOUNDED_SURFACE ( )  B_SPLINE_SURFACE ( 3, 1, ( 
 ( #40170, #47787 ),
 ( #32988, #18220 ),
 ( #10381, #25387 ),
 ( #43877, #36673 ),
 ( #10607, #9658 ),
 ( #2960, #48031 ),
 ( #6441, #36929 ) ),
 .UNSPECIFIED., .T., .F., .F. ) 
 B_SPLINE_SURFACE_WITH_KNOTS ( ( 4, 3, 4 ),
 ( 2, 2 ),
 ( 0.000000000000000000, 0.5000000000000000000, 1.000000000000000000 ),
 ( 0.000000000000000000, 1.000000000000000000 ),
 .UNSPECIFIED. ) 
 GEOMETRIC_REPRESENTATION_ITEM ( )  RATIONAL_B_SPLINE_SURFACE ( (
 ( 1.000000000000000000, 1.000000000000000000),
 ( 0.3333333333333335369, 0.3333333333333330373),
 ( 0.3333333333333335369, 0.3333333333333330373),
 ( 1.000000000000000000, 1.000000000000000000),
 ( 0.3333333333333333703, 0.3333333333333333703),
 ( 0.3333333333333333703, 0.3333333333333333703),
 ( 1.000000000000000000, 1.000000000000000000) ) ) 
 REPRESENTATION_ITEM ( '' )  SURFACE ( )  );
#6434=CARTESIAN_POINT ( 'NONE',  ( -16.24532195521571865, -7.452882185367804446, 60.33995147283161486 ) ) ;
#6435=B_SPLINE_CURVE_WITH_KNOTS ( 'NONE', 3,
 ( #48434, #6357, #47713, #36135, #28762, #2419, #29485, #21137, #10052, #44770 ),
 .UNSPECIFIED., .F., .F.,
 ( 4, 2, 2, 2, 4 ),
 ( 0.6272669072877826713, 0.7522669073072950630, 0.8772669073268073436, 1.002266907346319735, 1.127266907365832127 ),
 .UNSPECIFIED. ) ;
#6437=CARTESIAN_POINT ( 'NONE',  ( -11.09714801257800865, -11.68115280588511773, 64.30448977214732054 ) ) ;
#6438=ORIENTED_EDGE ( 'NONE', *, *, #45422, .T. ) ;
#6440=CARTESIAN_POINT ( 'NONE',  ( -16.97945985512182787, -21.84517132341290591, 72.16543221430227106 ) ) ;
#6441=CARTESIAN_POINT ( 'NONE',  ( -24.47066272824306665, -14.57993217219608795, 62.99824437345093031 ) ) ;
#6442=CARTESIAN_POINT ( 'NONE',  ( -21.95523322170430092, -8.895446802377390938, 66.77654591769551473 ) ) ;
#6443=ORIENTED_EDGE ( 'NONE', *, *, #12398, .F. ) ;
#6444=PLANE ( 'NONE',  #23571 ) ;
#6445=( BOUNDED_SURFACE ( )  B_SPLINE_SURFACE ( 3, 1, ( 
 ( #45830, #27099 ),
 ( #42125, #42372 ),
 ( #8643, #23666 ),
 ( #35206, #1476 ),
 ( #32262, #16236 ),
 ( #39875, #47022 ),
 ( #6149, #16491 ) ),
 .UNSPECIFIED., .T., .F., .F. ) 
 B_SPLINE_SURFACE_WITH_KNOTS ( ( 4, 3, 4 ),
 ( 2, 2 ),
 ( 0.000000000000000000, 0.5000000000000000000, 1.000000000000000000 ),
 ( 0.000000000000000000, 1.000000000000000000 ),
 .UNSPECIFIED. ) 
 GEOMETRIC_REPRESENTATION_ITEM ( )  RATIONAL_B_SPLINE_SURFACE ( (
 ( 1.000000000000000000, 1.000000000000000000),
 ( 0.3333333333333335369, 0.3333333333333330373),
 ( 0.3333333333333335369, 0.3333333333333330373),
 ( 1.000000000000000000, 1.000000000000000000),
 ( 0.3333333333333333703, 0.3333333333333333703),
 ( 0.3333333333333333703, 0.3333333333333333703),
 ( 1.000000000000000000, 1.000000000000000000) ) ) 
 REPRESENTATION_ITEM ( '' )  SURFACE ( )  );
#6446=ORIENTED_EDGE ( 'NONE', *, *, #18757, .F. ) ;
#6447=CARTESIAN_POINT ( 'NONE',  ( -24.08638337272136098, -17.13919944035470522, 66.09924551876292753 ) ) ;
#6449=CARTESIAN_POINT ( 'NONE',  ( -19.36999377412127288, -21.53330303623953057, 58.63393313907128856 ) ) ;
#6451=CARTESIAN_POINT ( 'NONE',  ( -24.47401588439613818, -14.84236418521736312, 59.54300237059217693 ) ) ;
#6455=CARTESIAN_POINT ( 'NONE',  ( -12.23220172533775241, -19.57856247689574403, 57.92682373937842044 ) ) ;
#6456=EDGE_LOOP ( 'NONE', ( #32457, #404 ) ) ;
#6457=FACE_OUTER_BOUND ( 'NONE', #48275, .T. ) ;
#6458=CARTESIAN_POINT ( 'NONE',  ( -11.87925614048969614, -19.08186516019194201, 71.75973838716171826 ) ) ;
#6461=EDGE_CURVE ( 'NONE', #29021, #22071, #877, .T. ) ;
#6462=CARTESIAN_POINT ( 'NONE',  ( -15.99552465959851233, -21.71601670177824417, 58.70074462513652236 ) ) ;
#6463=CARTESIAN_POINT ( 'NONE',  ( -11.85162103594838001, -10.49015045520576983, 71.25420998615621215 ) ) ;
#6465=VERTEX_POINT ( 'NONE', #34156 ) ;
#6467=CARTESIAN_POINT ( 'NONE',  ( -10.86613940586139471, -12.21176972022029972, 57.42037321672007266 ) ) ;
#6469=CARTESIAN_POINT ( 'NONE',  ( -23.47491605241627255, -11.19111043747921208, 73.36193326491972755 ) ) ;
#6470=LINE ( 'NONE', #31602, #47113 ) ;
#6471=CARTESIAN_POINT ( 'NONE',  ( -11.79792992861738909, -18.97409303405279957, 71.98685885147807539 ) ) ;
#6473=CARTESIAN_POINT ( 'NONE',  ( -22.22371030936713510, -9.111184089457765367, 59.90666523727240644 ) ) ;
#6474=CARTESIAN_POINT ( 'NONE',  ( -22.78678303852979425, -9.565966637465477262, 54.27966884056655061 ) ) ;
#6475=FACE_BOUND ( 'NONE', #9485, .T. ) ;
#6477=DIRECTION ( 'NONE',  ( 0.9375570856950864451, -0.3478314405900309603, 3.549360974553816870E-17 ) ) ;
#6478=B_SPLINE_CURVE_WITH_KNOTS ( 'NONE', 3,
 ( #45291, #45536, #11539, #22888, #11794, #41837, #8110, #38117, #4394, #43289 ),
 .UNSPECIFIED., .F., .F.,
 ( 4, 2, 2, 2, 4 ),
 ( 0.000000000000000000, 0.2500000000000000000, 0.5000000000000000000, 0.7500000000000000000, 1.000000000000000000 ),
 .UNSPECIFIED. ) ;
#6479=CARTESIAN_POINT ( 'NONE',  ( -20.69652669518947263, -8.116311108972663391, 63.35475588450814399 ) ) ;
#6482=VECTOR ( 'NONE', #27973, 1000.000000000000000 ) ;
#6485=CARTESIAN_POINT ( 'NONE',  ( -10.70366717127368084, -11.59369238842668359, 71.13214950009151494 ) ) ;
#6486=CARTESIAN_POINT ( 'NONE',  ( -13.54792730259346456, -8.920061342218058797, 57.25495614889487683 ) ) ;
#6488=ORIENTED_EDGE ( 'NONE', *, *, #38402, .T. ) ;
#6491=B_SPLINE_CURVE_WITH_KNOTS ( 'NONE', 3,
 ( #6343, #19305, #21375, #25967, #40986, #33565, #14847, #15844, #16318, #1309 ),
 .UNSPECIFIED., .F., .F.,
 ( 4, 2, 2, 2, 4 ),
 ( 0.6272669072877875562, 0.7522669073072943968, 0.8772669073268013484, 1.002266907346308189, 1.127266907365815030 ),
 .UNSPECIFIED. ) ;
#6492=EDGE_CURVE ( 'NONE', #23748, #15544, #32864, .T. ) ;
#6494=FACE_OUTER_BOUND ( 'NONE', #48057, .T. ) ;
#6495=CARTESIAN_POINT ( 'NONE',  ( -11.73157977884637226, -10.00306985186507269, 67.75542791425031908 ) ) ;
#6496=EDGE_CURVE ( 'NONE', #37312, #48665, #35483, .T. ) ;
#6498=CARTESIAN_POINT ( 'NONE',  ( -10.37714865501246564, -15.10143083228766159, 74.68290095780284332 ) ) ;
#6499=ORIENTED_EDGE ( 'NONE', *, *, #12701, .F. ) ;
#6500=B_SPLINE_CURVE_WITH_KNOTS ( 'NONE', 3,
 ( #35378, #27990, #12493, #23836, #38836, #43017, #23108, #38099, #4380, #36096 ),
 .UNSPECIFIED., .F., .F.,
 ( 4, 2, 2, 2, 4 ),
 ( 0.6272669072877699037, 0.7522669073072681956, 0.8772669073267664874, 1.002266907346264890, 1.127266907365763071 ),
 .UNSPECIFIED. ) ;
#6502=CARTESIAN_POINT ( 'NONE',  ( -20.66122932390920752, -21.07544863110783950, 62.52960166509647166 ) ) ;
#6504=LINE ( 'NONE', #18039, #40678 ) ;
#6505=B_SPLINE_CURVE_WITH_KNOTS ( 'NONE', 3,
 ( #11230, #25748, #18854, #44726, #26485, #37295, #22811, #33119, #21814, #10501 ),
 .UNSPECIFIED., .F., .F.,
 ( 4, 2, 2, 2, 4 ),
 ( 0.1272669073658691807, 0.2522669073463420508, 0.3772669073268148932, 0.5022669073072877355, 0.6272669072877605778 ),
 .UNSPECIFIED. ) ;
#6506=CARTESIAN_POINT ( 'NONE',  ( -23.27284462870851911, -18.74605969774991010, 66.10917289053097079 ) ) ;
#6507=ORIENTED_EDGE ( 'NONE', *, *, #39062, .T. ) ;
#6508=CARTESIAN_POINT ( 'NONE',  ( -13.57572078670752447, -20.65643022133334128, 61.81646323932617548 ) ) ;
#6510=ORIENTED_EDGE ( 'NONE', *, *, #46542, .T. ) ;
#6511=CARTESIAN_POINT ( 'NONE',  ( -11.91343869374197695, -19.82283377674160718, 58.04186948019505365 ) ) ;
#6512=EDGE_CURVE ( 'NONE', #24347, #44745, #29428, .T. ) ;
#6513=CARTESIAN_POINT ( 'NONE',  ( -23.32920267011340698, -18.57114636909328453, 72.95295412063659057 ) ) ;
#6514=CARTESIAN_POINT ( 'NONE',  ( -16.63459736671760325, -21.76466575500571921, 65.52564349350808470 ) ) ;
#6515=CARTESIAN_POINT ( 'NONE',  ( -24.69661721059186377, -13.19217688614222084, 59.53984779040520436 ) ) ;
#6516=ORIENTED_EDGE ( 'NONE', *, *, #17217, .F. ) ;
#6517=FACE_OUTER_BOUND ( 'NONE', #2193, .T. ) ;
#6518=CARTESIAN_POINT ( 'NONE',  ( -14.60689764421331560, -8.346551857622415582, 63.78978840692986552 ) ) ;
#6519=DIRECTION ( 'NONE',  ( 3.289814896819423347E-07, 7.277561374119425783E-07, -0.9999999999996811439 ) ) ;
#6520=CARTESIAN_POINT ( 'NONE',  ( -11.47140389976542529, -10.32934621678965037, 74.69531023250135604 ) ) ;
#6521=EDGE_CURVE ( 'NONE', #11451, #17592, #31021, .T. ) ;
#6522=CARTESIAN_POINT ( 'NONE',  ( -16.71379370341422543, -22.22534705626145879, 68.95206582789661809 ) ) ;
#6523=CARTESIAN_POINT ( 'NONE',  ( -24.24394117090890788, -12.99133827687660059, 59.51834745271546723 ) ) ;
#6524=ORIENTED_EDGE ( 'NONE', *, *, #28355, .T. ) ;
#6525=CARTESIAN_POINT ( 'NONE',  ( -24.32109429401129930, -17.62606226209447158, 66.05083068898602505 ) ) ;
#6526=( BOUNDED_CURVE ( )  B_SPLINE_CURVE ( 3, ( #1804, #20527, #5976, #24219 ),
 .UNSPECIFIED., .F., .F. ) 
 B_SPLINE_CURVE_WITH_KNOTS ( ( 4, 4 ),
 ( 0.4074455897393669535, 0.5000000000000000000 ),
 .UNSPECIFIED. ) 
 CURVE ( )  GEOMETRIC_REPRESENTATION_ITEM ( )  RATIONAL_B_SPLINE_CURVE ( ( 0.6983129098260987266, 0.7760317562606950936, 0.8765941196519931866, 0.9999999999999873435 ) ) 
 REPRESENTATION_ITEM ( '' )  );
#6527=CARTESIAN_POINT ( 'NONE',  ( -14.28913879486226435, -8.050816564744696535, 67.37479651646088996 ) ) ;
#6528=DIRECTION ( 'NONE',  ( -0.7847243476406476903, -0.6198448985189423110, 4.433022207822355740E-08 ) ) ;
#6532=EDGE_LOOP ( 'NONE', ( #17111, #8368, #27777, #35397, #20732 ) ) ;
#6535=CARTESIAN_POINT ( 'NONE',  ( -18.83586040784625126, -7.494106175837369044, 70.48572642001049360 ) ) ;
#6536=CARTESIAN_POINT ( 'NONE',  ( -23.72735656903896029, -11.76458228029187936, 59.70909150386957265 ) ) ;
#6537=CARTESIAN_POINT ( 'NONE',  ( -14.44809135640554487, -8.473323881223761234, 67.55975083863336295 ) ) ;
#6538=CARTESIAN_POINT ( 'NONE',  ( -12.83255559692156567, -9.459361206898796226, 74.31923029311820983 ) ) ;
#6539=ORIENTED_EDGE ( 'NONE', *, *, #12516, .T. ) ;
#6540=ORIENTED_EDGE ( 'NONE', *, *, #10979, .T. ) ;
#6544=LINE ( 'NONE', #33094, #8738 ) ;
#6546=ADVANCED_FACE ( 'NONE', ( #9543 ), #20953, .T. ) ;
#6548=ORIENTED_EDGE ( 'NONE', *, *, #873, .T. ) ;
#6549=CARTESIAN_POINT ( 'NONE',  ( -15.14815771252334820, -21.49015593068176244, 72.19008430323151515 ) ) ;
#6550=EDGE_CURVE ( 'NONE', #31760, #20698, #36340, .T. ) ;
#6551=CARTESIAN_POINT ( 'NONE',  ( -22.58065782673598321, -12.89613362149922438, 53.49899999999994549 ) ) ;
#6554=DIRECTION ( 'NONE',  ( 0.6621635203543605463, 0.7493593746073505812, 2.316976118889565779E-08 ) ) ;
#6556=B_SPLINE_CURVE_WITH_KNOTS ( 'NONE', 1,
 ( #33242, #25164 ),
 .UNSPECIFIED., .F., .F.,
 ( 2, 2 ),
 ( 0.000000000000000000, 1.000000000000000000 ),
 .UNSPECIFIED. ) ;
#6558=CARTESIAN_POINT ( 'NONE',  ( -18.26831188466123024, -21.75822359800944739, 68.81514735240074288 ) ) ;
#6559=CARTESIAN_POINT ( 'NONE',  ( -11.37040629063227115, -11.19590673242557166, 60.67885808612489029 ) ) ;
#6562=ORIENTED_EDGE ( 'NONE', *, *, #33024, .T. ) ;
#6563=CARTESIAN_POINT ( 'NONE',  ( -12.79645718024698553, -9.490555657722758554, 74.61922982865735321 ) ) ;
#6564=( BOUNDED_CURVE ( )  B_SPLINE_CURVE ( 3, ( #9706, #33038, #3264, #18268 ),
 .UNSPECIFIED., .F., .F. ) 
 B_SPLINE_CURVE_WITH_KNOTS ( ( 4, 4 ),
 ( 0.5000000000000000000, 0.9074455897393690629 ),
 .UNSPECIFIED. ) 
 CURVE ( )  GEOMETRIC_REPRESENTATION_ITEM ( )  RATIONAL_B_SPLINE_CURVE ( ( 1.000000000000022871, 0.4567392136813325232, 0.3561768502900143352, 0.6983129098260932865 ) ) 
 REPRESENTATION_ITEM ( '' )  );
#6565=CARTESIAN_POINT ( 'NONE',  ( -18.44528782684011858, -21.78515541812411982, 72.29983070759432451 ) ) ;
#6566=CYLINDRICAL_SURFACE ( 'NONE', #35480, 0.1500000000000002720 ) ;
#6567=EDGE_LOOP ( 'NONE', ( #25976, #8133 ) ) ;
#6568=DIRECTION ( 'NONE',  ( 0.5820088206811424580, -0.8131824719270213109, 7.019974882119936121E-08 ) ) ;
#6569=CARTESIAN_POINT ( 'NONE',  ( -21.41863048803933012, -8.999699081277377388, 73.61600897546567523 ) ) ;
#6570=CARTESIAN_POINT ( 'NONE',  ( -15.03263910315855512, -8.176888424288378587, 56.86472059657746314 ) ) ;
#6572=CARTESIAN_POINT ( 'NONE',  ( -13.47696527960146895, -8.967565513329615712, 60.44510101887779996 ) ) ;
#6573=EDGE_LOOP ( 'NONE', ( #2111, #48700, #24313, #16481, #3614 ) ) ;
#6574=CARTESIAN_POINT ( 'NONE',  ( -10.72530867274958233, -17.00760959713300480, 57.97288447305808745 ) ) ;
#6575=CARTESIAN_POINT ( 'NONE',  ( -24.65228577264951326, -13.00463492950681754, 62.93925847568694820 ) ) ;
#6577=CARTESIAN_POINT ( 'NONE',  ( -14.97188219925329378, -8.199429090594037461, 56.84999999999994458 ) ) ;
#6579=DIRECTION ( 'NONE',  ( -5.224165706511165539E-06, 4.853367013834837651E-07, 0.9999999999862362321 ) ) ;
#6581=CARTESIAN_POINT ( 'NONE',  ( -15.43182990062313742, -8.046249867383863830, 74.36513541778452918 ) ) ;
#6582=ORIENTED_EDGE ( 'NONE', *, *, #24625, .T. ) ;
#6584=( BOUNDED_CURVE ( )  B_SPLINE_CURVE ( 3, ( #1055, #12373, #98, #31092 ),
 .UNSPECIFIED., .F., .F. ) 
 B_SPLINE_CURVE_WITH_KNOTS ( ( 4, 4 ),
 ( 0.5000000000000000000, 0.9074455897393682857 ),
 .UNSPECIFIED. ) 
 CURVE ( )  GEOMETRIC_REPRESENTATION_ITEM ( )  RATIONAL_B_SPLINE_CURVE ( ( 1.000000000000003331, 0.4567392136813345216, 0.3561768502900287681, 0.6983129098260898449 ) ) 
 REPRESENTATION_ITEM ( '' )  );
#6585=CARTESIAN_POINT ( 'NONE',  ( -24.66692207690629246, -13.06418342283853562, 63.08910124536953390 ) ) ;
#6586=ORIENTED_EDGE ( 'NONE', *, *, #23398, .T. ) ;
#6588=CARTESIAN_POINT ( 'NONE',  ( -15.15660932275500095, -21.48492473237050859, 65.39124617759186719 ) ) ;
#6590=LINE ( 'NONE', #28753, #31365 ) ;
#6591=CARTESIAN_POINT ( 'NONE',  ( -23.46013293835336100, -11.16077341686890989, 69.77721965307074470 ) ) ;
#6592=EDGE_CURVE ( 'NONE', #8287, #1510, #7304, .T. ) ;
#6595=CARTESIAN_POINT ( 'NONE',  ( -17.86169286162045111, -7.371900692872102034, 60.22027394188889815 ) ) ;
#6596=ORIENTED_EDGE ( 'NONE', *, *, #48055, .T. ) ;
#6597=VERTEX_POINT ( 'NONE', #33121 ) ;
#6598=EDGE_CURVE ( 'NONE', #15615, #12505, #15492, .T. ) ;
#6601=CARTESIAN_POINT ( 'NONE',  ( -21.92638982964590255, -9.447133096874894775, 63.38080841974745283 ) ) ;
#6603=CARTESIAN_POINT ( 'NONE',  ( -24.40624982674571086, -15.81067781142186313, 73.09483948631277883 ) ) ;
#6607=CARTESIAN_POINT ( 'NONE',  ( -22.02980920716174396, -20.08072702813828414, 62.23439177585281357 ) ) ;
#6608=EDGE_CURVE ( 'NONE', #4181, #20377, #39503, .T. ) ;
#6610=CARTESIAN_POINT ( 'NONE',  ( -10.46291082975850806, -15.97406517396614944, 61.19356052171543325 ) ) ;
#6611=EDGE_CURVE ( 'NONE', #8331, #38907, #48160, .T. ) ;
#6614=CARTESIAN_POINT ( 'NONE',  ( -13.59269417415731063, -21.19935819725622039, 65.09973481642835225 ) ) ;
#6615=CARTESIAN_POINT ( 'NONE',  ( -22.37667958203292784, -9.786583861647388360, 73.48161084599418302 ) ) ;
#6616=CARTESIAN_POINT ( 'NONE',  ( -17.33262245845742910, -7.759502110702281463, 67.30567542699309058 ) ) ;
#6617=EDGE_CURVE ( 'NONE', #43505, #25227, #44536, .T. ) ;
#6618=CARTESIAN_POINT ( 'NONE',  ( -16.26184114368905043, -7.855670183028919062, 60.20028478909662795 ) ) ;
#6619=ORIENTED_EDGE ( 'NONE', *, *, #34698, .T. ) ;
#6620=DIRECTION ( 'NONE',  ( -0.2737502900231350011, -0.9618007999124593699, 5.400150802763565900E-08 ) ) ;
#6621=ORIENTED_EDGE ( 'NONE', *, *, #45360, .T. ) ;
#6623=( BOUNDED_CURVE ( )  B_SPLINE_CURVE ( 3, ( #5230, #39197, #39923, #21220 ),
 .UNSPECIFIED., .F., .F. ) 
 B_SPLINE_CURVE_WITH_KNOTS ( ( 4, 4 ),
 ( 0.9074455897393651771, 1.000000000000000000 ),
 .UNSPECIFIED. ) 
 CURVE ( )  GEOMETRIC_REPRESENTATION_ITEM ( )  RATIONAL_B_SPLINE_CURVE ( ( 0.6983129098261127155, 0.7760317562607151887, 0.8765941196520109502, 1.000000000000000000 ) ) 
 REPRESENTATION_ITEM ( '' )  );
#6625=CARTESIAN_POINT ( 'NONE',  ( -17.64564815875613846, -7.362378996003227094, 63.72869765717685198 ) ) ;
#6627=CARTESIAN_POINT ( 'NONE',  ( -20.43185948505062299, -8.432683554863363184, 66.79576150497511833 ) ) ;
#6629=CARTESIAN_POINT ( 'NONE',  ( -12.84615363328625826, -20.17103110633857455, 72.09181604382622766 ) ) ;
#6631=CARTESIAN_POINT ( 'NONE',  ( -18.86498748457869468, -7.957467553504502078, 70.48141235020942474 ) ) ;
#6632=B_SPLINE_CURVE_WITH_KNOTS ( 'NONE', 3,
 ( #47752, #13990, #6154, #32497, #36894, #40367, #17218, #33196, #10575, #47522 ),
 .UNSPECIFIED., .F., .F.,
 ( 4, 2, 2, 2, 4 ),
 ( 0.000000000000000000, 0.2500000000000000000, 0.5000000000000000000, 0.7500000000000000000, 1.000000000000000000 ),
 .UNSPECIFIED. ) ;
#6635=VERTEX_POINT ( 'NONE', #29450 ) ;
#6637=FACE_OUTER_BOUND ( 'NONE', #6807, .T. ) ;
#6638=CARTESIAN_POINT ( 'NONE',  ( -23.00454255336054743, -10.50046069577333263, 59.88731295783226471 ) ) ;
#6640=ORIENTED_EDGE ( 'NONE', *, *, #11617, .F. ) ;
#6641=CARTESIAN_POINT ( 'NONE',  ( -11.84809292083425802, -10.57729547379942225, 71.19566414032826174 ) ) ;
#6642=ORIENTED_EDGE ( 'NONE', *, *, #36773, .T. ) ;
#6645=CARTESIAN_POINT ( 'NONE',  ( -10.60570718526854961, -17.81143598018131158, 71.68222757358374508 ) ) ;
#6647=CARTESIAN_POINT ( 'NONE',  ( -12.90353999865511625, -8.887351178413068098, 67.49447498869417927 ) ) ;
#6648=CARTESIAN_POINT ( 'NONE',  ( -23.67325187062781566, -18.86515452381667757, 69.39397745686399332 ) ) ;
#6649=DIRECTION ( 'NONE',  ( -0.9584484254710482487, -0.2852658684667118139, 3.516456354099036852E-08 ) ) ;
#6650=VERTEX_POINT ( 'NONE', #395 ) ;
#6651=CARTESIAN_POINT ( 'NONE',  ( -11.79630000206883977, -19.05592701419838519, 71.97213747039440079 ) ) ;
#6652=CARTESIAN_POINT ( 'NONE',  ( -12.41315160057549960, -9.850077812919039388, 57.23935532239169532 ) ) ;
#6654=ORIENTED_EDGE ( 'NONE', *, *, #3524, .T. ) ;
#6656=VERTEX_POINT ( 'NONE', #14885 ) ;
#6658=AXIS2_PLACEMENT_3D ( 'NONE', #1853, #5071, #13398 ) ;
#6659=CARTESIAN_POINT ( 'NONE',  ( -23.64032756017451220, -11.59062047747720925, 63.17891664429986776 ) ) ;
#6660=EDGE_CURVE ( 'NONE', #1656, #23182, #17248, .T. ) ;
#6662=FACE_OUTER_BOUND ( 'NONE', #9758, .T. ) ;
#6663=ORIENTED_EDGE ( 'NONE', *, *, #8009, .F. ) ;
#6665=ADVANCED_FACE ( 'NONE', ( #18592 ), #44728, .T. ) ;
#6666=CARTESIAN_POINT ( 'NONE',  ( -23.82052202658861972, -17.65274426584190692, 59.19481648357778170 ) ) ;
#6667=ORIENTED_EDGE ( 'NONE', *, *, #34772, .T. ) ;
#6668=LINE ( 'NONE', #3451, #28418 ) ;
#6669=ADVANCED_FACE ( 'NONE', ( #11713 ), #26243, .T. ) ;
#6670=CARTESIAN_POINT ( 'NONE',  ( -19.69296339593938328, -21.90548865816194635, 65.62632728502332213 ) ) ;
#6671=CARTESIAN_POINT ( 'NONE',  ( -23.20936678059565494, -18.85217346302747643, 59.03977614772677640 ) ) ;
#6672=VERTEX_POINT ( 'NONE', #33863 ) ;
#6673=DIRECTION ( 'NONE',  ( -5.731567514496413899E-31, -1.020425574103664789E-16, -1.000000000000000000 ) ) ;
#6674=EDGE_LOOP ( 'NONE', ( #6177, #24953 ) ) ;
#6676=B_SPLINE_CURVE_WITH_KNOTS ( 'NONE', 3,
 ( #31802, #38449, #23937, #5219, #12597, #27623, #19761, #1040, #42659, #35238 ),
 .UNSPECIFIED., .F., .F.,
 ( 4, 2, 2, 2, 4 ),
 ( 0.000000000000000000, 0.2500000000000000000, 0.5000000000000000000, 0.7500000000000000000, 1.000000000000000000 ),
 .UNSPECIFIED. ) ;
#6677=CARTESIAN_POINT ( 'NONE',  ( -24.39889739404874192, -14.21436921164216116, 69.65275261046649291 ) ) ;
#6679=CARTESIAN_POINT ( 'NONE',  ( -10.59656512619885227, -13.05092609425065397, 68.02360230423870746 ) ) ;
#6680=CARTESIAN_POINT ( 'NONE',  ( -23.99887651489391871, -12.24265264118830387, 73.39792675737896843 ) ) ;
#6682=ADVANCED_FACE ( 'NONE', ( #26006 ), #41022, .T. ) ;
#6683=CARTESIAN_POINT ( 'NONE',  ( -10.04932599622759248, -15.86565813568266492, 64.61497449378698832 ) ) ;
#6685=CARTESIAN_POINT ( 'NONE',  ( -12.38489527708928684, -19.74478370405832806, 58.13502342243108245 ) ) ;
#6686=VERTEX_POINT ( 'NONE', #164 ) ;
#6687=DIRECTION ( 'NONE',  ( -9.444166282346144476E-07, 1.975884201625194781E-06, 0.9999999999976019183 ) ) ;
#6688=EDGE_CURVE ( 'NONE', #38712, #28574, #14261, .T. ) ;
#6689=CARTESIAN_POINT ( 'NONE',  ( -10.39679176622870038, -14.24023819782134304, 64.40275955115841100 ) ) ;
#6690=CARTESIAN_POINT ( 'NONE',  ( -22.63560516303400050, -20.13310814558360917, 69.28922553891734992 ) ) ;
#6692=CARTESIAN_POINT ( 'NONE',  ( -13.29845860553889203, -21.01266621750898267, 61.63151044148704472 ) ) ;
#6693=CARTESIAN_POINT ( 'NONE',  ( -18.57019874455824393, -7.903669367688619829, 70.47953930074716311 ) ) ;
#6694=EDGE_CURVE ( 'NONE', #19021, #6412, #36595, .T. ) ;
#6695=CARTESIAN_POINT ( 'NONE',  ( -24.25486363958986757, -13.06355980472538469, 63.11792038370487035 ) ) ;
#6696=AXIS2_PLACEMENT_3D ( 'NONE', #41097, #15897, #7380 ) ;
#6697=VERTEX_POINT ( 'NONE', #23051 ) ;
#6698=VERTEX_POINT ( 'NONE', #12433 ) ;
#6702=CARTESIAN_POINT ( 'NONE',  ( -10.37818533259200748, -17.22973363664382873, 61.27247698181179913 ) ) ;
#6703=DIRECTION ( 'NONE',  ( 0.8705373987491421550, -0.4921022631314296292, 4.758021987246392057E-08 ) ) ;
#6704=CARTESIAN_POINT ( 'NONE',  ( -24.17271849214968071, -12.95015691860989371, 66.60246741689840633 ) ) ;
#6705=CARTESIAN_POINT ( 'NONE',  ( -12.10131192688100477, -10.18592936015514638, 64.31442259820508411 ) ) ;
#6706=CARTESIAN_POINT ( 'NONE',  ( -12.10599122619147749, -20.02663529450013513, 61.58173959111590534 ) ) ;
#6707=( BOUNDED_CURVE ( )  B_SPLINE_CURVE ( 3, ( #3665, #239, #33679, #26821 ),
 .UNSPECIFIED., .F., .F. ) 
 B_SPLINE_CURVE_WITH_KNOTS ( ( 4, 4 ),
 ( 0.5000000000000000000, 0.9074455897393706172 ),
 .UNSPECIFIED. ) 
 CURVE ( )  GEOMETRIC_REPRESENTATION_ITEM ( )  RATIONAL_B_SPLINE_CURVE ( ( 1.000000000000017986, 0.4567392136813281378, 0.3561768502900162781, 0.6983129098261018353 ) ) 
 REPRESENTATION_ITEM ( '' )  );
#6708=B_SPLINE_CURVE_WITH_KNOTS ( 'NONE', 3,
 ( #3464, #48043, #44601, #48521, #2081, #17082, #14756, #25629, #6019, #9731 ),
 .UNSPECIFIED., .F., .F.,
 ( 4, 2, 2, 2, 4 ),
 ( 0.000000000000000000, 0.2500000000000000000, 0.5000000000000000000, 0.7500000000000000000, 1.000000000000000000 ),
 .UNSPECIFIED. ) ;
#6709=CARTESIAN_POINT ( 'NONE',  ( -23.86426264037124056, -17.55550176324236489, 66.17187017368655688 ) ) ;
#6710=CARTESIAN_POINT ( 'NONE',  ( -11.46205946457914315, -19.27670325764784920, 71.86402743521411196 ) ) ;
#6711=CARTESIAN_POINT ( 'NONE',  ( -20.82184643845504723, -8.178298495136663959, 63.49776821231386492 ) ) ;
#6713=CARTESIAN_POINT ( 'NONE',  ( -16.32575768948312600, -7.844986739114469643, 60.21500614002425777 ) ) ;
#6714=CARTESIAN_POINT ( 'NONE',  ( -10.69992066440855361, -12.66433694503948004, 67.88265386532016521 ) ) ;
#6715=CARTESIAN_POINT ( 'NONE',  ( -23.96075645138428101, -17.45014240273063066, 65.94357239682317129 ) ) ;
#6716=CARTESIAN_POINT ( 'NONE',  ( -22.53375553849141610, -19.66661599265353644, 72.94400550747238299 ) ) ;
#6717=CARTESIAN_POINT ( 'NONE',  ( -10.70297003644833644, -11.59513240183115279, 71.27356180636090244 ) ) ;
#6718=( BOUNDED_SURFACE ( )  B_SPLINE_SURFACE ( 3, 1, ( 
 ( #19583, #33602 ),
 ( #23049, #14882 ),
 ( #11229, #162 ),
 ( #33861, #38270 ),
 ( #7790, #34103 ),
 ( #41996, #22547 ),
 ( #30197, #29946 ) ),
 .UNSPECIFIED., .T., .F., .F. ) 
 B_SPLINE_SURFACE_WITH_KNOTS ( ( 4, 3, 4 ),
 ( 2, 2 ),
 ( 0.000000000000000000, 0.5000000000000000000, 1.000000000000000000 ),
 ( 0.000000000000000000, 1.000000000000000000 ),
 .UNSPECIFIED. ) 
 GEOMETRIC_REPRESENTATION_ITEM ( )  RATIONAL_B_SPLINE_SURFACE ( (
 ( 1.000000000000000000, 1.000000000000000000),
 ( 0.3333333333333335369, 0.3333333333333330373),
 ( 0.3333333333333335369, 0.3333333333333330373),
 ( 1.000000000000000000, 1.000000000000000000),
 ( 0.3333333333333333703, 0.3333333333333333703),
 ( 0.3333333333333333703, 0.3333333333333333703),
 ( 1.000000000000000000, 1.000000000000000000) ) ) 
 REPRESENTATION_ITEM ( '' )  SURFACE ( )  );
#6719=CARTESIAN_POINT ( 'NONE',  ( -16.44450502417200255, -21.74194820930941319, 65.33637549174824244 ) ) ;
#6720=( BOUNDED_CURVE ( )  B_SPLINE_CURVE ( 3, ( #28601, #43628, #9888, #15491 ),
 .UNSPECIFIED., .F., .F. ) 
 B_SPLINE_CURVE_WITH_KNOTS ( ( 4, 4 ),
 ( 0.5000000000000000000, 0.9074455897393645110 ),
 .UNSPECIFIED. ) 
 CURVE ( )  GEOMETRIC_REPRESENTATION_ITEM ( )  RATIONAL_B_SPLINE_CURVE ( ( 1.000000000000031308, 0.4567392136813358539, 0.3561768502900097833, 0.6983129098260869583 ) ) 
 REPRESENTATION_ITEM ( '' )  );
#6721=EDGE_LOOP ( 'NONE', ( #9698, #10674, #36944, #26915, #2651 ) ) ;
#6726=CARTESIAN_POINT ( 'NONE',  ( -23.99919889754976410, -17.21122886273513330, 69.71339796235052688 ) ) ;
#6727=B_SPLINE_CURVE_WITH_KNOTS ( 'NONE', 3,
 ( #41654, #34976, #26640, #15522, #1494, #16250, #531, #31058, #42641, #16507 ),
 .UNSPECIFIED., .F., .F.,
 ( 4, 2, 2, 2, 4 ),
 ( 0.6272669072782977029, 0.7522669073001729823, 0.8772669073220482616, 1.002266907343923652, 1.127266907365798820 ),
 .UNSPECIFIED. ) ;
#6728=( BOUNDED_SURFACE ( )  B_SPLINE_SURFACE ( 3, 1, ( 
 ( #35661, #31746 ),
 ( #35180, #43063 ),
 ( #42604, #27317 ),
 ( #1941, #23882 ),
 ( #34705, #38642 ),
 ( #15977, #16941 ),
 ( #31983, #46998 ) ),
 .UNSPECIFIED., .T., .F., .F. ) 
 B_SPLINE_SURFACE_WITH_KNOTS ( ( 4, 3, 4 ),
 ( 2, 2 ),
 ( 0.000000000000000000, 0.5000000000000000000, 1.000000000000000000 ),
 ( 0.000000000000000000, 1.000000000000000000 ),
 .UNSPECIFIED. ) 
 GEOMETRIC_REPRESENTATION_ITEM ( )  RATIONAL_B_SPLINE_SURFACE ( (
 ( 1.000000000000000000, 1.000000000000000000),
 ( 0.3333333333333335369, 0.3333333333333330373),
 ( 0.3333333333333335369, 0.3333333333333330373),
 ( 1.000000000000000000, 1.000000000000000000),
 ( 0.3333333333333333703, 0.3333333333333333703),
 ( 0.3333333333333333703, 0.3333333333333333703),
 ( 1.000000000000000000, 1.000000000000000000) ) ) 
 REPRESENTATION_ITEM ( '' )  SURFACE ( )  );
#6730=EDGE_CURVE ( 'NONE', #43248, #1779, #42490, .T. ) ;
#6731=CARTESIAN_POINT ( 'NONE',  ( -10.51729497052147977, -16.22293520194095606, 71.74750383215044280 ) ) ;
#6732=CARTESIAN_POINT ( 'NONE',  ( -20.84119746710919330, -20.97572115929791892, 62.11471400470772863 ) ) ;
#6733=ORIENTED_EDGE ( 'NONE', *, *, #14764, .F. ) ;
#6735=CARTESIAN_POINT ( 'NONE',  ( -13.53325528467554406, -21.16256411608339150, 65.17124155742401115 ) ) ;
#6736=CARTESIAN_POINT ( 'NONE',  ( -21.06634951290973845, -21.30826427787840771, 62.29966696806321380 ) ) ;
#6737=ORIENTED_EDGE ( 'NONE', *, *, #44845, .T. ) ;
#6738=CARTESIAN_POINT ( 'NONE',  ( -17.91451193640577344, -22.24313339626381847, 61.99040498927033127 ) ) ;
#6739=B_SPLINE_CURVE_WITH_KNOTS ( 'NONE', 3,
 ( #11468, #18597, #41262, #44988, #7802, #11235, #33609, #40526, #36567, #25754 ),
 .UNSPECIFIED., .F., .F.,
 ( 4, 2, 2, 2, 4 ),
 ( 0.1272669073658314609, 0.2522669073463261746, 0.3772669073268208884, 0.5022669073073156021, 0.6272669072878103158 ),
 .UNSPECIFIED. ) ;
#6740=CARTESIAN_POINT ( 'NONE',  ( -14.90981263331598150, -21.39562362703504306, 61.93600440604521395 ) ) ;
#6742=CARTESIAN_POINT ( 'NONE',  ( -23.46741908093438767, -19.16603997859080266, 62.53902161361033052 ) ) ;
#6743=CARTESIAN_POINT ( 'NONE',  ( -10.05862351292959467, -15.92886012141397245, 64.69266982328383619 ) ) ;
#6744=B_SPLINE_CURVE_WITH_KNOTS ( 'NONE', 3,
 ( #14441, #40572, #11284, #6852, #44532, #7601, #40823, #37112, #3395, #37602 ),
 .UNSPECIFIED., .F., .F.,
 ( 4, 2, 2, 2, 4 ),
 ( 0.000000000000000000, 0.2500000000000000000, 0.5000000000000000000, 0.7500000000000000000, 1.000000000000000000 ),
 .UNSPECIFIED. ) ;
#6745=CARTESIAN_POINT ( 'NONE',  ( -22.84116833803633284, -10.28479860924217704, 59.75770304231562591 ) ) ;
#6746=EDGE_LOOP ( 'NONE', ( #19195, #1390, #29201, #47397, #16087 ) ) ;
#6748=CARTESIAN_POINT ( 'NONE',  ( -24.41897112398753933, -17.37347453850100720, 69.59835118672229726 ) ) ;
#6749=CARTESIAN_POINT ( 'NONE',  ( -15.07489227400421861, -21.40335501537338203, 65.10596683994182854 ) ) ;
#6750=CARTESIAN_POINT ( 'NONE',  ( -22.22619359738691003, -20.50513629785891823, 58.94938195453792673 ) ) ;
#6754=EDGE_CURVE ( 'NONE', #17630, #4066, #1597, .T. ) ;
#6755=CARTESIAN_POINT ( 'NONE',  ( -18.06825732353542335, -21.77950449724592730, 62.06639155695750532 ) ) ;
#6756=EDGE_CURVE ( 'NONE', #14865, #33892, #46414, .T. ) ;
#6757=EDGE_CURVE ( 'NONE', #43621, #44791, #10209, .T. ) ;
#6760=CARTESIAN_POINT ( 'NONE',  ( -16.05890242020153380, -7.889590739215661230, 60.08539615417584656 ) ) ;
#6761=CARTESIAN_POINT ( 'NONE',  ( -24.72811879990099726, -13.33785195616451169, 59.54923321989076612 ) ) ;
#6762=VERTEX_POINT ( 'NONE', #8503 ) ;
#6763=CARTESIAN_POINT ( 'NONE',  ( -24.34502428176253019, -17.56683243011407924, 66.12852677468319484 ) ) ;
#6765=CARTESIAN_POINT ( 'NONE',  ( -22.20320178312271153, -19.92390373660361291, 65.70421731406698029 ) ) ;
#6766=VERTEX_POINT ( 'NONE', #41998 ) ;
#6770=ORIENTED_EDGE ( 'NONE', *, *, #22503, .F. ) ;
#6771=VERTEX_POINT ( 'NONE', #30684 ) ;
#6772=CARTESIAN_POINT ( 'NONE',  ( -23.15350085761965460, -9.941038866939328145, 54.02312124697527196 ) ) ;
#6773=CARTESIAN_POINT ( 'NONE',  ( -23.74619265052512773, -11.68934008440960248, 62.95218278636777143 ) ) ;
#6774=FACE_OUTER_BOUND ( 'NONE', #18468, .T. ) ;
#6775=VERTEX_POINT ( 'NONE', #27701 ) ;
#6776=ORIENTED_EDGE ( 'NONE', *, *, #7123, .F. ) ;
#6778=B_SPLINE_CURVE_WITH_KNOTS ( 'NONE', 3,
 ( #20404, #38621, #5385, #35406, #8846, #23623, #20150, #23862, #24340, #34683 ),
 .UNSPECIFIED., .F., .F.,
 ( 4, 2, 2, 2, 4 ),
 ( 0.000000000000000000, 0.2500000000000000000, 0.5000000000000000000, 0.7500000000000000000, 1.000000000000000000 ),
 .UNSPECIFIED. ) ;
#6779=EDGE_CURVE ( 'NONE', #784, #46311, #39591, .T. ) ;
#6780=CARTESIAN_POINT ( 'NONE',  ( -22.34470957656571599, -19.78791530553215949, 69.47417989488683077 ) ) ;
#6781=DIRECTION ( 'NONE',  ( 0.6264825908887947659, -0.7794354131762691873, 3.858680029754496192E-08 ) ) ;
#6784=CARTESIAN_POINT ( 'NONE',  ( -24.35706380436459995, -15.77560588608014136, 69.83307488757523629 ) ) ;
#6786=CARTESIAN_POINT ( 'NONE',  ( -20.66696855643225916, -21.06909979829503854, 58.94475164909854925 ) ) ;
#6787=CARTESIAN_POINT ( 'NONE',  ( -21.36489355414517632, -8.963473290115421932, 73.90128753234840531 ) ) ;
#6788=EDGE_LOOP ( 'NONE', ( #10456, #40530, #1033, #17296, #12189 ) ) ;
#6789=CARTESIAN_POINT ( 'NONE',  ( -11.24765530704275385, -11.51409840800856621, 67.90248063513186594 ) ) ;
#6791=ORIENTED_EDGE ( 'NONE', *, *, #42576, .F. ) ;
#6792=CARTESIAN_POINT ( 'NONE',  ( -22.44463050228041467, -9.931189664211119705, 73.49663562641346459 ) ) ;
#6793=CARTESIAN_POINT ( 'NONE',  ( -10.11671990330600579, -16.26064306581185903, 71.57033522450831242 ) ) ;
#6794=CARTESIAN_POINT ( 'NONE',  ( -21.55974298755023000, -21.00590022698144921, 72.72457636846944240 ) ) ;
#6796=FACE_OUTER_BOUND ( 'NONE', #15142, .T. ) ;
#6797=CARTESIAN_POINT ( 'NONE',  ( -24.18217652367932047, -11.67366674157813122, 59.67509901561481911 ) ) ;
#6798=( BOUNDED_CURVE ( )  B_SPLINE_CURVE ( 3, ( #36683, #14280, #29568, #24915 ),
 .UNSPECIFIED., .F., .F. ) 
 B_SPLINE_CURVE_WITH_KNOTS ( ( 4, 4 ),
 ( 0.4074455897393635673, 0.5000000000000000000 ),
 .UNSPECIFIED. ) 
 CURVE ( )  GEOMETRIC_REPRESENTATION_ITEM ( )  RATIONAL_B_SPLINE_CURVE ( ( 0.6983129098260953960, 0.7760317562607027542, 0.8765941196520051770, 1.000000000000004219 ) ) 
 REPRESENTATION_ITEM ( '' )  );
#6799=CARTESIAN_POINT ( 'NONE',  ( -13.17078218117215549, -9.186392337449538203, 67.39414915108072535 ) ) ;
#6800=CARTESIAN_POINT ( 'NONE',  ( -24.30537484439201990, -16.09989820848641173, 66.13495298149886992 ) ) ;
#6801=ORIENTED_EDGE ( 'NONE', *, *, #30149, .F. ) ;
#6802=CARTESIAN_POINT ( 'NONE',  ( -24.83421645677935174, -15.58062944684732365, 73.16337087059751809 ) ) ;
#6805=VERTEX_POINT ( 'NONE', #26975 ) ;
#6806=CARTESIAN_POINT ( 'NONE',  ( -15.14522032754860703, -21.97383469840033854, 53.76227901944321275 ) ) ;
#6807=EDGE_LOOP ( 'NONE', ( #35182, #11770 ) ) ;
#6808=ADVANCED_FACE ( 'NONE', ( #19585 ), #5855, .T. ) ;
#6809=EDGE_CURVE ( 'NONE', #17056, #44664, #10882, .T. ) ;
#6810=CARTESIAN_POINT ( 'NONE',  ( -13.93897074462874919, -20.93787812888889377, 68.74153005185598886 ) ) ;
#6812=CARTESIAN_POINT ( 'NONE',  ( -22.65633733904555669, -10.15891943096868744, 70.01178531762562329 ) ) ;
#6813=ORIENTED_EDGE ( 'NONE', *, *, #34483, .T. ) ;
#6814=CARTESIAN_POINT ( 'NONE',  ( -10.45863951484398946, -14.11462368554138536, 60.91821294131582931 ) ) ;
#6815=ORIENTED_EDGE ( 'NONE', *, *, #42546, .F. ) ;
#6818=CARTESIAN_POINT ( 'NONE',  ( -11.20499100338089349, -18.91108562151346462, 64.84683437277969631 ) ) ;
#6821=LINE ( 'NONE', #24587, #25142 ) ;
#6824=EDGE_CURVE ( 'NONE', #4227, #29981, #17485, .T. ) ;
#6827=CARTESIAN_POINT ( 'NONE',  ( -23.47587192523704047, -19.15443292186558111, 62.51440210027411837 ) ) ;
#6828=CARTESIAN_POINT ( 'NONE',  ( -12.31054147697317802, -19.59141247267844932, 61.46848823829365216 ) ) ;
#6830=CARTESIAN_POINT ( 'NONE',  ( -17.77594298899184366, -7.367433885636743618, 60.26556189360973548 ) ) ;
#6831=VECTOR ( 'NONE', #16278, 1000.000000000000114 ) ;
#6832=AXIS2_PLACEMENT_3D ( 'NONE', #11954, #38521, #23277 ) ;
#6833=ORIENTED_EDGE ( 'NONE', *, *, #33578, .T. ) ;
#6834=ORIENTED_EDGE ( 'NONE', *, *, #7030, .F. ) ;
#6835=PLANE ( 'NONE',  #24970 ) ;
#6836=ADVANCED_FACE ( 'NONE', ( #27937 ), #43705, .T. ) ;
#6838=CARTESIAN_POINT ( 'NONE',  ( -23.65624057141236847, -11.51332318074561911, 66.72214514605295221 ) ) ;
#6839=DIRECTION ( 'NONE',  ( 1.295331059719046080E-06, -6.890485863767693062E-07, -0.9999999999989236388 ) ) ;
#6843=ORIENTED_EDGE ( 'NONE', *, *, #48198, .T. ) ;
#6844=CYLINDRICAL_SURFACE ( 'NONE', #9162, 0.1499999999999977185 ) ;
#6845=DIRECTION ( 'NONE',  ( -0.5420872618288283817, -0.8403222004463036798, 7.592316861452270591E-08 ) ) ;
#6846=FACE_OUTER_BOUND ( 'NONE', #34814, .T. ) ;
#6848=B_SPLINE_CURVE_WITH_KNOTS ( 'NONE', 3,
 ( #39132, #3342, #46774, #14629, #9355, #10729, #36807, #39382, #44725, #20677 ),
 .UNSPECIFIED., .F., .F.,
 ( 4, 2, 2, 2, 4 ),
 ( 0.000000000000000000, 0.2500000000000000000, 0.5000000000000000000, 0.7500000000000000000, 1.000000000000000000 ),
 .UNSPECIFIED. ) ;
#6849=( BOUNDED_CURVE ( )  B_SPLINE_CURVE ( 3, ( #4769, #12387, #19295, #16557 ),
 .UNSPECIFIED., .F., .F. ) 
 B_SPLINE_CURVE_WITH_KNOTS ( ( 4, 4 ),
 ( 0.4074455897393655657, 0.5000000000000000000 ),
 .UNSPECIFIED. ) 
 CURVE ( )  GEOMETRIC_REPRESENTATION_ITEM ( )  RATIONAL_B_SPLINE_CURVE ( ( 0.6983129098260966172, 0.7760317562606876551, 0.8765941196519846379, 0.9999999999999783507 ) ) 
 REPRESENTATION_ITEM ( '' )  );
#6850=ORIENTED_EDGE ( 'NONE', *, *, #43579, .T. ) ;
#6851=CARTESIAN_POINT ( 'NONE',  ( -11.56806251476610115, -18.73522173559940995, 65.03234934376791898 ) ) ;
#6852=CARTESIAN_POINT ( 'NONE',  ( -21.54646308099719931, -9.151741662630445973, 66.73437983189968747 ) ) ;
#6853=ORIENTED_EDGE ( 'NONE', *, *, #41449, .T. ) ;
#6854=CARTESIAN_POINT ( 'NONE',  ( -15.23980195177804831, -21.45974831136452110, 65.17884789245921695 ) ) ;
#6856=CARTESIAN_POINT ( 'NONE',  ( -6.795509042373261366, -13.90955010341581044, 54.49999999999995026 ) ) ;
#6858=CARTESIAN_POINT ( 'NONE',  ( -17.92193066645248578, -21.84160715981037981, 62.02535923543162966 ) ) ;
#6859=( BOUNDED_SURFACE ( )  B_SPLINE_SURFACE ( 3, 1, ( 
 ( #16155, #19880 ),
 ( #1150, #16403 ),
 ( #4610, #11766 ),
 ( #41808, #27741 ),
 ( #8089, #1388 ),
 ( #34153, #38088 ),
 ( #4369, #45759 ) ),
 .UNSPECIFIED., .T., .F., .F. ) 
 B_SPLINE_SURFACE_WITH_KNOTS ( ( 4, 3, 4 ),
 ( 2, 2 ),
 ( 0.000000000000000000, 0.5000000000000000000, 1.000000000000000000 ),
 ( 0.000000000000000000, 1.000000000000000000 ),
 .UNSPECIFIED. ) 
 GEOMETRIC_REPRESENTATION_ITEM ( )  RATIONAL_B_SPLINE_SURFACE ( (
 ( 1.000000000000000000, 1.000000000000000000),
 ( 0.3333333333333335369, 0.3333333333333330373),
 ( 0.3333333333333335369, 0.3333333333333330373),
 ( 1.000000000000000000, 1.000000000000000000),
 ( 0.3333333333333333703, 0.3333333333333333703),
 ( 0.3333333333333333703, 0.3333333333333333703),
 ( 1.000000000000000000, 1.000000000000000000) ) ) 
 REPRESENTATION_ITEM ( '' )  SURFACE ( )  );
#6860=AXIS2_PLACEMENT_3D ( 'NONE', #43489, #21321, #28692 ) ;
#6862=ORIENTED_EDGE ( 'NONE', *, *, #1030, .F. ) ;
#6864=CARTESIAN_POINT ( 'NONE',  ( -18.66311988809301425, -7.868636481342422329, 70.65595886192740238 ) ) ;
#6866=EDGE_CURVE ( 'NONE', #33816, #45314, #16183, .T. ) ;
#6868=CARTESIAN_POINT ( 'NONE',  ( -20.24469356570329737, -8.402152009130100296, 70.53483737320162561 ) ) ;
#6869=EDGE_LOOP ( 'NONE', ( #23322, #29989, #351, #30970, #2624 ) ) ;
#6872=CARTESIAN_POINT ( 'NONE',  ( -19.77435985551070274, -21.87886194922281646, 65.64981515446680760 ) ) ;
#6873=CARTESIAN_POINT ( 'NONE',  ( -21.63003847667031820, -8.659812987350562707, 73.74095428391912321 ) ) ;
#6874=ORIENTED_EDGE ( 'NONE', *, *, #48193, .F. ) ;
#6880=ORIENTED_EDGE ( 'NONE', *, *, #3825, .T. ) ;
#6881=EDGE_CURVE ( 'NONE', #30739, #25120, #36319, .T. ) ;
#6883=CARTESIAN_POINT ( 'NONE',  ( -16.93008532196563820, -7.826600119876228057, 73.97520714747764714 ) ) ;
#6884=PLANE ( 'NONE',  #40624 ) ;
#6886=EDGE_CURVE ( 'NONE', #46504, #39476, #28909, .T. ) ;
#6887=PLANE ( 'NONE',  #2975 ) ;
#6888=CARTESIAN_POINT ( 'NONE',  ( -12.84691039585993444, -8.931012183600500975, 67.56438067310742213 ) ) ;
#6889=CARTESIAN_POINT ( 'NONE',  ( -15.55171241031346696, -7.598245096497682205, 70.79485117658632021 ) ) ;
#6890=CARTESIAN_POINT ( 'NONE',  ( -14.66287603173356757, -8.376693951416614325, 63.78978834288939481 ) ) ;
#6892=DIRECTION ( 'NONE',  ( -0.5729733056696844073, 0.8195740302071246042, 7.403245352187747277E-08 ) ) ;
#6895=CARTESIAN_POINT ( 'NONE',  ( -13.53206638028301434, -8.990422041175579082, 60.72333783371806248 ) ) ;
#6897=EDGE_LOOP ( 'NONE', ( #35135, #6316, #21399, #30806, #43864 ) ) ;
#6900=CARTESIAN_POINT ( 'NONE',  ( -23.35165829388149561, -19.32240830869099923, 59.04443984693184433 ) ) ;
#6901=CARTESIAN_POINT ( 'NONE',  ( -24.31482301288783887, -13.31912224170856796, 59.66267924674055223 ) ) ;
#6905=CARTESIAN_POINT ( 'NONE',  ( -13.54792730259346456, -8.920061342218058797, 57.25495614889487683 ) ) ;
#6906=FACE_OUTER_BOUND ( 'NONE', #24024, .T. ) ;
#6907=ORIENTED_EDGE ( 'NONE', *, *, #17076, .T. ) ;
#6910=CARTESIAN_POINT ( 'NONE',  ( -10.88209242003807908, -17.29963164818252608, 64.62739380462950578 ) ) ;
#6913=CARTESIAN_POINT ( 'NONE',  ( -24.12942661661615418, -12.79921782163564004, 70.07243032623514978 ) ) ;
#6914=ORIENTED_EDGE ( 'NONE', *, *, #17197, .T. ) ;
#6915=CARTESIAN_POINT ( 'NONE',  ( -19.49109506855409180, -21.54969648977046148, 62.28031529404344013 ) ) ;
#6916=CARTESIAN_POINT ( 'NONE',  ( -23.66739264960602540, -11.53441051760089842, 66.42214525760398658 ) ) ;
#6918=CARTESIAN_POINT ( 'NONE',  ( -24.18037300165767434, -17.94870813986570113, 59.18873840842728384 ) ) ;
#6919=CARTESIAN_POINT ( 'NONE',  ( -10.44916039635137039, -15.83526825291551177, 64.50771589744864798 ) ) ;
#6924=CARTESIAN_POINT ( 'NONE',  ( -24.26435699358934883, -17.76123410301217120, 62.51715077956382771 ) ) ;
#6925=CARTESIAN_POINT ( 'NONE',  ( -22.86648298414092650, -19.29628210902822261, 58.97590826583130763 ) ) ;
#6927=ORIENTED_EDGE ( 'NONE', *, *, #20467, .T. ) ;
#6928=CARTESIAN_POINT ( 'NONE',  ( -24.87238774844131584, -14.64917985650991206, 62.81322232226264646 ) ) ;
#6929=AXIS2_PLACEMENT_3D ( 'NONE', #9965, #5561, #35807 ) ;
#6931=CARTESIAN_POINT ( 'NONE',  ( -10.70566838141854404, -16.94585318031169763, 57.83760548748448116 ) ) ;
#6933=DIRECTION ( 'NONE',  ( -1.420801289120338746E-06, -1.008342286982562053E-05, 0.9999999999481529178 ) ) ;
#6934=CARTESIAN_POINT ( 'NONE',  ( -16.26195973558533936, -21.76306465430365122, 58.57113428431811997 ) ) ;
#6936=VERTEX_POINT ( 'NONE', #28440 ) ;
#6939=FACE_OUTER_BOUND ( 'NONE', #7012, .T. ) ;
#6943=CARTESIAN_POINT ( 'NONE',  ( -20.72574062298286535, -8.580111251864035893, 59.84125250080548142 ) ) ;
#6944=CARTESIAN_POINT ( 'NONE',  ( -15.32650908999326411, -21.54008551964724560, 68.87033137010456585 ) ) ;
#6946=CARTESIAN_POINT ( 'NONE',  ( -11.65778227265581712, -18.77778952248012345, 64.85592980783576422 ) ) ;
#6947=EDGE_CURVE ( 'NONE', #33004, #32745, #28438, .T. ) ;
#6948=CARTESIAN_POINT ( 'NONE',  ( -12.41310947992116098, -19.76871611099698001, 61.68206578716802113 ) ) ;
#6949=FACE_BOUND ( 'NONE', #26041, .T. ) ;
#6951=FACE_OUTER_BOUND ( 'NONE', #6294, .T. ) ;
#6952=EDGE_CURVE ( 'NONE', #15253, #12237, #32522, .T. ) ;
#6954=VERTEX_POINT ( 'NONE', #44430 ) ;
#6955=CARTESIAN_POINT ( 'NONE',  ( -24.12380779853282675, -11.55065473049533686, 63.13031021406904841 ) ) ;
#6957=FACE_OUTER_BOUND ( 'NONE', #47813, .T. ) ;
#6958=CARTESIAN_POINT ( 'NONE',  ( -21.89826263122328953, -8.852228171720549099, 66.84645388252840803 ) ) ;
#6960=LINE ( 'NONE', #38875, #27567 ) ;
#6961=CARTESIAN_POINT ( 'NONE',  ( -16.09877598409873656, -7.881120331165020865, 67.44007573990704429 ) ) ;
#6963=EDGE_LOOP ( 'NONE', ( #47608, #33860 ) ) ;
#6964=VERTEX_POINT ( 'NONE', #19043 ) ;
#6967=CARTESIAN_POINT ( 'NONE',  ( -17.35317073117489173, -7.359421519614389062, 67.14226862839939258 ) ) ;
#6968=VECTOR ( 'NONE', #14827, 1000.000000000000114 ) ;
#6969=CARTESIAN_POINT ( 'NONE',  ( -18.71951286714620011, -7.876189896296080128, 66.78582905748461940 ) ) ;
#6972=LINE ( 'NONE', #10434, #41039 ) ;
#6973=CARTESIAN_POINT ( 'NONE',  ( -9.974215871585233373, -14.86485004610319827, 74.91283608227215041 ) ) ;
#6975=CARTESIAN_POINT ( 'NONE',  ( -13.11946000997128436, -9.225961346166455357, 67.52942785706356688 ) ) ;
#6976=CARTESIAN_POINT ( 'NONE',  ( -22.07446999803020660, -20.10798665040887556, 62.23439171591935093 ) ) ;
#6977=EDGE_LOOP ( 'NONE', ( #46460, #5730, #37325, #740 ) ) ;
#6979=EDGE_CURVE ( 'NONE', #29080, #17056, #41360, .T. ) ;
#6982=CARTESIAN_POINT ( 'NONE',  ( -19.23170823189057543, -21.62663761134119156, 62.40992444795293892 ) ) ;
#6983=CARTESIAN_POINT ( 'NONE',  ( -20.89619716791787596, -20.95408004043368067, 69.19883325555726117 ) ) ;
#6986=CARTESIAN_POINT ( 'NONE',  ( -17.72634075389897035, -21.85272461700124680, 58.55553378267870812 ) ) ;
#6987=CARTESIAN_POINT ( 'NONE',  ( -24.39403741458288266, -17.44049236422942784, 69.52844466935830781 ) ) ;
#6988=( BOUNDED_SURFACE ( )  B_SPLINE_SURFACE ( 3, 1, ( 
 ( #42877, #24655 ),
 ( #31546, #1753 ),
 ( #9387, #9641 ),
 ( #43114, #20473 ),
 ( #1988, #1501 ),
 ( #16981, #8907 ),
 ( #20949, #24407 ) ),
 .UNSPECIFIED., .T., .F., .F. ) 
 B_SPLINE_SURFACE_WITH_KNOTS ( ( 4, 3, 4 ),
 ( 2, 2 ),
 ( 0.000000000000000000, 0.5000000000000000000, 1.000000000000000000 ),
 ( 0.000000000000000000, 1.000000000000000000 ),
 .UNSPECIFIED. ) 
 GEOMETRIC_REPRESENTATION_ITEM ( )  RATIONAL_B_SPLINE_SURFACE ( (
 ( 1.000000000000000000, 1.000000000000000000),
 ( 0.3333333333333335369, 0.3333333333333330373),
 ( 0.3333333333333335369, 0.3333333333333330373),
 ( 1.000000000000000000, 1.000000000000000000),
 ( 0.3333333333333333703, 0.3333333333333333703),
 ( 0.3333333333333333703, 0.3333333333333333703),
 ( 1.000000000000000000, 1.000000000000000000) ) ) 
 REPRESENTATION_ITEM ( '' )  SURFACE ( )  );
#6989=CARTESIAN_POINT ( 'NONE',  ( -14.97037705864080337, -21.36678033093551221, 65.21669700154754423 ) ) ;
#6990=FACE_OUTER_BOUND ( 'NONE', #43084, .T. ) ;
#6993=EDGE_CURVE ( 'NONE', #2344, #11451, #22528, .T. ) ;
#6994=CYLINDRICAL_SURFACE ( 'NONE', #5830, 0.1500000000000067668 ) ;
#6995=CARTESIAN_POINT ( 'NONE',  ( -23.37999588001404661, -18.58199455739222827, 69.57899840282863124 ) ) ;
#6998=B_SPLINE_CURVE_WITH_KNOTS ( 'NONE', 3,
 ( #10980, #41017, #29943, #14385, #22301, #11227, #7299, #44005, #29206, #10258 ),
 .UNSPECIFIED., .F., .F.,
 ( 4, 2, 2, 2, 4 ),
 ( 0.6272669072878331864, 0.7522669073073295909, 0.8772669073268261064, 1.002266907346322622, 1.127266907365819026 ),
 .UNSPECIFIED. ) ;
#6999=DIRECTION ( 'NONE',  ( 6.651268170491444817E-06, 3.577353459756793540E-06, 0.9999999999714814791 ) ) ;
#7000=CARTESIAN_POINT ( 'NONE',  ( -24.38570565625541064, -13.64691002463509939, 59.50701104079105619 ) ) ;
#7001=ORIENTED_EDGE ( 'NONE', *, *, #40614, .F. ) ;
#7002=CARTESIAN_POINT ( 'NONE',  ( -19.22579309969192707, -21.57336792462666253, 58.52507384993226225 ) ) ;
#7004=CARTESIAN_POINT ( 'NONE',  ( -24.47401588851211329, -14.84236380343934592, 59.24300237059242136 ) ) ;
#7005=CARTESIAN_POINT ( 'NONE',  ( -21.33159362617910659, -4.962723823544877177, 53.49999999999995026 ) ) ;
#7007=( BOUNDED_CURVE ( )  B_SPLINE_CURVE ( 3, ( #19819, #27194, #1091, #5038 ),
 .UNSPECIFIED., .F., .F. ) 
 B_SPLINE_CURVE_WITH_KNOTS ( ( 4, 4 ),
 ( 0.4074455897393602921, 0.5000000000000000000 ),
 .UNSPECIFIED. ) 
 CURVE ( )  GEOMETRIC_REPRESENTATION_ITEM ( )  RATIONAL_B_SPLINE_CURVE ( ( 0.6983129098260847378, 0.7760317562606872110, 0.8765941196519910772, 0.9999999999999936717 ) ) 
 REPRESENTATION_ITEM ( '' )  );
#7008=LINE ( 'NONE', #14118, #2676 ) ;
#7012=EDGE_LOOP ( 'NONE', ( #28332, #45638, #21521, #274, #1766 ) ) ;
#7016=EDGE_CURVE ( 'NONE', #43308, #43598, #11899, .T. ) ;
#7017=EDGE_CURVE ( 'NONE', #1136, #8232, #42427, .T. ) ;
#7018=CARTESIAN_POINT ( 'NONE',  ( -23.75972628784533569, -10.79550978475970346, 53.49999999999994316 ) ) ;
#7019=DIRECTION ( 'NONE',  ( -0.3478314405900310158, -0.9375570856950865561, 0.000000000000000000 ) ) ;
#7020=CARTESIAN_POINT ( 'NONE',  ( -21.97361464010840493, -9.423584070311036953, 60.02171205573912260 ) ) ;
#7021=B_SPLINE_CURVE_WITH_KNOTS ( 'NONE', 3,
 ( #13511, #33189, #44311, #48222, #25342, #9614, #28557, #18174, #28788, #2913 ),
 .UNSPECIFIED., .F., .F.,
 ( 4, 2, 2, 2, 4 ),
 ( 0.000000000000000000, 0.2500000000000000000, 0.5000000000000000000, 0.7500000000000000000, 1.000000000000000000 ),
 .UNSPECIFIED. ) ;
#7023=( BOUNDED_CURVE ( )  B_SPLINE_CURVE ( 3, ( #33708, #11, #8367, #19199 ),
 .UNSPECIFIED., .F., .F. ) 
 B_SPLINE_CURVE_WITH_KNOTS ( ( 4, 4 ),
 ( 0.5000000000000000000, 0.9074455897393643999 ),
 .UNSPECIFIED. ) 
 CURVE ( )  GEOMETRIC_REPRESENTATION_ITEM ( )  RATIONAL_B_SPLINE_CURVE ( ( 1.000000000000001998, 0.4567392136813338555, 0.3561768502900293787, 0.6983129098260909551 ) ) 
 REPRESENTATION_ITEM ( '' )  );
#7024=VERTEX_POINT ( 'NONE', #26431 ) ;
#7027=CARTESIAN_POINT ( 'NONE',  ( -11.43418267526448417, -10.37927948953321966, 74.63159157388955123 ) ) ;
#7028=FACE_OUTER_BOUND ( 'NONE', #753, .T. ) ;
#7030=EDGE_CURVE ( 'NONE', #38940, #23317, #44924, .T. ) ;
#7031=ADVANCED_FACE ( 'NONE', ( #18292 ), #15905, .T. ) ;
#7032=ORIENTED_EDGE ( 'NONE', *, *, #47835, .F. ) ;
#7033=EDGE_CURVE ( 'NONE', #36030, #47790, #14210, .T. ) ;
#7034=EDGE_CURVE ( 'NONE', #31755, #32446, #33299, .T. ) ;
#7035=CARTESIAN_POINT ( 'NONE',  ( -24.37622078247382618, -15.62647719184611184, 69.72410579710512479 ) ) ;
#7036=AXIS2_PLACEMENT_3D ( 'NONE', #2397, #13698, #21601 ) ;
#7037=CARTESIAN_POINT ( 'NONE',  ( -18.76269919900832761, -7.938388845612718292, 67.09174861995765582 ) ) ;
#7038=CARTESIAN_POINT ( 'NONE',  ( -21.31115985637654120, -8.927249709250720144, 73.88656608925673197 ) ) ;
#7039=VERTEX_POINT ( 'NONE', #27163 ) ;
#7042=VECTOR ( 'NONE', #44218, 1000.000000000000000 ) ;
#7043=VERTEX_POINT ( 'NONE', #27645 ) ;
#7045=CARTESIAN_POINT ( 'NONE',  ( -10.12771871015461755, -16.31437777856581661, 71.64739150203183726 ) ) ;
#7046=CARTESIAN_POINT ( 'NONE',  ( -24.42338698107307948, -14.97596128575578511, 59.31470420106809627 ) ) ;
#7047=CARTESIAN_POINT ( 'NONE',  ( -12.15399301493812878, -9.543295845094297292, 57.20440096431307353 ) ) ;
#7048=ORIENTED_EDGE ( 'NONE', *, *, #32245, .T. ) ;
#7050=AXIS2_PLACEMENT_3D ( 'NONE', #35810, #21543, #14110 ) ;
#7051=CARTESIAN_POINT ( 'NONE',  ( -24.42568804794990811, -14.79584343669470847, 62.82369473970615559 ) ) ;
#7052=DIRECTION ( 'NONE',  ( -0.1922068328301543838, -0.9813544382196449645, 7.804899501296265607E-08 ) ) ;
#7053=DIRECTION ( 'NONE',  ( -2.191687988502693051E-06, 1.258878959409210278E-05, 0.9999999999183594168 ) ) ;
#7054=ORIENTED_EDGE ( 'NONE', *, *, #36469, .T. ) ;
#7055=LINE ( 'NONE', #22068, #44870 ) ;
#7056=CARTESIAN_POINT ( 'NONE',  ( -14.66630222544869078, -8.320656262913125545, 63.80450889863892172 ) ) ;
#7057=CARTESIAN_POINT ( 'NONE',  ( -18.69688219364054049, -7.467975623574482746, 70.48412626434020467 ) ) ;
#7059=FACE_BOUND ( 'NONE', #45629, .T. ) ;
#7060=EDGE_LOOP ( 'NONE', ( #48713, #11075 ) ) ;
#7061=DIRECTION ( 'NONE',  ( 0.05202058437830280740, -0.9986460127597464043, 1.657953767687799580E-08 ) ) ;
#7062=CARTESIAN_POINT ( 'NONE',  ( -13.64037081340465818, -20.69854240475087437, 61.53148696990430011 ) ) ;
#7063=EDGE_CURVE ( 'NONE', #8174, #26823, #20667, .T. ) ;
#7064=VECTOR ( 'NONE', #41091, 1000.000000000000227 ) ;
#7065=CARTESIAN_POINT ( 'NONE',  ( -24.42218830512229388, -14.64588455312011739, 63.01296487252135137 ) ) ;
#7067=CARTESIAN_POINT ( 'NONE',  ( -21.41863048803933012, -8.999699081277377388, 73.61600897546567523 ) ) ;
#7069=ORIENTED_EDGE ( 'NONE', *, *, #45635, .F. ) ;
#7070=LINE ( 'NONE', #37315, #32885 ) ;
#7071=CARTESIAN_POINT ( 'NONE',  ( -15.48628188820593543, -7.614865071177022493, 74.26641013817956605 ) ) ;
#7072=ORIENTED_EDGE ( 'NONE', *, *, #25606, .T. ) ;
#7073=CARTESIAN_POINT ( 'NONE',  ( -10.16572694778485442, -13.12977483508055165, 71.38545448699323970 ) ) ;
#7074=DIRECTION ( 'NONE',  ( 5.935091885992485906E-07, 2.117535305676834604E-07, -0.9999999999998013811 ) ) ;
#7075=EDGE_CURVE ( 'NONE', #38907, #36780, #16587, .T. ) ;
#7076=ORIENTED_EDGE ( 'NONE', *, *, #23328, .T. ) ;
#7077=ORIENTED_EDGE ( 'NONE', *, *, #17029, .F. ) ;
#7078=CARTESIAN_POINT ( 'NONE',  ( -13.99679447977218061, -20.97040113148658591, 71.94079819673058296 ) ) ;
#7080=FACE_OUTER_BOUND ( 'NONE', #12844, .T. ) ;
#7081=CARTESIAN_POINT ( 'NONE',  ( -23.47573984560501259, -19.15461428502270280, 62.49260334658298177 ) ) ;
#7082=CARTESIAN_POINT ( 'NONE',  ( -10.03581529055505506, -13.85215573028183655, 57.64836240523872846 ) ) ;
#7083=CARTESIAN_POINT ( 'NONE',  ( -21.23815497595111879, -21.20890771667191999, 65.69115622141528377 ) ) ;
#7085=CARTESIAN_POINT ( 'NONE',  ( -20.57133303063786300, -8.056536552513840377, 67.03749994897439990 ) ) ;
#7087=ORIENTED_EDGE ( 'NONE', *, *, #40842, .T. ) ;
#7088=ORIENTED_EDGE ( 'NONE', *, *, #25562, .F. ) ;
#7089=CARTESIAN_POINT ( 'NONE',  ( -24.84033948030421968, -15.52542097194404569, 73.11648385888869939 ) ) ;
#7090=CARTESIAN_POINT ( 'NONE',  ( -19.70639647806698136, -21.90109437720271757, 65.57990800639531415 ) ) ;
#7091=CARTESIAN_POINT ( 'NONE',  ( -14.60689786731817286, -8.346551761976032324, 63.93978840692965093 ) ) ;
#7092=AXIS2_PLACEMENT_3D ( 'NONE', #33179, #36393, #20913 ) ;
#7097=B_SPLINE_CURVE_WITH_KNOTS ( 'NONE', 3,
 ( #36362, #34071, #7269, #7510, #22515, #25060, #48607, #33320, #23023, #15591 ),
 .UNSPECIFIED., .F., .F.,
 ( 4, 2, 2, 2, 4 ),
 ( 0.000000000000000000, 0.2500000000000000000, 0.5000000000000000000, 0.7500000000000000000, 1.000000000000000000 ),
 .UNSPECIFIED. ) ;
#7098=ORIENTED_EDGE ( 'NONE', *, *, #16877, .T. ) ;
#7099=EDGE_CURVE ( 'NONE', #19673, #3400, #41079, .T. ) ;
#7101=CARTESIAN_POINT ( 'NONE',  ( -20.03282965983824226, -21.84088468745754597, 56.49999999999994316 ) ) ;
#7103=LINE ( 'NONE', #11032, #4796 ) ;
#7105=EDGE_CURVE ( 'NONE', #24743, #39816, #4837, .T. ) ;
#7107=CARTESIAN_POINT ( 'NONE',  ( -18.87585836598739064, -7.910150609727056192, 67.19511962462686938 ) ) ;
#7110=ORIENTED_EDGE ( 'NONE', *, *, #46959, .T. ) ;
#7111=CARTESIAN_POINT ( 'NONE',  ( -15.18457398882241449, -21.44135615956592744, 65.39131358081642986 ) ) ;
#7112=AXIS2_PLACEMENT_3D ( 'NONE', #31268, #12555, #12310 ) ;
#7114=ORIENTED_EDGE ( 'NONE', *, *, #40980, .F. ) ;
#7115=B_SPLINE_CURVE_WITH_KNOTS ( 'NONE', 1,
 ( #5488, #1533 ),
 .UNSPECIFIED., .F., .F.,
 ( 2, 2 ),
 ( 0.000000000000000000, 1.000000000000000000 ),
 .UNSPECIFIED. ) ;
#7116=DIRECTION ( 'NONE',  ( 0.9942595023566569434, -0.1069955231469581769, 3.800058679842193584E-08 ) ) ;
#7117=CIRCLE ( 'NONE', #44882, 6.899999999999999467 ) ;
#7118=ORIENTED_EDGE ( 'NONE', *, *, #46416, .T. ) ;
#7121=EDGE_LOOP ( 'NONE', ( #48578, #25530 ) ) ;
#7122=CARTESIAN_POINT ( 'NONE',  ( -12.95890174405234241, -8.844667670358365541, 67.56598159878524257 ) ) ;
#7123=EDGE_CURVE ( 'NONE', #10658, #27516, #23694, .T. ) ;
#7124=CARTESIAN_POINT ( 'NONE',  ( -18.62040859620581301, -22.16269830898913540, 72.44544270657438290 ) ) ;
#7125=VERTEX_POINT ( 'NONE', #45885 ) ;
#7126=DIRECTION ( 'NONE',  ( -0.5263399769092093061, 0.8502742079512978224, 7.678741024442198749E-08 ) ) ;
#7129=CARTESIAN_POINT ( 'NONE',  ( -24.86571005758334252, -14.45474999747601252, 66.29018563260261487 ) ) ;
#7131=FACE_OUTER_BOUND ( 'NONE', #17963, .T. ) ;
#7135=ORIENTED_EDGE ( 'NONE', *, *, #14447, .T. ) ;
#7136=CARTESIAN_POINT ( 'NONE',  ( -22.76532612177806314, -10.19550891705927498, 73.62593845350987465 ) ) ;
#7137=CARTESIAN_POINT ( 'NONE',  ( -16.87238795883161657, -7.830921832911093894, 74.03306333698706965 ) ) ;
#7138=FACE_OUTER_BOUND ( 'NONE', #7905, .T. ) ;
#7140=CARTESIAN_POINT ( 'NONE',  ( -24.08977912471840810, -11.48169904069885661, 62.99572364416607684 ) ) ;
#7141=CARTESIAN_POINT ( 'NONE',  ( -13.06813783877040969, -9.265530354883374287, 67.66470656304637998 ) ) ;
#7143=CARTESIAN_POINT ( 'NONE',  ( -16.56797618387698279, -22.20990603440958111, 65.41838526417717503 ) ) ;
#7145=CYLINDRICAL_SURFACE ( 'NONE', #48547, 0.1500000000000039913 ) ;
#7146=CARTESIAN_POINT ( 'NONE',  ( -14.43441977789444763, -8.421195553735145722, 71.14446303425738449 ) ) ;
#7150=( BOUNDED_CURVE ( )  B_SPLINE_CURVE ( 3, ( #43493, #27728, #21069, #39538 ),
 .UNSPECIFIED., .F., .F. ) 
 B_SPLINE_CURVE_WITH_KNOTS ( ( 4, 4 ),
 ( 4.712388980384689674, 4.921828490624009511 ),
 .UNSPECIFIED. ) 
 CURVE ( )  GEOMETRIC_REPRESENTATION_ITEM ( )  RATIONAL_B_SPLINE_CURVE ( ( 1.000000000000000000, 0.9963479302455154896, 0.9963479302455154896, 1.000000000000000000 ) ) 
 REPRESENTATION_ITEM ( '' )  );
#7151=AXIS2_PLACEMENT_3D ( 'NONE', #40231, #28177, #39500 ) ;
#7153=ORIENTED_EDGE ( 'NONE', *, *, #44651, .T. ) ;
#7156=CARTESIAN_POINT ( 'NONE',  ( -23.00441852451001523, -19.11762575345012749, 58.88410642058936872 ) ) ;
#7158=PLANE ( 'NONE',  #15420 ) ;
#7159=B_SPLINE_CURVE_WITH_KNOTS ( 'NONE', 3,
 ( #34126, #7329, #3365, #25775, #11486, #22572, #14650, #22326, #40791, #18371 ),
 .UNSPECIFIED., .F., .F.,
 ( 4, 2, 2, 2, 4 ),
 ( 0.000000000000000000, 0.2500000000000000000, 0.5000000000000000000, 0.7500000000000000000, 1.000000000000000000 ),
 .UNSPECIFIED. ) ;
#7161=( BOUNDED_CURVE ( )  B_SPLINE_CURVE ( 3, ( #14014, #17721, #32520, #47062 ),
 .UNSPECIFIED., .F., .F. ) 
 B_SPLINE_CURVE_WITH_KNOTS ( ( 4, 4 ),
 ( 0.5000000000000000000, 0.9074455897393561843 ),
 .UNSPECIFIED. ) 
 CURVE ( )  GEOMETRIC_REPRESENTATION_ITEM ( )  RATIONAL_B_SPLINE_CURVE ( ( 1.000000000000013545, 0.4567392136813450132, 0.3561768502900254374, 0.6983129098260696388 ) ) 
 REPRESENTATION_ITEM ( '' )  );
#7162=CARTESIAN_POINT ( 'NONE',  ( -23.61204096558246235, -11.53669824655086451, 66.72214514747398084 ) ) ;
#7163=EDGE_CURVE ( 'NONE', #11354, #38153, #27399, .T. ) ;
#7171=EDGE_CURVE ( 'NONE', #30917, #41834, #39205, .T. ) ;
#7172=CARTESIAN_POINT ( 'NONE',  ( -22.96481576609224717, -19.16891988936071556, 58.89882756593014790 ) ) ;
#7173=VERTEX_POINT ( 'NONE', #1786 ) ;
#7174=CARTESIAN_POINT ( 'NONE',  ( -20.15112924866626187, -10.01741632518351643, 53.69233794759168887 ) ) ;
#7175=ORIENTED_EDGE ( 'NONE', *, *, #32228, .T. ) ;
#7176=CARTESIAN_POINT ( 'NONE',  ( -19.44142144650348314, -21.98165757830647138, 62.18158996068683564 ) ) ;
#7177=B_SPLINE_CURVE_WITH_KNOTS ( 'NONE', 3,
 ( #20683, #40299, #42617, #1464, #31759, #9116, #46299, #5177, #47928, #46779 ),
 .UNSPECIFIED., .F., .F.,
 ( 4, 2, 2, 2, 4 ),
 ( 0.000000000000000000, 0.2500000000000000000, 0.5000000000000000000, 0.7500000000000000000, 1.000000000000000000 ),
 .UNSPECIFIED. ) ;
#7179=ORIENTED_EDGE ( 'NONE', *, *, #14546, .T. ) ;
#7180=CARTESIAN_POINT ( 'NONE',  ( -24.15358334166845111, -18.00564352615971941, 59.19716716663268130 ) ) ;
#7181=CARTESIAN_POINT ( 'NONE',  ( -10.39215589072981416, -14.30487699944780289, 64.68803863382906627 ) ) ;
#7182=EDGE_CURVE ( 'NONE', #9242, #18330, #35738, .T. ) ;
#7185=CARTESIAN_POINT ( 'NONE',  ( -14.42683419600289341, -8.428067575814653267, 67.55975083869262221 ) ) ;
#7187=FACE_OUTER_BOUND ( 'NONE', #24691, .T. ) ;
#7190=LINE ( 'NONE', #44145, #23128 ) ;
#7191=CARTESIAN_POINT ( 'NONE',  ( -9.990737576226866423, -14.31032742905966337, 64.43157936802064967 ) ) ;
#7192=CARTESIAN_POINT ( 'NONE',  ( -14.45653002406802834, -7.975746824180188099, 63.98990036560820016 ) ) ;
#7193=CARTESIAN_POINT ( 'NONE',  ( -12.55411140858086760, -19.90724249994213935, 65.15202838036978505 ) ) ;
#7194=B_SPLINE_CURVE_WITH_KNOTS ( 'NONE', 1,
 ( #18867, #44494 ),
 .UNSPECIFIED., .F., .F.,
 ( 2, 2 ),
 ( 0.000000000000000000, 1.000000000000000000 ),
 .UNSPECIFIED. ) ;
#7195=CARTESIAN_POINT ( 'NONE',  ( -18.71757194967216975, -7.929750632967406787, 70.37068030597254165 ) ) ;
#7196=CARTESIAN_POINT ( 'NONE',  ( -23.81024829756716343, -18.64597716098235836, 72.94863620959463901 ) ) ;
#7197=ORIENTED_EDGE ( 'NONE', *, *, #36790, .T. ) ;
#7200=CARTESIAN_POINT ( 'NONE',  ( -14.86277779823650391, -8.294567775944363675, 57.07673407009221478 ) ) ;
#7201=EDGE_LOOP ( 'NONE', ( #43513, #21073, #36835, #15298 ) ) ;
#7202=CARTESIAN_POINT ( 'NONE',  ( -14.68550372792196335, -21.30572237930008939, 58.17177643121559782 ) ) ;
#7205=CARTESIAN_POINT ( 'NONE',  ( -20.68222199850074361, -8.109235517929556991, 63.47154877063784539 ) ) ;
#7206=CARTESIAN_POINT ( 'NONE',  ( -22.33142775017075010, -9.202805011845722305, 59.90826508960974195 ) ) ;
#7207=CARTESIAN_POINT ( 'NONE',  ( -11.29219319990544079, -18.28864530752396433, 57.82186711835544912 ) ) ;
#7208=CARTESIAN_POINT ( 'NONE',  ( -11.07238894598444112, -11.74315414212633080, 67.50375847841529264 ) ) ;
#7209=CARTESIAN_POINT ( 'NONE',  ( -11.45241200840138340, -19.26367093908298500, 71.79347555607934339 ) ) ;
#7210=CARTESIAN_POINT ( 'NONE',  ( -16.78865379391102408, -21.78030513117466072, 68.69560651887046276 ) ) ;
#7211=VERTEX_POINT ( 'NONE', #43406 ) ;
#7212=CARTESIAN_POINT ( 'NONE',  ( -24.09981952095640167, -11.50204489274636366, 63.15207061483707207 ) ) ;
#7213=CARTESIAN_POINT ( 'NONE',  ( -21.50517322895428052, -9.056100137350421519, 66.86969788852485408 ) ) ;
#7214=CARTESIAN_POINT ( 'NONE',  ( -24.70336335543259665, -13.22337356223611060, 59.56256691634375500 ) ) ;
#7216=CARTESIAN_POINT ( 'NONE',  ( -24.59748878097435210, -12.79772186451832994, 66.34600794915635902 ) ) ;
#7217=EDGE_CURVE ( 'NONE', #21955, #5832, #32591, .T. ) ;
#7218=CARTESIAN_POINT ( 'NONE',  ( -11.83525287003876336, -10.59418596192610096, 74.73885130397258081 ) ) ;
#7220=VERTEX_POINT ( 'NONE', #24689 ) ;
#7221=ORIENTED_EDGE ( 'NONE', *, *, #22516, .F. ) ;
#7223=B_SPLINE_CURVE_WITH_KNOTS ( 'NONE', 1,
 ( #4196, #22917 ),
 .UNSPECIFIED., .F., .F.,
 ( 2, 2 ),
 ( 0.000000000000000000, 1.000000000000000000 ),
 .UNSPECIFIED. ) ;
#7224=AXIS2_PLACEMENT_3D ( 'NONE', #12951, #13432, #13904 ) ;
#7227=CARTESIAN_POINT ( 'NONE',  ( -22.23733836534369601, -19.96043719841513564, 65.85421731380807842 ) ) ;
#7228=CARTESIAN_POINT ( 'NONE',  ( -24.01119280393830024, -17.17795836609833415, 69.69874480771339620 ) ) ;
#7229=CARTESIAN_POINT ( 'NONE',  ( -24.61791017297192852, -12.87185432802827734, 66.48059519668728967 ) ) ;
#7231=ORIENTED_EDGE ( 'NONE', *, *, #25336, .T. ) ;
#7232=EDGE_CURVE ( 'NONE', #27202, #37668, #35737, .T. ) ;
#7233=CARTESIAN_POINT ( 'NONE',  ( -24.37280409347697230, -15.65865158627326537, 73.28687223815994400 ) ) ;
#7235=LINE ( 'NONE', #15307, #27321 ) ;
#7237=ORIENTED_EDGE ( 'NONE', *, *, #48000, .F. ) ;
#7240=EDGE_LOOP ( 'NONE', ( #6843, #27671 ) ) ;
#7241=EDGE_CURVE ( 'NONE', #29883, #30739, #25983, .T. ) ;
#7242=CARTESIAN_POINT ( 'NONE',  ( -19.50997552649656086, -21.96132259753523996, 62.25149580216906742 ) ) ;
#7243=CARTESIAN_POINT ( 'NONE',  ( -21.12516169987187098, -20.80993955427394582, 69.06922321213187388 ) ) ;
#7244=CARTESIAN_POINT ( 'NONE',  ( -13.11946129443726861, -9.225960368241006293, 67.37942785707224402 ) ) ;
#7245=VERTEX_POINT ( 'NONE', #16785 ) ;
#7246=CARTESIAN_POINT ( 'NONE',  ( -11.16823349194678627, -11.55205338407005122, 71.50349565124497531 ) ) ;
#7247=CARTESIAN_POINT ( 'NONE',  ( -11.64235026963700470, -18.84330375823651949, 68.21689631561287115 ) ) ;
#7251=ORIENTED_EDGE ( 'NONE', *, *, #35624, .T. ) ;
#7252=CARTESIAN_POINT ( 'NONE',  ( -11.13352401182878459, -11.60862911821036292, 74.70272630447266238 ) ) ;
#7254=CYLINDRICAL_SURFACE ( 'NONE', #30195, 0.1500000000000040190 ) ;
#7255=DIRECTION ( 'NONE',  ( -0.6043825497304157190, 0.7966942535134532433, -5.656674838623230539E-08 ) ) ;
#7257=B_SPLINE_CURVE_WITH_KNOTS ( 'NONE', 3,
 ( #5722, #40171, #14028, #32531, #21690, #43137, #28109, #25149, #9890, #43393 ),
 .UNSPECIFIED., .F., .F.,
 ( 4, 2, 2, 2, 4 ),
 ( 0.6272669072979107918, 0.7522669073148898766, 0.8772669073318688504, 1.002266907348847935, 1.127266907365827020 ),
 .UNSPECIFIED. ) ;
#7260=FACE_OUTER_BOUND ( 'NONE', #5682, .T. ) ;
#7261=CARTESIAN_POINT ( 'NONE',  ( -18.31357764725860093, -21.80286926110680668, 68.96514702303620936 ) ) ;
#7262=ORIENTED_EDGE ( 'NONE', *, *, #43370, .F. ) ;
#7263=CARTESIAN_POINT ( 'NONE',  ( -22.34731130624134465, -19.85564328841742920, 69.17977748773124347 ) ) ;
#7265=CARTESIAN_POINT ( 'NONE',  ( -11.69162037657732078, -10.05084142047440565, 67.69171023900449313 ) ) ;
#7266=B_SPLINE_CURVE_WITH_KNOTS ( 'NONE', 3,
 ( #7195, #17523, #10150, #32783, #6693, #8168, #23180, #45346, #26375, #22950 ),
 .UNSPECIFIED., .F., .F.,
 ( 4, 2, 2, 2, 4 ),
 ( 0.000000000000000000, 0.2500000000000000000, 0.5000000000000000000, 0.7500000000000000000, 1.000000000000000000 ),
 .UNSPECIFIED. ) ;
#7267=ORIENTED_EDGE ( 'NONE', *, *, #42489, .F. ) ;
#7269=CARTESIAN_POINT ( 'NONE',  ( -10.68182963115602924, -12.92559189733731273, 67.75449013086223715 ) ) ;
#7270=ORIENTED_EDGE ( 'NONE', *, *, #12278, .T. ) ;
#7273=CARTESIAN_POINT ( 'NONE',  ( -13.60238606012557483, -8.884930320952351579, 56.96967755506135234 ) ) ;
#7275=EDGE_CURVE ( 'NONE', #6219, #39482, #3690, .T. ) ;
#7276=CARTESIAN_POINT ( 'NONE',  ( -24.84793640206982701, -14.18443463346696909, 69.83770693398628282 ) ) ;
#7278=VERTEX_POINT ( 'NONE', #31584 ) ;
#7279=VERTEX_POINT ( 'NONE', #20506 ) ;
#7281=B_SPLINE_CURVE_WITH_KNOTS ( 'NONE', 1,
 ( #26922, #30380 ),
 .UNSPECIFIED., .F., .F.,
 ( 2, 2 ),
 ( 0.000000000000000000, 1.000000000000000000 ),
 .UNSPECIFIED. ) ;
#7283=CARTESIAN_POINT ( 'NONE',  ( -10.48067290732983281, -16.03043740265091444, 67.97767830707738312 ) ) ;
#7285=VERTEX_POINT ( 'NONE', #12856 ) ;
#7287=ADVANCED_FACE ( 'NONE', ( #6204 ), #7448, .T. ) ;
#7289=B_SPLINE_CURVE_WITH_KNOTS ( 'NONE', 3,
 ( #26832, #41852, #8124, #11556, #4911, #33958, #12281, #251, #15719, #41603 ),
 .UNSPECIFIED., .F., .F.,
 ( 4, 2, 2, 2, 4 ),
 ( 0.6272669072877233853, 0.7522669073072442147, 0.8772669073267651552, 1.002266907346285985, 1.127266907365806814 ),
 .UNSPECIFIED. ) ;
#7291=( BOUNDED_CURVE ( )  B_SPLINE_CURVE ( 3, ( #32510, #44103, #10357, #33208 ),
 .UNSPECIFIED., .F., .F. ) 
 B_SPLINE_CURVE_WITH_KNOTS ( ( 4, 4 ),
 ( 0.9074455897393668424, 1.000000000000000000 ),
 .UNSPECIFIED. ) 
 CURVE ( )  GEOMETRIC_REPRESENTATION_ITEM ( )  RATIONAL_B_SPLINE_CURVE ( ( 0.6983129098261178225, 0.7760317562607195185, 0.8765941196520136147, 1.000000000000000000 ) ) 
 REPRESENTATION_ITEM ( '' )  );
#7292=EDGE_LOOP ( 'NONE', ( #4606, #28442, #47581, #8493 ) ) ;
#7293=CARTESIAN_POINT ( 'NONE',  ( -23.08261055559088248, -18.93003034027461950, 62.65406880913197796 ) ) ;
#7294=EDGE_LOOP ( 'NONE', ( #19657, #13406, #48208, #16702, #35099 ) ) ;
#7295=EDGE_CURVE ( 'NONE', #24855, #23931, #48334, .T. ) ;
#7296=CARTESIAN_POINT ( 'NONE',  ( -13.01353397724842154, -8.804979801064929390, 64.09441804368185558 ) ) ;
#7297=CARTESIAN_POINT ( 'NONE',  ( -24.82750195234013191, -13.97654432178796569, 73.30766915316792165 ) ) ;
#7299=CARTESIAN_POINT ( 'NONE',  ( -9.992295536073678264, -14.28860446562057085, 64.48780235712654019 ) ) ;
#7300=ORIENTED_EDGE ( 'NONE', *, *, #36737, .T. ) ;
#7301=CARTESIAN_POINT ( 'NONE',  ( -11.29219319990544079, -18.28864530752396433, 57.82186711835544912 ) ) ;
#7302=CYLINDRICAL_SURFACE ( 'NONE', #9299, 0.1500000000000050737 ) ;
#7304=LINE ( 'NONE', #14631, #14778 ) ;
#7305=CARTESIAN_POINT ( 'NONE',  ( -10.08870644134023387, -16.11102152315157099, 68.17756598889880593 ) ) ;
#7306=VERTEX_POINT ( 'NONE', #41382 ) ;
#7307=CARTESIAN_POINT ( 'NONE',  ( -10.55690563545519822, -17.69827471655239037, 68.23575463352698023 ) ) ;
#7308=CARTESIAN_POINT ( 'NONE',  ( -18.53714847821261458, -22.17566945187693506, 72.54156883610106377 ) ) ;
#7309=( BOUNDED_CURVE ( )  B_SPLINE_CURVE ( 3, ( #19014, #34018, #19490, #788 ),
 .UNSPECIFIED., .F., .F. ) 
 B_SPLINE_CURVE_WITH_KNOTS ( ( 4, 4 ),
 ( 0.000000000000000000, 0.4074455897393702286 ),
 .UNSPECIFIED. ) 
 CURVE ( )  GEOMETRIC_REPRESENTATION_ITEM ( )  RATIONAL_B_SPLINE_CURVE ( ( 1.000000000000000000, 0.4567392136813277492, 0.3561768502900287126, 0.6983129098261028345 ) ) 
 REPRESENTATION_ITEM ( '' )  );
#7310=CARTESIAN_POINT ( 'NONE',  ( -10.83536388074712598, -17.31742051234312640, 64.92739380450886699 ) ) ;
#7312=FACE_BOUND ( 'NONE', #12358, .T. ) ;
#7314=CARTESIAN_POINT ( 'NONE',  ( -11.29385027892729987, -19.04286830487734861, 68.33194243210506613 ) ) ;
#7315=CARTESIAN_POINT ( 'NONE',  ( -13.64007738217462062, -20.69835563907848552, 61.80180905510582789 ) ) ;
#7316=CARTESIAN_POINT ( 'NONE',  ( -16.91478550490786859, -21.84108428878278119, 72.18015306840750611 ) ) ;
#7319=CARTESIAN_POINT ( 'NONE',  ( -10.44762901317458414, -14.23035498823898415, 64.40420498733567456 ) ) ;
#7321=CARTESIAN_POINT ( 'NONE',  ( -17.83653785972521177, -7.771132672202180736, 60.08620545617123554 ) ) ;
#7322=CARTESIAN_POINT ( 'NONE',  ( -10.95349617038790591, -18.50195306419159991, 57.94681249741275764 ) ) ;
#7325=ORIENTED_EDGE ( 'NONE', *, *, #17608, .T. ) ;
#7326=FACE_OUTER_BOUND ( 'NONE', #44405, .T. ) ;
#7327=( BOUNDED_CURVE ( )  B_SPLINE_CURVE ( 3, ( #3153, #22604, #41075, #7359 ),
 .UNSPECIFIED., .F., .F. ) 
 B_SPLINE_CURVE_WITH_KNOTS ( ( 4, 4 ),
 ( 0.000000000000000000, 0.4074455897393614023 ),
 .UNSPECIFIED. ) 
 CURVE ( )  GEOMETRIC_REPRESENTATION_ITEM ( )  RATIONAL_B_SPLINE_CURVE ( ( 1.000000000000000000, 0.4567392136813356318, 0.3561768502900316546, 0.6983129098260881795 ) ) 
 REPRESENTATION_ITEM ( '' )  );
#7329=CARTESIAN_POINT ( 'NONE',  ( -13.44722279732532577, -20.56995410411473202, 58.04650027625321940 ) ) ;
#7330=EDGE_CURVE ( 'NONE', #48127, #7024, #12460, .T. ) ;
#7331=ORIENTED_EDGE ( 'NONE', *, *, #15055, .F. ) ;
#7332=EDGE_LOOP ( 'NONE', ( #45098, #25248 ) ) ;
#7334=CARTESIAN_POINT ( 'NONE',  ( -20.50783594841701785, -8.027295835816985914, 66.96599399791791996 ) ) ;
#7335=CARTESIAN_POINT ( 'NONE',  ( -12.74836358285320159, -20.08597126951521261, 71.82125749157572159 ) ) ;
#7336=CARTESIAN_POINT ( 'NONE',  ( -10.04001549485839995, -13.81937382109866341, 57.57108164808059314 ) ) ;
#7337=B_SPLINE_CURVE_WITH_KNOTS ( 'NONE', 1,
 ( #47991, #10334 ),
 .UNSPECIFIED., .F., .F.,
 ( 2, 2 ),
 ( 0.000000000000000000, 1.000000000000000000 ),
 .UNSPECIFIED. ) ;
#7340=CARTESIAN_POINT ( 'NONE',  ( -22.47245519635065492, -19.73066437834766873, 72.65872596779033188 ) ) ;
#7341=ORIENTED_EDGE ( 'NONE', *, *, #29731, .F. ) ;
#7342=ORIENTED_EDGE ( 'NONE', *, *, #9764, .F. ) ;
#7343=CARTESIAN_POINT ( 'NONE',  ( -22.54166034846558020, -20.22352459525847834, 65.82608991095307260 ) ) ;
#7344=CARTESIAN_POINT ( 'NONE',  ( -11.12207588469793329, -10.83591208581314369, 57.35903209041984496 ) ) ;
#7347=B_SPLINE_CURVE_WITH_KNOTS ( 'NONE', 3,
 ( #23298, #4112, #16792, #46852, #4340, #5499, #45467, #2028, #20514, #23064 ),
 .UNSPECIFIED., .F., .F.,
 ( 4, 2, 2, 2, 4 ),
 ( 0.6272669072877261609, 0.7522669073072449919, 0.8772669073267638229, 1.002266907346282654, 1.127266907365801485 ),
 .UNSPECIFIED. ) ;
#7349=ORIENTED_EDGE ( 'NONE', *, *, #7033, .T. ) ;
#7350=B_SPLINE_CURVE_WITH_KNOTS ( 'NONE', 1,
 ( #41979, #15855 ),
 .UNSPECIFIED., .F., .F.,
 ( 2, 2 ),
 ( 0.000000000000000000, 1.000000000000000000 ),
 .UNSPECIFIED. ) ;
#7351=CARTESIAN_POINT ( 'NONE',  ( -10.68551981713787136, -12.73596763222149164, 64.28308208171728211 ) ) ;
#7352=CARTESIAN_POINT ( 'NONE',  ( -10.70296955259081351, -11.59513340129999648, 71.27356289404251299 ) ) ;
#7355=EDGE_LOOP ( 'NONE', ( #11017, #16189 ) ) ;
#7357=EDGE_CURVE ( 'NONE', #21857, #20491, #13613, .T. ) ;
#7358=CARTESIAN_POINT ( 'NONE',  ( -24.17273098822645494, -12.76985232770863021, 69.77243020554645625 ) ) ;
#7359=CARTESIAN_POINT ( 'NONE',  ( -21.34581862946232889, -20.66775363590295100, 72.52446429492309221 ) ) ;
#7360=ORIENTED_EDGE ( 'NONE', *, *, #12824, .T. ) ;
#7361=CARTESIAN_POINT ( 'NONE',  ( -10.43707426929608673, -13.86785048687512756, 57.45384848714355996 ) ) ;
#7362=CARTESIAN_POINT ( 'NONE',  ( -21.94239094699587511, -20.22099839777041907, 58.91442899523080001 ) ) ;
#7363=LINE ( 'NONE', #28838, #24479 ) ;
#7364=ORIENTED_EDGE ( 'NONE', *, *, #11905, .T. ) ;
#7365=PLANE ( 'NONE',  #6298 ) ;
#7368=CARTESIAN_POINT ( 'NONE',  ( -23.34481640033245853, -18.63641755246780107, 69.59371984262205046 ) ) ;
#7369=ORIENTED_EDGE ( 'NONE', *, *, #8609, .T. ) ;
#7371=CARTESIAN_POINT ( 'NONE',  ( -12.41315173547891781, -9.850077678253004621, 57.38935532239157311 ) ) ;
#7372=ORIENTED_EDGE ( 'NONE', *, *, #7513, .T. ) ;
#7373=CARTESIAN_POINT ( 'NONE',  ( -21.35244737031881712, -20.60314787972549055, 72.82446376343101235 ) ) ;
#7374=CARTESIAN_POINT ( 'NONE',  ( -19.77435985551070274, -21.87886194922281646, 65.64981515446680760 ) ) ;
#7375=FACE_OUTER_BOUND ( 'NONE', #44179, .T. ) ;
#7376=EDGE_LOOP ( 'NONE', ( #28946, #22586, #26965, #31523, #35413 ) ) ;
#7377=CARTESIAN_POINT ( 'NONE',  ( -15.03263910315855512, -8.176888424288378587, 56.86472059657746314 ) ) ;
#7378=ADVANCED_FACE ( 'NONE', ( #33738 ), #37607, .T. ) ;
#7379=FACE_OUTER_BOUND ( 'NONE', #36818, .T. ) ;
#7380=DIRECTION ( 'NONE',  ( 2.027460367431315085E-06, 1.195255636818703571E-05, -0.9999999999265127837 ) ) ;
#7382=EDGE_CURVE ( 'NONE', #5194, #34163, #39085, .T. ) ;
#7388=DIRECTION ( 'NONE',  ( -0.5820088206811425691, 0.8131824719270214219, -7.019974882119856712E-08 ) ) ;
#7391=CARTESIAN_POINT ( 'NONE',  ( -20.25191534917341230, -8.350868906188830820, 70.26572394742477456 ) ) ;
#7392=FACE_OUTER_BOUND ( 'NONE', #38004, .T. ) ;
#7394=CARTESIAN_POINT ( 'NONE',  ( -17.15406633445637397, -7.764231093976030174, 70.78476080101584955 ) ) ;
#7396=LINE ( 'NONE', #41605, #41482 ) ;
#7397=CARTESIAN_POINT ( 'NONE',  ( -14.81662578951906184, -8.255127344917362109, 64.08978803669116076 ) ) ;
#7398=CARTESIAN_POINT ( 'NONE',  ( -12.81450638858427737, -9.474958432310776502, 74.46923006088778152 ) ) ;
#7400=ORIENTED_EDGE ( 'NONE', *, *, #47455, .F. ) ;
#7402=DIRECTION ( 'NONE',  ( -0.7171836970970658642, 0.6968841687240311389, -4.479616660400631173E-09 ) ) ;
#7404=CARTESIAN_POINT ( 'NONE',  ( -11.40851146197636012, -18.49244098807202974, 64.83887356883496977 ) ) ;
#7405=ORIENTED_EDGE ( 'NONE', *, *, #41247, .F. ) ;
#7406=CARTESIAN_POINT ( 'NONE',  ( -23.46260529264824157, -11.17067950781535579, 73.36193301757424479 ) ) ;
#7407=AXIS2_PLACEMENT_3D ( 'NONE', #1751, #16743, #31785 ) ;
#7408=FACE_OUTER_BOUND ( 'NONE', #21590, .T. ) ;
#7412=FACE_OUTER_BOUND ( 'NONE', #14050, .T. ) ;
#7413=ADVANCED_FACE ( 'NONE', ( #22683 ), #16909, .T. ) ;
#7414=LINE ( 'NONE', #41132, #21032 ) ;
#7415=CARTESIAN_POINT ( 'NONE',  ( -24.77723877343947478, -16.00713684962007122, 66.24820200538215431 ) ) ;
#7416=ORIENTED_EDGE ( 'NONE', *, *, #8575, .T. ) ;
#7418=ORIENTED_EDGE ( 'NONE', *, *, #5941, .F. ) ;
#7419=CARTESIAN_POINT ( 'NONE',  ( -10.44370662133100325, -17.41289724721067600, 64.76705995214548750 ) ) ;
#7420=CARTESIAN_POINT ( 'NONE',  ( -12.60227155074094441, -19.95281705956671559, 68.35129494334645983 ) ) ;
#7421=ORIENTED_EDGE ( 'NONE', *, *, #15124, .T. ) ;
#7422=DIRECTION ( 'NONE',  ( 8.766499717996234600E-07, 3.805972784084494839E-07, -0.9999999999995433653 ) ) ;
#7423=CARTESIAN_POINT ( 'NONE',  ( -20.12075396405374406, -21.75404021237947916, 72.50504483600978745 ) ) ;
#7425=CARTESIAN_POINT ( 'NONE',  ( -21.35693516282594828, -21.13669309701779397, 69.23262968960160890 ) ) ;
#7426=CARTESIAN_POINT ( 'NONE',  ( -10.05862351292959467, -15.92886012141397245, 64.69266982328383619 ) ) ;
#7427=DIRECTION ( 'NONE',  ( 0.9942595023566571655, -0.1069955231469582047, 3.800058679842194246E-08 ) ) ;
#7428=CARTESIAN_POINT ( 'NONE',  ( -16.61119863413175679, -21.81222516549900092, 65.52564366564290310 ) ) ;
#7429=ORIENTED_EDGE ( 'NONE', *, *, #19200, .T. ) ;
#7430=CARTESIAN_POINT ( 'NONE',  ( -12.24602769423020199, -10.02462455777539141, 60.85358326865326717 ) ) ;
#7431=LINE ( 'NONE', #17748, #45514 ) ;
#7433=CARTESIAN_POINT ( 'NONE',  ( -10.76785811675247118, -12.48515291162924434, 57.61385273545094066 ) ) ;
#7434=FACE_OUTER_BOUND ( 'NONE', #14137, .T. ) ;
#7435=B_SPLINE_CURVE_WITH_KNOTS ( 'NONE', 1,
 ( #31792, #17483 ),
 .UNSPECIFIED., .F., .F.,
 ( 2, 2 ),
 ( 0.000000000000000000, 1.000000000000000000 ),
 .UNSPECIFIED. ) ;
#7438=EDGE_CURVE ( 'NONE', #22280, #3333, #9307, .T. ) ;
#7440=ORIENTED_EDGE ( 'NONE', *, *, #33169, .F. ) ;
#7442=VERTEX_POINT ( 'NONE', #42794 ) ;
#7443=CARTESIAN_POINT ( 'NONE',  ( -14.70574402281689963, -21.31410033361279233, 58.16617881512491550 ) ) ;
#7444=DIRECTION ( 'NONE',  ( 0.5540494244615070674, -0.8324837747691378187, 8.494877338007802962E-17 ) ) ;
#7446=CARTESIAN_POINT ( 'NONE',  ( -15.68725519569583504, -21.64564087395307368, 72.25395315099507343 ) ) ;
#7447=CARTESIAN_POINT ( 'NONE',  ( -14.60635853056651001, -21.70587488938233278, 58.20971981907628390 ) ) ;
#7448=( BOUNDED_SURFACE ( )  B_SPLINE_SURFACE ( 3, 1, ( 
 ( #24198, #43152 ),
 ( #17513, #32542 ),
 ( #27881, #44141 ),
 ( #48523, #2976 ),
 ( #22194, #44856 ),
 ( #11112, #21473 ),
 ( #3465, #26133 ) ),
 .UNSPECIFIED., .T., .F., .F. ) 
 B_SPLINE_SURFACE_WITH_KNOTS ( ( 4, 3, 4 ),
 ( 2, 2 ),
 ( 0.000000000000000000, 0.5000000000000000000, 1.000000000000000000 ),
 ( 0.000000000000000000, 1.000000000000000000 ),
 .UNSPECIFIED. ) 
 GEOMETRIC_REPRESENTATION_ITEM ( )  RATIONAL_B_SPLINE_SURFACE ( (
 ( 1.000000000000000000, 1.000000000000000000),
 ( 0.3333333333333335369, 0.3333333333333330373),
 ( 0.3333333333333335369, 0.3333333333333330373),
 ( 1.000000000000000000, 1.000000000000000000),
 ( 0.3333333333333333703, 0.3333333333333333703),
 ( 0.3333333333333333703, 0.3333333333333333703),
 ( 1.000000000000000000, 1.000000000000000000) ) ) 
 REPRESENTATION_ITEM ( '' )  SURFACE ( )  );
#7449=FACE_BOUND ( 'NONE', #41795, .T. ) ;
#7450=CARTESIAN_POINT ( 'NONE',  ( -24.29522497960104843, -16.38737818751056352, 59.12332460191262840 ) ) ;
#7453=ADVANCED_FACE ( 'NONE', ( #20633 ), #287, .T. ) ;
#7455=CARTESIAN_POINT ( 'NONE',  ( -23.70135507383723805, -11.71146680393053607, 62.95218278684509983 ) ) ;
#7456=ORIENTED_EDGE ( 'NONE', *, *, #9354, .F. ) ;
#7458=CARTESIAN_POINT ( 'NONE',  ( -16.54004712951985923, -22.20656829664746468, 65.37564387897450047 ) ) ;
#7459=CARTESIAN_POINT ( 'NONE',  ( -10.88286923018596575, -17.43962093083235843, 68.11193994895104709 ) ) ;
#7463=CYLINDRICAL_SURFACE ( 'NONE', #35819, 0.1500000000000051015 ) ;
#7464=PLANE ( 'NONE',  #1730 ) ;
#7466=CARTESIAN_POINT ( 'NONE',  ( -23.78758865751629514, -10.93498413477609255, 73.40547355347567304 ) ) ;
#7467=( BOUNDED_CURVE ( )  B_SPLINE_CURVE ( 3, ( #42623, #46306, #38666, #12562 ),
 .UNSPECIFIED., .F., .F. ) 
 B_SPLINE_CURVE_WITH_KNOTS ( ( 4, 4 ),
 ( 1.570796326794896558, 1.780235837034217505 ),
 .UNSPECIFIED. ) 
 CURVE ( )  GEOMETRIC_REPRESENTATION_ITEM ( )  RATIONAL_B_SPLINE_CURVE ( ( 1.000000000000000000, 0.9963479302455154896, 0.9963479302455154896, 1.000000000000000000 ) ) 
 REPRESENTATION_ITEM ( '' )  );
#7468=VERTEX_POINT ( 'NONE', #26620 ) ;
#7469=ORIENTED_EDGE ( 'NONE', *, *, #18299, .F. ) ;
#7472=B_SPLINE_CURVE_WITH_KNOTS ( 'NONE', 3,
 ( #36878, #25339, #3165, #48458, #6625, #33185, #21642, #29763, #48220, #44793 ),
 .UNSPECIFIED., .F., .F.,
 ( 4, 2, 2, 2, 4 ),
 ( 0.1272669073658833083, 0.2522669073488315039, 0.3772669073317797550, 0.5022669073147280061, 0.6272669072976762017 ),
 .UNSPECIFIED. ) ;
#7473=ADVANCED_FACE ( 'NONE', ( #24326 ), #23846, .T. ) ;
#7476=CARTESIAN_POINT ( 'NONE',  ( -11.26648862653211935, -11.47983201339611981, 64.16384439635776005 ) ) ;
#7477=CARTESIAN_POINT ( 'NONE',  ( -21.36489679027069499, -8.963475500412677377, 73.60128753237400190 ) ) ;
#7478=ORIENTED_EDGE ( 'NONE', *, *, #45815, .T. ) ;
#7479=CARTESIAN_POINT ( 'NONE',  ( -23.12535539932854078, -10.01343808792704237, 66.65686846082743955 ) ) ;
#7480=DIRECTION ( 'NONE',  ( -5.731567514496413899E-31, -1.020425574103664789E-16, -1.000000000000000000 ) ) ;
#7481=ORIENTED_EDGE ( 'NONE', *, *, #47868, .T. ) ;
#7482=CARTESIAN_POINT ( 'NONE',  ( -10.37181755932410532, -14.66692344988656238, 75.09779103571921155 ) ) ;
#7483=CARTESIAN_POINT ( 'NONE',  ( -23.97105468032384579, -17.28687603139987772, 69.71339789080803939 ) ) ;
#7485=ORIENTED_EDGE ( 'NONE', *, *, #19500, .T. ) ;
#7486=CARTESIAN_POINT ( 'NONE',  ( -22.53429313110963506, -9.952421254863264011, 73.78161091678163075 ) ) ;
#7487=DIRECTION ( 'NONE',  ( 7.340779720199402358E-07, -8.195271891664201640E-07, 0.9999999999993947064 ) ) ;
#7488=CARTESIAN_POINT ( 'NONE',  ( -23.16791676868475491, -10.71612278230448823, 60.01692287334890352 ) ) ;
#7489=ORIENTED_EDGE ( 'NONE', *, *, #26517, .T. ) ;
#7490=CARTESIAN_POINT ( 'NONE',  ( -10.89650306282988090, -11.21840595405411101, 64.34156176843734443 ) ) ;
#7492=LINE ( 'NONE', #22492, #46213 ) ;
#7493=ADVANCED_FACE ( 'NONE', ( #12504 ), #1667, .F. ) ;
#7495=VERTEX_POINT ( 'NONE', #16177 ) ;
#7496=CARTESIAN_POINT ( 'NONE',  ( -10.85811841353450369, -12.22020323829153554, 74.71407760726656022 ) ) ;
#7499=CARTESIAN_POINT ( 'NONE',  ( -11.42587710518540334, -11.10406226247761019, 57.49431069621225276 ) ) ;
#7502=EDGE_LOOP ( 'NONE', ( #45119, #18041, #33546, #34238, #47057 ) ) ;
#7503=CARTESIAN_POINT ( 'NONE',  ( -17.77921064978749044, -22.25082400685520057, 58.59048811498988840 ) ) ;
#7504=CARTESIAN_POINT ( 'NONE',  ( -14.41828383943595959, -8.428772226827717873, 63.67490250008367525 ) ) ;
#7506=CARTESIAN_POINT ( 'NONE',  ( -11.32985570452711777, -19.09447181111026381, 68.32351299657294419 ) ) ;
#7508=LINE ( 'NONE', #7005, #27461 ) ;
#7510=CARTESIAN_POINT ( 'NONE',  ( -10.69617340855713827, -12.87194068125527302, 67.81002665770238025 ) ) ;
#7511=ORIENTED_EDGE ( 'NONE', *, *, #10767, .F. ) ;
#7513=EDGE_CURVE ( 'NONE', #20304, #12385, #14008, .T. ) ;
#7515=CARTESIAN_POINT ( 'NONE',  ( -11.03149232240643052, -10.98320184173030256, 60.93531726291125494 ) ) ;
#7516=LINE ( 'NONE', #3812, #27534 ) ;
#7517=B_SPLINE_CURVE_WITH_KNOTS ( 'NONE', 3,
 ( #7982, #27394, #4754, #22997, #37985, #15320, #46114, #45651, #7490, #30138 ),
 .UNSPECIFIED., .F., .F.,
 ( 4, 2, 2, 2, 4 ),
 ( 0.1272669073658008188, 0.2522669073439062215, 0.3772669073220116243, 0.5022669073001170270, 0.6272669072782224298 ),
 .UNSPECIFIED. ) ;
#7518=CARTESIAN_POINT ( 'NONE',  ( -10.76763519559319882, -17.13171766695033327, 61.15743118826002700 ) ) ;
#7520=ORIENTED_EDGE ( 'NONE', *, *, #47557, .F. ) ;
#7521=AXIS2_PLACEMENT_3D ( 'NONE', #12935, #5578, #2822 ) ;
#7525=CARTESIAN_POINT ( 'NONE',  ( -9.534148923395315833, -8.271570107951246698, 53.49999999999995026 ) ) ;
#7533=EDGE_LOOP ( 'NONE', ( #48591, #18366, #42982, #12694, #10875 ) ) ;
#7534=CARTESIAN_POINT ( 'NONE',  ( -12.58579432961061606, -9.143940464819721115, 74.44206132019799327 ) ) ;
#7535=CARTESIAN_POINT ( 'NONE',  ( -10.11541557277654313, -16.25427077284050270, 71.60896933323357416 ) ) ;
#7539=CARTESIAN_POINT ( 'NONE',  ( -20.06975372951847447, -8.274133229585533655, 73.73568642813194174 ) ) ;
#7540=CARTESIAN_POINT ( 'NONE',  ( -15.32518304399999387, -21.95751765168108349, 72.16080051677664642 ) ) ;
#7541=EDGE_CURVE ( 'NONE', #42734, #43742, #3072, .T. ) ;
#7542=CARTESIAN_POINT ( 'NONE',  ( -13.13835185842056674, -9.211395881110181705, 67.37942811378734120 ) ) ;
#7543=CARTESIAN_POINT ( 'NONE',  ( -19.84608771793053705, -21.43027439227859077, 69.22922701166929471 ) ) ;
#7545=B_SPLINE_CURVE_WITH_KNOTS ( 'NONE', 3,
 ( #800, #30856, #6434, #21454, #5715, #17251, #10372, #13306, #32296, #36207 ),
 .UNSPECIFIED., .F., .F.,
 ( 4, 2, 2, 2, 4 ),
 ( 0.1272669073658491412, 0.2522669073463209566, 0.3772669073267927997, 0.5022669073072645318, 0.6272669072877363750 ),
 .UNSPECIFIED. ) ;
#7546=CARTESIAN_POINT ( 'NONE',  ( -22.71059208588729561, -10.14448404190931186, 70.02650598627910483 ) ) ;
#7547=DIRECTION ( 'NONE',  ( -0.9529680021988312655, 0.3030709269876716294, 3.918663088761644638E-08 ) ) ;
#7548=CARTESIAN_POINT ( 'NONE',  ( -12.57222285659330119, -19.85510226960975899, 64.86674893738813807 ) ) ;
#7549=AXIS2_PLACEMENT_3D ( 'NONE', #6652, #48016, #6416 ) ;
#7550=FACE_BOUND ( 'NONE', #46042, .T. ) ;
#7554=CARTESIAN_POINT ( 'NONE',  ( -13.06813783877040791, -9.265530354883376063, 67.66470656304637998 ) ) ;
#7555=DIRECTION ( 'NONE',  ( -2.200805985157658208E-07, -3.006001589187115340E-06, -0.9999999999954577445 ) ) ;
#7556=ORIENTED_EDGE ( 'NONE', *, *, #8949, .T. ) ;
#7557=CARTESIAN_POINT ( 'NONE',  ( -14.13242279744181573, -8.574497162196568212, 74.21426705364891063 ) ) ;
#7558=ORIENTED_EDGE ( 'NONE', *, *, #17524, .T. ) ;
#7559=CARTESIAN_POINT ( 'NONE',  ( -17.81466184404888509, -7.769993126244952641, 60.08060774817733574 ) ) ;
#7560=FACE_OUTER_BOUND ( 'NONE', #16673, .T. ) ;
#7561=CARTESIAN_POINT ( 'NONE',  ( -21.61180957605408537, -8.647524312981719419, 73.70854620271380497 ) ) ;
#7563=CARTESIAN_POINT ( 'NONE',  ( -10.60286062419423914, -17.80505434777429841, 71.74530924410473176 ) ) ;
#7565=ORIENTED_EDGE ( 'NONE', *, *, #38303, .F. ) ;
#7567=ORIENTED_EDGE ( 'NONE', *, *, #48159, .F. ) ;
#7569=EDGE_CURVE ( 'NONE', #6936, #48202, #42676, .T. ) ;
#7570=FACE_OUTER_BOUND ( 'NONE', #16719, .T. ) ;
#7571=CARTESIAN_POINT ( 'NONE',  ( -21.15336808330806662, -20.73310000539657949, 69.35450185099439580 ) ) ;
#7572=EDGE_CURVE ( 'NONE', #946, #37616, #28888, .T. ) ;
#7573=CARTESIAN_POINT ( 'NONE',  ( -16.79181145072023185, -21.83380975027498039, 65.11075561446135396 ) ) ;
#7578=VERTEX_POINT ( 'NONE', #2863 ) ;
#7579=B_SPLINE_CURVE_WITH_KNOTS ( 'NONE', 3,
 ( #35519, #43160, #32074, #5746, #46621, #32325, #9434, #16303, #47349, #24459 ),
 .UNSPECIFIED., .F., .F.,
 ( 4, 2, 2, 2, 4 ),
 ( 0.6272669072877639085, 0.7522669073072798529, 0.8772669073267959083, 1.002266907346311964, 1.127266907365827908 ),
 .UNSPECIFIED. ) ;
#7580=EDGE_CURVE ( 'NONE', #5194, #40684, #47693, .T. ) ;
#7581=CARTESIAN_POINT ( 'NONE',  ( -16.19792114999740562, -7.866354181730329742, 60.48556343814865954 ) ) ;
#7582=CARTESIAN_POINT ( 'NONE',  ( -22.48430581236326731, -20.27711595259535571, 65.81926302645771898 ) ) ;
#7586=VERTEX_POINT ( 'NONE', #47936 ) ;
#7587=EDGE_CURVE ( 'NONE', #37103, #4167, #40064, .T. ) ;
#7588=( BOUNDED_CURVE ( )  B_SPLINE_CURVE ( 3, ( #2595, #14122, #29179, #1864 ),
 .UNSPECIFIED., .F., .F. ) 
 B_SPLINE_CURVE_WITH_KNOTS ( ( 4, 4 ),
 ( 0.4074455897393613468, 0.5000000000000000000 ),
 .UNSPECIFIED. ) 
 CURVE ( )  GEOMETRIC_REPRESENTATION_ITEM ( )  RATIONAL_B_SPLINE_CURVE ( ( 0.6983129098260874024, 0.7760317562606928732, 0.8765941196519969614, 0.9999999999999992228 ) ) 
 REPRESENTATION_ITEM ( '' )  );
#7590=VECTOR ( 'NONE', #22126, 1000.000000000000114 ) ;
#7593=PLANE ( 'NONE',  #36641 ) ;
#7595=CARTESIAN_POINT ( 'NONE',  ( -21.99178500617274779, -9.439039195359633538, 59.72171213140594404 ) ) ;
#7598=( BOUNDED_SURFACE ( )  B_SPLINE_SURFACE ( 3, 1, ( 
 ( #5378, #31469 ),
 ( #28010, #16186 ),
 ( #1911, #35398 ),
 ( #28264, #46014 ),
 ( #1676, #5136 ),
 ( #12267, #38856 ),
 ( #31714, #27290 ) ),
 .UNSPECIFIED., .T., .F., .F. ) 
 B_SPLINE_SURFACE_WITH_KNOTS ( ( 4, 3, 4 ),
 ( 2, 2 ),
 ( 0.000000000000000000, 0.5000000000000000000, 1.000000000000000000 ),
 ( 0.000000000000000000, 1.000000000000000000 ),
 .UNSPECIFIED. ) 
 GEOMETRIC_REPRESENTATION_ITEM ( )  RATIONAL_B_SPLINE_SURFACE ( (
 ( 1.000000000000000000, 1.000000000000000000),
 ( 0.3333333333333335369, 0.3333333333333330373),
 ( 0.3333333333333335369, 0.3333333333333330373),
 ( 1.000000000000000000, 1.000000000000000000),
 ( 0.3333333333333333703, 0.3333333333333333703),
 ( 0.3333333333333333703, 0.3333333333333333703),
 ( 1.000000000000000000, 1.000000000000000000) ) ) 
 REPRESENTATION_ITEM ( '' )  SURFACE ( )  );
#7599=ADVANCED_FACE ( 'NONE', ( #6331 ), #6081, .T. ) ;
#7600=CARTESIAN_POINT ( 'NONE',  ( -10.51729497052147977, -16.22293520194095606, 71.74750383215044280 ) ) ;
#7601=CARTESIAN_POINT ( 'NONE',  ( -21.53401928346354310, -9.142769119308555403, 66.85253116148227548 ) ) ;
#7602=ORIENTED_EDGE ( 'NONE', *, *, #32541, .T. ) ;
#7603=LINE ( 'NONE', #22606, #7698 ) ;
#7606=DIRECTION ( 'NONE',  ( -0.9501515917649785425, -0.3117883138709295898, 1.594035198720926202E-08 ) ) ;
#7607=VERTEX_POINT ( 'NONE', #43769 ) ;
#7608=CARTESIAN_POINT ( 'NONE',  ( -11.14069317138369719, -11.72368909046683072, 71.38860884459683120 ) ) ;
#7609=( BOUNDED_CURVE ( )  B_SPLINE_CURVE ( 3, ( #17302, #32352, #43679, #44895 ),
 .UNSPECIFIED., .F., .F. ) 
 B_SPLINE_CURVE_WITH_KNOTS ( ( 4, 4 ),
 ( 4.712388980384690562, 4.921828490624010399 ),
 .UNSPECIFIED. ) 
 CURVE ( )  GEOMETRIC_REPRESENTATION_ITEM ( )  RATIONAL_B_SPLINE_CURVE ( ( 1.000000000000000000, 0.9963479302455154896, 0.9963479302455154896, 1.000000000000000000 ) ) 
 REPRESENTATION_ITEM ( '' )  );
#7610=ORIENTED_EDGE ( 'NONE', *, *, #33760, .F. ) ;
#7612=CARTESIAN_POINT ( 'NONE',  ( -11.49187567532494114, -18.52825065318211983, 64.85780276779384224 ) ) ;
#7613=B_SPLINE_CURVE_WITH_KNOTS ( 'NONE', 3,
 ( #39856, #21633, #36389, #13730, #43809, #25330, #6373, #31989, #2669, #9831 ),
 .UNSPECIFIED., .F., .F.,
 ( 4, 2, 2, 2, 4 ),
 ( 0.000000000000000000, 0.2500000000000000000, 0.5000000000000000000, 0.7500000000000000000, 1.000000000000000000 ),
 .UNSPECIFIED. ) ;
#7615=CARTESIAN_POINT ( 'NONE',  ( -13.38504989191835826, -9.021193483636507082, 67.52375889928833885 ) ) ;
#7616=CARTESIAN_POINT ( 'NONE',  ( -24.53780083649505173, -12.59584922708229904, 69.95738295622972203 ) ) ;
#7617=CARTESIAN_POINT ( 'NONE',  ( -20.20879974760366693, -8.386827295270064653, 70.25100337495888425 ) ) ;
#7618=EDGE_LOOP ( 'NONE', ( #13729, #47553 ) ) ;
#7619=CARTESIAN_POINT ( 'NONE',  ( -16.58751391467172098, -21.80939466075598077, 65.52564390317479592 ) ) ;
#7620=CARTESIAN_POINT ( 'NONE',  ( -22.20320197231171733, -19.92390356480266433, 66.00421731406686376 ) ) ;
#7621=DIRECTION ( 'NONE',  ( 0.6538427738826437796, 0.7566304428460743914, -5.916677973025938575E-08 ) ) ;
#7622=ORIENTED_EDGE ( 'NONE', *, *, #35174, .T. ) ;
#7623=EDGE_CURVE ( 'NONE', #16942, #5056, #17637, .T. ) ;
#7624=CARTESIAN_POINT ( 'NONE',  ( -14.99424598590282365, -8.191132179135481195, 56.84999999999990195 ) ) ;
#7625=VECTOR ( 'NONE', #15246, 999.9999999999998863 ) ;
#7627=CARTESIAN_POINT ( 'NONE',  ( -13.38462805196022920, -20.58720062598995426, 58.34650077712429095 ) ) ;
#7628=CARTESIAN_POINT ( 'NONE',  ( -16.99557573331350824, -4.388301432589208240, 54.58422952202461431 ) ) ;
#7631=CARTESIAN_POINT ( 'NONE',  ( -23.34553101626436700, -10.28815885117376716, 59.79477560945002779 ) ) ;
#7632=CARTESIAN_POINT ( 'NONE',  ( -10.70671044302858022, -11.58740612280508842, 71.19522567356285947 ) ) ;
#7634=CARTESIAN_POINT ( 'NONE',  ( -10.39679176622870038, -14.24023819782134481, 64.40275955115841100 ) ) ;
#7636=CARTESIAN_POINT ( 'NONE',  ( -24.44055745662519641, -14.11932379769929113, 73.13743607903229815 ) ) ;
#7637=FACE_OUTER_BOUND ( 'NONE', #16896, .T. ) ;
#7638=CARTESIAN_POINT ( 'NONE',  ( -23.83512934130040861, -17.76108582422602922, 66.08789927488301430 ) ) ;
#7640=VERTEX_POINT ( 'NONE', #14167 ) ;
#7642=CYLINDRICAL_SURFACE ( 'NONE', #29713, 0.1499999999999964140 ) ;
#7643=B_SPLINE_CURVE_WITH_KNOTS ( 'NONE', 1,
 ( #37065, #33605 ),
 .UNSPECIFIED., .F., .F.,
 ( 2, 2 ),
 ( 0.000000000000000000, 1.000000000000000000 ),
 .UNSPECIFIED. ) ;
#7645=CARTESIAN_POINT ( 'NONE',  ( -19.90432934692537614, -21.83431937171774706, 69.04987052938618319 ) ) ;
#7646=B_SPLINE_CURVE_WITH_KNOTS ( 'NONE', 3,
 ( #18360, #44741, #19108, #8278, #34352, #887, #638, #30933, #16614, #1116 ),
 .UNSPECIFIED., .F., .F.,
 ( 4, 2, 2, 2, 4 ),
 ( 0.000000000000000000, 0.2500000000000000000, 0.5000000000000000000, 0.7500000000000000000, 1.000000000000000000 ),
 .UNSPECIFIED. ) ;
#7647=VERTEX_POINT ( 'NONE', #33878 ) ;
#7648=EDGE_LOOP ( 'NONE', ( #14952, #28828 ) ) ;
#7651=CARTESIAN_POINT ( 'NONE',  ( -15.32518304399999387, -21.95751765168108349, 72.16080051677664642 ) ) ;
#7652=DIRECTION ( 'NONE',  ( 0.9893874368562772803, -0.1453014101478918851, 3.604276813338690116E-17 ) ) ;
#7653=ADVANCED_FACE ( 'NONE', ( #14643 ), #10997, .T. ) ;
#7654=VERTEX_POINT ( 'NONE', #45233 ) ;
#7655=EDGE_CURVE ( 'NONE', #28162, #2827, #7194, .T. ) ;
#7656=CARTESIAN_POINT ( 'NONE',  ( -20.72574062298286535, -8.580111251864035893, 59.84125250080548852 ) ) ;
#7657=AXIS2_PLACEMENT_3D ( 'NONE', #7822, #18617, #22092 ) ;
#7658=PLANE ( 'NONE',  #10763 ) ;
#7659=ADVANCED_FACE ( 'NONE', ( #8057 ), #19077, .T. ) ;
#7663=CARTESIAN_POINT ( 'NONE',  ( -17.50083907013572571, -21.86240119160683193, 58.49733361235234952 ) ) ;
#7664=CARTESIAN_POINT ( 'NONE',  ( -24.32132670238839012, -16.30692182044891325, 66.20758098450045281 ) ) ;
#7665=VERTEX_POINT ( 'NONE', #23065 ) ;
#7666=DIRECTION ( 'NONE',  ( -0.9930145540378109148, 0.1179919296777755394, 4.526730167978063816E-08 ) ) ;
#7667=ORIENTED_EDGE ( 'NONE', *, *, #17828, .T. ) ;
#7668=CARTESIAN_POINT ( 'NONE',  ( -23.82366785274684418, -10.99486113721019009, 73.47697904737684382 ) ) ;
#7669=CARTESIAN_POINT ( 'NONE',  ( -20.45862069896310231, -8.501076506802965227, 63.59656160843943695 ) ) ;
#7672=CARTESIAN_POINT ( 'NONE',  ( -20.14513467918862233, -21.74452124448403723, 72.50455117424338880 ) ) ;
#7676=CARTESIAN_POINT ( 'NONE',  ( -24.43113031232903865, -15.58634216689856800, 73.30303748141028564 ) ) ;
#7677=CARTESIAN_POINT ( 'NONE',  ( -15.09544287645192284, -21.46351977604527761, 65.10596681500476279 ) ) ;
#7679=CARTESIAN_POINT ( 'NONE',  ( -10.43687275975356599, -14.38543977226298587, 64.40306298683110242 ) ) ;
#7680=CARTESIAN_POINT ( 'NONE',  ( -10.00073915290244564, -14.17087342314384735, 64.57459177551746166 ) ) ;
#7682=CARTESIAN_POINT ( 'NONE',  ( -10.85841931818429629, -17.37798394237198707, 64.91267318220633342 ) ) ;
#7683=CARTESIAN_POINT ( 'NONE',  ( -10.39241571269986331, -17.41794234916963191, 47.99999999999994316 ) ) ;
#7684=CARTESIAN_POINT ( 'NONE',  ( -13.33151401730585306, -20.55006798877650454, 58.06122216312902395 ) ) ;
#7685=EDGE_CURVE ( 'NONE', #2617, #773, #15972, .T. ) ;
#7686=ORIENTED_EDGE ( 'NONE', *, *, #43580, .T. ) ;
#7687=ORIENTED_EDGE ( 'NONE', *, *, #15513, .F. ) ;
#7688=CARTESIAN_POINT ( 'NONE',  ( -16.83291263600079191, -21.78581067597523813, 72.35470271977608547 ) ) ;
#7691=CARTESIAN_POINT ( 'NONE',  ( -21.00380318978402627, -21.34292366101719196, 62.22975991904223747 ) ) ;
#7693=CARTESIAN_POINT ( 'NONE',  ( -11.61674064386953198, -18.71759577841732280, 65.03241660559515935 ) ) ;
#7694=CARTESIAN_POINT ( 'NONE',  ( -10.46596968387485305, -15.57428492597166780, 57.64080867646067219 ) ) ;
#7696=CARTESIAN_POINT ( 'NONE',  ( -10.79572441526863180, -11.40795732096215254, 67.80359905390240272 ) ) ;
#7698=VECTOR ( 'NONE', #33411, 1000.000000000000000 ) ;
#7699=CARTESIAN_POINT ( 'NONE',  ( -16.81376820967965457, -9.329655637006117885, 53.69233794759168887 ) ) ;
#7700=CARTESIAN_POINT ( 'NONE',  ( -24.39640304805111981, -15.43122313838688164, 73.19406873947340841 ) ) ;
#7703=CARTESIAN_POINT ( 'NONE',  ( -12.06147410079331195, -19.98082143093137830, 61.50404465172076840 ) ) ;
#7704=AXIS2_PLACEMENT_3D ( 'NONE', #30383, #22250, #33298 ) ;
#7706=CARTESIAN_POINT ( 'NONE',  ( -24.59706363142188934, -12.79617847886399140, 66.48742024426742603 ) ) ;
#7708=VECTOR ( 'NONE', #12869, 1000.000000000000114 ) ;
#7709=ORIENTED_EDGE ( 'NONE', *, *, #46210, .T. ) ;
#7710=ORIENTED_EDGE ( 'NONE', *, *, #11285, .T. ) ;
#7714=CARTESIAN_POINT ( 'NONE',  ( -11.23206301587313050, -11.54443178946509008, 64.33985160186854557 ) ) ;
#7717=CARTESIAN_POINT ( 'NONE',  ( -16.98991503782990975, -22.24662993548692214, 72.35038528954983406 ) ) ;
#7718=EDGE_LOOP ( 'NONE', ( #37718, #38382 ) ) ;
#7719=DIRECTION ( 'NONE',  ( 0.8788484374452872894, -0.3260506722428090920, -0.3483050145059486957 ) ) ;
#7723=CARTESIAN_POINT ( 'NONE',  ( -22.31982660061501633, -20.42496915584003148, 62.39585669079483665 ) ) ;
#7726=VECTOR ( 'NONE', #24446, 1000.000000000000000 ) ;
#7727=ORIENTED_EDGE ( 'NONE', *, *, #31153, .T. ) ;
#7728=ADVANCED_FACE ( 'NONE', ( #34118 ), #533, .T. ) ;
#7731=CARTESIAN_POINT ( 'NONE',  ( -21.00588228679873382, -20.88502978299158741, 69.46939052609951659 ) ) ;
#7732=CARTESIAN_POINT ( 'NONE',  ( -17.21423163961297220, -7.362113418316746483, 70.68374130334144922 ) ) ;
#7734=CARTESIAN_POINT ( 'NONE',  ( -10.59656512619885227, -13.05092609425065397, 68.02360230423870746 ) ) ;
#7737=( BOUNDED_CURVE ( )  B_SPLINE_CURVE ( 3, ( #35564, #5554, #38776, #34836 ),
 .UNSPECIFIED., .F., .F. ) 
 B_SPLINE_CURVE_WITH_KNOTS ( ( 4, 4 ),
 ( 0.9074455897393708392, 1.000000000000000000 ),
 .UNSPECIFIED. ) 
 CURVE ( )  GEOMETRIC_REPRESENTATION_ITEM ( )  RATIONAL_B_SPLINE_CURVE ( ( 0.6983129098261093848, 0.7760317562607123021, 0.8765941196520091738, 1.000000000000000000 ) ) 
 REPRESENTATION_ITEM ( '' )  );
#7738=CARTESIAN_POINT ( 'NONE',  ( -24.35831120643470982, -13.52022779156689936, 59.77756816219774549 ) ) ;
#7741=CARTESIAN_POINT ( 'NONE',  ( -11.02242957576233273, -11.85532881267382166, 74.57312195644870201 ) ) ;
#7742=DIRECTION ( 'NONE',  ( -1.078708504911322448E-05, -7.367657518828247499E-06, -0.9999999999146781393 ) ) ;
#7744=CARTESIAN_POINT ( 'NONE',  ( -10.77303304197945621, -12.62668734528506853, 61.09853568451838868 ) ) ;
#7745=FACE_OUTER_BOUND ( 'NONE', #7240, .T. ) ;
#7746=CARTESIAN_POINT ( 'NONE',  ( -23.93094852480032486, -11.18081511418321305, 70.01493868496932294 ) ) ;
#7750=ORIENTED_EDGE ( 'NONE', *, *, #32917, .F. ) ;
#7751=CARTESIAN_POINT ( 'NONE',  ( -17.73316510640421129, -22.25279988176325574, 58.60564575049652802 ) ) ;
#7752=CARTESIAN_POINT ( 'NONE',  ( -14.41428275390769365, -7.994163218335415877, 63.97474169571218283 ) ) ;
#7753=ORIENTED_EDGE ( 'NONE', *, *, #42902, .F. ) ;
#7754=CARTESIAN_POINT ( 'NONE',  ( -24.40658449907487793, -15.78251210865724907, 69.53307488410803217 ) ) ;
#7755=CARTESIAN_POINT ( 'NONE',  ( -24.47432067347917695, -14.77756146504815327, 59.52828185648635184 ) ) ;
#7757=CARTESIAN_POINT ( 'NONE',  ( -23.54928233522715075, -11.31107727082186720, 66.42214407614666527 ) ) ;
#7758=( BOUNDED_CURVE ( )  B_SPLINE_CURVE ( 3, ( #9366, #20689, #9617, #18178 ),
 .UNSPECIFIED., .F., .F. ) 
 B_SPLINE_CURVE_WITH_KNOTS ( ( 4, 4 ),
 ( 0.9074455897393697290, 1.000000000000000000 ),
 .UNSPECIFIED. ) 
 CURVE ( )  GEOMETRIC_REPRESENTATION_ITEM ( )  RATIONAL_B_SPLINE_CURVE ( ( 0.6983129098260870693, 0.7760317562606930952, 0.8765941196519974055, 1.000000000000000000 ) ) 
 REPRESENTATION_ITEM ( '' )  );
#7759=CARTESIAN_POINT ( 'NONE',  ( -10.45859239952313224, -15.89938452881993847, 64.79299464097340433 ) ) ;
#7760=CARTESIAN_POINT ( 'NONE',  ( -18.40708155023567016, -22.19419919850242806, 68.99231578116254582 ) ) ;
#7763=CARTESIAN_POINT ( 'NONE',  ( -11.32522400900782067, -11.27219014254736074, 60.96413645226084554 ) ) ;
#7765=DIRECTION ( 'NONE',  ( -0.9562635972186039890, 0.2925062950340274193, -4.666065131241666896E-08 ) ) ;
#7770=ORIENTED_EDGE ( 'NONE', *, *, #46963, .T. ) ;
#7772=CARTESIAN_POINT ( 'NONE',  ( -20.38226043987465630, -7.971587899251926679, 70.36605015394232510 ) ) ;
#7775=CARTESIAN_POINT ( 'NONE',  ( -23.14235562961970416, -18.93896739645850502, 59.09230457533665515 ) ) ;
#7777=CARTESIAN_POINT ( 'NONE',  ( -10.63004074901718532, -12.92571453866564646, 67.75304464120749515 ) ) ;
#7778=CARTESIAN_POINT ( 'NONE',  ( -18.77740661349481144, -7.941208124173705585, 67.12745024023926987 ) ) ;
#7779=CARTESIAN_POINT ( 'NONE',  ( -24.38756562526642213, -15.91227465074932290, 66.34852784166324113 ) ) ;
#7780=EDGE_LOOP ( 'NONE', ( #10691, #32985 ) ) ;
#7781=CARTESIAN_POINT ( 'NONE',  ( -24.87206580614764206, -14.63538509624143380, 62.86296487661732613 ) ) ;
#7782=ORIENTED_EDGE ( 'NONE', *, *, #34151, .F. ) ;
#7784=CARTESIAN_POINT ( 'NONE',  ( -12.58002213166789041, -9.148928514680237711, 74.43427606957253317 ) ) ;
#7785=CARTESIAN_POINT ( 'NONE',  ( -21.18000576974785787, -20.77541348745421246, 69.35450184739246993 ) ) ;
#7786=CARTESIAN_POINT ( 'NONE',  ( -12.52062984216016162, -9.200252406392841920, 74.44110225673207992 ) ) ;
#7787=DIRECTION ( 'NONE',  ( 0.06498076606345293271, 0.4424675129789839567, 0.8944271909999157444 ) ) ;
#7788=EDGE_CURVE ( 'NONE', #936, #30190, #42976, .T. ) ;
#7789=ORIENTED_EDGE ( 'NONE', *, *, #28832, .T. ) ;
#7790=CARTESIAN_POINT ( 'NONE',  ( -10.65715545825994681, -16.81507633650918976, 61.30175972107676330 ) ) ;
#7792=CARTESIAN_POINT ( 'NONE',  ( -24.42310453188136776, -14.68514332193893068, 62.71296481370961118 ) ) ;
#7793=EDGE_CURVE ( 'NONE', #36602, #33816, #5579, .T. ) ;
#7794=AXIS2_PLACEMENT_3D ( 'NONE', #2048, #24718, #5985 ) ;
#7795=CARTESIAN_POINT ( 'NONE',  ( -13.11946129443726861, -9.225960368241006293, 67.37942785707224402 ) ) ;
#7796=CYLINDRICAL_SURFACE ( 'NONE', #10331, 0.1499999999999986067 ) ;
#7798=CARTESIAN_POINT ( 'NONE',  ( -22.98834342787593243, -19.14440809158465839, 62.65407131744080260 ) ) ;
#7799=CARTESIAN_POINT ( 'NONE',  ( -18.17795515447646792, -21.82680332084924046, 72.42944048533317414 ) ) ;
#7802=CARTESIAN_POINT ( 'NONE',  ( -10.73717317386910608, -11.52448149694614443, 71.26673621149227245 ) ) ;
#7803=FACE_BOUND ( 'NONE', #14688, .T. ) ;
#7804=ORIENTED_EDGE ( 'NONE', *, *, #39962, .F. ) ;
#7805=CARTESIAN_POINT ( 'NONE',  ( -23.83043763270304538, -11.86620476845630279, 59.48235732590899261 ) ) ;
#7807=CARTESIAN_POINT ( 'NONE',  ( -23.27284462870851911, -18.74605969774991010, 66.10917289053097079 ) ) ;
#7808=CARTESIAN_POINT ( 'NONE',  ( -21.31115985637654120, -8.927249709250721921, 73.88656608925673197 ) ) ;
#7810=CARTESIAN_POINT ( 'NONE',  ( -10.13258914451759019, -16.33817228489381179, 71.63245656337019796 ) ) ;
#7815=CARTESIAN_POINT ( 'NONE',  ( -14.54391382047218784, -7.937654553327920581, 63.97634087063163122 ) ) ;
#7816=VERTEX_POINT ( 'NONE', #45726 ) ;
#7817=CARTESIAN_POINT ( 'NONE',  ( -11.01268028240570551, -17.61879301183672197, 68.28825229171054900 ) ) ;
#7820=ORIENTED_EDGE ( 'NONE', *, *, #33523, .F. ) ;
#7821=FACE_OUTER_BOUND ( 'NONE', #38897, .T. ) ;
#7822=CARTESIAN_POINT ( 'NONE',  ( -23.88415220289344276, -17.63235127459526908, 62.62360984996717406 ) ) ;
#7823=CARTESIAN_POINT ( 'NONE',  ( -13.93897074462874919, -20.93787812888889377, 68.74153005185598886 ) ) ;
#7824=CARTESIAN_POINT ( 'NONE',  ( -10.57110035550071103, -13.38215360593666325, 74.97817647590578360 ) ) ;
#7825=CARTESIAN_POINT ( 'NONE',  ( -10.38101357771169653, -17.23783955604091034, 61.35081420447383493 ) ) ;
#7826=CARTESIAN_POINT ( 'NONE',  ( -14.09914643654217947, -8.649277595337252933, 74.49954655170296292 ) ) ;
#7827=CARTESIAN_POINT ( 'NONE',  ( -19.32724462824635836, -8.072771342010748086, 60.26093028616645597 ) ) ;
#7828=ORIENTED_EDGE ( 'NONE', *, *, #44217, .T. ) ;
#7829=ORIENTED_EDGE ( 'NONE', *, *, #21502, .T. ) ;
#7832=DIRECTION ( 'NONE',  ( 0.3109111061729914471, 0.9504389954427826526, 3.354176643444177759E-08 ) ) ;
#7833=FACE_OUTER_BOUND ( 'NONE', #15759, .T. ) ;
#7834=EDGE_LOOP ( 'NONE', ( #23473, #10464, #35662, #36662 ) ) ;
#7835=EDGE_CURVE ( 'NONE', #10344, #20228, #23299, .T. ) ;
#7837=B_SPLINE_CURVE_WITH_KNOTS ( 'NONE', 1,
 ( #20669, #1943 ),
 .UNSPECIFIED., .F., .F.,
 ( 2, 2 ),
 ( 0.000000000000000000, 1.000000000000000000 ),
 .UNSPECIFIED. ) ;
#7838=VECTOR ( 'NONE', #39698, 1000.000000000000000 ) ;
#7840=CARTESIAN_POINT ( 'NONE',  ( -21.56447292742736721, -9.102906949739807629, 70.13692356594822286 ) ) ;
#7841=CARTESIAN_POINT ( 'NONE',  ( -10.60570718526854961, -17.81143598018131158, 71.68222757358374508 ) ) ;
#7842=CYLINDRICAL_SURFACE ( 'NONE', #36995, 0.1500000000000032696 ) ;
#7843=AXIS2_PLACEMENT_3D ( 'NONE', #45179, #25707, #11417 ) ;
#7845=CARTESIAN_POINT ( 'NONE',  ( -20.33883497535441975, -7.953047583504734064, 70.45089127635624493 ) ) ;
#7846=CARTESIAN_POINT ( 'NONE',  ( -14.66805042590366170, -8.374595077462174686, 60.42882391711909662 ) ) ;
#7849=ORIENTED_EDGE ( 'NONE', *, *, #16016, .T. ) ;
#7851=EDGE_CURVE ( 'NONE', #36492, #43726, #25929, .T. ) ;
#7852=CARTESIAN_POINT ( 'NONE',  ( -10.12265238338418705, -16.28962619459307604, 71.54776144607544097 ) ) ;
#7855=CARTESIAN_POINT ( 'NONE',  ( -10.51016334156404319, -15.90393143234257067, 64.79306193244994461 ) ) ;
#7856=ORIENTED_EDGE ( 'NONE', *, *, #18122, .T. ) ;
#7858=CARTESIAN_POINT ( 'NONE',  ( -24.74075702715665770, -16.21285080831185965, 62.77823949964436423 ) ) ;
#7859=ADVANCED_FACE ( 'NONE', ( #42011 ), #46436, .T. ) ;
#7862=FACE_OUTER_BOUND ( 'NONE', #28431, .T. ) ;
#7863=CARTESIAN_POINT ( 'NONE',  ( -12.57192052008188199, -9.689650089559323831, 57.18115496948411192 ) ) ;
#7864=VERTEX_POINT ( 'NONE', #46186 ) ;
#7865=CARTESIAN_POINT ( 'NONE',  ( -21.38192084656556702, -20.58297848677295150, 72.53948803543819679 ) ) ;
#7866=EDGE_CURVE ( 'NONE', #47823, #9916, #39282, .T. ) ;
#7869=ORIENTED_EDGE ( 'NONE', *, *, #48308, .F. ) ;
#7870=CARTESIAN_POINT ( 'NONE',  ( -24.72694767484942702, -16.28301260341204326, 62.70833288210281609 ) ) ;
#7871=CARTESIAN_POINT ( 'NONE',  ( -23.30443023073026509, -19.38357886444350342, 59.07748956515449379 ) ) ;
#7873=ORIENTED_EDGE ( 'NONE', *, *, #15376, .T. ) ;
#7874=PLANE ( 'NONE',  #8681 ) ;
#7875=CARTESIAN_POINT ( 'NONE',  ( -10.69992486892027372, -11.60142258341215360, 71.21048119115297936 ) ) ;
#7877=ORIENTED_EDGE ( 'NONE', *, *, #36498, .T. ) ;
#7880=CARTESIAN_POINT ( 'NONE',  ( -20.31796842471441522, -7.944138697998205600, 70.29454436300783016 ) ) ;
#7881=( BOUNDED_CURVE ( )  B_SPLINE_CURVE ( 3, ( #18699, #38143, #37155, #30791 ),
 .UNSPECIFIED., .F., .F. ) 
 B_SPLINE_CURVE_WITH_KNOTS ( ( 4, 4 ),
 ( 0.5000000000000000000, 0.9074455897393671755 ),
 .UNSPECIFIED. ) 
 CURVE ( )  GEOMETRIC_REPRESENTATION_ITEM ( )  RATIONAL_B_SPLINE_CURVE ( ( 0.9999999999999786837, 0.4567392136813255288, 0.3561768502900427014, 0.6983129098261070533 ) ) 
 REPRESENTATION_ITEM ( '' )  );
#7882=CARTESIAN_POINT ( 'NONE',  ( -11.55573855159262386, -10.21941529800896653, 71.15388400389697665 ) ) ;
#7883=DIRECTION ( 'NONE',  ( 0.8083598999316397027, 0.5886886037477749856, 6.671815825018552065E-08 ) ) ;
#7884=CARTESIAN_POINT ( 'NONE',  ( -10.51729421260818498, -16.22293138110306998, 71.44750383217574097 ) ) ;
#7886=CARTESIAN_POINT ( 'NONE',  ( -12.52591642561268515, -9.195683996340104471, 74.50418400381258266 ) ) ;
#7888=CARTESIAN_POINT ( 'NONE',  ( -15.03427660820159772, -21.44211488324610571, 65.12068745241758450 ) ) ;
#7889=EDGE_CURVE ( 'NONE', #25586, #22230, #27710, .T. ) ;
#7891=ORIENTED_EDGE ( 'NONE', *, *, #42221, .F. ) ;
#7895=VECTOR ( 'NONE', #6673, 1000.000000000000000 ) ;
#7896=DIRECTION ( 'NONE',  ( -7.130145686836404013E-06, 1.088473443322539125E-05, 0.9999999999153418306 ) ) ;
#7902=DIRECTION ( 'NONE',  ( 0.8565259173193583431, -0.5161040137028850561, 6.301967848571307172E-08 ) ) ;
#7903=( BOUNDED_CURVE ( )  B_SPLINE_CURVE ( 3, ( #48675, #14921, #11259, #41289 ),
 .UNSPECIFIED., .F., .F. ) 
 B_SPLINE_CURVE_WITH_KNOTS ( ( 4, 4 ),
 ( 0.4074455897393655657, 0.5000000000000000000 ),
 .UNSPECIFIED. ) 
 CURVE ( )  GEOMETRIC_REPRESENTATION_ITEM ( )  RATIONAL_B_SPLINE_CURVE ( ( 0.6983129098261043888, 0.7760317562606969810, 0.8765941196519924095, 0.9999999999999825695 ) ) 
 REPRESENTATION_ITEM ( '' )  );
#7905=EDGE_LOOP ( 'NONE', ( #19932, #19808, #19258, #1310, #32469 ) ) ;
#7906=EDGE_CURVE ( 'NONE', #30992, #16763, #25682, .T. ) ;
#7907=CARTESIAN_POINT ( 'NONE',  ( -20.85096102773972504, -21.42427126083335764, 58.79475164009666344 ) ) ;
#7910=CARTESIAN_POINT ( 'NONE',  ( -10.86812120810698801, -17.26293121805600705, 64.92739382021848371 ) ) ;
#7912=CARTESIAN_POINT ( 'NONE',  ( -11.56806251476610115, -18.73522173559940995, 65.03234934376791898 ) ) ;
#7916=CARTESIAN_POINT ( 'NONE',  ( -11.10300763040008398, -10.86615618544839457, 57.39398486019972268 ) ) ;
#7917=ORIENTED_EDGE ( 'NONE', *, *, #42007, .F. ) ;
#7919=CARTESIAN_POINT ( 'NONE',  ( -10.40852245472632198, -14.07667478671615591, 64.68803976623010499 ) ) ;
#7921=CYLINDRICAL_SURFACE ( 'NONE', #5576, 0.1499999999999987454 ) ;
#7924=CARTESIAN_POINT ( 'NONE',  ( -23.00442008925061188, -19.11762375203660724, 59.18410642057862248 ) ) ;
#7926=ORIENTED_EDGE ( 'NONE', *, *, #7587, .F. ) ;
#7927=CARTESIAN_POINT ( 'NONE',  ( -23.89200480383413350, -11.11192299349349533, 70.07706151945906470 ) ) ;
#7929=CARTESIAN_POINT ( 'NONE',  ( -22.34687024958758172, -20.40107231831204970, 62.33464913462860579 ) ) ;
#7932=EDGE_LOOP ( 'NONE', ( #1770, #41077, #44996, #9290, #13060 ) ) ;
#7933=ORIENTED_EDGE ( 'NONE', *, *, #17579, .F. ) ;
#7935=CARTESIAN_POINT ( 'NONE',  ( -18.49053343615340239, -7.435173160506244550, 73.95409006490955051 ) ) ;
#7936=FACE_OUTER_BOUND ( 'NONE', #15900, .T. ) ;
#7937=ORIENTED_EDGE ( 'NONE', *, *, #14758, .F. ) ;
#7938=CARTESIAN_POINT ( 'NONE',  ( -17.00708550189658652, -7.821638742870105965, 73.96018273346899718 ) ) ;
#7939=CARTESIAN_POINT ( 'NONE',  ( -16.37589109965827561, -22.18522525038468984, 61.93284991378958892 ) ) ;
#7941=CARTESIAN_POINT ( 'NONE',  ( -10.46772245883852115, -15.58952514204506556, 57.75896008322165187 ) ) ;
#7943=DIRECTION ( 'NONE',  ( -0.8875028193683940358, -0.4608022847308269609, 4.020963237607658939E-08 ) ) ;
#7950=ADVANCED_FACE ( 'NONE', ( #28679 ), #11894, .T. ) ;
#7951=CARTESIAN_POINT ( 'NONE',  ( -14.42683414290149813, -8.428067600363897682, 67.25975083869262505 ) ) ;
#7952=AXIS2_PLACEMENT_3D ( 'NONE', #23817, #24547, #38818 ) ;
#7955=CARTESIAN_POINT ( 'NONE',  ( -24.61562913124599916, -12.86357381044341430, 66.55892682786348757 ) ) ;
#7957=VERTEX_POINT ( 'NONE', #32839 ) ;
#7958=ORIENTED_EDGE ( 'NONE', *, *, #10371, .F. ) ;
#7960=ORIENTED_EDGE ( 'NONE', *, *, #30922, .F. ) ;
#7961=CARTESIAN_POINT ( 'NONE',  ( -11.49688049385021138, -18.62690763749001732, 64.76179218520604763 ) ) ;
#7962=CARTESIAN_POINT ( 'NONE',  ( -21.86436131997776755, -11.54087357708903916, 53.69233794759168887 ) ) ;
#7963=AXIS2_PLACEMENT_3D ( 'NONE', #40098, #43317, #20659 ) ;
#7964=B_SPLINE_CURVE_WITH_KNOTS ( 'NONE', 1,
 ( #43056, #31490 ),
 .UNSPECIFIED., .F., .F.,
 ( 2, 2 ),
 ( 0.000000000000000000, 1.000000000000000000 ),
 .UNSPECIFIED. ) ;
#7965=CARTESIAN_POINT ( 'NONE',  ( -13.70631952225474137, -20.74045397679160629, 65.28628931288089632 ) ) ;
#7966=CARTESIAN_POINT ( 'NONE',  ( -17.77754172124238963, -7.367517167730140315, 60.12414849856542531 ) ) ;
#7967=ORIENTED_EDGE ( 'NONE', *, *, #150, .F. ) ;
#7968=B_SPLINE_CURVE_WITH_KNOTS ( 'NONE', 1,
 ( #38864, #46974 ),
 .UNSPECIFIED., .F., .F.,
 ( 2, 2 ),
 ( 0.000000000000000000, 1.000000000000000000 ),
 .UNSPECIFIED. ) ;
#7969=AXIS2_PLACEMENT_3D ( 'NONE', #21647, #25106, #40126 ) ;
#7970=CARTESIAN_POINT ( 'NONE',  ( -16.02724774380223849, -7.491242405164911133, 63.78515641179975404 ) ) ;
#7972=VERTEX_POINT ( 'NONE', #47877 ) ;
#7975=CARTESIAN_POINT ( 'NONE',  ( -14.73375560093340120, -21.75656996136207866, 61.75105004614717785 ) ) ;
#7978=CARTESIAN_POINT ( 'NONE',  ( -15.11475081961187428, -8.199755259496424031, 57.07829799881444899 ) ) ;
#7979=ADVANCED_FACE ( 'NONE', ( #20811 ), #10221, .T. ) ;
#7981=VERTEX_POINT ( 'NONE', #17583 ) ;
#7982=CARTESIAN_POINT ( 'NONE',  ( -10.92750425249182022, -11.16255029878774252, 64.26386639478288032 ) ) ;
#7985=CARTESIAN_POINT ( 'NONE',  ( -16.15549277074025980, -7.924674425949475243, 63.68627727349057466 ) ) ;
#7986=CARTESIAN_POINT ( 'NONE',  ( -24.12651600458584511, -12.62191667979047160, 73.25697658996381278 ) ) ;
#7988=B_SPLINE_CURVE_WITH_KNOTS ( 'NONE', 3,
 ( #1865, #36068, #47651, #32156, #10236, #21066, #6536, #13165, #28214, #42988 ),
 .UNSPECIFIED., .F., .F.,
 ( 4, 2, 2, 2, 4 ),
 ( 0.000000000000000000, 0.2500000000000000000, 0.5000000000000000000, 0.7500000000000000000, 1.000000000000000000 ),
 .UNSPECIFIED. ) ;
#7989=LINE ( 'NONE', #34050, #19382 ) ;
#7991=CARTESIAN_POINT ( 'NONE',  ( -20.52841364755139963, -8.479414496750122154, 63.61121502499755564 ) ) ;
#7992=CARTESIAN_POINT ( 'NONE',  ( -20.81696265954430558, -20.93198702957875668, 62.11471400680572685 ) ) ;
#7993=CARTESIAN_POINT ( 'NONE',  ( -10.48723278405693016, -15.75052974003975770, 64.79155073336579562 ) ) ;
#7997=LINE ( 'NONE', #37502, #12529 ) ;
#8000=CARTESIAN_POINT ( 'NONE',  ( -10.45256745270239307, -15.43993597667916795, 57.86792809192976961 ) ) ;
#8001=CARTESIAN_POINT ( 'NONE',  ( -22.56581679224888504, -9.985589735435180359, 73.48720857917361116 ) ) ;
#8002=CARTESIAN_POINT ( 'NONE',  ( -10.81170448216924740, -12.36318809540519048, 57.34329390664808557 ) ) ;
#8003=ORIENTED_EDGE ( 'NONE', *, *, #22600, .F. ) ;
#8004=CARTESIAN_POINT ( 'NONE',  ( -14.74510888451587753, -8.287885092648833663, 60.61436521918190579 ) ) ;
#8006=DIRECTION ( 'NONE',  ( -0.3374354101627465297, -0.9413486835218387583, -1.423378189644413276E-08 ) ) ;
#8007=AXIS2_PLACEMENT_3D ( 'NONE', #15121, #42219, #18834 ) ;
#8008=CARTESIAN_POINT ( 'NONE',  ( -18.32857646159318676, -22.20418385865972155, 68.93019298464047040 ) ) ;
#8009=EDGE_CURVE ( 'NONE', #4181, #48314, #47159, .T. ) ;
#8010=EDGE_CURVE ( 'NONE', #32569, #21373, #47026, .T. ) ;
#8011=ORIENTED_EDGE ( 'NONE', *, *, #16142, .T. ) ;
#8013=VECTOR ( 'NONE', #12048, 1000.000000000000114 ) ;
#8015=CARTESIAN_POINT ( 'NONE',  ( -24.82475127085388422, -15.66597259679895693, 73.11808347143848152 ) ) ;
#8016=CARTESIAN_POINT ( 'NONE',  ( -14.03189736672541166, -8.176154092714252641, 70.90674531289162985 ) ) ;
#8017=CARTESIAN_POINT ( 'NONE',  ( -13.50459945683549279, -9.009416567501544293, 57.07853663195904659 ) ) ;
#8018=ORIENTED_EDGE ( 'NONE', *, *, #37471, .F. ) ;
#8019=ORIENTED_EDGE ( 'NONE', *, *, #47262, .T. ) ;
#8021=CARTESIAN_POINT ( 'NONE',  ( -12.06140467229625912, -20.05244645202335008, 54.27966884056654351 ) ) ;
#8023=CARTESIAN_POINT ( 'NONE',  ( -22.83095840648717711, -19.93459376977450859, 72.82895984417613988 ) ) ;
#8024=( BOUNDED_SURFACE ( )  B_SPLINE_SURFACE ( 3, 1, ( 
 ( #25423, #36962 ),
 ( #25186, #48299 ),
 ( #14062, #29110 ),
 ( #26154, #40205 ),
 ( #29850, #21721 ),
 ( #14534, #40918 ),
 ( #40433, #37446 ) ),
 .UNSPECIFIED., .T., .F., .F. ) 
 B_SPLINE_SURFACE_WITH_KNOTS ( ( 4, 3, 4 ),
 ( 2, 2 ),
 ( 0.000000000000000000, 0.5000000000000000000, 1.000000000000000000 ),
 ( 0.000000000000000000, 1.000000000000000000 ),
 .UNSPECIFIED. ) 
 GEOMETRIC_REPRESENTATION_ITEM ( )  RATIONAL_B_SPLINE_SURFACE ( (
 ( 1.000000000000000000, 1.000000000000000000),
 ( 0.3333333333333335369, 0.3333333333333330373),
 ( 0.3333333333333335369, 0.3333333333333330373),
 ( 1.000000000000000000, 1.000000000000000000),
 ( 0.3333333333333333703, 0.3333333333333333703),
 ( 0.3333333333333333703, 0.3333333333333333703),
 ( 1.000000000000000000, 1.000000000000000000) ) ) 
 REPRESENTATION_ITEM ( '' )  SURFACE ( )  );
#8026=B_SPLINE_CURVE_WITH_KNOTS ( 'NONE', 3,
 ( #24593, #44274, #21126, #5865 ),
 .UNSPECIFIED., .F., .F.,
 ( 4, 4 ),
 ( 0.7089964807430767513, 1.000000000000000000 ),
 .UNSPECIFIED. ) ;
#8027=CARTESIAN_POINT ( 'NONE',  ( -23.04402284766838349, -19.06632961612601918, 59.16938527523783620 ) ) ;
#8029=PLANE ( 'NONE',  #42715 ) ;
#8030=AXIS2_PLACEMENT_3D ( 'NONE', #16545, #24918, #31585 ) ;
#8032=CARTESIAN_POINT ( 'NONE',  ( -21.06702863216100496, -20.84540773593990792, 65.86981821684420879 ) ) ;
#8033=VERTEX_POINT ( 'NONE', #43714 ) ;
#8034=( BOUNDED_CURVE ( )  B_SPLINE_CURVE ( 3, ( #10874, #18491, #8173, #42637 ),
 .UNSPECIFIED., .F., .F. ) 
 B_SPLINE_CURVE_WITH_KNOTS ( ( 4, 4 ),
 ( 0.5000000000000000000, 0.9074455897393562953 ),
 .UNSPECIFIED. ) 
 CURVE ( )  GEOMETRIC_REPRESENTATION_ITEM ( )  RATIONAL_B_SPLINE_CURVE ( ( 1.000000000000025091, 0.4567392136813530623, 0.3561768502900203859, 0.6983129098260543177 ) ) 
 REPRESENTATION_ITEM ( '' )  );
#8038=CARTESIAN_POINT ( 'NONE',  ( -21.83505603848428933, -9.305730678460758298, 59.60682523891489382 ) ) ;
#8039=CARTESIAN_POINT ( 'NONE',  ( -9.974042462495141592, -14.85071659844522429, 74.95925431899817681 ) ) ;
#8040=CARTESIAN_POINT ( 'NONE',  ( -18.56294146299573100, -7.902357174719097266, 74.14064450187080979 ) ) ;
#8051=( BOUNDED_CURVE ( )  B_SPLINE_CURVE ( 3, ( #20907, #2899, #35664, #17914 ),
 .UNSPECIFIED., .F., .F. ) 
 B_SPLINE_CURVE_WITH_KNOTS ( ( 4, 4 ),
 ( 0.4074455897393648440, 0.5000000000000000000 ),
 .UNSPECIFIED. ) 
 CURVE ( )  GEOMETRIC_REPRESENTATION_ITEM ( )  RATIONAL_B_SPLINE_CURVE ( ( 0.6983129098260953960, 0.7760317562607079722, 0.8765941196520117273, 1.000000000000012212 ) ) 
 REPRESENTATION_ITEM ( '' )  );
#8052=FACE_BOUND ( 'NONE', #28784, .T. ) ;
#8054=ORIENTED_EDGE ( 'NONE', *, *, #4814, .T. ) ;
#8057=FACE_OUTER_BOUND ( 'NONE', #9022, .T. ) ;
#8061=CARTESIAN_POINT ( 'NONE',  ( -22.42006521943993391, -9.190894407991624604, 53.76227901944321985 ) ) ;
#8062=CARTESIAN_POINT ( 'NONE',  ( -22.88419684932020459, -10.42887832691348926, 63.37185995611467604 ) ) ;
#8066=ADVANCED_FACE ( 'NONE', ( #9968 ), #9738, .T. ) ;
#8067=VERTEX_POINT ( 'NONE', #6276 ) ;
#8068=EDGE_LOOP ( 'NONE', ( #19728, #36979, #41897, #27954, #38695 ) ) ;
#8070=CARTESIAN_POINT ( 'NONE',  ( -20.31413516131974362, -8.378470924821744603, 67.06632013881642251 ) ) ;
#8071=CARTESIAN_POINT ( 'NONE',  ( -15.74783386771837890, -7.961078896070159061, 70.62461975990308360 ) ) ;
#8072=PLANE ( 'NONE',  #15313 ) ;
#8074=CARTESIAN_POINT ( 'NONE',  ( -10.50811820331624524, -16.17810198025521728, 71.45310207454518547 ) ) ;
#8077=ADVANCED_FACE ( 'NONE', ( #24526 ), #5280, .T. ) ;
#8078=EDGE_CURVE ( 'NONE', #5029, #21537, #10312, .T. ) ;
#8079=EDGE_CURVE ( 'NONE', #14112, #6378, #18060, .T. ) ;
#8080=CARTESIAN_POINT ( 'NONE',  ( -24.84793640206982701, -14.18443463346696909, 69.83770693398628282 ) ) ;
#8081=CARTESIAN_POINT ( 'NONE',  ( -14.07539642552819359, -8.605278304397881328, 74.19954655214911554 ) ) ;
#8082=CARTESIAN_POINT ( 'NONE',  ( -23.66133370835450833, -18.88359203746988868, 69.40876704922922613 ) ) ;
#8083=EDGE_CURVE ( 'NONE', #43727, #25852, #34113, .T. ) ;
#8086=VERTEX_POINT ( 'NONE', #14349 ) ;
#8088=EDGE_CURVE ( 'NONE', #34579, #25977, #14720, .T. ) ;
#8089=CARTESIAN_POINT ( 'NONE',  ( -12.13424045023392139, -19.48172391048287011, 61.54111352175390692 ) ) ;
#8092=CARTESIAN_POINT ( 'NONE',  ( -10.42609550623400416, -14.63933595658813935, 67.93088217856531230 ) ) ;
#8093=CARTESIAN_POINT ( 'NONE',  ( -22.79669589439772537, -19.97039224088601372, 72.74426291965076530 ) ) ;
#8095=CARTESIAN_POINT ( 'NONE',  ( -10.61779597260244401, -12.95740878981562361, 71.50828843252445211 ) ) ;
#8096=CARTESIAN_POINT ( 'NONE',  ( -24.12651600458584511, -12.62191667979047338, 73.25697658996379857 ) ) ;
#8097=CARTESIAN_POINT ( 'NONE',  ( -19.33359430827714576, -8.018871227582772931, 63.73089477487069132 ) ) ;
#8098=ORIENTED_EDGE ( 'NONE', *, *, #16939, .F. ) ;
#8099=CARTESIAN_POINT ( 'NONE',  ( -16.02724774380223849, -7.491242405164911133, 63.78515641179975404 ) ) ;
#8101=CARTESIAN_POINT ( 'NONE',  ( -10.18401476999287425, -13.05278034840643286, 71.32333300961973066 ) ) ;
#8102=EDGE_LOOP ( 'NONE', ( #37352, #15853, #37088, #36769 ) ) ;
#8104=CARTESIAN_POINT ( 'NONE',  ( -10.99582178678916833, -11.91441492378913480, 74.85840195586327184 ) ) ;
#8105=CARTESIAN_POINT ( 'NONE',  ( -24.23114935566793804, -13.17655915171226866, 63.13264225663914431 ) ) ;
#8106=ORIENTED_EDGE ( 'NONE', *, *, #6947, .F. ) ;
#8108=EDGE_CURVE ( 'NONE', #27480, #5623, #7997, .T. ) ;
#8109=FACE_OUTER_BOUND ( 'NONE', #38678, .T. ) ;
#8110=CARTESIAN_POINT ( 'NONE',  ( -11.43159037681183321, -11.19109104294698298, 57.43576446439195848 ) ) ;
#8111=ORIENTED_EDGE ( 'NONE', *, *, #29597, .T. ) ;
#8112=CARTESIAN_POINT ( 'NONE',  ( -12.26841837488882092, -9.996323195260892192, 56.97446934404248964 ) ) ;
#8118=CARTESIAN_POINT ( 'NONE',  ( -10.51737753838112610, -13.38018574993044219, 71.09339731095114701 ) ) ;
#8119=FACE_OUTER_BOUND ( 'NONE', #9412, .T. ) ;
#8120=( BOUNDED_CURVE ( )  B_SPLINE_CURVE ( 3, ( #31402, #39028, #30693, #8772 ),
 .UNSPECIFIED., .F., .F. ) 
 B_SPLINE_CURVE_WITH_KNOTS ( ( 4, 4 ),
 ( 0.000000000000000000, 0.4074455897393606807 ),
 .UNSPECIFIED. ) 
 CURVE ( )  GEOMETRIC_REPRESENTATION_ITEM ( )  RATIONAL_B_SPLINE_CURVE ( ( 1.000000000000000000, 0.4567392136813414050, 0.3561768502900338196, 0.6983129098260772993 ) ) 
 REPRESENTATION_ITEM ( '' )  );
#8122=CARTESIAN_POINT ( 'NONE',  ( -24.83498170362974022, -14.04605013716215822, 73.37917436033832530 ) ) ;
#8124=CARTESIAN_POINT ( 'NONE',  ( -9.975269291463440879, -14.95070888436857715, 74.95812242214459786 ) ) ;
#8125=ORIENTED_EDGE ( 'NONE', *, *, #34829, .F. ) ;
#8126=DIRECTION ( 'NONE',  ( 0.4182840851231336421, -0.9083162577718748576, 8.112345261759808545E-09 ) ) ;
#8127=( LENGTH_UNIT ( ) NAMED_UNIT ( * ) SI_UNIT ( .MILLI., .METRE. ) );
#8128=AXIS2_PLACEMENT_3D ( 'NONE', #20556, #39735, #35551 ) ;
#8129=ADVANCED_FACE ( 'NONE', ( #7260 ), #3047, .T. ) ;
#8130=CARTESIAN_POINT ( 'NONE',  ( -24.53556902878502655, -12.58855298716505366, 69.94959881007889635 ) ) ;
#8131=FACE_OUTER_BOUND ( 'NONE', #2099, .T. ) ;
#8132=ADVANCED_FACE ( 'NONE', ( #33817 ), #3540, .F. ) ;
#8133=ORIENTED_EDGE ( 'NONE', *, *, #2974, .T. ) ;
#8134=EDGE_CURVE ( 'NONE', #32577, #27062, #31771, .T. ) ;
#8136=DIRECTION ( 'NONE',  ( -0.8037372918934695409, 0.5949843406508663612, 7.322964617522835370E-08 ) ) ;
#8137=CARTESIAN_POINT ( 'NONE',  ( -12.84615363328625648, -20.17103110633857455, 72.09181604382622766 ) ) ;
#8138=CARTESIAN_POINT ( 'NONE',  ( -21.68042710870613732, -9.185287987594811909, 63.07665001108087921 ) ) ;
#8139=DIRECTION ( 'NONE',  ( -7.105595949593054157E-06, -6.912614924914188927E-07, 0.9999999999745162738 ) ) ;
#8140=ADVANCED_FACE ( 'NONE', ( #30153 ), #33571, .T. ) ;
#8141=ORIENTED_EDGE ( 'NONE', *, *, #45192, .T. ) ;
#8142=CARTESIAN_POINT ( 'NONE',  ( -20.84119746710918974, -20.97572115929791892, 62.11471400470772863 ) ) ;
#8143=CARTESIAN_POINT ( 'NONE',  ( -23.10710312199593730, -6.455677289120571594, 54.49999999999995026 ) ) ;
#8145=EDGE_LOOP ( 'NONE', ( #5454, #26803, #45626, #26115, #3120 ) ) ;
#8146=B_SPLINE_CURVE_WITH_KNOTS ( 'NONE', 3,
 ( #42718, #6253, #12898, #28421, #43446, #9715, #42947, #20300, #8981, #47382 ),
 .UNSPECIFIED., .F., .F.,
 ( 4, 2, 2, 2, 4 ),
 ( 0.000000000000000000, 0.2500000000000000000, 0.5000000000000000000, 0.7500000000000000000, 1.000000000000000000 ),
 .UNSPECIFIED. ) ;
#8147=DIRECTION ( 'NONE',  ( -0.3996021513128670266, -0.9166886716143755054, -9.834836654444679756E-09 ) ) ;
#8148=CARTESIAN_POINT ( 'NONE',  ( -13.91545454884148825, -8.237059506355153715, 74.45600559034086530 ) ) ;
#8149=ORIENTED_EDGE ( 'NONE', *, *, #48262, .F. ) ;
#8152=DIRECTION ( 'NONE',  ( 0.7224352045700188629, 0.6914386272098739239, -9.340627245513718311E-09 ) ) ;
#8153=DIRECTION ( 'NONE',  ( -0.9660698163281072892, -0.2582810677919976650, 5.363434502754641456E-08 ) ) ;
#8154=ORIENTED_EDGE ( 'NONE', *, *, #18400, .T. ) ;
#8155=CARTESIAN_POINT ( 'NONE',  ( -24.42850061278427987, -15.61005279108867860, 73.00303770028719441 ) ) ;
#8159=CARTESIAN_POINT ( 'NONE',  ( -17.64597121246115563, -21.80612736696262033, 58.42169971083756508 ) ) ;
#8160=( BOUNDED_SURFACE ( )  B_SPLINE_SURFACE ( 3, 1, ( 
 ( #4987, #20001 ),
 ( #6437, #25861 ),
 ( #18458, #36439 ),
 ( #2956, #32526 ),
 ( #22178, #25613 ),
 ( #29553, #2491 ),
 ( #21686, #10604 ) ),
 .UNSPECIFIED., .T., .F., .F. ) 
 B_SPLINE_SURFACE_WITH_KNOTS ( ( 4, 3, 4 ),
 ( 2, 2 ),
 ( 0.000000000000000000, 0.5000000000000000000, 1.000000000000000000 ),
 ( 0.000000000000000000, 1.000000000000000000 ),
 .UNSPECIFIED. ) 
 GEOMETRIC_REPRESENTATION_ITEM ( )  RATIONAL_B_SPLINE_SURFACE ( (
 ( 1.000000000000000000, 1.000000000000000000),
 ( 0.3333333333333335369, 0.3333333333333330373),
 ( 0.3333333333333335369, 0.3333333333333330373),
 ( 1.000000000000000000, 1.000000000000000000),
 ( 0.3333333333333333703, 0.3333333333333333703),
 ( 0.3333333333333333703, 0.3333333333333333703),
 ( 1.000000000000000000, 1.000000000000000000) ) ) 
 REPRESENTATION_ITEM ( '' )  SURFACE ( )  );
#8162=CARTESIAN_POINT ( 'NONE',  ( -19.17437844398820346, -7.979623566120205957, 63.44561363416070776 ) ) ;
#8163=CARTESIAN_POINT ( 'NONE',  ( -22.28468842640967651, -19.91619389767071269, 65.98949666203347419 ) ) ;
#8165=DIRECTION ( 'NONE',  ( 0.1648596854219665508, 0.9863170302304251624, -7.074492695212681195E-08 ) ) ;
#8168=CARTESIAN_POINT ( 'NONE',  ( -18.56951349870198342, -7.903555673074887267, 70.56171098378509043 ) ) ;
#8169=CARTESIAN_POINT ( 'NONE',  ( -22.78971111612053946, -9.640535285194584247, 73.64194477181111154 ) ) ;
#8171=VERTEX_POINT ( 'NONE', #27172 ) ;
#8172=CARTESIAN_POINT ( 'NONE',  ( -16.78411710364782650, -21.83009890335197767, 68.99560651669348488 ) ) ;
#8173=CARTESIAN_POINT ( 'NONE',  ( -17.69371375962564841, -21.85776310150506774, 62.17535971309806087 ) ) ;
#8174=VERTEX_POINT ( 'NONE', #35274 ) ;
#8175=CARTESIAN_POINT ( 'NONE',  ( -24.03794055889475345, -17.10236460774399703, 72.88336037747278340 ) ) ;
#8176=CARTESIAN_POINT ( 'NONE',  ( -16.34521610185216645, -22.18068367542918651, 61.85544494263961468 ) ) ;
#8179=CARTESIAN_POINT ( 'NONE',  ( -24.39996002416654264, -14.20937999902714743, 73.31198592523365676 ) ) ;
#8180=CARTESIAN_POINT ( 'NONE',  ( -10.76351158211370240, -11.46999907741044034, 67.73209273364366823 ) ) ;
#8181=( BOUNDED_CURVE ( )  B_SPLINE_CURVE ( 3, ( #48526, #14044, #7430, #10863 ),
 .UNSPECIFIED., .F., .F. ) 
 B_SPLINE_CURVE_WITH_KNOTS ( ( 4, 4 ),
 ( 0.9074455897393653991, 1.000000000000000000 ),
 .UNSPECIFIED. ) 
 CURVE ( )  GEOMETRIC_REPRESENTATION_ITEM ( )  RATIONAL_B_SPLINE_CURVE ( ( 0.6983129098260947298, 0.7760317562606996455, 0.8765941196520014023, 1.000000000000000000 ) ) 
 REPRESENTATION_ITEM ( '' )  );
#8182=CARTESIAN_POINT ( 'NONE',  ( -16.34629159056375514, -21.77648264143983781, 61.76127952027446355 ) ) ;
#8185=CARTESIAN_POINT ( 'NONE',  ( -14.46825175861997437, -8.408613495736075194, 67.26534847800355976 ) ) ;
#8186=EDGE_CURVE ( 'NONE', #47879, #1165, #6849, .T. ) ;
#8187=CARTESIAN_POINT ( 'NONE',  ( -19.58764298555839289, -21.52291637062162621, 69.23482530291350656 ) ) ;
#8188=CARTESIAN_POINT ( 'NONE',  ( -17.63137588941029676, -7.812166007189589756, 63.55057029281473291 ) ) ;
#8189=CARTESIAN_POINT ( 'NONE',  ( -12.71689659754714441, -19.99233245408618487, 71.99580697112106975 ) ) ;
#8192=ORIENTED_EDGE ( 'NONE', *, *, #20460, .F. ) ;
#8194=ADVANCED_FACE ( 'NONE', ( #23740 ), #46624, .F. ) ;
#8195=ORIENTED_EDGE ( 'NONE', *, *, #29857, .T. ) ;
#8196=FACE_OUTER_BOUND ( 'NONE', #28768, .T. ) ;
#8197=VECTOR ( 'NONE', #42374, 1000.000000000000000 ) ;
#8198=CARTESIAN_POINT ( 'NONE',  ( -10.42302287260171312, -13.97751933429587012, 57.73352905910142852 ) ) ;
#8199=EDGE_CURVE ( 'NONE', #2092, #11637, #45666, .T. ) ;
#8200=CARTESIAN_POINT ( 'NONE',  ( -17.42409385541300892, -14.80920654474439679, 56.49999999999994316 ) ) ;
#8202=CARTESIAN_POINT ( 'NONE',  ( -14.11063322135152909, -21.03236308526469855, 72.21135587486895702 ) ) ;
#8203=CARTESIAN_POINT ( 'NONE',  ( -10.68602809008750576, -16.88409676349039046, 57.70232650191087487 ) ) ;
#8204=EDGE_LOOP ( 'NONE', ( #2819, #45737 ) ) ;
#8206=EDGE_CURVE ( 'NONE', #44919, #29409, #33884, .T. ) ;
#8207=DIRECTION ( 'NONE',  ( 0.2737502900231349456, 0.9618007999124593699, -5.400150802740512045E-08 ) ) ;
#8209=EDGE_LOOP ( 'NONE', ( #16439, #43841 ) ) ;
#8211=CARTESIAN_POINT ( 'NONE',  ( -22.50287964365704241, -20.25976079877567670, 65.90432929200700585 ) ) ;
#8212=CARTESIAN_POINT ( 'NONE',  ( -17.15896312645611843, -7.363872641478732106, 70.68310009708541486 ) ) ;
#8214=ORIENTED_EDGE ( 'NONE', *, *, #22006, .F. ) ;
#8215=CARTESIAN_POINT ( 'NONE',  ( -24.27033112822875438, -13.12649005559073068, 63.13264177271826583 ) ) ;
#8216=EDGE_CURVE ( 'NONE', #1066, #28162, #45562, .T. ) ;
#8217=CARTESIAN_POINT ( 'NONE',  ( -16.07865488608826254, -7.939723797651444315, 63.67011030349581091 ) ) ;
#8218=CARTESIAN_POINT ( 'NONE',  ( -24.45125044792649049, -12.33277093510790579, 73.35570258362008644 ) ) ;
#8219=ORIENTED_EDGE ( 'NONE', *, *, #27467, .F. ) ;
#8221=CARTESIAN_POINT ( 'NONE',  ( -13.51885987070619954, -20.68321654889814099, 65.28629170358011891 ) ) ;
#8222=CARTESIAN_POINT ( 'NONE',  ( -13.53325622885376944, -21.16256470055228789, 65.17124264509627096 ) ) ;
#8223=DIRECTION ( 'NONE',  ( -5.731567514496413899E-31, -1.020425574103664789E-16, -1.000000000000000000 ) ) ;
#8225=( BOUNDED_SURFACE ( )  B_SPLINE_SURFACE ( 3, 1, ( 
 ( #8933, #9896 ),
 ( #28371, #1780 ),
 ( #20245, #28607 ),
 ( #46358, #1529 ),
 ( #16778, #43634 ),
 ( #32057, #35730 ),
 ( #42903, #2255 ) ),
 .UNSPECIFIED., .T., .F., .F. ) 
 B_SPLINE_SURFACE_WITH_KNOTS ( ( 4, 3, 4 ),
 ( 2, 2 ),
 ( 0.000000000000000000, 0.5000000000000000000, 1.000000000000000000 ),
 ( 0.000000000000000000, 1.000000000000000000 ),
 .UNSPECIFIED. ) 
 GEOMETRIC_REPRESENTATION_ITEM ( )  RATIONAL_B_SPLINE_SURFACE ( (
 ( 1.000000000000000000, 1.000000000000000000),
 ( 0.3333333333333335369, 0.3333333333333330373),
 ( 0.3333333333333335369, 0.3333333333333330373),
 ( 1.000000000000000000, 1.000000000000000000),
 ( 0.3333333333333333703, 0.3333333333333333703),
 ( 0.3333333333333333703, 0.3333333333333333703),
 ( 1.000000000000000000, 1.000000000000000000) ) ) 
 REPRESENTATION_ITEM ( '' )  SURFACE ( )  );
#8228=AXIS2_PLACEMENT_3D ( 'NONE', #15451, #8343, #37626 ) ;
#8231=CARTESIAN_POINT ( 'NONE',  ( -11.03586941931242826, -10.97581178645133093, 60.85698564304344416 ) ) ;
#8232=VERTEX_POINT ( 'NONE', #584 ) ;
#8233=FACE_OUTER_BOUND ( 'NONE', #41585, .T. ) ;
#8237=PLANE ( 'NONE',  #5858 ) ;
#8238=CARTESIAN_POINT ( 'NONE',  ( -16.93941734680483080, -7.775588144984237005, 74.24546186738449194 ) ) ;
#8239=CARTESIAN_POINT ( 'NONE',  ( -10.08052675126636721, -16.06451543208143917, 68.09272439531302723 ) ) ;
#8240=VERTEX_POINT ( 'NONE', #30642 ) ;
#8241=CARTESIAN_POINT ( 'NONE',  ( -18.52802763510036499, -22.17709038376527175, 72.40794071233227669 ) ) ;
#8242=CARTESIAN_POINT ( 'NONE',  ( -24.39137686751062617, -17.44764348928926623, 69.53622875020744232 ) ) ;
#8243=CARTESIAN_POINT ( 'NONE',  ( -10.38847021856859421, -14.31440148336201545, 60.80332504197532728 ) ) ;
#8244=FACE_OUTER_BOUND ( 'NONE', #15896, .T. ) ;
#8246=ORIENTED_EDGE ( 'NONE', *, *, #28982, .T. ) ;
#8247=EDGE_LOOP ( 'NONE', ( #22421, #5942 ) ) ;
#8249=ADVANCED_FACE ( 'NONE', ( #830 ), #19795, .T. ) ;
#8252=CARTESIAN_POINT ( 'NONE',  ( -20.38078961538757028, -7.970959937923086436, 70.50746246719650401 ) ) ;
#8255=CARTESIAN_POINT ( 'NONE',  ( -10.80190725398411011, -17.07816814126333327, 61.15743131804588728 ) ) ;
#8256=CARTESIAN_POINT ( 'NONE',  ( -21.00642299473589247, -8.276168789376990631, 60.02780591114678543 ) ) ;
#8257=CARTESIAN_POINT ( 'NONE',  ( -18.70000984002059852, -7.871953501822487098, 67.10891511697577982 ) ) ;
#8259=ORIENTED_EDGE ( 'NONE', *, *, #45635, .T. ) ;
#8260=PLANE ( 'NONE',  #40629 ) ;
#8262=ORIENTED_EDGE ( 'NONE', *, *, #37841, .T. ) ;
#8263=CARTESIAN_POINT ( 'NONE',  ( -19.14088062437382831, -4.707495580760234333, 53.49999999999995026 ) ) ;
#8264=CARTESIAN_POINT ( 'NONE',  ( -9.974795159103587494, -14.91206505565066109, 74.99767674250446703 ) ) ;
#8265=EDGE_CURVE ( 'NONE', #34680, #22085, #13006, .T. ) ;
#8266=FACE_OUTER_BOUND ( 'NONE', #45605, .T. ) ;
#8270=ORIENTED_EDGE ( 'NONE', *, *, #34978, .F. ) ;
#8271=CARTESIAN_POINT ( 'NONE',  ( -10.35661233123872371, -12.45241144375540365, 60.91358254413026430 ) ) ;
#8272=CARTESIAN_POINT ( 'NONE',  ( -20.87473523085085247, -8.206369618537406652, 60.01842129422883687 ) ) ;
#8273=VERTEX_POINT ( 'NONE', #39220 ) ;
#8274=CARTESIAN_POINT ( 'NONE',  ( -18.44528782684011503, -21.78515541812411982, 72.29983070759432451 ) ) ;
#8275=CARTESIAN_POINT ( 'NONE',  ( -17.72970361830877195, -22.25294841905989074, 58.50579124373946627 ) ) ;
#8276=CARTESIAN_POINT ( 'NONE',  ( -10.88941126017583905, -11.23118345116917460, 64.27069259981260529 ) ) ;
#8277=FACE_BOUND ( 'NONE', #31300, .T. ) ;
#8278=CARTESIAN_POINT ( 'NONE',  ( -22.15958588924365102, -19.96439345820419220, 62.30727227379612287 ) ) ;
#8279=CARTESIAN_POINT ( 'NONE',  ( -10.56627859465609376, -16.21290490039525167, 71.44750383612122846 ) ) ;
#8280=LINE ( 'NONE', #640, #5372 ) ;
#8281=CARTESIAN_POINT ( 'NONE',  ( -24.37542404773270022, -16.00605899042400537, 69.62487740803682357 ) ) ;
#8282=VERTEX_POINT ( 'NONE', #24929 ) ;
#8284=ORIENTED_EDGE ( 'NONE', *, *, #32978, .T. ) ;
#8285=CARTESIAN_POINT ( 'NONE',  ( -12.20772364030515611, -10.14112086625394049, 64.32914330961887117 ) ) ;
#8286=CARTESIAN_POINT ( 'NONE',  ( -12.36756753426621813, -9.896138138887707214, 57.37463480816234096 ) ) ;
#8287=VERTEX_POINT ( 'NONE', #17030 ) ;
#8288=AXIS2_PLACEMENT_3D ( 'NONE', #192, #29723, #30471 ) ;
#8289=CARTESIAN_POINT ( 'NONE',  ( -12.75184123886795717, -9.006184337177792543, 70.98892004851447268 ) ) ;
#8291=EDGE_CURVE ( 'NONE', #46544, #12446, #37070, .T. ) ;
#8293=EDGE_LOOP ( 'NONE', ( #3779, #41037 ) ) ;
#8294=ORIENTED_EDGE ( 'NONE', *, *, #10452, .F. ) ;
#8295=LINE ( 'NONE', #8788, #47734 ) ;
#8296=CARTESIAN_POINT ( 'NONE',  ( -19.44376929052122449, -7.638105555415076076, 60.07597592072836790 ) ) ;
#8297=CARTESIAN_POINT ( 'NONE',  ( -17.39742543611924575, -7.759256981132186759, 67.32039592192056432 ) ) ;
#8298=( BOUNDED_CURVE ( )  B_SPLINE_CURVE ( 3, ( #14311, #37208, #40925, #33768 ),
 .UNSPECIFIED., .F., .F. ) 
 B_SPLINE_CURVE_WITH_KNOTS ( ( 4, 4 ),
 ( 0.000000000000000000, 0.4074455897393644555 ),
 .UNSPECIFIED. ) 
 CURVE ( )  GEOMETRIC_REPRESENTATION_ITEM ( )  RATIONAL_B_SPLINE_CURVE ( ( 1.000000000000000000, 0.4567392136813305803, 0.3561768502900297673, 0.6983129098260976164 ) ) 
 REPRESENTATION_ITEM ( '' )  );
#8300=CARTESIAN_POINT ( 'NONE',  ( -10.43098718212803000, -15.70539730037032911, 61.32316937334011442 ) ) ;
#8302=EDGE_LOOP ( 'NONE', ( #1637, #16733 ) ) ;
#8305=EDGE_CURVE ( 'NONE', #25305, #17691, #17284, .T. ) ;
#8306=CARTESIAN_POINT ( 'NONE',  ( -9.990623107247818879, -14.31192343302863179, 64.57299167182827659 ) ) ;
#8307=CARTESIAN_POINT ( 'NONE',  ( -21.04590028053454631, -21.31959600062944205, 62.21447769906016845 ) ) ;
#8312=( BOUNDED_CURVE ( )  B_SPLINE_CURVE ( 3, ( #23651, #34947, #39130, #990 ),
 .UNSPECIFIED., .F., .F. ) 
 B_SPLINE_CURVE_WITH_KNOTS ( ( 4, 4 ),
 ( 4.712388980384689674, 4.921828490624010399 ),
 .UNSPECIFIED. ) 
 CURVE ( )  GEOMETRIC_REPRESENTATION_ITEM ( )  RATIONAL_B_SPLINE_CURVE ( ( 1.000000000000000000, 0.9963479302455154896, 0.9963479302455154896, 1.000000000000000000 ) ) 
 REPRESENTATION_ITEM ( '' )  );
#8313=ORIENTED_EDGE ( 'NONE', *, *, #18818, .T. ) ;
#8314=CARTESIAN_POINT ( 'NONE',  ( -24.70578670907444163, -13.23458007007709547, 59.51267921514076420 ) ) ;
#8315=CARTESIAN_POINT ( 'NONE',  ( -16.55933827844250672, -21.80960967909763681, 68.78740806194913660 ) ) ;
#8316=CYLINDRICAL_SURFACE ( 'NONE', #27605, 0.1500000000000052125 ) ;
#8317=ORIENTED_EDGE ( 'NONE', *, *, #32128, .F. ) ;
#8319=( BOUNDED_CURVE ( )  B_SPLINE_CURVE ( 3, ( #4627, #44012, #13447, #20855 ),
 .UNSPECIFIED., .F., .F. ) 
 B_SPLINE_CURVE_WITH_KNOTS ( ( 4, 4 ),
 ( 0.5000000000000000000, 0.9074455897393642889 ),
 .UNSPECIFIED. ) 
 CURVE ( )  GEOMETRIC_REPRESENTATION_ITEM ( )  RATIONAL_B_SPLINE_CURVE ( ( 1.000000000000025313, 0.4567392136813321901, 0.3561768502900123923, 0.6983129098260936196 ) ) 
 REPRESENTATION_ITEM ( '' )  );
#8321=CARTESIAN_POINT ( 'NONE',  ( -11.37476892658000160, -19.15884210479704208, 68.33034228280476441 ) ) ;
#8322=EDGE_CURVE ( 'NONE', #3873, #43420, #42095, .T. ) ;
#8324=CARTESIAN_POINT ( 'NONE',  ( -12.26841837488882092, -9.996323195260892192, 56.97446934404248964 ) ) ;
#8326=CARTESIAN_POINT ( 'NONE',  ( -10.43905175586412426, -15.29054565531327370, 57.75719864210760335 ) ) ;
#8327=CARTESIAN_POINT ( 'NONE',  ( -17.50157081909136991, -7.358860168393607459, 67.20694839074946003 ) ) ;
#8331=VERTEX_POINT ( 'NONE', #47815 ) ;
#8333=ADVANCED_FACE ( 'NONE', ( #32078 ), #38634, .T. ) ;
#8336=CARTESIAN_POINT ( 'NONE',  ( -16.29919166237813144, -22.17386956490665639, 62.01214078850637890 ) ) ;
#8339=CARTESIAN_POINT ( 'NONE',  ( -22.12520620670305860, -9.029593692166299590, 63.31436867790266376 ) ) ;
#8340=CARTESIAN_POINT ( 'NONE',  ( -16.27008067537174796, -7.904986561263926959, 60.50028479261354875 ) ) ;
#8341=DIRECTION ( 'NONE',  ( 9.009792911740839922E-08, -1.813722297350279449E-06, 0.9999999999983510968 ) ) ;
#8342=ORIENTED_EDGE ( 'NONE', *, *, #4644, .T. ) ;
#8343=DIRECTION ( 'NONE',  ( 0.9087012777736581670, -0.4174469879787381932, -4.853707507795077342E-09 ) ) ;
#8346=ORIENTED_EDGE ( 'NONE', *, *, #37354, .T. ) ;
#8348=CARTESIAN_POINT ( 'NONE',  ( -23.30282546666849086, -18.60927426030231047, 69.59371984657600763 ) ) ;
#8349=CARTESIAN_POINT ( 'NONE',  ( -10.70296955259081351, -11.59513340129999648, 71.27356289404251299 ) ) ;
#8350=CARTESIAN_POINT ( 'NONE',  ( -15.28291064399146038, -21.52618758091310980, 68.57592918174772478 ) ) ;
#8352=CARTESIAN_POINT ( 'NONE',  ( -24.45563843384471880, -14.25946414430215903, 73.53760260359439371 ) ) ;
#8353=CARTESIAN_POINT ( 'NONE',  ( -11.35824946695446691, -11.21643166988602047, 60.82885780703593070 ) ) ;
#8354=CARTESIAN_POINT ( 'NONE',  ( -18.58355647720519599, -7.449975798599677290, 74.04053169813657576 ) ) ;
#8355=CARTESIAN_POINT ( 'NONE',  ( -10.34288728022239923, -21.73268535153714254, 53.49999999999995026 ) ) ;
#8359=CARTESIAN_POINT ( 'NONE',  ( -14.41791765924166135, -21.19496194411871315, 58.31050579099508724 ) ) ;
#8360=CARTESIAN_POINT ( 'NONE',  ( -10.91670087826603464, -17.52156819001323740, 68.39721947804264346 ) ) ;
#8361=DIRECTION ( 'NONE',  ( 0.9325317756203296282, -0.3459670625490731677, -0.1033986416233826505 ) ) ;
#8362=ORIENTED_EDGE ( 'NONE', *, *, #23521, .F. ) ;
#8364=PLANE ( 'NONE',  #12308 ) ;
#8365=CARTESIAN_POINT ( 'NONE',  ( -19.60046948880987117, -21.46228020301366257, 65.76486213989072382 ) ) ;
#8367=CARTESIAN_POINT ( 'NONE',  ( -11.58245751978128268, -10.85571050334743859, 57.50903504724044524 ) ) ;
#8368=ORIENTED_EDGE ( 'NONE', *, *, #25971, .T. ) ;
#8370=CARTESIAN_POINT ( 'NONE',  ( -24.41553149706675896, -15.71832598455623398, 69.81835354388927328 ) ) ;
#8372=VERTEX_POINT ( 'NONE', #17756 ) ;
#8373=CARTESIAN_POINT ( 'NONE',  ( -12.88826169612582717, -20.14091212239222983, 72.09188343144306543 ) ) ;
#8374=CARTESIAN_POINT ( 'NONE',  ( -13.79242041809915875, -8.303469675591347965, 74.31299407998417905 ) ) ;
#8375=ORIENTED_EDGE ( 'NONE', *, *, #47773, .T. ) ;
#8376=CARTESIAN_POINT ( 'NONE',  ( -12.36019758273501701, -19.71856390219481980, 65.28163476484961336 ) ) ;
#8380=EDGE_CURVE ( 'NONE', #5475, #34362, #22241, .T. ) ;
#8381=PLANE ( 'NONE',  #27528 ) ;
#8382=CARTESIAN_POINT ( 'NONE',  ( -23.77312771997254615, -18.70709664074277612, 72.87872845841107505 ) ) ;
#8383=ORIENTED_EDGE ( 'NONE', *, *, #13802, .T. ) ;
#8384=CARTESIAN_POINT ( 'NONE',  ( -20.34937902005098920, -7.957549317960647350, 70.40100341510218129 ) ) ;
#8385=CARTESIAN_POINT ( 'NONE',  ( -18.64625997845222116, -21.76055708611507100, 68.97081679896227513 ) ) ;
#8386=EDGE_CURVE ( 'NONE', #14119, #39039, #38924, .T. ) ;
#8388=CARTESIAN_POINT ( 'NONE',  ( -21.35088739213495757, -21.14050036012818268, 69.21596729481782972 ) ) ;
#8389=( BOUNDED_SURFACE ( )  B_SPLINE_SURFACE ( 3, 1, ( 
 ( #37445, #2999 ),
 ( #22212, #44163 ),
 ( #40665, #44624 ),
 ( #14533, #29354 ),
 ( #32793, #47593 ),
 ( #10642, #18006 ),
 ( #6948, #6706 ) ),
 .UNSPECIFIED., .T., .F., .F. ) 
 B_SPLINE_SURFACE_WITH_KNOTS ( ( 4, 3, 4 ),
 ( 2, 2 ),
 ( 0.000000000000000000, 0.5000000000000000000, 1.000000000000000000 ),
 ( 0.000000000000000000, 1.000000000000000000 ),
 .UNSPECIFIED. ) 
 GEOMETRIC_REPRESENTATION_ITEM ( )  RATIONAL_B_SPLINE_SURFACE ( (
 ( 1.000000000000000000, 1.000000000000000000),
 ( 0.3333333333333335369, 0.3333333333333330373),
 ( 0.3333333333333335369, 0.3333333333333330373),
 ( 1.000000000000000000, 1.000000000000000000),
 ( 0.3333333333333333703, 0.3333333333333333703),
 ( 0.3333333333333333703, 0.3333333333333333703),
 ( 1.000000000000000000, 1.000000000000000000) ) ) 
 REPRESENTATION_ITEM ( '' )  SURFACE ( )  );
#8391=CARTESIAN_POINT ( 'NONE',  ( -19.30978178441422699, -7.601027468210772575, 63.61744607541091767 ) ) ;
#8393=ORIENTED_EDGE ( 'NONE', *, *, #48116, .T. ) ;
#8394=CARTESIAN_POINT ( 'NONE',  ( -24.47371109942907808, -14.90716652360855576, 59.25772288469824645 ) ) ;
#8396=CARTESIAN_POINT ( 'NONE',  ( -13.62949042321701398, -8.926946430974666669, 56.96967755885751217 ) ) ;
#8397=CARTESIAN_POINT ( 'NONE',  ( -18.44140615910215431, -21.73495079426802690, 69.04187996903171154 ) ) ;
#8398=CARTESIAN_POINT ( 'NONE',  ( -12.36019758273501701, -19.71856390219481980, 65.28163476484961336 ) ) ;
#8399=EDGE_LOOP ( 'NONE', ( #18707, #36073 ) ) ;
#8400=ORIENTED_EDGE ( 'NONE', *, *, #42193, .T. ) ;
#8401=FACE_OUTER_BOUND ( 'NONE', #41398, .T. ) ;
#8402=CARTESIAN_POINT ( 'NONE',  ( -24.30032249061147098, -16.12038754366300353, 62.59328623469320974 ) ) ;
#8403=EDGE_LOOP ( 'NONE', ( #16910, #27933 ) ) ;
#8405=CARTESIAN_POINT ( 'NONE',  ( -15.82259855879412846, -7.533287975791289171, 67.25511890406325222 ) ) ;
#8407=CARTESIAN_POINT ( 'NONE',  ( -22.11926001268504294, -9.024814352312150234, 63.30658345311071855 ) ) ;
#8408=CARTESIAN_POINT ( 'NONE',  ( -18.14707656476823772, -21.82566862371319871, 62.08355883028285405 ) ) ;
#8409=CARTESIAN_POINT ( 'NONE',  ( -15.84273041897837864, -7.988518076557024727, 70.72063026278281939 ) ) ;
#8410=CARTESIAN_POINT ( 'NONE',  ( -16.32745258320347759, -21.77369344365219561, 61.77040269689842944 ) ) ;
#8411=ORIENTED_EDGE ( 'NONE', *, *, #5615, .T. ) ;
#8413=B_SPLINE_CURVE_WITH_KNOTS ( 'NONE', 3,
 ( #3432, #6890, #3679, #11074, #17950, #18437, #21667, #37144, #29536, #29791 ),
 .UNSPECIFIED., .F., .F.,
 ( 4, 2, 2, 2, 4 ),
 ( 0.000000000000000000, 0.2500000000000000000, 0.5000000000000000000, 0.7500000000000000000, 1.000000000000000000 ),
 .UNSPECIFIED. ) ;
#8414=CARTESIAN_POINT ( 'NONE',  ( -19.74200936563729769, -21.46758226568296024, 68.94954551542706156 ) ) ;
#8416=CARTESIAN_POINT ( 'NONE',  ( -20.70232472158584969, -8.624289250480600799, 59.84125250310036392 ) ) ;
#8417=CARTESIAN_POINT ( 'NONE',  ( -15.96294338902451493, -7.962954265068761472, 67.42390783910214225 ) ) ;
#8418=ORIENTED_EDGE ( 'NONE', *, *, #33650, .T. ) ;
#8419=VECTOR ( 'NONE', #18, 999.9999999999998863 ) ;
#8420=ORIENTED_EDGE ( 'NONE', *, *, #31788, .T. ) ;
#8425=CARTESIAN_POINT ( 'NONE',  ( -11.77169535943213319, -10.59578862612641714, 74.73885051658085388 ) ) ;
#8427=EDGE_CURVE ( 'NONE', #18022, #4434, #44185, .T. ) ;
#8428=ORIENTED_EDGE ( 'NONE', *, *, #41946, .T. ) ;
#8429=DIRECTION ( 'NONE',  ( -0.3478314405900309048, -0.9375570856950864451, 0.000000000000000000 ) ) ;
#8430=CARTESIAN_POINT ( 'NONE',  ( -16.06904454444675778, -7.890656075740461795, 63.67011029959335389 ) ) ;
#8431=EDGE_LOOP ( 'NONE', ( #7135, #12321, #16287, #22248, #35584 ) ) ;
#8432=CARTESIAN_POINT ( 'NONE',  ( -20.88147576600584543, -8.209942340109883219, 60.02620652709861560 ) ) ;
#8433=CARTESIAN_POINT ( 'NONE',  ( -10.48085350821551742, -13.91959267249018950, 57.44825035245948186 ) ) ;
#8435=( BOUNDED_CURVE ( )  B_SPLINE_CURVE ( 3, ( #47980, #14216, #29271, #8096 ),
 .UNSPECIFIED., .F., .F. ) 
 B_SPLINE_CURVE_WITH_KNOTS ( ( 4, 4 ),
 ( 0.4074455897393700066, 0.5000000000000000000 ),
 .UNSPECIFIED. ) 
 CURVE ( )  GEOMETRIC_REPRESENTATION_ITEM ( )  RATIONAL_B_SPLINE_CURVE ( ( 0.6983129098261058321, 0.7760317562607081943, 0.8765941196520058432, 0.9999999999999983347 ) ) 
 REPRESENTATION_ITEM ( '' )  );
#8436=CARTESIAN_POINT ( 'NONE',  ( -11.30361347545239958, -11.41219030243732391, 64.14882039658046153 ) ) ;
#8437=VERTEX_POINT ( 'NONE', #14526 ) ;
#8440=VERTEX_POINT ( 'NONE', #3479 ) ;
#8441=CARTESIAN_POINT ( 'NONE',  ( -12.77926086925118554, -20.11284637564935807, 71.80653681455748938 ) ) ;
#8443=ADVANCED_FACE ( 'NONE', ( #6939 ), #16624, .T. ) ;
#8444=CARTESIAN_POINT ( 'NONE',  ( -15.25055861359784259, -21.51969010973779817, 72.34575615124376213 ) ) ;
#8445=CARTESIAN_POINT ( 'NONE',  ( -21.29994498387370427, -20.70774380606181708, 65.74020874375150925 ) ) ;
#8446=CARTESIAN_POINT ( 'NONE',  ( -24.37947880424689018, -14.01905714813458914, 73.12271482014924118 ) ) ;
#8447=CARTESIAN_POINT ( 'NONE',  ( -10.42334066387008029, -15.64104445138816146, 61.03789045260960222 ) ) ;
#8448=( BOUNDED_CURVE ( )  B_SPLINE_CURVE ( 3, ( #6570, #35199, #12795, #9118 ),
 .UNSPECIFIED., .F., .F. ) 
 B_SPLINE_CURVE_WITH_KNOTS ( ( 4, 4 ),
 ( 0.5000000000000000000, 0.9074455897393685078 ),
 .UNSPECIFIED. ) 
 CURVE ( )  GEOMETRIC_REPRESENTATION_ITEM ( )  RATIONAL_B_SPLINE_CURVE ( ( 1.000000000000005995, 0.4567392136813286929, 0.3561768502900247713, 0.6983129098261008361 ) ) 
 REPRESENTATION_ITEM ( '' )  );
#8454=CARTESIAN_POINT ( 'NONE',  ( -13.49409790474204840, -20.66256726344224504, 61.53118467422925164 ) ) ;
#8457=CARTESIAN_POINT ( 'NONE',  ( -21.78913961794832588, -8.771810275399618106, 70.24637145832762997 ) ) ;
#8458=CARTESIAN_POINT ( 'NONE',  ( -24.26085316502931377, -16.31268185143223093, 59.12332382745086079 ) ) ;
#8459=ORIENTED_EDGE ( 'NONE', *, *, #40614, .T. ) ;
#8461=CYLINDRICAL_SURFACE ( 'NONE', #43617, 0.1500000000000051847 ) ;
#8463=CARTESIAN_POINT ( 'NONE',  ( -12.71430834099865415, -19.98797453911052457, 68.63657440637429374 ) ) ;
#8464=CARTESIAN_POINT ( 'NONE',  ( -17.65006842549283306, -20.30456235612524196, 53.49999999999995026 ) ) ;
#8466=EDGE_LOOP ( 'NONE', ( #5217, #27514, #17967, #24117, #36220 ) ) ;
#8467=ADVANCED_FACE ( 'NONE', ( #37694 ), #28845, .T. ) ;
#8468=CARTESIAN_POINT ( 'NONE',  ( -10.37852926856506386, -14.47236211977926246, 71.41962671695536358 ) ) ;
#8469=CARTESIAN_POINT ( 'NONE',  ( -17.19980177718173309, -7.762775310937220397, 70.49035839668022163 ) ) ;
#8470=CARTESIAN_POINT ( 'NONE',  ( -24.00447786525511518, -11.31618815658438315, 66.62203293136848004 ) ) ;
#8472=CARTESIAN_POINT ( 'NONE',  ( -18.52866185626436746, -22.17699158182255559, 72.46323720911766486 ) ) ;
#8474=CARTESIAN_POINT ( 'NONE',  ( -23.98503169607928953, -17.39005800936845603, 66.22885190747201989 ) ) ;
#8475=B_SPLINE_CURVE_WITH_KNOTS ( 'NONE', 3,
 ( #4832, #42504, #1122, #16122, #43480, #24529, #13155, #32618, #43719, #2094 ),
 .UNSPECIFIED., .F., .F.,
 ( 4, 2, 2, 2, 4 ),
 ( 0.1272669073659042638, 0.2522669073487938673, 0.3772669073316834432, 0.5022669073145730190, 0.6272669072974625948 ),
 .UNSPECIFIED. ) ;
#8482=CARTESIAN_POINT ( 'NONE',  ( -23.37982836330400005, -11.13088026761028182, 73.64727903829775357 ) ) ;
#8483=LINE ( 'NONE', #30421, #11929 ) ;
#8484=EDGE_CURVE ( 'NONE', #43615, #21832, #21824, .T. ) ;
#8485=VECTOR ( 'NONE', #9331, 1000.000000000000114 ) ;
#8487=B_SPLINE_CURVE_WITH_KNOTS ( 'NONE', 1,
 ( #44300, #36869 ),
 .UNSPECIFIED., .F., .F.,
 ( 2, 2 ),
 ( 0.000000000000000000, 1.000000000000000000 ),
 .UNSPECIFIED. ) ;
#8489=CARTESIAN_POINT ( 'NONE',  ( -20.48833051011514073, -8.513735643284267240, 66.97031093069610108 ) ) ;
#8490=CARTESIAN_POINT ( 'NONE',  ( -20.32146343473794303, -8.373352561929221949, 73.86529255602565058 ) ) ;
#8492=CARTESIAN_POINT ( 'NONE',  ( -24.75383108144848165, -16.14659837148148824, 66.24980321609697853 ) ) ;
#8493=ORIENTED_EDGE ( 'NONE', *, *, #9347, .T. ) ;
#8494=CARTESIAN_POINT ( 'NONE',  ( -22.01092588021961660, -8.937695967300268052, 66.84805351483468883 ) ) ;
#8495=ADVANCED_FACE ( 'NONE', ( #8401 ), #27107, .T. ) ;
#8498=FACE_OUTER_BOUND ( 'NONE', #32042, .T. ) ;
#8499=CARTESIAN_POINT ( 'NONE',  ( -13.64083825785024295, -8.860125017712917384, 56.97527577494557249 ) ) ;
#8500=VERTEX_POINT ( 'NONE', #15770 ) ;
#8501=CARTESIAN_POINT ( 'NONE',  ( -18.14803087600414955, -22.22395683015660239, 65.54543360577268629 ) ) ;
#8503=CARTESIAN_POINT ( 'NONE',  ( -20.19053640067075506, -7.838066347919499854, 54.27966884056654351 ) ) ;
#8505=EDGE_LOOP ( 'NONE', ( #18843, #24171, #21513, #20822, #44751 ) ) ;
#8506=CARTESIAN_POINT ( 'NONE',  ( -21.68042710870613732, -9.185287987594811909, 63.07665001108087921 ) ) ;
#8508=CARTESIAN_POINT ( 'NONE',  ( -23.81024772113315890, -18.64597811008791695, 72.94863512192290500 ) ) ;
#8509=FACE_OUTER_BOUND ( 'NONE', #15654, .T. ) ;
#8511=ADVANCED_FACE ( 'NONE', ( #20203 ), #22954, .T. ) ;
#8512=CARTESIAN_POINT ( 'NONE',  ( -11.44474483503512197, -18.44890233052262829, 57.99817723587980112 ) ) ;
#8513=CARTESIAN_POINT ( 'NONE',  ( -18.34350352696802844, -21.80264126034385441, 65.55352047473381560 ) ) ;
#8514=EDGE_CURVE ( 'NONE', #12740, #11221, #3592, .T. ) ;
#8517=DIRECTION ( 'NONE',  ( 0.4599824152910792496, 0.8879280250239794947, 2.250728352126283681E-08 ) ) ;
#8518=ADVANCED_FACE ( 'NONE', ( #26634 ), #40493, .T. ) ;
#8520=VECTOR ( 'NONE', #36653, 1000.000000000000114 ) ;
#8521=DIRECTION ( 'NONE',  ( -1.075201462585828720E-05, 1.608194665399622665E-06, 0.9999999999409039386 ) ) ;
#8522=CARTESIAN_POINT ( 'NONE',  ( -13.25597978444290170, -9.183840967339035544, 67.45113130188182993 ) ) ;
#8524=CARTESIAN_POINT ( 'NONE',  ( -14.86627107493491984, -7.811969877679347363, 56.96504568426624360 ) ) ;
#8527=FACE_BOUND ( 'NONE', #9626, .T. ) ;
#8528=B_SPLINE_CURVE_WITH_KNOTS ( 'NONE', 3,
 ( #37847, #4857, #4138, #15416, #30484, #45498, #11756, #1142, #16147, #26778 ),
 .UNSPECIFIED., .F., .F.,
 ( 4, 2, 2, 2, 4 ),
 ( 0.000000000000000000, 0.2500000000000000000, 0.5000000000000000000, 0.7500000000000000000, 1.000000000000000000 ),
 .UNSPECIFIED. ) ;
#8530=VERTEX_POINT ( 'NONE', #11858 ) ;
#8533=LINE ( 'NONE', #34622, #21632 ) ;
#8534=CARTESIAN_POINT ( 'NONE',  ( -17.44579964618406009, -7.359071133328546566, 67.18186073236977052 ) ) ;
#8535=EDGE_CURVE ( 'NONE', #44852, #26302, #41895, .T. ) ;
#8536=CARTESIAN_POINT ( 'NONE',  ( -10.27391136003569905, -12.71670657087258327, 64.31190181376453552 ) ) ;
#8537=CARTESIAN_POINT ( 'NONE',  ( -12.52694624409642898, -20.42352324341258907, 72.00664875469250603 ) ) ;
#8539=ORIENTED_EDGE ( 'NONE', *, *, #47721, .T. ) ;
#8540=ORIENTED_EDGE ( 'NONE', *, *, #231, .F. ) ;
#8542=EDGE_CURVE ( 'NONE', #19435, #1693, #31053, .T. ) ;
#8543=EDGE_CURVE ( 'NONE', #30739, #11687, #33473, .T. ) ;
#8544=LINE ( 'NONE', #35360, #9479 ) ;
#8545=DIRECTION ( 'NONE',  ( 1.420801291081008049E-06, 1.008342286629444690E-05, -0.9999999999481530288 ) ) ;
#8547=EDGE_LOOP ( 'NONE', ( #14794, #1681, #31046, #40880, #48704 ) ) ;
#8550=CARTESIAN_POINT ( 'NONE',  ( -21.54665965586444543, -9.090157682337041578, 70.13132566468406992 ) ) ;
#8551=CARTESIAN_POINT ( 'NONE',  ( -15.37138615481495840, -21.50153415455971384, 68.86127572257412055 ) ) ;
#8553=CARTESIAN_POINT ( 'NONE',  ( -10.40277079310570052, -15.44444055846370745, 57.71792809063055785 ) ) ;
#8555=B_SPLINE_CURVE_WITH_KNOTS ( 'NONE', 3,
 ( #11476, #44493, #26017, #41034, #44994, #14898, #29222, #44258, #11241, #7065 ),
 .UNSPECIFIED., .F., .F.,
 ( 4, 2, 2, 2, 4 ),
 ( 0.000000000000000000, 0.2500000000000000000, 0.5000000000000000000, 0.7500000000000000000, 1.000000000000000000 ),
 .UNSPECIFIED. ) ;
#8558=AXIS2_PLACEMENT_3D ( 'NONE', #31842, #32792, #36247 ) ;
#8559=AXIS2_PLACEMENT_3D ( 'NONE', #41362, #3954, #30551 ) ;
#8560=CARTESIAN_POINT ( 'NONE',  ( -22.05250757621314150, -8.971161105938598723, 63.33007234022110055 ) ) ;
#8561=ADVANCED_FACE ( 'NONE', ( #16245 ), #34487, .T. ) ;
#8563=ORIENTED_EDGE ( 'NONE', *, *, #17663, .F. ) ;
#8565=CARTESIAN_POINT ( 'NONE',  ( -15.11195830621016256, -21.41632612911037370, 65.40596681519618016 ) ) ;
#8566=B_SPLINE_CURVE_WITH_KNOTS ( 'NONE', 3,
 ( #21232, #40186, #13092, #6458, #32322, #1791, #6209, #43412, #24693, #20512 ),
 .UNSPECIFIED., .F., .F.,
 ( 4, 2, 2, 2, 4 ),
 ( 0.000000000000000000, 0.2500000000000000000, 0.5000000000000000000, 0.7500000000000000000, 1.000000000000000000 ),
 .UNSPECIFIED. ) ;
#8567=FACE_OUTER_BOUND ( 'NONE', #16879, .T. ) ;
#8569=VERTEX_POINT ( 'NONE', #27597 ) ;
#8570=CARTESIAN_POINT ( 'NONE',  ( -10.44216256679811217, -13.77595636612621988, 61.06254307272654813 ) ) ;
#8571=VERTEX_POINT ( 'NONE', #23916 ) ;
#8572=CARTESIAN_POINT ( 'NONE',  ( -11.08846142298070880, -18.82290330472913098, 47.99999999999994316 ) ) ;
#8573=CARTESIAN_POINT ( 'NONE',  ( -11.79792992861738909, -18.97409303405279957, 71.98685885147807539 ) ) ;
#8574=ORIENTED_EDGE ( 'NONE', *, *, #23587, .F. ) ;
#8575=EDGE_CURVE ( 'NONE', #39260, #37877, #15018, .T. ) ;
#8576=FACE_OUTER_BOUND ( 'NONE', #11668, .T. ) ;
#8577=CARTESIAN_POINT ( 'NONE',  ( -24.22593759466564123, -12.94379566627669753, 70.18731784193515466 ) ) ;
#8581=CARTESIAN_POINT ( 'NONE',  ( -11.12219343327886811, -17.98741664779230121, 71.72285496256920112 ) ) ;
#8582=( BOUNDED_CURVE ( )  B_SPLINE_CURVE ( 3, ( #30578, #19234, #34236, #41891 ),
 .UNSPECIFIED., .F., .F. ) 
 B_SPLINE_CURVE_WITH_KNOTS ( ( 4, 4 ),
 ( 1.570796326794896780, 1.780235837034204183 ),
 .UNSPECIFIED. ) 
 CURVE ( )  GEOMETRIC_REPRESENTATION_ITEM ( )  RATIONAL_B_SPLINE_CURVE ( ( 1.000000000000000000, 0.9963479302455159337, 0.9963479302455159337, 1.000000000000000000 ) ) 
 REPRESENTATION_ITEM ( '' )  );
#8583=FACE_OUTER_BOUND ( 'NONE', #2196, .T. ) ;
#8585=CARTESIAN_POINT ( 'NONE',  ( -12.00450496360434727, -9.697323582995780455, 60.66643917381700390 ) ) ;
#8586=EDGE_LOOP ( 'NONE', ( #35722, #24033, #36198, #46208, #26997 ) ) ;
#8587=CARTESIAN_POINT ( 'NONE',  ( -10.63676228191995321, -11.73759119428953390, 74.65865931763289609 ) ) ;
#8588=CARTESIAN_POINT ( 'NONE',  ( -24.72694767484942702, -16.28301260341204326, 62.70833288210281609 ) ) ;
#8590=ORIENTED_EDGE ( 'NONE', *, *, #7438, .F. ) ;
#8591=CARTESIAN_POINT ( 'NONE',  ( -10.49233462046909793, -15.78425219969246562, 61.22892196979352519 ) ) ;
#8592=CARTESIAN_POINT ( 'NONE',  ( -10.57990114081760957, -13.11695186304741334, 71.22300718686659593 ) ) ;
#8593=VECTOR ( 'NONE', #35755, 1000.000000000000000 ) ;
#8594=CARTESIAN_POINT ( 'NONE',  ( -10.37739347266510670, -15.12138602804827414, 75.00598708744817600 ) ) ;
#8599=CARTESIAN_POINT ( 'NONE',  ( -19.77436091090941517, -21.87886160397694368, 65.64981624214608757 ) ) ;
#8601=VECTOR ( 'NONE', #30338, 1000.000000000000000 ) ;
#8603=ADVANCED_FACE ( 'NONE', ( #21183 ), #5916, .T. ) ;
#8604=CARTESIAN_POINT ( 'NONE',  ( -23.70711844648210942, -18.01498993332871734, 59.09558460557502713 ) ) ;
#8606=ORIENTED_EDGE ( 'NONE', *, *, #38145, .F. ) ;
#8607=CARTESIAN_POINT ( 'NONE',  ( -12.35277332135121675, -20.26681466537264242, 68.45162004874669037 ) ) ;
#8608=EDGE_CURVE ( 'NONE', #14812, #9213, #25827, .T. ) ;
#8609=EDGE_CURVE ( 'NONE', #23558, #24381, #19384, .T. ) ;
#8610=CARTESIAN_POINT ( 'NONE',  ( -13.65110163016468015, -21.23324793748626504, 68.57129851394472553 ) ) ;
#8613=CARTESIAN_POINT ( 'NONE',  ( -14.88240180108872934, -21.38896689746768587, 65.19776689114348756 ) ) ;
#8615=( BOUNDED_SURFACE ( )  B_SPLINE_SURFACE ( 3, 1, ( 
 ( #37245, #37991 ),
 ( #33547, #48592 ),
 ( #14826, #29896 ),
 ( #11409, #14260 ),
 ( #48024, #40390 ),
 ( #29310, #40619 ),
 ( #9220, #46652 ) ),
 .UNSPECIFIED., .T., .F., .F. ) 
 B_SPLINE_SURFACE_WITH_KNOTS ( ( 4, 3, 4 ),
 ( 2, 2 ),
 ( 0.000000000000000000, 0.5000000000000000000, 1.000000000000000000 ),
 ( 0.000000000000000000, 1.000000000000000000 ),
 .UNSPECIFIED. ) 
 GEOMETRIC_REPRESENTATION_ITEM ( )  RATIONAL_B_SPLINE_SURFACE ( (
 ( 1.000000000000000000, 1.000000000000000000),
 ( 0.3333333333333335369, 0.3333333333333330373),
 ( 0.3333333333333335369, 0.3333333333333330373),
 ( 1.000000000000000000, 1.000000000000000000),
 ( 0.3333333333333333703, 0.3333333333333333703),
 ( 0.3333333333333333703, 0.3333333333333333703),
 ( 1.000000000000000000, 1.000000000000000000) ) ) 
 REPRESENTATION_ITEM ( '' )  SURFACE ( )  );
#8616=ADVANCED_FACE ( 'NONE', ( #39887 ), #16735, .T. ) ;
#8618=VERTEX_POINT ( 'NONE', #43600 ) ;
#8619=DIRECTION ( 'NONE',  ( 0.9979768094191902028, 0.06357898915123888495, 3.501668460141639105E-17 ) ) ;
#8620=CARTESIAN_POINT ( 'NONE',  ( -23.42915847708036381, -11.11517115755410146, 73.64721174900437006 ) ) ;
#8621=CARTESIAN_POINT ( 'NONE',  ( -15.61430862894485649, -21.57127090070544639, 72.11863486128041245 ) ) ;
#8622=CARTESIAN_POINT ( 'NONE',  ( -23.34481640033245853, -18.63641755246779752, 69.59371984262205046 ) ) ;
#8623=ORIENTED_EDGE ( 'NONE', *, *, #40310, .T. ) ;
#8624=CARTESIAN_POINT ( 'NONE',  ( -20.82033344162761423, -20.98728273936873734, 62.11471416939660628 ) ) ;
#8627=ORIENTED_EDGE ( 'NONE', *, *, #35831, .F. ) ;
#8628=CARTESIAN_POINT ( 'NONE',  ( -22.04114742393716142, -9.481025248639417313, 59.73643293354757589 ) ) ;
#8629=CARTESIAN_POINT ( 'NONE',  ( -22.14599171854093740, -19.97736010173111509, 65.72038334521670322 ) ) ;
#8631=PLANE ( 'NONE',  #37741 ) ;
#8634=CARTESIAN_POINT ( 'NONE',  ( -14.07539661982785262, -8.605278201040592378, 74.34954655214895070 ) ) ;
#8636=VERTEX_POINT ( 'NONE', #20461 ) ;
#8637=CARTESIAN_POINT ( 'NONE',  ( -24.23636321612255173, -17.82529083293033167, 62.58865660992282898 ) ) ;
#8643=CARTESIAN_POINT ( 'NONE',  ( -15.10203878652056630, -21.46900354431040725, 61.52111843893123933 ) ) ;
#8644=VERTEX_POINT ( 'NONE', #1974 ) ;
#8645=CARTESIAN_POINT ( 'NONE',  ( -19.08084885026315902, -21.61197540051820454, 58.71434541541806595 ) ) ;
#8646=CARTESIAN_POINT ( 'NONE',  ( -11.42962537269896117, -10.38539323336976494, 74.62380298385740218 ) ) ;
#8648=CARTESIAN_POINT ( 'NONE',  ( -20.50090549915545424, -8.024104330060138679, 66.95820990016825647 ) ) ;
#8649=LINE ( 'NONE', #38913, #37249 ) ;
#8650=VERTEX_POINT ( 'NONE', #31777 ) ;
#8651=EDGE_LOOP ( 'NONE', ( #36103, #29902 ) ) ;
#8652=APPLICATION_CONTEXT ( 'automotive_design' ) ;
#8653=CARTESIAN_POINT ( 'NONE',  ( -21.33694788700791278, -9.004934622526002741, 73.60128753634342047 ) ) ;
#8654=CYLINDRICAL_SURFACE ( 'NONE', #6135, 0.1500000000000034084 ) ;
#8655=VERTEX_POINT ( 'NONE', #13277 ) ;
#8656=CARTESIAN_POINT ( 'NONE',  ( -22.18998830427771196, -20.00468049915955859, 65.71893796558269685 ) ) ;
#8657=CARTESIAN_POINT ( 'NONE',  ( -24.04530722081856453, -17.24086825362277509, 66.15177283638185202 ) ) ;
#8659=CARTESIAN_POINT ( 'NONE',  ( -17.35131678204048455, -7.807977840370839751, 70.67962813217452833 ) ) ;
#8660=CARTESIAN_POINT ( 'NONE',  ( -14.61306878872958137, -8.340592061241681066, 67.67463703838096478 ) ) ;
#8663=EDGE_LOOP ( 'NONE', ( #18675, #13790, #34368, #16394, #12354 ) ) ;
#8665=EDGE_CURVE ( 'NONE', #1976, #9242, #1823, .T. ) ;
#8666=CARTESIAN_POINT ( 'NONE',  ( -19.21561283247386598, -21.62782285876819088, 58.52507411012581429 ) ) ;
#8667=VECTOR ( 'NONE', #7666, 1000.000000000000114 ) ;
#8669=CARTESIAN_POINT ( 'NONE',  ( -10.23610968374255314, -12.85046669463587143, 67.85336945107273721 ) ) ;
#8670=CARTESIAN_POINT ( 'NONE',  ( -14.13242279744181573, -8.574497162196568212, 74.21426705364891063 ) ) ;
#8676=EDGE_CURVE ( 'NONE', #18372, #34964, #35463, .T. ) ;
#8677=ORIENTED_EDGE ( 'NONE', *, *, #2717, .T. ) ;
#8678=CARTESIAN_POINT ( 'NONE',  ( -11.56806251476610115, -18.73522173559940995, 65.03234934376791898 ) ) ;
#8679=EDGE_CURVE ( 'NONE', #32808, #5810, #48004, .T. ) ;
#8680=CARTESIAN_POINT ( 'NONE',  ( -16.39888349198502127, -21.73372412438269308, 62.05568132716130236 ) ) ;
#8681=AXIS2_PLACEMENT_3D ( 'NONE', #42582, #30280, #15711 ) ;
#8683=ORIENTED_EDGE ( 'NONE', *, *, #26599, .T. ) ;
#8684=CARTESIAN_POINT ( 'NONE',  ( -10.79572390357762046, -11.40795830647630282, 67.80360014157953685 ) ) ;
#8685=CARTESIAN_POINT ( 'NONE',  ( -10.40860991809309155, -15.50898095412354571, 57.85320721669017985 ) ) ;
#8686=EDGE_CURVE ( 'NONE', #29406, #33012, #26992, .T. ) ;
#8689=CARTESIAN_POINT ( 'NONE',  ( -23.90062161048602363, -17.60374255572093816, 59.00378367634043997 ) ) ;
#8690=( BOUNDED_CURVE ( )  B_SPLINE_CURVE ( 3, ( #45505, #14935, #26786, #3896 ),
 .UNSPECIFIED., .F., .F. ) 
 B_SPLINE_CURVE_WITH_KNOTS ( ( 4, 4 ),
 ( 0.4074455897393590154, 0.5000000000000000000 ),
 .UNSPECIFIED. ) 
 CURVE ( )  GEOMETRIC_REPRESENTATION_ITEM ( )  RATIONAL_B_SPLINE_CURVE ( ( 0.6983129098260651979, 0.7760317562606895425, 0.8765941196520058432, 1.000000000000024647 ) ) 
 REPRESENTATION_ITEM ( '' )  );
#8691=CARTESIAN_POINT ( 'NONE',  ( -23.04367355717579358, -10.55211556811382678, 59.90203429191419104 ) ) ;
#8692=ORIENTED_EDGE ( 'NONE', *, *, #553, .T. ) ;
#8693=CARTESIAN_POINT ( 'NONE',  ( -19.83852420082105894, -21.85790785478787868, 69.12137763959520953 ) ) ;
#8694=CARTESIAN_POINT ( 'NONE',  ( -17.39742496553465756, -7.759256980052345654, 67.02039592192092243 ) ) ;
#8695=ORIENTED_EDGE ( 'NONE', *, *, #11564, .T. ) ;
#8698=CARTESIAN_POINT ( 'NONE',  ( -17.23693881351924517, -7.361390637904862366, 70.65182322704724527 ) ) ;
#8699=ORIENTED_EDGE ( 'NONE', *, *, #23779, .F. ) ;
#8701=CARTESIAN_POINT ( 'NONE',  ( -15.53265176333180619, -21.60105060138385014, 72.33103357390284316 ) ) ;
#8706=VECTOR ( 'NONE', #17664, 999.9999999999998863 ) ;
#8707=CARTESIAN_POINT ( 'NONE',  ( -20.23440041452680660, -8.343390979720714640, 70.25660101728180962 ) ) ;
#8708=DIRECTION ( 'NONE',  ( -1.061592179903616477E-06, -3.103086884670442514E-06, 0.9999999999946218576 ) ) ;
#8709=CARTESIAN_POINT ( 'NONE',  ( -17.81896166628845180, -7.766655581923772367, 63.64237022204054028 ) ) ;
#8710=CARTESIAN_POINT ( 'NONE',  ( -10.45863924090583552, -14.11462608630872317, 61.21821294130609914 ) ) ;
#8712=EDGE_LOOP ( 'NONE', ( #42634, #29654, #16805, #9133, #24631 ) ) ;
#8713=CARTESIAN_POINT ( 'NONE',  ( -12.77013062424865630, -8.927826924028673616, 47.99999999999994316 ) ) ;
#8717=CARTESIAN_POINT ( 'NONE',  ( -15.00426899868425856, -21.85539911116967104, 65.28313592555664968 ) ) ;
#8718=CIRCLE ( 'NONE', #27572, 6.899999999999997691 ) ;
#8719=CARTESIAN_POINT ( 'NONE',  ( -10.60920434360279074, -17.81927616673939596, 71.76056483618631887 ) ) ;
#8721=CARTESIAN_POINT ( 'NONE',  ( -14.67456124858633615, -21.24707893775024203, 58.18234469924885133 ) ) ;
#8722=EDGE_CURVE ( 'NONE', #35691, #26935, #15256, .T. ) ;
#8724=CARTESIAN_POINT ( 'NONE',  ( -23.76058118794394503, -11.83148257926706393, 63.02388499825810442 ) ) ;
#8725=DIRECTION ( 'NONE',  ( -0.3037135924646501839, 0.9527633776296273727, 2.170275161112374231E-08 ) ) ;
#8726=CARTESIAN_POINT ( 'NONE',  ( -23.99668814781213300, -11.30145868231390338, 66.61488666845116313 ) ) ;
#8727=EDGE_CURVE ( 'NONE', #2574, #48564, #20374, .T. ) ;
#8730=FACE_OUTER_BOUND ( 'NONE', #5215, .T. ) ;
#8731=CARTESIAN_POINT ( 'NONE',  ( -24.39160045767772544, -17.44704251381193316, 69.59152525453608007 ) ) ;
#8734=CARTESIAN_POINT ( 'NONE',  ( -21.01123855637963089, -20.87838213191899683, 65.58453944497207999 ) ) ;
#8735=VERTEX_POINT ( 'NONE', #30038 ) ;
#8736=ORIENTED_EDGE ( 'NONE', *, *, #25231, .F. ) ;
#8738=VECTOR ( 'NONE', #17603, 1000.000000000000114 ) ;
#8739=CARTESIAN_POINT ( 'NONE',  ( -19.88526343185200673, -21.36290080982552553, 72.42701748270100381 ) ) ;
#8740=ADVANCED_FACE ( 'NONE', ( #32732 ), #37317, .T. ) ;
#8741=VECTOR ( 'NONE', #16373, 999.9999999999998863 ) ;
#8743=ADVANCED_FACE ( 'NONE', ( #21894 ), #26091, .T. ) ;
#8744=( BOUNDED_SURFACE ( )  B_SPLINE_SURFACE ( 3, 1, ( 
 ( #37216, #15057 ),
 ( #30600, #45624 ),
 ( #26404, #3500 ),
 ( #37459, #19492 ),
 ( #41415, #30115 ),
 ( #26902, #34507 ),
 ( #3751, #18766 ) ),
 .UNSPECIFIED., .T., .F., .F. ) 
 B_SPLINE_SURFACE_WITH_KNOTS ( ( 4, 3, 4 ),
 ( 2, 2 ),
 ( 0.000000000000000000, 0.5000000000000000000, 1.000000000000000000 ),
 ( 0.000000000000000000, 1.000000000000000000 ),
 .UNSPECIFIED. ) 
 GEOMETRIC_REPRESENTATION_ITEM ( )  RATIONAL_B_SPLINE_SURFACE ( (
 ( 1.000000000000000000, 1.000000000000000000),
 ( 0.3333333333333335369, 0.3333333333333330373),
 ( 0.3333333333333335369, 0.3333333333333330373),
 ( 1.000000000000000000, 1.000000000000000000),
 ( 0.3333333333333333703, 0.3333333333333333703),
 ( 0.3333333333333333703, 0.3333333333333333703),
 ( 1.000000000000000000, 1.000000000000000000) ) ) 
 REPRESENTATION_ITEM ( '' )  SURFACE ( )  );
#8749=FACE_OUTER_BOUND ( 'NONE', #4212, .T. ) ;
#8751=CARTESIAN_POINT ( 'NONE',  ( -24.26499789074519597, -17.75976756996305639, 62.65856417960095825 ) ) ;
#8752=ADVANCED_FACE ( 'NONE', ( #47756 ), #13993, .T. ) ;
#8753=ORIENTED_EDGE ( 'NONE', *, *, #13321, .T. ) ;
#8754=( BOUNDED_CURVE ( )  B_SPLINE_CURVE ( 3, ( #1466, #46555, #20443, #21354 ),
 .UNSPECIFIED., .F., .F. ) 
 B_SPLINE_CURVE_WITH_KNOTS ( ( 4, 4 ),
 ( 0.4074455897393638448, 0.5000000000000000000 ),
 .UNSPECIFIED. ) 
 CURVE ( )  GEOMETRIC_REPRESENTATION_ITEM ( )  RATIONAL_B_SPLINE_CURVE ( ( 0.6983129098261096068, 0.7760317562607167430, 0.8765941196520149470, 1.000000000000006883 ) ) 
 REPRESENTATION_ITEM ( '' )  );
#8755=CARTESIAN_POINT ( 'NONE',  ( -12.84719963800786502, -9.512789006345032661, 74.31923006385322594 ) ) ;
#8756=EDGE_LOOP ( 'NONE', ( #33372, #40660, #13366, #18822, #45939 ) ) ;
#8757=CARTESIAN_POINT ( 'NONE',  ( -10.72530867274958233, -17.00760959713300480, 57.97288447305808745 ) ) ;
#8759=ORIENTED_EDGE ( 'NONE', *, *, #26530, .T. ) ;
#8760=CARTESIAN_POINT ( 'NONE',  ( -13.25841313310420766, -9.121485346447943954, 64.20946499508677618 ) ) ;
#8761=B_SPLINE_CURVE_WITH_KNOTS ( 'NONE', 3,
 ( #40455, #14325, #47850, #14558, #29380, #3508, #10195, #10437, #14806, #40945 ),
 .UNSPECIFIED., .F., .F.,
 ( 4, 2, 2, 2, 4 ),
 ( 0.6272669072878209739, 0.7522669073073412482, 0.8772669073268615225, 1.002266907346381686, 1.127266907365902071 ),
 .UNSPECIFIED. ) ;
#8763=CARTESIAN_POINT ( 'NONE',  ( -20.03377823521572765, -8.313858397182363191, 70.44203619096923319 ) ) ;
#8764=CARTESIAN_POINT ( 'NONE',  ( -20.88906156096523148, -8.213963083740734916, 59.94786934217235341 ) ) ;
#8765=ORIENTED_EDGE ( 'NONE', *, *, #5531, .F. ) ;
#8766=CARTESIAN_POINT ( 'NONE',  ( -21.89130958583942288, -9.354787850460871468, 63.20625856529903075 ) ) ;
#8767=CARTESIAN_POINT ( 'NONE',  ( -24.44055745662519641, -14.11932379769929113, 73.13743607903229815 ) ) ;
#8768=FACE_OUTER_BOUND ( 'NONE', #45115, .T. ) ;
#8769=CARTESIAN_POINT ( 'NONE',  ( -18.39951368268757648, -22.19516171751901368, 69.00010101991060196 ) ) ;
#8772=CARTESIAN_POINT ( 'NONE',  ( -20.66696756681432490, -21.06910030335248152, 58.64475164910062688 ) ) ;
#8773=CARTESIAN_POINT ( 'NONE',  ( -23.46260529264823447, -11.17067950781535579, 73.36193301757424479 ) ) ;
#8774=DIRECTION ( 'NONE',  ( 0.7150252244155715919, -0.6990986543038554268, 7.133781456731073326E-17 ) ) ;
#8776=FACE_OUTER_BOUND ( 'NONE', #7932, .T. ) ;
#8777=ORIENTED_EDGE ( 'NONE', *, *, #31906, .T. ) ;
#8778=LINE ( 'NONE', #5077, #25079 ) ;
#8779=CARTESIAN_POINT ( 'NONE',  ( -13.26878139971602621, -9.173971005569262260, 67.56869938284187072 ) ) ;
#8780=EDGE_CURVE ( 'NONE', #6936, #47492, #4649, .T. ) ;
#8781=EDGE_LOOP ( 'NONE', ( #5908, #43495 ) ) ;
#8784=FACE_BOUND ( 'NONE', #28335, .T. ) ;
#8785=ORIENTED_EDGE ( 'NONE', *, *, #36642, .T. ) ;
#8786=ORIENTED_EDGE ( 'NONE', *, *, #39724, .F. ) ;
#8788=CARTESIAN_POINT ( 'NONE',  ( -10.99582178678916833, -11.91441492378913658, 74.85840195586327184 ) ) ;
#8792=CARTESIAN_POINT ( 'NONE',  ( -14.58386025153609467, -8.409552409253036487, 67.44902071755305428 ) ) ;
#8793=CARTESIAN_POINT ( 'NONE',  ( -21.12516169987187098, -20.80993955427394582, 69.06922321213187388 ) ) ;
#8794=CARTESIAN_POINT ( 'NONE',  ( -13.43328788299345966, -9.058103587765096165, 60.73950223935946013 ) ) ;
#8795=VERTEX_POINT ( 'NONE', #34185 ) ;
#8798=ADVANCED_FACE ( 'NONE', ( #3929 ), #7874, .T. ) ;
#8799=B_SPLINE_CURVE_WITH_KNOTS ( 'NONE', 3,
 ( #44166, #43671, #44626, #44387, #25424, #10416, #25653, #10884, #3001, #2285 ),
 .UNSPECIFIED., .F., .F.,
 ( 4, 2, 2, 2, 4 ),
 ( 0.6272669072877721241, 0.7522669073073040558, 0.8772669073268360984, 1.002266907346368141, 1.127266907365900073 ),
 .UNSPECIFIED. ) ;
#8800=PLANE ( 'NONE',  #46466 ) ;
#8801=CARTESIAN_POINT ( 'NONE',  ( -21.62013776805207854, -9.204234041992926052, 70.32059703345998969 ) ) ;
#8802=ORIENTED_EDGE ( 'NONE', *, *, #22750, .T. ) ;
#8804=EDGE_LOOP ( 'NONE', ( #48377, #7087, #34679, #24510, #4994 ) ) ;
#8807=CARTESIAN_POINT ( 'NONE',  ( -23.02753331400065662, -10.61361262881353085, 59.60203474230917919 ) ) ;
#8809=CARTESIAN_POINT ( 'NONE',  ( -17.26260884657101258, -7.811009669971855196, 67.09327729553568531 ) ) ;
#8812=CARTESIAN_POINT ( 'NONE',  ( -13.27770617114843965, -9.107455183738579763, 64.05946529205222362 ) ) ;
#8813=CARTESIAN_POINT ( 'NONE',  ( -22.39254715322108780, -9.803279359720651343, 73.36672461330924477 ) ) ;
#8814=CARTESIAN_POINT ( 'NONE',  ( -10.81230840161673790, -17.25685697075765646, 64.64211442681141762 ) ) ;
#8815=CARTESIAN_POINT ( 'NONE',  ( -23.12302657392458016, -18.95946740514217765, 62.35406880581413702 ) ) ;
#8820=DIRECTION ( 'NONE',  ( 0.5562740912439652075, 0.8309988781043535777, 7.851267780903551505E-08 ) ) ;
#8822=ORIENTED_EDGE ( 'NONE', *, *, #27799, .T. ) ;
#8823=CARTESIAN_POINT ( 'NONE',  ( -10.42930205768512941, -13.90492575851057211, 61.33310083575204885 ) ) ;
#8824=EDGE_CURVE ( 'NONE', #46544, #12446, #18770, .T. ) ;
#8826=CARTESIAN_POINT ( 'NONE',  ( -21.73098984888145679, -8.730191469543168381, 70.31627926275058371 ) ) ;
#8827=CARTESIAN_POINT ( 'NONE',  ( -14.79922921121938195, -7.836842249070715916, 57.03495322699122738 ) ) ;
#8829=EDGE_CURVE ( 'NONE', #19901, #38378, #28800, .T. ) ;
#8831=CARTESIAN_POINT ( 'NONE',  ( -21.79520202288280117, -20.27875078180004920, 58.95369995708556843 ) ) ;
#8832=CARTESIAN_POINT ( 'NONE',  ( -24.24046477733709182, -13.21445941831622761, 63.11647676942984475 ) ) ;
#8835=CARTESIAN_POINT ( 'NONE',  ( -24.14992870231961319, -18.01341063617936911, 59.11883102335588802 ) ) ;
#8836=CARTESIAN_POINT ( 'NONE',  ( -20.64758834049123593, -8.594144569355316676, 63.38291771811893938 ) ) ;
#8837=CARTESIAN_POINT ( 'NONE',  ( -23.12535539932854078, -10.01343808792704237, 66.65686846082743955 ) ) ;
#8840=CARTESIAN_POINT ( 'NONE',  ( -24.73606664458329263, -16.23668146098944831, 62.79317443719546787 ) ) ;
#8841=ORIENTED_EDGE ( 'NONE', *, *, #27206, .T. ) ;
#8842=ORIENTED_EDGE ( 'NONE', *, *, #7063, .T. ) ;
#8844=CARTESIAN_POINT ( 'NONE',  ( -22.78465872505329770, -10.30744173788789908, 66.54182281442142255 ) ) ;
#8845=CARTESIAN_POINT ( 'NONE',  ( -13.44410990971816666, -8.986443949771105721, 64.32435409333248799 ) ) ;
#8846=CARTESIAN_POINT ( 'NONE',  ( -10.42732927771101359, -14.54885032245585386, 71.43855692335705498 ) ) ;
#8848=CARTESIAN_POINT ( 'NONE',  ( -15.47038452772150663, -21.58309165278561537, 72.04575460769355288 ) ) ;
#8849=CARTESIAN_POINT ( 'NONE',  ( -22.51726247777427758, -19.68384842258191725, 72.94400547081133368 ) ) ;
#8851=CARTESIAN_POINT ( 'NONE',  ( -24.40658499505740053, -15.78250870199476807, 69.83307488408829045 ) ) ;
#8852=EDGE_LOOP ( 'NONE', ( #26050, #10541, #35046, #33401, #10688 ) ) ;
#8853=ORIENTED_EDGE ( 'NONE', *, *, #11726, .F. ) ;
#8856=CARTESIAN_POINT ( 'NONE',  ( -23.64864541627648009, -11.60591314845866684, 66.70597954916981109 ) ) ;
#8857=CARTESIAN_POINT ( 'NONE',  ( -22.48114071483173149, -19.64927648862363796, 72.94400547034429394 ) ) ;
#8858=CARTESIAN_POINT ( 'NONE',  ( -18.83585931754296183, -7.494105970839488151, 70.48572750873847781 ) ) ;
#8863=DIRECTION ( 'NONE',  ( 0.7621627669932626858, -0.6473854467078885566, 3.680865982637999709E-08 ) ) ;
#8864=CARTESIAN_POINT ( 'NONE',  ( -11.10069974846098262, -18.74849293576752984, 61.46984965132461554 ) ) ;
#8865=VERTEX_POINT ( 'NONE', #26572 ) ;
#8867=VERTEX_POINT ( 'NONE', #8348 ) ;
#8868=DIRECTION ( 'NONE',  ( 1.352396030810764649E-06, 5.694414615768204918E-07, 0.9999999999989234167 ) ) ;
#8869=( BOUNDED_CURVE ( )  B_SPLINE_CURVE ( 3, ( #5244, #26931, #20261, #31101 ),
 .UNSPECIFIED., .F., .F. ) 
 B_SPLINE_CURVE_WITH_KNOTS ( ( 4, 4 ),
 ( 4.712388980384691450, 4.921828490624010399 ),
 .UNSPECIFIED. ) 
 CURVE ( )  GEOMETRIC_REPRESENTATION_ITEM ( )  RATIONAL_B_SPLINE_CURVE ( ( 1.000000000000000000, 0.9963479302455156006, 0.9963479302455156006, 1.000000000000000000 ) ) 
 REPRESENTATION_ITEM ( '' )  );
#8872=CARTESIAN_POINT ( 'NONE',  ( -10.48085350821551742, -13.91959267249018950, 57.44825035245948186 ) ) ;
#8873=EDGE_CURVE ( 'NONE', #35369, #1693, #37590, .T. ) ;
#8874=ORIENTED_EDGE ( 'NONE', *, *, #15055, .T. ) ;
#8876=CARTESIAN_POINT ( 'NONE',  ( -21.61813247623101830, -8.651786778886961571, 73.71633474065167491 ) ) ;
#8877=ORIENTED_EDGE ( 'NONE', *, *, #20906, .T. ) ;
#8878=FACE_OUTER_BOUND ( 'NONE', #36345, .T. ) ;
#8879=ADVANCED_FACE ( 'NONE', ( #4903 ), #16892, .T. ) ;
#8881=CARTESIAN_POINT ( 'NONE',  ( -18.51768661843271602, -21.77690966467453393, 68.70025907080108141 ) ) ;
#8883=FACE_OUTER_BOUND ( 'NONE', #8852, .T. ) ;
#8884=CARTESIAN_POINT ( 'NONE',  ( -14.79922921121938195, -7.836842249070715916, 57.03495322699122738 ) ) ;
#8885=DIRECTION ( 'NONE',  ( -2.403795749289375575E-06, -2.069898561751298366E-06, -0.9999999999949685803 ) ) ;
#8886=EDGE_LOOP ( 'NONE', ( #12482, #10563, #46876, #38395, #38706 ) ) ;
#8887=( BOUNDED_CURVE ( )  B_SPLINE_CURVE ( 3, ( #44337, #10589, #14722, #37148 ),
 .UNSPECIFIED., .F., .F. ) 
 B_SPLINE_CURVE_WITH_KNOTS ( ( 4, 4 ),
 ( 0.4074455897393665649, 0.5000000000000000000 ),
 .UNSPECIFIED. ) 
 CURVE ( )  GEOMETRIC_REPRESENTATION_ITEM ( )  RATIONAL_B_SPLINE_CURVE ( ( 0.6983129098260959511, 0.7760317562607057518, 0.8765941196520083967, 1.000000000000007772 ) ) 
 REPRESENTATION_ITEM ( '' )  );
#8889=CARTESIAN_POINT ( 'NONE',  ( -10.47368616940683772, -17.49164935309025282, 64.67093470525151133 ) ) ;
#8890=B_SPLINE_CURVE_WITH_KNOTS ( 'NONE', 3,
 ( #33151, #21612, #17422, #32454, #40798, #7083, #6350, #21380, #18380, #43784 ),
 .UNSPECIFIED., .F., .F.,
 ( 4, 2, 2, 2, 4 ),
 ( 0.6272669072877604668, 0.7522669073072733026, 0.8772669073267862494, 1.002266907346299085, 1.127266907365811921 ),
 .UNSPECIFIED. ) ;
#8893=CARTESIAN_POINT ( 'NONE',  ( -24.76302562995550716, -16.09181782173303077, 66.20291600427756862 ) ) ;
#8894=EDGE_LOOP ( 'NONE', ( #28083, #40268, #32080, #16621, #37192 ) ) ;
#8895=VERTEX_POINT ( 'NONE', #17156 ) ;
#8896=CARTESIAN_POINT ( 'NONE',  ( -24.47598042472018776, -12.40625281542414449, 73.43499722901042048 ) ) ;
#8897=DIRECTION ( 'NONE',  ( -0.7171836970970659753, 0.6968841687240312499, -4.479616660400631173E-09 ) ) ;
#8898=EDGE_LOOP ( 'NONE', ( #25578, #34378 ) ) ;
#8899=CARTESIAN_POINT ( 'NONE',  ( -15.68463861365884249, -7.564349260043091938, 67.25351876580783994 ) ) ;
#8901=CARTESIAN_POINT ( 'NONE',  ( -23.02926993209503337, -10.53310206560860074, 59.90203402044859615 ) ) ;
#8902=CARTESIAN_POINT ( 'NONE',  ( -13.01353307917097268, -8.804980454159759162, 64.09441913135431435 ) ) ;
#8903=CARTESIAN_POINT ( 'NONE',  ( -24.28619334359350290, -16.42731978468327014, 59.13804568661029037 ) ) ;
#8905=( BOUNDED_CURVE ( )  B_SPLINE_CURVE ( 3, ( #36814, #3099, #18107, #44485 ),
 .UNSPECIFIED., .F., .F. ) 
 B_SPLINE_CURVE_WITH_KNOTS ( ( 4, 4 ),
 ( 0.9074455897393663983, 1.000000000000000000 ),
 .UNSPECIFIED. ) 
 CURVE ( )  GEOMETRIC_REPRESENTATION_ITEM ( )  RATIONAL_B_SPLINE_CURVE ( ( 0.6983129098261118273, 0.7760317562607144115, 0.8765941196520105061, 1.000000000000000000 ) ) 
 REPRESENTATION_ITEM ( '' )  );
#8906=ORIENTED_EDGE ( 'NONE', *, *, #34780, .F. ) ;
#8907=CARTESIAN_POINT ( 'NONE',  ( -16.50613596612109646, -22.20251566029174128, 65.48210330380625521 ) ) ;
#8908=EDGE_CURVE ( 'NONE', #25681, #35257, #27064, .T. ) ;
#8909=CARTESIAN_POINT ( 'NONE',  ( -20.83485798093626329, -8.694536558548913163, 59.95198372774736129 ) ) ;
#8910=CARTESIAN_POINT ( 'NONE',  ( -22.51432625447135649, -9.926136081597567440, 70.01178455096938080 ) ) ;
#8912=CARTESIAN_POINT ( 'NONE',  ( -21.49815937814055999, -9.116931945208399668, 70.43132539264750847 ) ) ;
#8916=VERTEX_POINT ( 'NONE', #31474 ) ;
#8917=EDGE_CURVE ( 'NONE', #14347, #21243, #32024, .T. ) ;
#8918=CARTESIAN_POINT ( 'NONE',  ( -12.01449246772864576, -9.686654477736338364, 60.73730818761442407 ) ) ;
#8919=EDGE_CURVE ( 'NONE', #6766, #26691, #38745, .T. ) ;
#8920=CARTESIAN_POINT ( 'NONE',  ( -11.00038316533314919, -18.58284169098544680, 57.98431467230947334 ) ) ;
#8922=ORIENTED_EDGE ( 'NONE', *, *, #31100, .T. ) ;
#8923=CARTESIAN_POINT ( 'NONE',  ( -10.43244324318236593, -14.46516609096106265, 67.85800133269570722 ) ) ;
#8926=ORIENTED_EDGE ( 'NONE', *, *, #19348, .F. ) ;
#8927=CARTESIAN_POINT ( 'NONE',  ( -10.64059482219176722, -17.88964966403732859, 71.70571712204632320 ) ) ;
#8928=CARTESIAN_POINT ( 'NONE',  ( -19.44371787714632305, -21.98101111209947334, 58.63852002154196441 ) ) ;
#8929=VERTEX_POINT ( 'NONE', #20401 ) ;
#8930=CARTESIAN_POINT ( 'NONE',  ( -11.30361205576526196, -11.41219277671509147, 64.44882039656690154 ) ) ;
#8931=CARTESIAN_POINT ( 'NONE',  ( -17.39742496553465401, -7.759256980052345654, 67.02039592192090822 ) ) ;
#8932=ORIENTED_EDGE ( 'NONE', *, *, #45634, .T. ) ;
#8933=CARTESIAN_POINT ( 'NONE',  ( -16.00544582274271477, -7.903112417841744453, 63.95538887075813506 ) ) ;
#8934=CARTESIAN_POINT ( 'NONE',  ( -22.21960400195047569, -20.51063794322999101, 58.87104585263988099 ) ) ;
#8937=CARTESIAN_POINT ( 'NONE',  ( -24.27074747244433794, -17.74661109614212506, 62.63394374183828006 ) ) ;
#8938=EDGE_CURVE ( 'NONE', #29708, #10558, #21123, .T. ) ;
#8939=EDGE_CURVE ( 'NONE', #28685, #47879, #43980, .T. ) ;
#8941=CARTESIAN_POINT ( 'NONE',  ( -20.06975372951847447, -8.274133229585533655, 73.73568642813194174 ) ) ;
#8942=CARTESIAN_POINT ( 'NONE',  ( -14.60783717270099835, -21.70648693424663378, 58.35113322083577003 ) ) ;
#8943=CARTESIAN_POINT ( 'NONE',  ( -24.47354813883760016, -12.39902559715248032, 73.42720875634239519 ) ) ;
#8944=DIRECTION ( 'NONE',  ( 3.549360974554993999E-17, -6.371834667797928663E-18, -1.000000000000000000 ) ) ;
#8946=CARTESIAN_POINT ( 'NONE',  ( -24.43362379028604536, -14.05489247495133753, 73.12271507725591846 ) ) ;
#8947=CARTESIAN_POINT ( 'NONE',  ( -23.46741973463711872, -19.16603908095663655, 62.53902270128352825 ) ) ;
#8948=CARTESIAN_POINT ( 'NONE',  ( -14.60689809042302834, -8.346551666329650843, 64.08978840692947188 ) ) ;
#8949=EDGE_CURVE ( 'NONE', #29810, #16043, #12178, .T. ) ;
#8956=DIRECTION ( 'NONE',  ( -0.7364384864160969935, 0.6765045127160409510, 1.031360481960658298E-08 ) ) ;
#8959=CARTESIAN_POINT ( 'NONE',  ( -10.60259942276942802, -17.80446876823743096, 71.69001273946355468 ) ) ;
#8960=EDGE_CURVE ( 'NONE', #41932, #891, #17616, .T. ) ;
#8963=ORIENTED_EDGE ( 'NONE', *, *, #15879, .F. ) ;
#8965=CARTESIAN_POINT ( 'NONE',  ( -12.32158608955787393, -9.943909642237139579, 60.57390139315987909 ) ) ;
#8967=EDGE_LOOP ( 'NONE', ( #17379, #39570, #12815, #22227, #26340 ) ) ;
#8968=CARTESIAN_POINT ( 'NONE',  ( -12.69763806180496601, -20.04058448603118592, 68.62185382311069759 ) ) ;
#8969=CARTESIAN_POINT ( 'NONE',  ( -24.23802539630901265, -11.79523892523793371, 59.66890987421792403 ) ) ;
#8970=CARTESIAN_POINT ( 'NONE',  ( -10.40062145488671241, -15.42068369279106221, 57.56792819272491357 ) ) ;
#8971=DIRECTION ( 'NONE',  ( -9.588436366354112311E-09, -2.115493567789935748E-07, -0.9999999999999775735 ) ) ;
#8973=ORIENTED_EDGE ( 'NONE', *, *, #23115, .T. ) ;
#8976=CARTESIAN_POINT ( 'NONE',  ( -22.99332866974948075, -9.860676417004754057, 70.18991268411126327 ) ) ;
#8977=B_SPLINE_CURVE_WITH_KNOTS ( 'NONE', 1,
 ( #11305, #26317 ),
 .UNSPECIFIED., .F., .F.,
 ( 2, 2 ),
 ( 0.000000000000000000, 1.000000000000000000 ),
 .UNSPECIFIED. ) ;
#8978=CARTESIAN_POINT ( 'NONE',  ( -19.01758550583589269, -21.68056959198661815, 58.82507637440430415 ) ) ;
#8979=B_SPLINE_CURVE_WITH_KNOTS ( 'NONE', 3,
 ( #39107, #39836, #2164, #13227, #6104, #12772, #5390, #20413, #9580, #47481 ),
 .UNSPECIFIED., .F., .F.,
 ( 4, 2, 2, 2, 4 ),
 ( 0.6272669072877348206, 0.7522669073072507651, 0.8772669073267668205, 1.002266907346282876, 1.127266907365798820 ),
 .UNSPECIFIED. ) ;
#8981=CARTESIAN_POINT ( 'NONE',  ( -13.94388580779785691, -20.88290965541650479, 68.75625091190090643 ) ) ;
#8982=ORIENTED_EDGE ( 'NONE', *, *, #39547, .F. ) ;
#8983=CARTESIAN_POINT ( 'NONE',  ( -10.36617775085144899, -14.83726598580069300, 68.01367321887373407 ) ) ;
#8984=CARTESIAN_POINT ( 'NONE',  ( -18.26345899425187369, -22.21252533677388286, 65.45876839498835409 ) ) ;
#8987=CARTESIAN_POINT ( 'NONE',  ( -21.25293954998800672, -20.66975872501122424, 72.54063127481728657 ) ) ;
#8988=CARTESIAN_POINT ( 'NONE',  ( -12.94846085306722294, -9.425284032318575811, 74.54752936559843590 ) ) ;
#8989=VECTOR ( 'NONE', #7883, 1000.000000000000227 ) ;
#8990=EDGE_LOOP ( 'NONE', ( #41040, #43919 ) ) ;
#8991=CARTESIAN_POINT ( 'NONE',  ( -13.29845767883066543, -21.01266560759323809, 61.63150935275904629 ) ) ;
#8992=CARTESIAN_POINT ( 'NONE',  ( -10.42338558849718311, -15.67229764252504332, 57.56792711140763430 ) ) ;
#8994=CARTESIAN_POINT ( 'NONE',  ( -12.14425528403576493, -10.13739698163135117, 64.02914326607979945 ) ) ;
#8995=EDGE_CURVE ( 'NONE', #31288, #9885, #47129, .T. ) ;
#8997=B_SPLINE_CURVE_WITH_KNOTS ( 'NONE', 3,
 ( #6442, #28602, #13313, #9660, #17730, #10382, #20969, #9413, #24675, #24437 ),
 .UNSPECIFIED., .F., .F.,
 ( 4, 2, 2, 2, 4 ),
 ( 0.1272669073658574679, 0.2522669073463327249, 0.3772669073268078987, 0.5022669073072831836, 0.6272669072877583574 ),
 .UNSPECIFIED. ) ;
#8998=FACE_OUTER_BOUND ( 'NONE', #27506, .T. ) ;
#8999=CARTESIAN_POINT ( 'NONE',  ( -15.15660932275500272, -21.48492473237050859, 65.39124617759186719 ) ) ;
#9000=CARTESIAN_POINT ( 'NONE',  ( -24.30269918248666272, -16.11583968492636032, 66.25252109504093312 ) ) ;
#9001=ORIENTED_EDGE ( 'NONE', *, *, #1094, .F. ) ;
#9004=CARTESIAN_POINT ( 'NONE',  ( -21.31115985637654120, -8.927249709250720144, 73.88656608925673197 ) ) ;
#9005=FACE_BOUND ( 'NONE', #29615, .T. ) ;
#9006=EDGE_CURVE ( 'NONE', #29810, #47031, #12921, .T. ) ;
#9007=CARTESIAN_POINT ( 'NONE',  ( -10.37462438995674319, -14.89569194323783208, 74.79778901495059529 ) ) ;
#9008=CARTESIAN_POINT ( 'NONE',  ( -17.60317953294568127, -7.758478677834707682, 67.43528183898541783 ) ) ;
#9011=ORIENTED_EDGE ( 'NONE', *, *, #10917, .T. ) ;
#9012=CARTESIAN_POINT ( 'NONE',  ( -23.64494593247637866, -11.48417377041487164, 62.95218242698565092 ) ) ;
#9014=ORIENTED_EDGE ( 'NONE', *, *, #9521, .F. ) ;
#9015=CARTESIAN_POINT ( 'NONE',  ( -11.71918404020638427, -18.95175453447547653, 71.70158022526054253 ) ) ;
#9017=ORIENTED_EDGE ( 'NONE', *, *, #44678, .T. ) ;
#9018=FACE_OUTER_BOUND ( 'NONE', #26145, .T. ) ;
#9019=CARTESIAN_POINT ( 'NONE',  ( -11.93195840498443516, -10.38844327383712773, 70.98365212470247343 ) ) ;
#9020=B_SPLINE_CURVE_WITH_KNOTS ( 'NONE', 3,
 ( #19521, #15562, #4752, #30867, #45881, #12136, #38468, #15079, #24192, #39199 ),
 .UNSPECIFIED., .F., .F.,
 ( 4, 2, 2, 2, 4 ),
 ( 0.000000000000000000, 0.2500000000000000000, 0.5000000000000000000, 0.7500000000000000000, 1.000000000000000000 ),
 .UNSPECIFIED. ) ;
#9022=EDGE_LOOP ( 'NONE', ( #24793, #22610, #3319, #14506, #35297 ) ) ;
#9023=ORIENTED_EDGE ( 'NONE', *, *, #22516, .T. ) ;
#9024=DIRECTION ( 'NONE',  ( -0.9118114225829225816, -0.4106092176842893182, -5.589476761700638731E-08 ) ) ;
#9026=EDGE_CURVE ( 'NONE', #41394, #33214, #7097, .T. ) ;
#9027=( BOUNDED_CURVE ( )  B_SPLINE_CURVE ( 3, ( #30337, #33747, #22200, #37187 ),
 .UNSPECIFIED., .F., .F. ) 
 B_SPLINE_CURVE_WITH_KNOTS ( ( 4, 4 ),
 ( 0.4074455897393669535, 0.5000000000000000000 ),
 .UNSPECIFIED. ) 
 CURVE ( )  GEOMETRIC_REPRESENTATION_ITEM ( )  RATIONAL_B_SPLINE_CURVE ( ( 0.6983129098260987266, 0.7760317562607002007, 0.8765941196519997369, 0.9999999999999954481 ) ) 
 REPRESENTATION_ITEM ( '' )  );
#9028=CARTESIAN_POINT ( 'NONE',  ( -21.22430400244884297, -8.930495821374908161, 73.67416693519540161 ) ) ;
#9029=CARTESIAN_POINT ( 'NONE',  ( -10.60833884242739522, -12.99528357717770355, 64.15347367985145866 ) ) ;
#9030=CARTESIAN_POINT ( 'NONE',  ( -13.65433549462749596, -7.199988887673270277, 54.38277594638588397 ) ) ;
#9031=EDGE_LOOP ( 'NONE', ( #17353, #1870 ) ) ;
#9032=ORIENTED_EDGE ( 'NONE', *, *, #336, .T. ) ;
#9033=VECTOR ( 'NONE', #36575, 1000.000000000000114 ) ;
#9037=CARTESIAN_POINT ( 'NONE',  ( -21.51679988820674438, -20.55329806219026523, 72.40957539702174017 ) ) ;
#9038=CARTESIAN_POINT ( 'NONE',  ( -20.68814852852636221, -21.05812772122902388, 58.94475156075989730 ) ) ;
#9039=DIRECTION ( 'NONE',  ( 6.651268170491444817E-06, 3.577353459756793540E-06, 0.9999999999714814791 ) ) ;
#9041=( BOUNDED_CURVE ( )  B_SPLINE_CURVE ( 3, ( #11325, #33452, #37394, #26337 ),
 .UNSPECIFIED., .F., .F. ) 
 B_SPLINE_CURVE_WITH_KNOTS ( ( 4, 4 ),
 ( 0.4074455897393630677, 0.5000000000000000000 ),
 .UNSPECIFIED. ) 
 CURVE ( )  GEOMETRIC_REPRESENTATION_ITEM ( )  RATIONAL_B_SPLINE_CURVE ( ( 0.6983129098260806300, 0.7760317562606832142, 0.8765941196519884127, 0.9999999999999931166 ) ) 
 REPRESENTATION_ITEM ( '' )  );
#9043=CARTESIAN_POINT ( 'NONE',  ( -14.73375560093340120, -21.75656996136207866, 61.75105004614717785 ) ) ;
#9045=CARTESIAN_POINT ( 'NONE',  ( -24.46050813376110611, -17.25744323842079098, 73.04482527373910727 ) ) ;
#9046=EDGE_CURVE ( 'NONE', #48213, #42290, #40095, .T. ) ;
#9047=EDGE_LOOP ( 'NONE', ( #46287, #34318, #45469, #4124, #1210 ) ) ;
#9048=CARTESIAN_POINT ( 'NONE',  ( -11.59752430615055729, -18.69167855836258596, 68.32762835703452708 ) ) ;
#9049=CARTESIAN_POINT ( 'NONE',  ( -10.37394849890712401, -14.76283852923608464, 71.61310637325181006 ) ) ;
#9050=LINE ( 'NONE', #24066, #20157 ) ;
#9051=CARTESIAN_POINT ( 'NONE',  ( -19.10873388551254948, -7.551407109436953924, 67.08727174327995613 ) ) ;
#9052=ORIENTED_EDGE ( 'NONE', *, *, #25102, .T. ) ;
#9053=CARTESIAN_POINT ( 'NONE',  ( -24.46506320217640962, -17.24406362331221132, 72.99840605271779737 ) ) ;
#9054=CARTESIAN_POINT ( 'NONE',  ( -22.88305309436651669, -19.19300359198548378, 58.95580955766958198 ) ) ;
#9055=CARTESIAN_POINT ( 'NONE',  ( -10.33431723597471930, -12.52035407725662886, 60.98348989824278732 ) ) ;
#9056=ORIENTED_EDGE ( 'NONE', *, *, #18929, .F. ) ;
#9057=CARTESIAN_POINT ( 'NONE',  ( -17.15134030326023051, -7.364115279526828317, 70.67531275522621570 ) ) ;
#9058=ORIENTED_EDGE ( 'NONE', *, *, #36915, .T. ) ;
#9063=CARTESIAN_POINT ( 'NONE',  ( -22.20754945420574700, -20.52070228389602136, 58.96431674811245927 ) ) ;
#9066=ADVANCED_FACE ( 'NONE', ( #37262 ), #29656, .T. ) ;
#9069=CARTESIAN_POINT ( 'NONE',  ( -13.42213083866590040, -20.61341924012868887, 58.34090257147585135 ) ) ;
#9071=EDGE_CURVE ( 'NONE', #4198, #48039, #29937, .T. ) ;
#9072=CARTESIAN_POINT ( 'NONE',  ( -20.81921488491704864, -21.44071703825394692, 58.75979854551385984 ) ) ;
#9073=B_SPLINE_CURVE_WITH_KNOTS ( 'NONE', 3,
 ( #40358, #21420, #24863, #29281, #6631, #17462, #2684, #25821, #10082, #44315 ),
 .UNSPECIFIED., .F., .F.,
 ( 4, 2, 2, 2, 4 ),
 ( 0.000000000000000000, 0.2500000000000000000, 0.5000000000000000000, 0.7500000000000000000, 1.000000000000000000 ),
 .UNSPECIFIED. ) ;
#9075=ORIENTED_EDGE ( 'NONE', *, *, #43117, .T. ) ;
#9076=CARTESIAN_POINT ( 'NONE',  ( -10.62601537294527176, -11.76145610990993617, 74.65816588861473235 ) ) ;
#9077=EDGE_CURVE ( 'NONE', #27516, #10658, #6491, .T. ) ;
#9078=DIRECTION ( 'NONE',  ( -0.9893874368562772803, 0.1453014101478918851, -1.482692748682289258E-17 ) ) ;
#9079=ORIENTED_EDGE ( 'NONE', *, *, #1762, .T. ) ;
#9085=FACE_OUTER_BOUND ( 'NONE', #35536, .T. ) ;
#9086=EDGE_CURVE ( 'NONE', #17474, #997, #21740, .T. ) ;
#9087=FACE_OUTER_BOUND ( 'NONE', #4120, .T. ) ;
#9088=CARTESIAN_POINT ( 'NONE',  ( -24.28125388808335927, -13.17092994507341430, 62.83823998052931614 ) ) ;
#9089=EDGE_CURVE ( 'NONE', #13644, #42456, #16997, .T. ) ;
#9091=ORIENTED_EDGE ( 'NONE', *, *, #33760, .T. ) ;
#9092=ORIENTED_EDGE ( 'NONE', *, *, #15458, .T. ) ;
#9093=CARTESIAN_POINT ( 'NONE',  ( -10.99668346656864060, -11.04197136062318307, 60.72239829427679325 ) ) ;
#9095=DIRECTION ( 'NONE',  ( 1.235321093103353499E-06, 4.801898924785047334E-07, 0.9999999999991215915 ) ) ;
#9096=CARTESIAN_POINT ( 'NONE',  ( -11.09043784728536863, -11.82832424043013475, 71.37395526268804247 ) ) ;
#9098=VERTEX_POINT ( 'NONE', #20037 ) ;
#9099=CARTESIAN_POINT ( 'NONE',  ( -22.96375064570672819, -10.44813988596692589, 63.08658113699938497 ) ) ;
#9101=CARTESIAN_POINT ( 'NONE',  ( -15.55814167568544448, -21.55598949654579144, 72.33110090557599392 ) ) ;
#9103=EDGE_CURVE ( 'NONE', #8372, #11939, #43472, .T. ) ;
#9105=CARTESIAN_POINT ( 'NONE',  ( -24.84806299871600643, -14.18603056061780343, 69.69629353939886585 ) ) ;
#9107=ORIENTED_EDGE ( 'NONE', *, *, #2590, .F. ) ;
#9108=CARTESIAN_POINT ( 'NONE',  ( -24.42331094633779998, -14.99212722102677198, 59.43227208747884305 ) ) ;
#9109=CARTESIAN_POINT ( 'NONE',  ( -12.94457089969240648, -20.18822822247345883, 71.99756910775208496 ) ) ;
#9110=CARTESIAN_POINT ( 'NONE',  ( -23.77562434277295367, -17.86939608417919345, 59.01850491586762359 ) ) ;
#9111=ORIENTED_EDGE ( 'NONE', *, *, #1768, .F. ) ;
#9112=ADVANCED_FACE ( 'NONE', ( #1808 ), #258, .T. ) ;
#9113=CARTESIAN_POINT ( 'NONE',  ( -12.96596342764269316, -9.347744029417796696, 71.14925352873375175 ) ) ;
#9116=CARTESIAN_POINT ( 'NONE',  ( -10.42420801082433712, -14.84918507598050219, 71.51885965942804546 ) ) ;
#9118=CARTESIAN_POINT ( 'NONE',  ( -14.97188219925329378, -8.199429090594037461, 57.14999999999993463 ) ) ;
#9120=ORIENTED_EDGE ( 'NONE', *, *, #39823, .T. ) ;
#9121=CARTESIAN_POINT ( 'NONE',  ( -24.46479344033866710, -14.44719916248949154, 66.33292729247949637 ) ) ;
#9122=CARTESIAN_POINT ( 'NONE',  ( -14.91112529534803066, -8.221969756899694559, 57.13527940342243028 ) ) ;
#9123=DIRECTION ( 'NONE',  ( -0.6478992145799704616, 0.7617260713318516618, -1.927832152310573586E-08 ) ) ;
#9124=VERTEX_POINT ( 'NONE', #45904 ) ;
#9128=CARTESIAN_POINT ( 'NONE',  ( -22.33041777183100507, -20.41561037748852669, 62.34943743628787161 ) ) ;
#9129=ADVANCED_FACE ( 'NONE', ( #45674 ), #1562, .T. ) ;
#9131=CARTESIAN_POINT ( 'NONE',  ( -20.81696448553514855, -20.93198605141084201, 62.41471400679856885 ) ) ;
#9132=ORIENTED_EDGE ( 'NONE', *, *, #9605, .T. ) ;
#9133=ORIENTED_EDGE ( 'NONE', *, *, #8010, .T. ) ;
#9134=EDGE_CURVE ( 'NONE', #16415, #48249, #39232, .T. ) ;
#9135=CARTESIAN_POINT ( 'NONE',  ( -24.17166340479750630, -16.86472320484777043, 72.88335999016837263 ) ) ;
#9136=DIRECTION ( 'NONE',  ( -1.770046493635803029E-07, 8.183081527205841035E-08, 0.9999999999999809042 ) ) ;
#9138=FACE_OUTER_BOUND ( 'NONE', #619, .T. ) ;
#9142=CARTESIAN_POINT ( 'NONE',  ( -10.79685900591816683, -12.39371430582574796, 61.09853628380557922 ) ) ;
#9143=ORIENTED_EDGE ( 'NONE', *, *, #19917, .T. ) ;
#9144=B_SPLINE_CURVE_WITH_KNOTS ( 'NONE', 3,
 ( #32211, #28989, #43543, #36123, #9807, #2406, #13709, #14181, #28751, #43781 ),
 .UNSPECIFIED., .F., .F.,
 ( 4, 2, 2, 2, 4 ),
 ( 0.1272669073657799188, 0.2522669073462755485, 0.3772669073267712614, 0.5022669073072668633, 0.6272669072877625762 ),
 .UNSPECIFIED. ) ;
#9145=CARTESIAN_POINT ( 'NONE',  ( -24.00901317767523935, -17.32824147414624960, 69.42811846502259243 ) ) ;
#9146=CARTESIAN_POINT ( 'NONE',  ( -20.82057464141327330, -8.686965885571435564, 59.91295551501632133 ) ) ;
#9147=FACE_OUTER_BOUND ( 'NONE', #45776, .T. ) ;
#9149=EDGE_CURVE ( 'NONE', #31450, #6597, #1146, .T. ) ;
#9151=ORIENTED_EDGE ( 'NONE', *, *, #5756, .F. ) ;
#9153=EDGE_CURVE ( 'NONE', #25767, #946, #11198, .T. ) ;
#9155=FACE_OUTER_BOUND ( 'NONE', #11562, .T. ) ;
#9156=CARTESIAN_POINT ( 'NONE',  ( -21.74910605648477713, -9.305107492218610332, 63.20656180270096769 ) ) ;
#9157=( BOUNDED_CURVE ( )  B_SPLINE_CURVE ( 3, ( #43959, #25230, #40254, #13395 ),
 .UNSPECIFIED., .F., .F. ) 
 B_SPLINE_CURVE_WITH_KNOTS ( ( 4, 4 ),
 ( 1.570796326794896780, 1.780235837034217727 ),
 .UNSPECIFIED. ) 
 CURVE ( )  GEOMETRIC_REPRESENTATION_ITEM ( )  RATIONAL_B_SPLINE_CURVE ( ( 1.000000000000000000, 0.9963479302455154896, 0.9963479302455154896, 1.000000000000000000 ) ) 
 REPRESENTATION_ITEM ( '' )  );
#9158=B_SPLINE_CURVE_WITH_KNOTS ( 'NONE', 3,
 ( #19399, #37611, #44539, #10791, #19157, #26303, #34164, #34401, #7608, #697 ),
 .UNSPECIFIED., .F., .F.,
 ( 4, 2, 2, 2, 4 ),
 ( 0.000000000000000000, 0.2500000000000000000, 0.5000000000000000000, 0.7500000000000000000, 1.000000000000000000 ),
 .UNSPECIFIED. ) ;
#9162=AXIS2_PLACEMENT_3D ( 'NONE', #17903, #33167, #47967 ) ;
#9164=ORIENTED_EDGE ( 'NONE', *, *, #12671, .T. ) ;
#9165=CARTESIAN_POINT ( 'NONE',  ( -20.13271805750754950, -8.299978134201072777, 70.53628287813307907 ) ) ;
#9166=PLANE ( 'NONE',  #40671 ) ;
#9167=ORIENTED_EDGE ( 'NONE', *, *, #48459, .F. ) ;
#9168=CARTESIAN_POINT ( 'NONE',  ( -10.79232760089606735, -12.56855635920591219, 57.40145450620173051 ) ) ;
#9169=ORIENTED_EDGE ( 'NONE', *, *, #7171, .F. ) ;
#9170=( BOUNDED_CURVE ( )  B_SPLINE_CURVE ( 3, ( #2878, #9810, #6101, #24822 ),
 .UNSPECIFIED., .F., .F. ) 
 B_SPLINE_CURVE_WITH_KNOTS ( ( 4, 4 ),
 ( 0.9074455897393666204, 1.000000000000000000 ),
 .UNSPECIFIED. ) 
 CURVE ( )  GEOMETRIC_REPRESENTATION_ITEM ( )  RATIONAL_B_SPLINE_CURVE ( ( 0.6983129098261039447, 0.7760317562607076392, 0.8765941196520062872, 1.000000000000000000 ) ) 
 REPRESENTATION_ITEM ( '' )  );
#9171=CARTESIAN_POINT ( 'NONE',  ( -12.01648241349452917, -10.28590705807702932, 67.49896869922172016 ) ) ;
#9172=ORIENTED_EDGE ( 'NONE', *, *, #4814, .F. ) ;
#9174=CARTESIAN_POINT ( 'NONE',  ( -16.84865286310842336, -21.83598151670433296, 68.98088545748413480 ) ) ;
#9176=VERTEX_POINT ( 'NONE', #44168 ) ;
#9177=CARTESIAN_POINT ( 'NONE',  ( -13.60238606012557483, -8.884930320952351579, 56.96967755506135234 ) ) ;
#9179=LINE ( 'NONE', #34341, #7726 ) ;
#9180=CARTESIAN_POINT ( 'NONE',  ( -21.89264518680100835, -20.26253109894388160, 58.77915004610762395 ) ) ;
#9181=CARTESIAN_POINT ( 'NONE',  ( -15.49415775405465645, -8.028509947901662613, 74.37985659017797957 ) ) ;
#9182=CYLINDRICAL_SURFACE ( 'NONE', #8030, 0.1499999999999962752 ) ;
#9183=CARTESIAN_POINT ( 'NONE',  ( -10.40425584863931263, -17.30445325246355992, 61.33460017742925174 ) ) ;
#9184=ORIENTED_EDGE ( 'NONE', *, *, #33343, .T. ) ;
#9185=( BOUNDED_SURFACE ( )  B_SPLINE_SURFACE ( 3, 1, ( 
 ( #34529, #27873 ),
 ( #11901, #46608 ),
 ( #46111, #810 ),
 ( #35012, #12370 ),
 ( #12615, #31330 ),
 ( #15815, #23228 ),
 ( #9174, #30624 ) ),
 .UNSPECIFIED., .T., .F., .F. ) 
 B_SPLINE_SURFACE_WITH_KNOTS ( ( 4, 3, 4 ),
 ( 2, 2 ),
 ( 0.000000000000000000, 0.5000000000000000000, 1.000000000000000000 ),
 ( 0.000000000000000000, 1.000000000000000000 ),
 .UNSPECIFIED. ) 
 GEOMETRIC_REPRESENTATION_ITEM ( )  RATIONAL_B_SPLINE_SURFACE ( (
 ( 1.000000000000000000, 1.000000000000000000),
 ( 0.3333333333333335369, 0.3333333333333330373),
 ( 0.3333333333333335369, 0.3333333333333330373),
 ( 1.000000000000000000, 1.000000000000000000),
 ( 0.3333333333333333703, 0.3333333333333333703),
 ( 0.3333333333333333703, 0.3333333333333333703),
 ( 1.000000000000000000, 1.000000000000000000) ) ) 
 REPRESENTATION_ITEM ( '' )  SURFACE ( )  );
#9186=LINE ( 'NONE', #20746, #32107 ) ;
#9187=CARTESIAN_POINT ( 'NONE',  ( -24.86367705086121660, -14.41520995907644753, 66.38281513983412196 ) ) ;
#9188=CARTESIAN_POINT ( 'NONE',  ( -9.974456273375457371, -14.72748566909688073, 71.51278126739182994 ) ) ;
#9189=CARTESIAN_POINT ( 'NONE',  ( -14.11401878847811986, -20.97727922448205007, 72.22607667752819793 ) ) ;
#9191=VERTEX_POINT ( 'NONE', #36008 ) ;
#9192=ADVANCED_FACE ( 'NONE', ( #9926 ), #21943, .T. ) ;
#9193=CARTESIAN_POINT ( 'NONE',  ( -22.67064388239395711, -10.17514023627220965, 66.76855582679374379 ) ) ;
#9194=FACE_OUTER_BOUND ( 'NONE', #329, .T. ) ;
#9195=VERTEX_POINT ( 'NONE', #17043 ) ;
#9196=DIRECTION ( 'NONE',  ( 0.9325317756203292952, -0.3459670625490730012, 0.1033986416233858563 ) ) ;
#9197=CARTESIAN_POINT ( 'NONE',  ( -23.62594491300536959, -11.45603751788689095, 66.70742424642772050 ) ) ;
#9198=CARTESIAN_POINT ( 'NONE',  ( -11.62870111763649028, -18.82374159213384601, 68.21689662501481166 ) ) ;
#9199=CARTESIAN_POINT ( 'NONE',  ( -22.71059208588729561, -10.14448404190931186, 70.02650598627910483 ) ) ;
#9200=CARTESIAN_POINT ( 'NONE',  ( -14.60783614669699304, -21.70648650955843806, 58.35113213314874514 ) ) ;
#9202=CARTESIAN_POINT ( 'NONE',  ( -22.47245519635065492, -19.73066437834766873, 72.65872596779033188 ) ) ;
#9203=VECTOR ( 'NONE', #44875, 1000.000000000000114 ) ;
#9205=CARTESIAN_POINT ( 'NONE',  ( -24.03011946566357437, -11.36467352769893324, 66.54497619818440057 ) ) ;
#9206=B_SPLINE_CURVE_WITH_KNOTS ( 'NONE', 3,
 ( #43823, #5900, #24379, #9841, #32712, #47738, #39867, #35918, #6139, #21164 ),
 .UNSPECIFIED., .F., .F.,
 ( 4, 2, 2, 2, 4 ),
 ( 0.1272669073658336814, 0.2522669073487979752, 0.3772669073317622690, 0.5022669073147265628, 0.6272669072976908566 ),
 .UNSPECIFIED. ) ;
#9207=ORIENTED_EDGE ( 'NONE', *, *, #10810, .F. ) ;
#9208=CARTESIAN_POINT ( 'NONE',  ( -17.15293984484763712, -7.364064364366409876, 70.53389935397558475 ) ) ;
#9209=CARTESIAN_POINT ( 'NONE',  ( -13.23553521163189828, -8.648101578109386622, 60.63288603205860738 ) ) ;
#9210=CARTESIAN_POINT ( 'NONE',  ( -21.84079810191280657, -9.314188493807273872, 63.49153755726582915 ) ) ;
#9211=CARTESIAN_POINT ( 'NONE',  ( -23.27284462870851911, -18.74605969774991010, 66.10917289053097079 ) ) ;
#9213=VERTEX_POINT ( 'NONE', #21726 ) ;
#9216=ADVANCED_FACE ( 'NONE', ( #47828 ), #2763, .T. ) ;
#9217=EDGE_CURVE ( 'NONE', #16722, #30190, #24013, .T. ) ;
#9218=CARTESIAN_POINT ( 'NONE',  ( -20.31413516131974717, -8.378470924821744603, 67.06632013881642251 ) ) ;
#9220=CARTESIAN_POINT ( 'NONE',  ( -11.79630000206883977, -19.05592701419838519, 71.97213747039440079 ) ) ;
#9221=EDGE_CURVE ( 'NONE', #30692, #29219, #32315, .T. ) ;
#9223=LINE ( 'NONE', #16824, #932 ) ;
#9224=CARTESIAN_POINT ( 'NONE',  ( -12.23301264461619553, -10.03852782535897958, 60.84446034103241630 ) ) ;
#9225=CARTESIAN_POINT ( 'NONE',  ( -19.94917705995926482, -8.226604131702123013, 74.00624557436877637 ) ) ;
#9226=CARTESIAN_POINT ( 'NONE',  ( -24.46479343890040425, -14.44719913075708995, 66.48292729247951627 ) ) ;
#9227=ORIENTED_EDGE ( 'NONE', *, *, #35121, .F. ) ;
#9228=CARTESIAN_POINT ( 'NONE',  ( -21.95395705827280963, -8.894478678276469097, 66.91795930326043162 ) ) ;
#9233=CARTESIAN_POINT ( 'NONE',  ( -12.36794899618824317, -19.72224014812425708, 61.69678633597965955 ) ) ;
#9234=CARTESIAN_POINT ( 'NONE',  ( -12.26902364965855519, -19.54473725125994221, 57.92682373989410394 ) ) ;
#9237=EDGE_CURVE ( 'NONE', #10986, #36933, #13429, .T. ) ;
#9238=CYLINDRICAL_SURFACE ( 'NONE', #40713, 0.1500000000000084044 ) ;
#9241=CARTESIAN_POINT ( 'NONE',  ( -11.06285897508056593, -17.73077265676491265, 71.85252885412863577 ) ) ;
#9242=VERTEX_POINT ( 'NONE', #3254 ) ;
#9243=FACE_OUTER_BOUND ( 'NONE', #27968, .T. ) ;
#9245=DIRECTION ( 'NONE',  ( 1.078708504465006897E-05, 7.367657514171588156E-06, 0.9999999999146782503 ) ) ;
#9246=FACE_BOUND ( 'NONE', #28492, .T. ) ;
#9247=CARTESIAN_POINT ( 'NONE',  ( -19.69746735473979271, -8.127384799358436496, 73.87663944647505332 ) ) ;
#9249=CARTESIAN_POINT ( 'NONE',  ( -16.02567528876233993, -7.491550372963335924, 63.92656979170173059 ) ) ;
#9250=VERTEX_POINT ( 'NONE', #48303 ) ;
#9254=EDGE_LOOP ( 'NONE', ( #35476, #7456, #18874, #32927 ) ) ;
#9255=CARTESIAN_POINT ( 'NONE',  ( -20.03744868119640898, -21.78660147720172802, 69.04827188316701836 ) ) ;
#9256=EDGE_LOOP ( 'NONE', ( #25208, #21883 ) ) ;
#9257=VERTEX_POINT ( 'NONE', #29600 ) ;
#9260=CARTESIAN_POINT ( 'NONE',  ( -23.19494370299929287, -18.77118727246694263, 65.82389430425217824 ) ) ;
#9262=CARTESIAN_POINT ( 'NONE',  ( -24.71482052093760373, -13.27635576790630090, 59.54080713533480917 ) ) ;
#9263=CARTESIAN_POINT ( 'NONE',  ( -23.46218685299048801, -18.44850610243709710, 73.06368207112421942 ) ) ;
#9267=ORIENTED_EDGE ( 'NONE', *, *, #20686, .F. ) ;
#9269=EDGE_CURVE ( 'NONE', #33912, #47972, #37030, .T. ) ;
#9270=CARTESIAN_POINT ( 'NONE',  ( -11.35824856342118139, -11.21643317443627375, 60.97885780702566194 ) ) ;
#9271=CARTESIAN_POINT ( 'NONE',  ( -14.90981300391231024, -21.39562377109201208, 61.63600440604547970 ) ) ;
#9273=CARTESIAN_POINT ( 'NONE',  ( -23.27033594065426314, -18.65917932524403966, 65.89677377228576916 ) ) ;
#9277=ORIENTED_EDGE ( 'NONE', *, *, #45851, .T. ) ;
#9278=CARTESIAN_POINT ( 'NONE',  ( -23.09439617342594886, -10.70187492079748282, 59.71276609431315308 ) ) ;
#9279=PLANE ( 'NONE',  #7224 ) ;
#9280=EDGE_CURVE ( 'NONE', #5788, #26302, #35153, .T. ) ;
#9281=CARTESIAN_POINT ( 'NONE',  ( -24.44689184067228638, -14.18710713894228270, 69.93803194250308763 ) ) ;
#9283=VERTEX_POINT ( 'NONE', #48072 ) ;
#9286=B_SPLINE_CURVE_WITH_KNOTS ( 'NONE', 1,
 ( #17072, #5786 ),
 .UNSPECIFIED., .F., .F.,
 ( 2, 2 ),
 ( 0.000000000000000000, 1.000000000000000000 ),
 .UNSPECIFIED. ) ;
#9287=CARTESIAN_POINT ( 'NONE',  ( -10.98710762053434387, -12.05856205565705785, 74.63128435701548824 ) ) ;
#9288=CARTESIAN_POINT ( 'NONE',  ( -24.47380067112417734, -14.88812224869491807, 59.24859996059156231 ) ) ;
#9289=ADVANCED_FACE ( 'NONE', ( #11373 ), #22217, .T. ) ;
#9290=ORIENTED_EDGE ( 'NONE', *, *, #32043, .T. ) ;
#9292=FACE_OUTER_BOUND ( 'NONE', #29945, .T. ) ;
#9294=CARTESIAN_POINT ( 'NONE',  ( -17.73278501768472992, -7.757988417614677168, 67.16472282884072342 ) ) ;
#9295=CARTESIAN_POINT ( 'NONE',  ( -17.98078221672114552, -21.78831896835910698, 65.41702429779255112 ) ) ;
#9299=AXIS2_PLACEMENT_3D ( 'NONE', #37062, #18589, #47922 ) ;
#9301=CARTESIAN_POINT ( 'NONE',  ( -23.46260370332431577, -11.17067683354235719, 73.66193301755811262 ) ) ;
#9302=FACE_OUTER_BOUND ( 'NONE', #15295, .T. ) ;
#9303=ORIENTED_EDGE ( 'NONE', *, *, #1565, .F. ) ;
#9305=CARTESIAN_POINT ( 'NONE',  ( -21.85024167232948855, -20.23279819819498115, 58.78059551072086464 ) ) ;
#9306=FACE_OUTER_BOUND ( 'NONE', #25238, .T. ) ;
#9307=LINE ( 'NONE', #5369, #47128 ) ;
#9309=CARTESIAN_POINT ( 'NONE',  ( -10.60635910294346651, -17.81289749453643978, 71.82364097624930821 ) ) ;
#9311=CARTESIAN_POINT ( 'NONE',  ( -20.88128654865952427, -21.40856141908871635, 58.68829242887799325 ) ) ;
#9312=( BOUNDED_SURFACE ( )  B_SPLINE_SURFACE ( 3, 1, ( 
 ( #6629, #47742 ),
 ( #28058, #25104 ),
 ( #10332, #13512 ),
 ( #6145, #21645 ),
 ( #21167, #36633 ),
 ( #13030, #25343 ),
 ( #2915, #2449 ) ),
 .UNSPECIFIED., .T., .F., .F. ) 
 B_SPLINE_SURFACE_WITH_KNOTS ( ( 4, 3, 4 ),
 ( 2, 2 ),
 ( 0.000000000000000000, 0.5000000000000000000, 1.000000000000000000 ),
 ( 0.000000000000000000, 1.000000000000000000 ),
 .UNSPECIFIED. ) 
 GEOMETRIC_REPRESENTATION_ITEM ( )  RATIONAL_B_SPLINE_SURFACE ( (
 ( 1.000000000000000000, 1.000000000000000000),
 ( 0.3333333333333335369, 0.3333333333333330373),
 ( 0.3333333333333335369, 0.3333333333333330373),
 ( 1.000000000000000000, 1.000000000000000000),
 ( 0.3333333333333333703, 0.3333333333333333703),
 ( 0.3333333333333333703, 0.3333333333333333703),
 ( 1.000000000000000000, 1.000000000000000000) ) ) 
 REPRESENTATION_ITEM ( '' )  SURFACE ( )  );
#9313=CARTESIAN_POINT ( 'NONE',  ( -23.45312108354205094, -19.18567332746851406, 62.55395650355025339 ) ) ;
#9316=CARTESIAN_POINT ( 'NONE',  ( -15.48424252676649182, -21.53505049348036948, 72.34575460973682937 ) ) ;
#9317=VERTEX_POINT ( 'NONE', #33506 ) ;
#9319=CARTESIAN_POINT ( 'NONE',  ( -24.08907123645992243, -11.48026457312919391, 63.13713595337925000 ) ) ;
#9325=CARTESIAN_POINT ( 'NONE',  ( -12.29706043583926345, -19.57525793408492731, 58.22682366956317424 ) ) ;
#9326=CARTESIAN_POINT ( 'NONE',  ( -18.62171053289692324, -7.456047208065794685, 74.03402725549381103 ) ) ;
#9327=( BOUNDED_CURVE ( )  B_SPLINE_CURVE ( 3, ( #17424, #31964, #43551, #24100 ),
 .UNSPECIFIED., .F., .F. ) 
 B_SPLINE_CURVE_WITH_KNOTS ( ( 4, 4 ),
 ( 0.5000000000000000000, 0.9074455897393693959 ),
 .UNSPECIFIED. ) 
 CURVE ( )  GEOMETRIC_REPRESENTATION_ITEM ( )  RATIONAL_B_SPLINE_CURVE ( ( 1.000000000000019318, 0.4567392136813193115, 0.3561768502900120592, 0.6983129098261183776 ) ) 
 REPRESENTATION_ITEM ( '' )  );
#9329=EDGE_LOOP ( 'NONE', ( #1618, #24797 ) ) ;
#9330=ORIENTED_EDGE ( 'NONE', *, *, #13611, .F. ) ;
#9331=DIRECTION ( 'NONE',  ( 0.6408936281290996684, 0.7676297007174210929, 4.260501105223829223E-08 ) ) ;
#9333=CARTESIAN_POINT ( 'NONE',  ( -21.01124108229941001, -20.87838065962769463, 65.88453944495783787 ) ) ;
#9335=CARTESIAN_POINT ( 'NONE',  ( -19.67760665824181388, -21.48965406232008490, 65.75014118398131302 ) ) ;
#9336=CARTESIAN_POINT ( 'NONE',  ( -19.98813040044048606, -21.37641421727040125, 72.40478737316021807 ) ) ;
#9340=EDGE_LOOP ( 'NONE', ( #3849, #22207, #12049, #29417, #46761 ) ) ;
#9342=CARTESIAN_POINT ( 'NONE',  ( -10.21398995055970893, -12.93320293812463007, 67.87685812613038649 ) ) ;
#9344=FACE_OUTER_BOUND ( 'NONE', #4526, .T. ) ;
#9347=EDGE_CURVE ( 'NONE', #32374, #40830, #22713, .T. ) ;
#9349=CARTESIAN_POINT ( 'NONE',  ( -23.59167294107103530, -11.49507482056193197, 70.08137858863322833 ) ) ;
#9351=CARTESIAN_POINT ( 'NONE',  ( -24.80769047312930553, -15.80232199467591947, 69.71802767292497549 ) ) ;
#9352=CARTESIAN_POINT ( 'NONE',  ( -18.90996118681096405, -7.968724231816139536, 67.20071784163268092 ) ) ;
#9353=CARTESIAN_POINT ( 'NONE',  ( -22.66918927228052283, -20.09991590937644901, 69.37406776248666063 ) ) ;
#9354=EDGE_CURVE ( 'NONE', #4066, #31755, #27271, .T. ) ;
#9355=CARTESIAN_POINT ( 'NONE',  ( -19.05654524761795443, -8.000564681511368903, 67.01144978564013854 ) ) ;
#9356=ORIENTED_EDGE ( 'NONE', *, *, #6211, .T. ) ;
#9357=DIRECTION ( 'NONE',  ( -3.549360974554993999E-17, 6.371834667797927122E-18, 1.000000000000000000 ) ) ;
#9359=DIRECTION ( 'NONE',  ( -2.723496480336737305E-06, -1.584719851758938193E-07, -0.9999999999962786434 ) ) ;
#9360=DIRECTION ( 'NONE',  ( 0.9163203205182085531, 0.4004460890125010053, -2.380681616944615956E-09 ) ) ;
#9366=CARTESIAN_POINT ( 'NONE',  ( -13.54823245630066175, -20.69819609872914157, 61.81646323537678001 ) ) ;
#9369=CARTESIAN_POINT ( 'NONE',  ( -10.89683688409922269, -17.33836331364876315, 64.92739378817780960 ) ) ;
#9371=CARTESIAN_POINT ( 'NONE',  ( -23.89126246139208121, -17.48811810169603831, 62.54649106506063561 ) ) ;
#9373=CARTESIAN_POINT ( 'NONE',  ( -11.47140389976542529, -10.32934621678965037, 74.69531023250135604 ) ) ;
#9374=CARTESIAN_POINT ( 'NONE',  ( -24.02655296236175175, -11.35792967378293916, 66.53719098615387395 ) ) ;
#9375=CARTESIAN_POINT ( 'NONE',  ( -20.78261577219678813, -20.95102001000085323, 62.41471427792803439 ) ) ;
#9376=ORIENTED_EDGE ( 'NONE', *, *, #43442, .T. ) ;
#9377=VERTEX_POINT ( 'NONE', #41406 ) ;
#9378=CARTESIAN_POINT ( 'NONE',  ( -22.67332665777710332, -19.52078802573384664, 72.85220588380256856 ) ) ;
#9379=FACE_OUTER_BOUND ( 'NONE', #36152, .T. ) ;
#9383=CARTESIAN_POINT ( 'NONE',  ( -23.83096212394601565, -11.00696669973021713, 73.52339839455761705 ) ) ;
#9384=ADVANCED_FACE ( 'NONE', ( #36873 ), #47731, .T. ) ;
#9386=EDGE_LOOP ( 'NONE', ( #39903, #12423 ) ) ;
#9387=CARTESIAN_POINT ( 'NONE',  ( -16.79181145072023185, -21.83380975027498039, 65.11075561446135396 ) ) ;
#9388=CARTESIAN_POINT ( 'NONE',  ( -19.43707224927095822, -8.044379180677138308, 63.57522333692026706 ) ) ;
#9389=CARTESIAN_POINT ( 'NONE',  ( -16.19814381282456495, -21.75179583453235210, 58.58585572026734667 ) ) ;
#9390=DIRECTION ( 'NONE',  ( 0.8858372764600319638, 0.4639960340712761533, -4.734734194490108743E-17 ) ) ;
#9392=EDGE_CURVE ( 'NONE', #8331, #38602, #13728, .T. ) ;
#9396=CARTESIAN_POINT ( 'NONE',  ( -10.83683317046381234, -12.44108562964681219, 57.62857332099802932 ) ) ;
#9397=CARTESIAN_POINT ( 'NONE',  ( -22.57847124554494300, -10.07283119406621452, 70.29713180003925288 ) ) ;
#9398=ADVANCED_FACE ( 'NONE', ( #25570 ), #25333, .T. ) ;
#9400=CARTESIAN_POINT ( 'NONE',  ( -10.98483237281456404, -18.55601372762673407, 57.90690960667243559 ) ) ;
#9401=( BOUNDED_SURFACE ( )  B_SPLINE_SURFACE ( 3, 1, ( 
 ( #33450, #18688 ),
 ( #25131, #44105 ),
 ( #18202, #48014 ),
 ( #33210, #10358 ),
 ( #40149, #36426 ),
 ( #7146, #25370 ),
 ( #6414, #11078 ) ),
 .UNSPECIFIED., .T., .F., .F. ) 
 B_SPLINE_SURFACE_WITH_KNOTS ( ( 4, 3, 4 ),
 ( 2, 2 ),
 ( 0.000000000000000000, 0.5000000000000000000, 1.000000000000000000 ),
 ( 0.000000000000000000, 1.000000000000000000 ),
 .UNSPECIFIED. ) 
 GEOMETRIC_REPRESENTATION_ITEM ( )  RATIONAL_B_SPLINE_SURFACE ( (
 ( 1.000000000000000000, 1.000000000000000000),
 ( 0.3333333333333335369, 0.3333333333333330373),
 ( 0.3333333333333335369, 0.3333333333333330373),
 ( 1.000000000000000000, 1.000000000000000000),
 ( 0.3333333333333333703, 0.3333333333333333703),
 ( 0.3333333333333333703, 0.3333333333333333703),
 ( 1.000000000000000000, 1.000000000000000000) ) ) 
 REPRESENTATION_ITEM ( '' )  SURFACE ( )  );
#9402=ORIENTED_EDGE ( 'NONE', *, *, #25351, .F. ) ;
#9404=CARTESIAN_POINT ( 'NONE',  ( -21.95523233784883033, -8.895446131873137929, 66.77654700642760588 ) ) ;
#9405=EDGE_CURVE ( 'NONE', #31463, #47353, #30459, .T. ) ;
#9406=CARTESIAN_POINT ( 'NONE',  ( -10.38423141237398895, -15.23952324640539935, 57.98281521108167880 ) ) ;
#9408=CARTESIAN_POINT ( 'NONE',  ( -11.42787535746950667, -18.52272177604094239, 57.69225786326394001 ) ) ;
#9410=ADVANCED_FACE ( 'NONE', ( #10072 ), #9607, .T. ) ;
#9411=CARTESIAN_POINT ( 'NONE',  ( -10.46342116995388061, -14.06823698635533759, 57.55710969353301465 ) ) ;
#9412=EDGE_LOOP ( 'NONE', ( #19311, #46300 ) ) ;
#9413=CARTESIAN_POINT ( 'NONE',  ( -21.91761355075745854, -8.866908028128893449, 66.86138764422409508 ) ) ;
#9416=ORIENTED_EDGE ( 'NONE', *, *, #44339, .T. ) ;
#9419=CARTESIAN_POINT ( 'NONE',  ( -21.04131466462198574, -20.86482832106620933, 62.11471242509498580 ) ) ;
#9421=CARTESIAN_POINT ( 'NONE',  ( -17.85555652284939043, -7.772123375420258107, 60.09532845646905486 ) ) ;
#9423=CARTESIAN_POINT ( 'NONE',  ( -22.19982498210932675, -20.00606685933203366, 58.92009921125114857 ) ) ;
#9424=EDGE_CURVE ( 'NONE', #36602, #32895, #18141, .T. ) ;
#9425=CARTESIAN_POINT ( 'NONE',  ( -19.80301194551662647, -21.44571530912114099, 68.93482476707502826 ) ) ;
#9427=CARTESIAN_POINT ( 'NONE',  ( -10.39215589072981416, -14.30487699944780289, 64.68803863382906627 ) ) ;
#9428=ORIENTED_EDGE ( 'NONE', *, *, #11661, .F. ) ;
#9429=FACE_OUTER_BOUND ( 'NONE', #24035, .T. ) ;
#9430=ADVANCED_FACE ( 'NONE', ( #17195 ), #17681, .T. ) ;
#9431=DIRECTION ( 'NONE',  ( 0.9466432954593471116, 0.3222832157619555660, 8.771047036255756069E-09 ) ) ;
#9432=CARTESIAN_POINT ( 'NONE',  ( -24.30112618867181240, -13.25578303422174997, 59.64795780745660636 ) ) ;
#9433=CARTESIAN_POINT ( 'NONE',  ( -23.58616457878146377, -18.99640866789479432, 66.00884704819274873 ) ) ;
#9434=CARTESIAN_POINT ( 'NONE',  ( -19.94963503706584973, -21.81807911492407825, 69.03458852897473719 ) ) ;
#9435=ADVANCED_FACE ( 'NONE', ( #36151 ), #2439, .F. ) ;
#9437=ORIENTED_EDGE ( 'NONE', *, *, #45815, .F. ) ;
#9440=CARTESIAN_POINT ( 'NONE',  ( -20.75354924259569245, -21.52967727414722532, 53.49999999999994316 ) ) ;
#9441=VERTEX_POINT ( 'NONE', #44069 ) ;
#9442=CARTESIAN_POINT ( 'NONE',  ( -11.37476892658000160, -19.15884210479704208, 68.33034228280476441 ) ) ;
#9443=DIRECTION ( 'NONE',  ( -0.2737502900231349456, -0.9618007999124592589, 5.400150802763565238E-08 ) ) ;
#9444=CARTESIAN_POINT ( 'NONE',  ( -11.60526899143904345, -18.79015832504765626, 68.23161775275829655 ) ) ;
#9446=LINE ( 'NONE', #24937, #25032 ) ;
#9448=CARTESIAN_POINT ( 'NONE',  ( -23.71873335871097410, -11.74668215431234586, 62.95218284853060453 ) ) ;
#9449=AXIS2_PLACEMENT_3D ( 'NONE', #47652, #21559, #17106 ) ;
#9451=CARTESIAN_POINT ( 'NONE',  ( -22.11565237232494496, -20.07634252930852981, 58.97262747901392288 ) ) ;
#9452=ORIENTED_EDGE ( 'NONE', *, *, #22163, .T. ) ;
#9453=DIRECTION ( 'NONE',  ( -0.7489133456531319455, -0.6626679415081375701, 6.686399169904807035E-09 ) ) ;
#9454=AXIS2_PLACEMENT_3D ( 'NONE', #14308, #58, #29358 ) ;
#9455=CARTESIAN_POINT ( 'NONE',  ( -13.37043874031056490, -9.101841881849773941, 63.92563223505148784 ) ) ;
#9456=CARTESIAN_POINT ( 'NONE',  ( -24.20371252810814866, -12.87440185077122834, 66.58774614429587757 ) ) ;
#9457=( BOUNDED_CURVE ( )  B_SPLINE_CURVE ( 3, ( #30063, #33464, #22923, #38148 ),
 .UNSPECIFIED., .F., .F. ) 
 B_SPLINE_CURVE_WITH_KNOTS ( ( 4, 4 ),
 ( 0.4074455897393656212, 0.5000000000000000000 ),
 .UNSPECIFIED. ) 
 CURVE ( )  GEOMETRIC_REPRESENTATION_ITEM ( )  RATIONAL_B_SPLINE_CURVE ( ( 0.6983129098260936196, 0.7760317562606803277, 0.8765941196519769774, 0.9999999999999708011 ) ) 
 REPRESENTATION_ITEM ( '' )  );
#9458=DIRECTION ( 'NONE',  ( 0.3667195576449455152, -0.9303315355510074491, -1.591455084066187253E-08 ) ) ;
#9460=ORIENTED_EDGE ( 'NONE', *, *, #22169, .T. ) ;
#9465=B_SPLINE_CURVE_WITH_KNOTS ( 'NONE', 3,
 ( #6300, #42997, #47429, #9273, #31678, #20354, #46467, #46933, #32409, #28476 ),
 .UNSPECIFIED., .F., .F.,
 ( 4, 2, 2, 2, 4 ),
 ( 0.000000000000000000, 0.2500000000000000000, 0.5000000000000000000, 0.7500000000000000000, 1.000000000000000000 ),
 .UNSPECIFIED. ) ;
#9466=CARTESIAN_POINT ( 'NONE',  ( -12.42812249138612835, -20.42751868149720096, 53.76227901944322696 ) ) ;
#9467=CARTESIAN_POINT ( 'NONE',  ( -12.09966231065201825, -10.17612992894743229, 71.11326093460978370 ) ) ;
#9469=EDGE_CURVE ( 'NONE', #48485, #9377, #40787, .T. ) ;
#9470=CARTESIAN_POINT ( 'NONE',  ( -14.15319410108614129, -8.620341405635986831, 70.80245711640594664 ) ) ;
#9471=CYLINDRICAL_SURFACE ( 'NONE', #8128, 0.1500000000000067668 ) ;
#9474=CARTESIAN_POINT ( 'NONE',  ( -21.11381757457507646, -20.75781470100932680, 65.69339893210704417 ) ) ;
#9475=AXIS2_PLACEMENT_3D ( 'NONE', #29391, #15078, #7487 ) ;
#9476=CYLINDRICAL_SURFACE ( 'NONE', #40625, 0.1500000000000049349 ) ;
#9477=VERTEX_POINT ( 'NONE', #24852 ) ;
#9478=FACE_OUTER_BOUND ( 'NONE', #17649, .T. ) ;
#9479=VECTOR ( 'NONE', #1631, 1000.000000000000227 ) ;
#9480=CARTESIAN_POINT ( 'NONE',  ( -11.92656900268342035, -15.22777080260183169, 53.88362224778186516 ) ) ;
#9481=( BOUNDED_CURVE ( )  B_SPLINE_CURVE ( 3, ( #36606, #2887, #47959, #29735 ),
 .UNSPECIFIED., .F., .F. ) 
 B_SPLINE_CURVE_WITH_KNOTS ( ( 4, 4 ),
 ( 0.5000000000000000000, 0.9074455897393665094 ),
 .UNSPECIFIED. ) 
 CURVE ( )  GEOMETRIC_REPRESENTATION_ITEM ( )  RATIONAL_B_SPLINE_CURVE ( ( 0.9999999999999996669, 0.4567392136813316350, 0.3561768502900302114, 0.6983129098260952849 ) ) 
 REPRESENTATION_ITEM ( '' )  );
#9482=EDGE_LOOP ( 'NONE', ( #41171, #19535, #8400, #28358, #43335 ) ) ;
#9484=PLANE ( 'NONE',  #641 ) ;
#9485=EDGE_LOOP ( 'NONE', ( #655, #1742 ) ) ;
#9486=CARTESIAN_POINT ( 'NONE',  ( -17.84905175390062837, -22.24782703323402444, 58.51898120184483076 ) ) ;
#9487=CARTESIAN_POINT ( 'NONE',  ( -19.57699614054808634, -21.94144247634149281, 62.17999043330664222 ) ) ;
#9490=CARTESIAN_POINT ( 'NONE',  ( -11.22844613476422282, -11.44458948612160221, 64.43409918096024569 ) ) ;
#9491=ORIENTED_EDGE ( 'NONE', *, *, #15666, .T. ) ;
#9492=DIRECTION ( 'NONE',  ( -6.446466763177039895E-06, 1.047023821809670710E-05, 0.9999999999244085780 ) ) ;
#9494=CARTESIAN_POINT ( 'NONE',  ( -16.98991614605047218, -22.24663000551990777, 72.35038637723081933 ) ) ;
#9497=EDGE_CURVE ( 'NONE', #31797, #9250, #3393, .T. ) ;
#9500=CARTESIAN_POINT ( 'NONE',  ( -11.44117212203710032, -11.17454305509652634, 60.69502469113133714 ) ) ;
#9502=DIRECTION ( 'NONE',  ( -0.09077643883959131410, 0.9958712959773468043, 4.338678762321648664E-08 ) ) ;
#9503=EDGE_LOOP ( 'NONE', ( #22385, #32622, #21112, #18164, #20398 ) ) ;
#9505=CARTESIAN_POINT ( 'NONE',  ( -14.30193168523162761, -8.044807666815707137, 67.42121571432790006 ) ) ;
#9506=CARTESIAN_POINT ( 'NONE',  ( -24.07704370891654122, -17.14264987453632827, 72.89808101046213551 ) ) ;
#9507=EDGE_LOOP ( 'NONE', ( #178, #29217, #29700, #47309, #37899 ) ) ;
#9508=CARTESIAN_POINT ( 'NONE',  ( -15.06493049075016977, -21.45670177733324380, 68.87592999875900546 ) ) ;
#9512=CARTESIAN_POINT ( 'NONE',  ( -18.81428322969336620, -7.490049256398734201, 70.47093791628151394 ) ) ;
#9513=DIRECTION ( 'NONE',  ( -0.3996021513128670266, -0.9166886716143755054, -9.834836654444679756E-09 ) ) ;
#9517=VECTOR ( 'NONE', #43744, 1000.000000000000000 ) ;
#9518=ORIENTED_EDGE ( 'NONE', *, *, #44068, .F. ) ;
#9519=ORIENTED_EDGE ( 'NONE', *, *, #42342, .T. ) ;
#9521=EDGE_CURVE ( 'NONE', #1086, #39806, #36624, .T. ) ;
#9522=DIRECTION ( 'NONE',  ( -2.161108586189011127E-06, -4.147204437186874712E-06, -0.9999999999890651914 ) ) ;
#9525=CARTESIAN_POINT ( 'NONE',  ( -11.79630000206883977, -19.05592701419838519, 71.97213747039440079 ) ) ;
#9527=ORIENTED_EDGE ( 'NONE', *, *, #44583, .F. ) ;
#9528=CARTESIAN_POINT ( 'NONE',  ( -12.27729947935473653, -9.991218615320079266, 60.85918086709605745 ) ) ;
#9529=DIRECTION ( 'NONE',  ( 0.1464579420318390945, -0.9892168979631278392, -7.284849527857772841E-08 ) ) ;
#9531=LINE ( 'NONE', #6551, #9517 ) ;
#9532=ORIENTED_EDGE ( 'NONE', *, *, #19917, .F. ) ;
#9533=B_SPLINE_CURVE_WITH_KNOTS ( 'NONE', 3,
 ( #25301, #7073, #10030, #17151, #13934, #6338, #10751, #24813, #32674, #25056 ),
 .UNSPECIFIED., .F., .F.,
 ( 4, 2, 2, 2, 4 ),
 ( 0.6272669072877784524, 0.7522669073072748569, 0.8772669073267711504, 1.002266907346267555, 1.127266907365763959 ),
 .UNSPECIFIED. ) ;
#9534=CARTESIAN_POINT ( 'NONE',  ( -11.59752488401249160, -18.69167939738282413, 68.40616817336767497 ) ) ;
#9535=B_SPLINE_CURVE_WITH_KNOTS ( 'NONE', 1,
 ( #7420, #26361 ),
 .UNSPECIFIED., .F., .F.,
 ( 2, 2 ),
 ( 0.000000000000000000, 1.000000000000000000 ),
 .UNSPECIFIED. ) ;
#9537=CARTESIAN_POINT ( 'NONE',  ( -23.78500266573477262, -11.88707733699690827, 59.78235732566622573 ) ) ;
#9538=CARTESIAN_POINT ( 'NONE',  ( -11.04141237841800560, -11.93494539390495568, 74.85840195306853673 ) ) ;
#9539=CARTESIAN_POINT ( 'NONE',  ( -18.85724798917316392, -7.906108138700305155, 67.18599644112759961 ) ) ;
#9540=AXIS2_PLACEMENT_3D ( 'NONE', #35866, #6333, #13930 ) ;
#9541=ORIENTED_EDGE ( 'NONE', *, *, #8305, .T. ) ;
#9542=CYLINDRICAL_SURFACE ( 'NONE', #40703, 0.1500000000000017153 ) ;
#9543=FACE_OUTER_BOUND ( 'NONE', #37135, .T. ) ;
#9545=CARTESIAN_POINT ( 'NONE',  ( -24.82717143659370507, -15.64415108208998539, 73.10329505203212364 ) ) ;
#9547=ORIENTED_EDGE ( 'NONE', *, *, #15031, .F. ) ;
#9548=CARTESIAN_POINT ( 'NONE',  ( -11.76616827618561878, -10.68746712392528764, 74.72419580846755593 ) ) ;
#9551=EDGE_CURVE ( 'NONE', #8240, #39661, #8435, .T. ) ;
#9552=CYLINDRICAL_SURFACE ( 'NONE', #38379, 7.500000000000001776 ) ;
#9553=CARTESIAN_POINT ( 'NONE',  ( -12.84719740098974583, -9.512790884556105553, 74.61923006383901225 ) ) ;
#9554=CARTESIAN_POINT ( 'NONE',  ( -24.20877031762658049, -12.89276232856998661, 66.59686929038259962 ) ) ;
#9555=B_SPLINE_CURVE_WITH_KNOTS ( 'NONE', 3,
 ( #13836, #36489, #2770, #3008, #43434, #9704, #24720, #5987, #21015, #2294 ),
 .UNSPECIFIED., .F., .F.,
 ( 4, 2, 2, 2, 4 ),
 ( 0.6272669072877555818, 0.7522669073072774104, 0.8772669073267993500, 1.002266907346321290, 1.127266907365843007 ),
 .UNSPECIFIED. ) ;
#9557=ORIENTED_EDGE ( 'NONE', *, *, #24060, .T. ) ;
#9558=CYLINDRICAL_SURFACE ( 'NONE', #17386, 7.500000000000001776 ) ;
#9560=CARTESIAN_POINT ( 'NONE',  ( -15.12736045941317897, -21.89643407171298151, 68.69097498501147925 ) ) ;
#9563=CARTESIAN_POINT ( 'NONE',  ( -10.61641583932764910, -11.78277314028518319, 74.74335662173743344 ) ) ;
#9566=CARTESIAN_POINT ( 'NONE',  ( -11.10470733248389230, -18.75498039752055490, 61.46206112672981448 ) ) ;
#9572=LINE ( 'NONE', #13471, #37580 ) ;
#9573=CARTESIAN_POINT ( 'NONE',  ( -21.08382089131013259, -22.19632712819893428, 53.49999999999995026 ) ) ;
#9576=CARTESIAN_POINT ( 'NONE',  ( -12.44869033171645611, -9.885248809711741913, 57.38935532200543577 ) ) ;
#9577=CYLINDRICAL_SURFACE ( 'NONE', #5925, 0.1500000000000007161 ) ;
#9579=CARTESIAN_POINT ( 'NONE',  ( -10.99582063857411995, -11.91441743271276188, 74.55840195587596497 ) ) ;
#9580=CARTESIAN_POINT ( 'NONE',  ( -13.83778161524790384, -21.33926439188370594, 72.03333559426305044 ) ) ;
#9582=ORIENTED_EDGE ( 'NONE', *, *, #8938, .T. ) ;
#9584=CARTESIAN_POINT ( 'NONE',  ( -18.79049830835916524, -7.892586073225762000, 70.38540174208183942 ) ) ;
#9585=ADVANCED_FACE ( 'NONE', ( #14687 ), #38098, .T. ) ;
#9588=CARTESIAN_POINT ( 'NONE',  ( -16.01712388020451883, -7.950755688058114501, 67.36837251840358931 ) ) ;
#9590=CARTESIAN_POINT ( 'NONE',  ( -20.94477883430487708, -21.37566986424753068, 58.75819861804361466 ) ) ;
#9593=CARTESIAN_POINT ( 'NONE',  ( -10.23043904185361086, -12.87167706366568787, 67.83858103935695283 ) ) ;
#9594=CARTESIAN_POINT ( 'NONE',  ( -14.60479746972646886, -7.913168098764732150, 60.50491608655884335 ) ) ;
#9595=CARTESIAN_POINT ( 'NONE',  ( -19.44376929052122449, -7.638105555415076076, 60.07597592072836790 ) ) ;
#9597=( BOUNDED_SURFACE ( )  B_SPLINE_SURFACE ( 3, 1, ( 
 ( #15525, #30590 ),
 ( #34495, #19739 ),
 ( #4464, #11865 ),
 ( #12103, #30833 ),
 ( #12339, #41902 ),
 ( #8660, #45848 ),
 ( #42144, #38429 ) ),
 .UNSPECIFIED., .T., .F., .F. ) 
 B_SPLINE_SURFACE_WITH_KNOTS ( ( 4, 3, 4 ),
 ( 2, 2 ),
 ( 0.000000000000000000, 0.5000000000000000000, 1.000000000000000000 ),
 ( 0.000000000000000000, 1.000000000000000000 ),
 .UNSPECIFIED. ) 
 GEOMETRIC_REPRESENTATION_ITEM ( )  RATIONAL_B_SPLINE_SURFACE ( (
 ( 1.000000000000000000, 1.000000000000000000),
 ( 0.3333333333333335369, 0.3333333333333330373),
 ( 0.3333333333333335369, 0.3333333333333330373),
 ( 1.000000000000000000, 1.000000000000000000),
 ( 0.3333333333333333703, 0.3333333333333333703),
 ( 0.3333333333333333703, 0.3333333333333333703),
 ( 1.000000000000000000, 1.000000000000000000) ) ) 
 REPRESENTATION_ITEM ( '' )  SURFACE ( )  );
#9598=ORIENTED_EDGE ( 'NONE', *, *, #7017, .F. ) ;
#9599=CARTESIAN_POINT ( 'NONE',  ( -11.49688049385021138, -18.62690763749001732, 64.76179218520604763 ) ) ;
#9603=CARTESIAN_POINT ( 'NONE',  ( -17.00410685006708178, -7.771727545396207582, 73.96018273221115180 ) ) ;
#9604=CARTESIAN_POINT ( 'NONE',  ( -14.80727700386144186, -7.833856537212772864, 56.95661706491381437 ) ) ;
#9605=EDGE_CURVE ( 'NONE', #19379, #596, #4642, .T. ) ;
#9606=( BOUNDED_SURFACE ( )  B_SPLINE_SURFACE ( 3, 1, ( 
 ( #4230, #27351 ),
 ( #19239, #41896 ),
 ( #19971, #42384 ),
 ( #34002, #30343 ),
 ( #23917, #34241 ),
 ( #26635, #41650 ),
 ( #23425, #38918 ) ),
 .UNSPECIFIED., .T., .F., .F. ) 
 B_SPLINE_SURFACE_WITH_KNOTS ( ( 4, 3, 4 ),
 ( 2, 2 ),
 ( 0.000000000000000000, 0.5000000000000000000, 1.000000000000000000 ),
 ( 0.000000000000000000, 1.000000000000000000 ),
 .UNSPECIFIED. ) 
 GEOMETRIC_REPRESENTATION_ITEM ( )  RATIONAL_B_SPLINE_SURFACE ( (
 ( 1.000000000000000000, 1.000000000000000000),
 ( 0.3333333333333335369, 0.3333333333333330373),
 ( 0.3333333333333335369, 0.3333333333333330373),
 ( 1.000000000000000000, 1.000000000000000000),
 ( 0.3333333333333333703, 0.3333333333333333703),
 ( 0.3333333333333333703, 0.3333333333333333703),
 ( 1.000000000000000000, 1.000000000000000000) ) ) 
 REPRESENTATION_ITEM ( '' )  SURFACE ( )  );
#9607=CYLINDRICAL_SURFACE ( 'NONE', #6307, 0.1499999999999975242 ) ;
#9608=EDGE_LOOP ( 'NONE', ( #22925, #14156, #627, #39821, #40220 ) ) ;
#9609=CARTESIAN_POINT ( 'NONE',  ( -20.91839308061383562, -20.87517752881106503, 65.60070617543843241 ) ) ;
#9611=CARTESIAN_POINT ( 'NONE',  ( -11.33040464740410158, -19.09525857600861798, 68.40963758452319610 ) ) ;
#9612=ORIENTED_EDGE ( 'NONE', *, *, #37190, .T. ) ;
#9613=EDGE_CURVE ( 'NONE', #20341, #10231, #33393, .T. ) ;
#9614=CARTESIAN_POINT ( 'NONE',  ( -18.35341188057322981, -21.74886570111500461, 72.47438094868762448 ) ) ;
#9616=VERTEX_POINT ( 'NONE', #26068 ) ;
#9617=CARTESIAN_POINT ( 'NONE',  ( -13.58645566915974889, -20.72335281391582384, 61.81086499241362731 ) ) ;
#9618=CARTESIAN_POINT ( 'NONE',  ( -22.07805708657739885, -20.69058616546009333, 53.49999999999994316 ) ) ;
#9619=CARTESIAN_POINT ( 'NONE',  ( -16.45566506110110083, -21.79267588865899086, 62.04095995016087528 ) ) ;
#9622=( BOUNDED_CURVE ( )  B_SPLINE_CURVE ( 3, ( #10784, #34827, #14942, #27205 ),
 .UNSPECIFIED., .F., .F. ) 
 B_SPLINE_CURVE_WITH_KNOTS ( ( 4, 4 ),
 ( 0.4074455897393676196, 0.5000000000000000000 ),
 .UNSPECIFIED. ) 
 CURVE ( )  GEOMETRIC_REPRESENTATION_ITEM ( )  RATIONAL_B_SPLINE_CURVE ( ( 0.6983129098260915102, 0.7760317562606854347, 0.8765941196519848599, 0.9999999999999816813 ) ) 
 REPRESENTATION_ITEM ( '' )  );
#9623=DIRECTION ( 'NONE',  ( -0.8858372764600319638, -0.4639960340712762088, -2.848505657311710446E-17 ) ) ;
#9626=EDGE_LOOP ( 'NONE', ( #40589, #15009 ) ) ;
#9630=CARTESIAN_POINT ( 'NONE',  ( -21.42200791050363051, -21.09572771556245740, 69.09804232902482113 ) ) ;
#9631=ORIENTED_EDGE ( 'NONE', *, *, #25497, .T. ) ;
#9632=CARTESIAN_POINT ( 'NONE',  ( -22.48547534937062409, -20.27602315292274326, 65.96067642556252508 ) ) ;
#9633=CARTESIAN_POINT ( 'NONE',  ( -19.33968086220931326, -21.54245668240326950, 62.01120308345613807 ) ) ;
#9635=ADVANCED_FACE ( 'NONE', ( #22360 ), #33926, .T. ) ;
#9636=CARTESIAN_POINT ( 'NONE',  ( -23.79069799282712339, -10.94014436760912545, 73.55467436599077757 ) ) ;
#9638=CARTESIAN_POINT ( 'NONE',  ( -12.36731060793778525, -9.968227952340054543, 60.84301481710932080 ) ) ;
#9639=ORIENTED_EDGE ( 'NONE', *, *, #45957, .F. ) ;
#9640=ADVANCED_FACE ( 'NONE', ( #44537 ), #47420, .T. ) ;
#9641=CARTESIAN_POINT ( 'NONE',  ( -16.57395829291861844, -22.21062093300318807, 65.26918445414273151 ) ) ;
#9642=CARTESIAN_POINT ( 'NONE',  ( -19.10460565471617755, -7.550450307296652674, 63.54433857513910056 ) ) ;
#9643=CARTESIAN_POINT ( 'NONE',  ( -24.47498361611929596, -14.63661054434306763, 59.12811639263489383 ) ) ;
#9647=ORIENTED_EDGE ( 'NONE', *, *, #2436, .T. ) ;
#9648=ORIENTED_EDGE ( 'NONE', *, *, #37063, .F. ) ;
#9650=CARTESIAN_POINT ( 'NONE',  ( -10.85011829770116876, -12.40413118360892142, 57.62857331434495478 ) ) ;
#9651=CARTESIAN_POINT ( 'NONE',  ( -23.68302403447913562, -11.67432076229741078, 62.95218272177768881 ) ) ;
#9652=CARTESIAN_POINT ( 'NONE',  ( -10.99655737938916289, -18.57624151290433900, 57.99209991576458378 ) ) ;
#9655=CARTESIAN_POINT ( 'NONE',  ( -10.00132051839154457, -15.44646819276786154, 57.82438731113803243 ) ) ;
#9656=ORIENTED_EDGE ( 'NONE', *, *, #5933, .T. ) ;
#9658=CARTESIAN_POINT ( 'NONE',  ( -24.87453101240845399, -14.74101577129048835, 62.89951734912977344 ) ) ;
#9659=ORIENTED_EDGE ( 'NONE', *, *, #6395, .F. ) ;
#9660=CARTESIAN_POINT ( 'NONE',  ( -21.96649320589808241, -8.903988768509519147, 66.82296524986966801 ) ) ;
#9661=EDGE_CURVE ( 'NONE', #12470, #11910, #45522, .T. ) ;
#9663=CARTESIAN_POINT ( 'NONE',  ( -10.58358060774661702, -13.32320000501192325, 71.28116551139133605 ) ) ;
#9664=ORIENTED_EDGE ( 'NONE', *, *, #15530, .T. ) ;
#9665=CARTESIAN_POINT ( 'NONE',  ( -11.90372551521334721, -19.81226007308474379, 58.06648994900333349 ) ) ;
#9666=CARTESIAN_POINT ( 'NONE',  ( -13.38462805196022742, -20.58720062598995426, 58.34650077712429095 ) ) ;
#9667=CARTESIAN_POINT ( 'NONE',  ( -19.45974256962118787, -21.56279627256283149, 58.52507131872702928 ) ) ;
#9671=DIRECTION ( 'NONE',  ( 0.3037135924646502394, -0.9527633776296273727, -2.170275161112332872E-08 ) ) ;
#9672=CARTESIAN_POINT ( 'NONE',  ( -11.18828695359561998, -11.51993516781315918, 67.62424403053286426 ) ) ;
#9674=CARTESIAN_POINT ( 'NONE',  ( -10.00368807899092971, -15.89896712085359098, 54.27966884056655061 ) ) ;
#9677=FACE_BOUND ( 'NONE', #16955, .T. ) ;
#9678=CARTESIAN_POINT ( 'NONE',  ( -24.69822963474414479, -13.19963333263893190, 59.54763306486673713 ) ) ;
#9679=CARTESIAN_POINT ( 'NONE',  ( -13.19099303553301716, -20.93988663701172470, 58.22366935847014702 ) ) ;
#9682=ORIENTED_EDGE ( 'NONE', *, *, #6824, .F. ) ;
#9684=CARTESIAN_POINT ( 'NONE',  ( -22.66113285952138767, -10.16448668345338646, 66.65068261271596839 ) ) ;
#9685=CARTESIAN_POINT ( 'NONE',  ( -24.82475139314513868, -15.66597149415626156, 73.11808456017074320 ) ) ;
#9686=ORIENTED_EDGE ( 'NONE', *, *, #24511, .T. ) ;
#9687=CARTESIAN_POINT ( 'NONE',  ( -11.29476715451500723, -19.04418240398407391, 68.47335581180095687 ) ) ;
#9689=FACE_OUTER_BOUND ( 'NONE', #23041, .T. ) ;
#9691=EDGE_CURVE ( 'NONE', #44542, #2764, #19889, .T. ) ;
#9693=ORIENTED_EDGE ( 'NONE', *, *, #29115, .T. ) ;
#9694=CARTESIAN_POINT ( 'NONE',  ( -24.41273239759876290, -14.40839838354480484, 66.18292728377200262 ) ) ;
#9696=EDGE_CURVE ( 'NONE', #24254, #19672, #45846, .T. ) ;
#9697=CARTESIAN_POINT ( 'NONE',  ( -14.85822224217540466, -7.814955975418383716, 57.04338293508369162 ) ) ;
#9698=ORIENTED_EDGE ( 'NONE', *, *, #12126, .F. ) ;
#9699=CARTESIAN_POINT ( 'NONE',  ( -22.07805708657739885, -20.69058616546009333, 54.27966884056654351 ) ) ;
#9700=CARTESIAN_POINT ( 'NONE',  ( -16.78341213209640159, -22.23169296657789928, 68.88056055876903372 ) ) ;
#9701=( BOUNDED_CURVE ( )  B_SPLINE_CURVE ( 3, ( #37678, #282, #7919, #7181 ),
 .UNSPECIFIED., .F., .F. ) 
 B_SPLINE_CURVE_WITH_KNOTS ( ( 4, 4 ),
 ( 0.5000000000000000000, 0.9074455897393652881 ),
 .UNSPECIFIED. ) 
 CURVE ( )  GEOMETRIC_REPRESENTATION_ITEM ( )  RATIONAL_B_SPLINE_CURVE ( ( 1.000000000000003775, 0.4567392136813372971, 0.3561768502900295452, 0.6983129098260845158 ) ) 
 REPRESENTATION_ITEM ( '' )  );
#9702=ADVANCED_FACE ( 'NONE', ( #8567 ), #30171, .T. ) ;
#9703=CARTESIAN_POINT ( 'NONE',  ( -13.30711168077662521, -9.147894172712071281, 64.20946529582356277 ) ) ;
#9704=CARTESIAN_POINT ( 'NONE',  ( -24.17671788954033474, -17.95647625464824060, 59.11040117746514255 ) ) ;
#9706=CARTESIAN_POINT ( 'NONE',  ( -22.04114742393716142, -9.481025248639417313, 59.73643293354757589 ) ) ;
#9708=VERTEX_POINT ( 'NONE', #16165 ) ;
#9710=CARTESIAN_POINT ( 'NONE',  ( -14.97188219925329378, -8.199429090594037461, 57.14999999999993463 ) ) ;
#9712=EDGE_CURVE ( 'NONE', #26867, #9986, #6383, .T. ) ;
#9714=DIRECTION ( 'NONE',  ( 0.3667195576449454042, -0.9303315355510073381, -1.591455084066186922E-08 ) ) ;
#9715=CARTESIAN_POINT ( 'NONE',  ( -14.03886453949006707, -20.93621418299524350, 68.64728233417358183 ) ) ;
#9717=CARTESIAN_POINT ( 'NONE',  ( -19.29319497538623551, -22.02110451082404907, 58.66474050209521351 ) ) ;
#9718=CARTESIAN_POINT ( 'NONE',  ( -24.14854887165027009, -16.95319183457820955, 69.56907079017828721 ) ) ;
#9720=CARTESIAN_POINT ( 'NONE',  ( -17.99345148343727985, -22.23754510569404630, 62.05252827920184444 ) ) ;
#9721=CARTESIAN_POINT ( 'NONE',  ( -12.87691022455662448, -9.487114556874418625, 74.61923044615130607 ) ) ;
#9722=ORIENTED_EDGE ( 'NONE', *, *, #13982, .F. ) ;
#9724=CARTESIAN_POINT ( 'NONE',  ( -14.93917828805464687, -21.41072449876059380, 58.16617918585938440 ) ) ;
#9727=CARTESIAN_POINT ( 'NONE',  ( -24.05420634179087358, -17.20676946999824608, 69.69867738674849988 ) ) ;
#9728=CARTESIAN_POINT ( 'NONE',  ( -16.78411497196904278, -21.83009869597352903, 68.69560651670111895 ) ) ;
#9729=CARTESIAN_POINT ( 'NONE',  ( -10.70566809389435647, -16.94585225683366048, 57.68760548748759476 ) ) ;
#9731=CARTESIAN_POINT ( 'NONE',  ( -14.44809135640554487, -8.473323881223761234, 67.55975083863336295 ) ) ;
#9732=CARTESIAN_POINT ( 'NONE',  ( -22.14090652532222236, -20.04928072148792495, 62.51967078134249078 ) ) ;
#9733=CARTESIAN_POINT ( 'NONE',  ( -15.44650868948020594, -21.52416737904487576, 72.04575487468440542 ) ) ;
#9734=DIRECTION ( 'NONE',  ( 0.9087012777736581670, -0.4174469879787382487, -4.853707507795077342E-09 ) ) ;
#9735=CARTESIAN_POINT ( 'NONE',  ( -19.94917705995926482, -8.226604131702123013, 74.00624557436877637 ) ) ;
#9736=CARTESIAN_POINT ( 'NONE',  ( -11.42128120280088943, -11.20812582466128760, 60.97885827003174342 ) ) ;
#9738=CYLINDRICAL_SURFACE ( 'NONE', #36901, 0.1500000000000035194 ) ;
#9739=CARTESIAN_POINT ( 'NONE',  ( -23.27284462870851911, -18.74605969774991010, 66.10917289053097079 ) ) ;
#9740=ORIENTED_EDGE ( 'NONE', *, *, #43640, .F. ) ;
#9742=CARTESIAN_POINT ( 'NONE',  ( -14.29604390987698714, -8.047573190463928938, 67.38258169132794251 ) ) ;
#9743=CARTESIAN_POINT ( 'NONE',  ( -20.79160213123634193, -10.44367524184475826, 53.88362224778187226 ) ) ;
#9745=ORIENTED_EDGE ( 'NONE', *, *, #27071, .F. ) ;
#9747=EDGE_CURVE ( 'NONE', #23337, #10698, #35764, .T. ) ;
#9748=ORIENTED_EDGE ( 'NONE', *, *, #38935, .T. ) ;
#9749=ORIENTED_EDGE ( 'NONE', *, *, #11263, .T. ) ;
#9750=EDGE_LOOP ( 'NONE', ( #19968, #4997 ) ) ;
#9753=CARTESIAN_POINT ( 'NONE',  ( -12.91473374035863841, -8.878720881321301661, 67.54089325269804078 ) ) ;
#9754=CARTESIAN_POINT ( 'NONE',  ( -20.66696806162329025, -21.06910005082376358, 58.79475164909958096 ) ) ;
#9756=CARTESIAN_POINT ( 'NONE',  ( -10.71275542623144972, -16.80315959844558549, 57.75930835357964099 ) ) ;
#9757=( BOUNDED_CURVE ( )  B_SPLINE_CURVE ( 3, ( #38239, #26449, #7757, #45901 ),
 .UNSPECIFIED., .F., .F. ) 
 B_SPLINE_CURVE_WITH_KNOTS ( ( 4, 4 ),
 ( 0.000000000000000000, 0.4074455897393695625 ),
 .UNSPECIFIED. ) 
 CURVE ( )  GEOMETRIC_REPRESENTATION_ITEM ( )  RATIONAL_B_SPLINE_CURVE ( ( 1.000000000000000000, 0.4567392136813288595, 0.3561768502900291566, 0.6983129098261007250 ) ) 
 REPRESENTATION_ITEM ( '' )  );
#9758=EDGE_LOOP ( 'NONE', ( #23837, #22042 ) ) ;
#9759=EDGE_LOOP ( 'NONE', ( #26592, #19100 ) ) ;
#9761=CARTESIAN_POINT ( 'NONE',  ( -24.87384330133638599, -14.87999890626018384, 59.35804801245023299 ) ) ;
#9762=CARTESIAN_POINT ( 'NONE',  ( -20.72573962529263625, -8.580110715261016097, 59.99125250080121674 ) ) ;
#9764=EDGE_CURVE ( 'NONE', #27258, #48679, #2106, .T. ) ;
#9766=AXIS2_PLACEMENT_3D ( 'NONE', #36758, #17340, #37013 ) ;
#9767=EDGE_LOOP ( 'NONE', ( #18322, #36387 ) ) ;
#9768=EDGE_CURVE ( 'NONE', #2153, #24134, #29314, .T. ) ;
#9769=EDGE_CURVE ( 'NONE', #21456, #27235, #28095, .T. ) ;
#9771=CARTESIAN_POINT ( 'NONE',  ( -24.36278207060129830, -15.73458306695098941, 69.53307441226529306 ) ) ;
#9772=AXIS2_PLACEMENT_3D ( 'NONE', #21477, #44371, #6687 ) ;
#9773=CARTESIAN_POINT ( 'NONE',  ( -10.64854695470030599, -12.86019059820356780, 64.55364013863997741 ) ) ;
#9774=ORIENTED_EDGE ( 'NONE', *, *, #5468, .T. ) ;
#9775=DIRECTION ( 'NONE',  ( -0.1464579420318390668, 0.9892168979631277281, 7.284849527811297202E-08 ) ) ;
#9776=CARTESIAN_POINT ( 'NONE',  ( -22.44487633517903902, -9.931440556337857828, 73.76695770713021716 ) ) ;
#9777=CARTESIAN_POINT ( 'NONE',  ( -21.38467548909741467, -8.976808945791946215, 73.60128784396469825 ) ) ;
#9778=CARTESIAN_POINT ( 'NONE',  ( -22.48547534937062409, -20.27602315292274326, 65.96067642556252508 ) ) ;
#9780=CARTESIAN_POINT ( 'NONE',  ( -22.58065782673598676, -12.89613362149922260, 54.49999999999995026 ) ) ;
#9782=CARTESIAN_POINT ( 'NONE',  ( -17.98078303480458473, -21.78831889235732078, 65.57362029541940274 ) ) ;
#9786=FACE_OUTER_BOUND ( 'NONE', #18427, .T. ) ;
#9787=CARTESIAN_POINT ( 'NONE',  ( -14.59168816866676188, -7.918454268363332993, 60.45849798934733599 ) ) ;
#9789=CARTESIAN_POINT ( 'NONE',  ( -13.17733471316897642, -8.687979735119538915, 60.61667131793516461 ) ) ;
#9791=ADVANCED_FACE ( 'NONE', ( #10532 ), #15310, .T. ) ;
#9792=CARTESIAN_POINT ( 'NONE',  ( -17.33887285826562774, -7.751749031259347333, 74.10451155337131013 ) ) ;
#9793=CARTESIAN_POINT ( 'NONE',  ( -14.27198868620293482, -8.503074456523135538, 70.72957634543823247 ) ) ;
#9794=ORIENTED_EDGE ( 'NONE', *, *, #38030, .F. ) ;
#9795=CARTESIAN_POINT ( 'NONE',  ( -16.36834455927873222, -22.18410795223847387, 61.94063518049016182 ) ) ;
#9797=CARTESIAN_POINT ( 'NONE',  ( -16.56382623105763230, -21.80656378348893654, 65.22564414072157035 ) ) ;
#9801=CARTESIAN_POINT ( 'NONE',  ( -24.35037712455101655, -13.45216126592925754, 62.97697330661279835 ) ) ;
#9804=ORIENTED_EDGE ( 'NONE', *, *, #37351, .T. ) ;
#9807=CARTESIAN_POINT ( 'NONE',  ( -10.02109181922889292, -15.64579944599920402, 61.21601811723743225 ) ) ;
#9809=CARTESIAN_POINT ( 'NONE',  ( -21.88682393090045508, -8.843550627677114306, 66.82183330550128630 ) ) ;
#9810=CARTESIAN_POINT ( 'NONE',  ( -10.40492013132468863, -15.46819742413635268, 57.86792798853620923 ) ) ;
#9811=FACE_OUTER_BOUND ( 'NONE', #26683, .T. ) ;
#9812=LINE ( 'NONE', #9579, #20022 ) ;
#9813=CARTESIAN_POINT ( 'NONE',  ( -16.69812366561379591, -22.22391868458808517, 68.85707174038356015 ) ) ;
#9814=VERTEX_POINT ( 'NONE', #40324 ) ;
#9815=EDGE_LOOP ( 'NONE', ( #10745, #27773 ) ) ;
#9817=CARTESIAN_POINT ( 'NONE',  ( -22.02419907101585395, -20.08547720931746383, 58.87328889079346794 ) ) ;
#9818=CARTESIAN_POINT ( 'NONE',  ( -19.55442184481404766, -21.52995072282663358, 65.47958309245051112 ) ) ;
#9819=CARTESIAN_POINT ( 'NONE',  ( -24.55648639541664124, -12.65693619758180688, 69.87968855437600268 ) ) ;
#9820=DIRECTION ( 'NONE',  ( -0.5497669574358331479, 0.8353180786453390239, 7.898837271846010071E-08 ) ) ;
#9823=ADVANCED_FACE ( 'NONE', ( #17659 ), #13443, .T. ) ;
#9825=DIRECTION ( 'NONE',  ( -2.117869065290744265E-07, -2.255668823645213100E-07, -0.9999999999999521494 ) ) ;
#9826=CARTESIAN_POINT ( 'NONE',  ( -10.43098718212803000, -15.70539730037032911, 61.32316937334011442 ) ) ;
#9827=EDGE_LOOP ( 'NONE', ( #28920, #23508, #32255, #28106, #27987 ) ) ;
#9829=EDGE_CURVE ( 'NONE', #6268, #44129, #19368, .T. ) ;
#9831=CARTESIAN_POINT ( 'NONE',  ( -10.56627932147773308, -16.21290872759732693, 71.74750383609593030 ) ) ;
#9835=CARTESIAN_POINT ( 'NONE',  ( -24.85359113602694237, -14.25571898851532460, 69.76779851910008290 ) ) ;
#9836=CARTESIAN_POINT ( 'NONE',  ( -10.90759836534377492, -17.49952001658422063, 68.39721944423101263 ) ) ;
#9837=ORIENTED_EDGE ( 'NONE', *, *, #32122, .F. ) ;
#9838=CARTESIAN_POINT ( 'NONE',  ( -23.01170616074242758, -19.02577216718165332, 58.89913050316314269 ) ) ;
#9840=CARTESIAN_POINT ( 'NONE',  ( -24.36611147337434957, -16.04009697885371111, 66.07797069094537790 ) ) ;
#9841=CARTESIAN_POINT ( 'NONE',  ( -10.23976007159296486, -12.83681284056133265, 67.89978877642941768 ) ) ;
#9843=CARTESIAN_POINT ( 'NONE',  ( -10.98022799891133516, -11.94040251240491202, 71.29680800581914468 ) ) ;
#9844=ADVANCED_FACE ( 'NONE', ( #45744 ), #4357, .T. ) ;
#9846=B_SPLINE_CURVE_WITH_KNOTS ( 'NONE', 1,
 ( #10843, #3958 ),
 .UNSPECIFIED., .F., .F.,
 ( 2, 2 ),
 ( 0.000000000000000000, 1.000000000000000000 ),
 .UNSPECIFIED. ) ;
#9847=EDGE_LOOP ( 'NONE', ( #29149, #35788, #18129, #14326, #4391 ) ) ;
#9849=CARTESIAN_POINT ( 'NONE',  ( -20.76617135726475993, -8.601540970369937256, 59.84685049461698014 ) ) ;
#9850=CARTESIAN_POINT ( 'NONE',  ( -23.83080496556880945, -17.75212211224490133, 59.28906343887996400 ) ) ;
#9851=ORIENTED_EDGE ( 'NONE', *, *, #1771, .F. ) ;
#9852=CARTESIAN_POINT ( 'NONE',  ( -19.96446419288020735, -21.81276346405129019, 69.12756636080516159 ) ) ;
#9853=CARTESIAN_POINT ( 'NONE',  ( -23.54964580958837672, -11.31912319124952759, 70.19210731698237282 ) ) ;
#9854=CARTESIAN_POINT ( 'NONE',  ( -24.14679772577363437, -12.68507108172156705, 70.05770892828130059 ) ) ;
#9855=CARTESIAN_POINT ( 'NONE',  ( -21.68499490698325971, -9.192515188766618550, 66.81149992326716358 ) ) ;
#9857=ORIENTED_EDGE ( 'NONE', *, *, #7587, .T. ) ;
#9858=CARTESIAN_POINT ( 'NONE',  ( -23.78452478447325547, -18.68833123104472449, 72.86393997050505789 ) ) ;
#9859=CARTESIAN_POINT ( 'NONE',  ( -21.12516169987187098, -20.80993955427394582, 69.06922321213187388 ) ) ;
#9860=ORIENTED_EDGE ( 'NONE', *, *, #29798, .F. ) ;
#9861=CARTESIAN_POINT ( 'NONE',  ( -17.74685204685923523, -7.816528611283073857, 60.38060757087333030 ) ) ;
#9863=CARTESIAN_POINT ( 'NONE',  ( -10.42462062702805703, -14.89507852762941198, 74.79778901763455679 ) ) ;
#9864=CARTESIAN_POINT ( 'NONE',  ( -10.90176001668674743, -17.49323270848192635, 71.98206789237249836 ) ) ;
#9867=CARTESIAN_POINT ( 'NONE',  ( -21.02205230129062485, -8.737166911425223503, 59.98558246646761916 ) ) ;
#9870=CARTESIAN_POINT ( 'NONE',  ( -11.82948135756627117, -23.21535936243710552, 54.54971261817297545 ) ) ;
#9872=( BOUNDED_SURFACE ( )  B_SPLINE_SURFACE ( 3, 1, ( 
 ( #28977, #29226 ),
 ( #32201, #2395 ),
 ( #47217, #13461 ),
 ( #47939, #28506 ),
 ( #24810, #14170 ),
 ( #25298, #21833 ),
 ( #6085, #40537 ) ),
 .UNSPECIFIED., .T., .F., .F. ) 
 B_SPLINE_SURFACE_WITH_KNOTS ( ( 4, 3, 4 ),
 ( 2, 2 ),
 ( 0.000000000000000000, 0.5000000000000000000, 1.000000000000000000 ),
 ( 0.000000000000000000, 1.000000000000000000 ),
 .UNSPECIFIED. ) 
 GEOMETRIC_REPRESENTATION_ITEM ( )  RATIONAL_B_SPLINE_SURFACE ( (
 ( 1.000000000000000000, 1.000000000000000000),
 ( 0.3333333333333335369, 0.3333333333333330373),
 ( 0.3333333333333335369, 0.3333333333333330373),
 ( 1.000000000000000000, 1.000000000000000000),
 ( 0.3333333333333333703, 0.3333333333333333703),
 ( 0.3333333333333333703, 0.3333333333333333703),
 ( 1.000000000000000000, 1.000000000000000000) ) ) 
 REPRESENTATION_ITEM ( '' )  SURFACE ( )  );
#9873=EDGE_LOOP ( 'NONE', ( #2133, #12822 ) ) ;
#9875=EDGE_CURVE ( 'NONE', #508, #40402, #10009, .T. ) ;
#9876=DIRECTION ( 'NONE',  ( 1.209056813000714825E-06, 5.657077699801570473E-07, 0.9999999999991090460 ) ) ;
#9878=CARTESIAN_POINT ( 'NONE',  ( -23.89622975106627223, -11.11939700565759459, 69.99872433690991613 ) ) ;
#9879=( BOUNDED_SURFACE ( )  B_SPLINE_SURFACE ( 3, 1, ( 
 ( #18808, #40724 ),
 ( #15337, #33818 ),
 ( #7504, #45180 ),
 ( #44684, #25958 ),
 ( #25470, #114 ),
 ( #11418, #26443 ),
 ( #41456, #7752 ) ),
 .UNSPECIFIED., .T., .F., .F. ) 
 B_SPLINE_SURFACE_WITH_KNOTS ( ( 4, 3, 4 ),
 ( 2, 2 ),
 ( 0.000000000000000000, 0.5000000000000000000, 1.000000000000000000 ),
 ( 0.000000000000000000, 1.000000000000000000 ),
 .UNSPECIFIED. ) 
 GEOMETRIC_REPRESENTATION_ITEM ( )  RATIONAL_B_SPLINE_SURFACE ( (
 ( 1.000000000000000000, 1.000000000000000000),
 ( 0.3333333333333335369, 0.3333333333333330373),
 ( 0.3333333333333335369, 0.3333333333333330373),
 ( 1.000000000000000000, 1.000000000000000000),
 ( 0.3333333333333333703, 0.3333333333333333703),
 ( 0.3333333333333333703, 0.3333333333333333703),
 ( 1.000000000000000000, 1.000000000000000000) ) ) 
 REPRESENTATION_ITEM ( '' )  SURFACE ( )  );
#9880=VERTEX_POINT ( 'NONE', #18888 ) ;
#9881=( BOUNDED_CURVE ( )  B_SPLINE_CURVE ( 3, ( #9710, #24239, #21514, #39730 ),
 .UNSPECIFIED., .F., .F. ) 
 B_SPLINE_CURVE_WITH_KNOTS ( ( 4, 4 ),
 ( 0.9074455897393685078, 1.000000000000000000 ),
 .UNSPECIFIED. ) 
 CURVE ( )  GEOMETRIC_REPRESENTATION_ITEM ( )  RATIONAL_B_SPLINE_CURVE ( ( 0.6983129098261030565, 0.7760317562607068620, 0.8765941196520058432, 1.000000000000000000 ) ) 
 REPRESENTATION_ITEM ( '' )  );
#9882=CARTESIAN_POINT ( 'NONE',  ( -24.26595263201846109, -13.32969024507516309, 59.66267925069213618 ) ) ;
#9884=CARTESIAN_POINT ( 'NONE',  ( -12.76547314785493192, -9.517330534081262172, 74.60450883341005124 ) ) ;
#9885=VERTEX_POINT ( 'NONE', #29980 ) ;
#9886=EDGE_CURVE ( 'NONE', #7245, #47302, #39261, .T. ) ;
#9887=CARTESIAN_POINT ( 'NONE',  ( -11.03161394367693049, -18.63672047605813376, 57.92059234540772650 ) ) ;
#9888=CARTESIAN_POINT ( 'NONE',  ( -20.40273017466792638, -8.415258652480821056, 70.55100319412855470 ) ) ;
#9889=EDGE_CURVE ( 'NONE', #2374, #41728, #31072, .T. ) ;
#9890=CARTESIAN_POINT ( 'NONE',  ( -23.37950063508610299, -10.33300044972819975, 59.70929291905022751 ) ) ;
#9891=B_SPLINE_CURVE_WITH_KNOTS ( 'NONE', 3,
 ( #35241, #5473, #23712, #27862, #20489, #15797, #20230, #38201, #43129, #8684 ),
 .UNSPECIFIED., .F., .F.,
 ( 4, 2, 2, 2, 4 ),
 ( 0.1272669073658402039, 0.2522669073488030267, 0.3772669073317658217, 0.5022669073147286722, 0.6272669072976915228 ),
 .UNSPECIFIED. ) ;
#9892=VERTEX_POINT ( 'NONE', #19131 ) ;
#9893=( BOUNDED_CURVE ( )  B_SPLINE_CURVE ( 3, ( #1277, #31326, #42425, #28369 ),
 .UNSPECIFIED., .F., .F. ) 
 B_SPLINE_CURVE_WITH_KNOTS ( ( 4, 4 ),
 ( 0.9074455897393621795, 1.000000000000000000 ),
 .UNSPECIFIED. ) 
 CURVE ( )  GEOMETRIC_REPRESENTATION_ITEM ( )  RATIONAL_B_SPLINE_CURVE ( ( 0.6983129098260923984, 0.7760317562606976471, 0.8765941196520001810, 1.000000000000000000 ) ) 
 REPRESENTATION_ITEM ( '' )  );
#9894=VECTOR ( 'NONE', #22399, 1000.000000000000000 ) ;
#9895=EDGE_LOOP ( 'NONE', ( #35276, #38994 ) ) ;
#9896=CARTESIAN_POINT ( 'NONE',  ( -15.95707318215220205, -7.504986700048139170, 63.85506303619484214 ) ) ;
#9897=CARTESIAN_POINT ( 'NONE',  ( -24.47658614515328779, -17.21021725504682109, 73.03336031685063290 ) ) ;
#9898=CARTESIAN_POINT ( 'NONE',  ( -18.11889358109259973, -21.82488563948435711, 65.64532159284070190 ) ) ;
#9899=ORIENTED_EDGE ( 'NONE', *, *, #16207, .T. ) ;
#9901=CARTESIAN_POINT ( 'NONE',  ( -10.29385316490627211, -12.64970523595484231, 64.38340807599202265 ) ) ;
#9902=FACE_OUTER_BOUND ( 'NONE', #33414, .T. ) ;
#9905=CARTESIAN_POINT ( 'NONE',  ( -20.51077960756537522, -21.09370107797763083, 58.75548229756886798 ) ) ;
#9906=ORIENTED_EDGE ( 'NONE', *, *, #27818, .T. ) ;
#9907=CARTESIAN_POINT ( 'NONE',  ( -24.80275449484538441, -15.83773296361996863, 69.68307485620266561 ) ) ;
#9908=FACE_OUTER_BOUND ( 'NONE', #40140, .T. ) ;
#9909=DIRECTION ( 'NONE',  ( -3.597453700672850830E-07, -4.264980243973025121E-06, 0.9999999999908403270 ) ) ;
#9910=CARTESIAN_POINT ( 'NONE',  ( -16.26195973558533936, -21.76306465430365122, 58.57113428431811997 ) ) ;
#9913=EDGE_LOOP ( 'NONE', ( #3613, #3786 ) ) ;
#9915=DIRECTION ( 'NONE',  ( 0.2843796944294933460, 0.9587117342539337450, 5.205739956168971478E-08 ) ) ;
#9916=VERTEX_POINT ( 'NONE', #34867 ) ;
#9918=CARTESIAN_POINT ( 'NONE',  ( -10.10423179225323054, -16.19963241119870645, 71.63405780323361682 ) ) ;
#9920=CARTESIAN_POINT ( 'NONE',  ( -22.98758735661991892, -9.854289139077749837, 70.26824437992965500 ) ) ;
#9921=CARTESIAN_POINT ( 'NONE',  ( -17.00402163565062708, -22.24752138760033660, 72.30396712152169414 ) ) ;
#9923=FACE_BOUND ( 'NONE', #20795, .T. ) ;
#9926=FACE_OUTER_BOUND ( 'NONE', #23938, .T. ) ;
#9930=CARTESIAN_POINT ( 'NONE',  ( -16.98029472128749617, -7.773148622573092581, 74.26018263347066295 ) ) ;
#9933=CARTESIAN_POINT ( 'NONE',  ( -10.70297003644833644, -11.59513240183115279, 71.27356180636090244 ) ) ;
#9934=FACE_OUTER_BOUND ( 'NONE', #44936, .T. ) ;
#9938=VECTOR ( 'NONE', #36268, 1000.000000000000000 ) ;
#9940=DIRECTION ( 'NONE',  ( 8.419732586906766855E-06, -4.907637678936094986E-06, -0.9999999999525116534 ) ) ;
#9941=CARTESIAN_POINT ( 'NONE',  ( -20.13067924262885100, -8.351893229360399573, 73.91023551582938467 ) ) ;
#9944=VERTEX_POINT ( 'NONE', #195 ) ;
#9945=EDGE_CURVE ( 'NONE', #26800, #44868, #11831, .T. ) ;
#9946=CARTESIAN_POINT ( 'NONE',  ( -10.99230636966125729, -11.04936141590450127, 60.80072991414726147 ) ) ;
#9949=ORIENTED_EDGE ( 'NONE', *, *, #36195, .F. ) ;
#9950=CARTESIAN_POINT ( 'NONE',  ( -24.41485939984550058, -14.44976655980182834, 66.48292729254383460 ) ) ;
#9951=CYLINDRICAL_SURFACE ( 'NONE', #20431, 0.1499999999999985234 ) ;
#9952=ORIENTED_EDGE ( 'NONE', *, *, #43579, .F. ) ;
#9953=EDGE_CURVE ( 'NONE', #17470, #13199, #25400, .T. ) ;
#9954=DIRECTION ( 'NONE',  ( 7.105595952316565779E-06, 6.912614981796274630E-07, -0.9999999999745162738 ) ) ;
#9956=ORIENTED_EDGE ( 'NONE', *, *, #9764, .T. ) ;
#9957=CARTESIAN_POINT ( 'NONE',  ( -10.51282180855659298, -13.41675832278428615, 74.97257849336672564 ) ) ;
#9958=CARTESIAN_POINT ( 'NONE',  ( -23.40706704545067041, -18.44294168544361057, 72.76368236816873036 ) ) ;
#9959=EDGE_CURVE ( 'NONE', #46068, #30656, #7150, .T. ) ;
#9960=CARTESIAN_POINT ( 'NONE',  ( -16.74223095289501018, -21.77591761258009839, 65.33450335857290270 ) ) ;
#9961=CARTESIAN_POINT ( 'NONE',  ( -10.57110082969170683, -13.38215148069720861, 74.67817647591368768 ) ) ;
#9963=CARTESIAN_POINT ( 'NONE',  ( -21.93816111929147539, -20.22843456855405364, 62.64927864921646261 ) ) ;
#9964=CARTESIAN_POINT ( 'NONE',  ( -24.37683822056718697, -15.97618770311995462, 66.06324926631656069 ) ) ;
#9965=CARTESIAN_POINT ( 'NONE',  ( -21.40553701582064150, -22.29995169140471845, 54.49999999999995026 ) ) ;
#9968=FACE_OUTER_BOUND ( 'NONE', #13619, .T. ) ;
#9969=CARTESIAN_POINT ( 'NONE',  ( -23.50612575731066656, -19.11299006986292071, 66.01044822673141255 ) ) ;
#9970=VERTEX_POINT ( 'NONE', #5328 ) ;
#9971=CARTESIAN_POINT ( 'NONE',  ( -24.34180841910587034, -17.57479211026192090, 66.05018951071652111 ) ) ;
#9972=( BOUNDED_CURVE ( )  B_SPLINE_CURVE ( 3, ( #24859, #36400, #13980, #6627 ),
 .UNSPECIFIED., .F., .F. ) 
 B_SPLINE_CURVE_WITH_KNOTS ( ( 4, 4 ),
 ( 0.4074455897393663428, 0.5000000000000000000 ),
 .UNSPECIFIED. ) 
 CURVE ( )  GEOMETRIC_REPRESENTATION_ITEM ( )  RATIONAL_B_SPLINE_CURVE ( ( 0.6983129098261003920, 0.7760317562607003117, 0.8765941196519989598, 0.9999999999999932276 ) ) 
 REPRESENTATION_ITEM ( '' )  );
#9973=VECTOR ( 'NONE', #9775, 1000.000000000000227 ) ;
#9975=CARTESIAN_POINT ( 'NONE',  ( -20.84119746710918974, -20.97572115929791892, 62.11471400470772863 ) ) ;
#9976=ORIENTED_EDGE ( 'NONE', *, *, #14187, .F. ) ;
#9977=CARTESIAN_POINT ( 'NONE',  ( -24.34138173484706158, -16.17068648017255583, 62.59328676670276792 ) ) ;
#9978=EDGE_LOOP ( 'NONE', ( #46193, #26231, #42590, #43524, #27930 ) ) ;
#9979=ORIENTED_EDGE ( 'NONE', *, *, #34875, .F. ) ;
#9980=EDGE_LOOP ( 'NONE', ( #10965, #3624 ) ) ;
#9984=FACE_OUTER_BOUND ( 'NONE', #16247, .T. ) ;
#9985=CARTESIAN_POINT ( 'NONE',  ( -12.74071780128996423, -9.015264284427722430, 70.96430057504635158 ) ) ;
#9986=VERTEX_POINT ( 'NONE', #5089 ) ;
#9987=ORIENTED_EDGE ( 'NONE', *, *, #47660, .F. ) ;
#9989=CARTESIAN_POINT ( 'NONE',  ( -14.09463846823036981, -8.088735815341543400, 54.27966884056655061 ) ) ;
#9992=EDGE_CURVE ( 'NONE', #656, #29137, #31591, .T. ) ;
#9994=AXIS2_PLACEMENT_3D ( 'NONE', #1560, #38985, #27667 ) ;
#9995=ORIENTED_EDGE ( 'NONE', *, *, #17579, .T. ) ;
#9999=EDGE_LOOP ( 'NONE', ( #29029, #11595 ) ) ;
#10001=VERTEX_POINT ( 'NONE', #12463 ) ;
#10003=CARTESIAN_POINT ( 'NONE',  ( -10.65419218092657339, -12.82848081120560479, 60.79853508363822101 ) ) ;
#10005=EDGE_CURVE ( 'NONE', #48717, #31810, #29853, .T. ) ;
#10006=EDGE_LOOP ( 'NONE', ( #37719, #36610 ) ) ;
#10007=CARTESIAN_POINT ( 'NONE',  ( -12.77988270905505175, -9.504878500073925096, 74.61363196716065715 ) ) ;
#10009=( BOUNDED_CURVE ( )  B_SPLINE_CURVE ( 3, ( #23084, #11750, #8074, #4850 ),
 .UNSPECIFIED., .F., .F. ) 
 B_SPLINE_CURVE_WITH_KNOTS ( ( 4, 4 ),
 ( 0.4074455897393599590, 0.5000000000000000000 ),
 .UNSPECIFIED. ) 
 CURVE ( )  GEOMETRIC_REPRESENTATION_ITEM ( )  RATIONAL_B_SPLINE_CURVE ( ( 0.6983129098260680845, 0.7760317562606778852, 0.8765941196519888567, 1.000000000000001998 ) ) 
 REPRESENTATION_ITEM ( '' )  );
#10010=CARTESIAN_POINT ( 'NONE',  ( -22.88419851978063591, -10.42888047092867865, 63.07185995612697837 ) ) ;
#10011=DIRECTION ( 'NONE',  ( 3.549360974554993999E-17, -6.371834667797928663E-18, -1.000000000000000000 ) ) ;
#10013=CYLINDRICAL_SURFACE ( 'NONE', #46, 0.1500000000000009104 ) ;
#10014=CARTESIAN_POINT ( 'NONE',  ( -24.84793648988037518, -14.18443574041886457, 69.83770584630335065 ) ) ;
#10016=CARTESIAN_POINT ( 'NONE',  ( -13.35818949714929360, -21.05197827947291955, 61.70141596610112344 ) ) ;
#10017=CARTESIAN_POINT ( 'NONE',  ( -16.25049964979334050, -21.71175520172467444, 61.94495303334971936 ) ) ;
#10018=EDGE_LOOP ( 'NONE', ( #9860, #22151, #12995, #17928 ) ) ;
#10019=CARTESIAN_POINT ( 'NONE',  ( -13.22450642086665873, -8.655658357931690361, 60.53976038923259750 ) ) ;
#10020=DIRECTION ( 'NONE',  ( -0.6562885720885137664, 0.7545099801500437797, 1.193821363054684963E-08 ) ) ;
#10021=CARTESIAN_POINT ( 'NONE',  ( -16.94458744105653381, -7.374567917109038362, 74.14513580114275726 ) ) ;
#10022=CARTESIAN_POINT ( 'NONE',  ( -21.24554616535955631, -21.20453920045676810, 65.76949338751086316 ) ) ;
#10023=ORIENTED_EDGE ( 'NONE', *, *, #1093, .F. ) ;
#10026=CARTESIAN_POINT ( 'NONE',  ( -19.01558049692976482, -7.531172701354427623, 67.10082990693875615 ) ) ;
#10027=CARTESIAN_POINT ( 'NONE',  ( -16.58751095051766455, -21.80939428823196025, 65.22564390318969174 ) ) ;
#10028=EDGE_CURVE ( 'NONE', #24855, #23931, #27490, .T. ) ;
#10030=CARTESIAN_POINT ( 'NONE',  ( -10.16417196683383217, -13.13632154568680477, 71.36861914326480871 ) ) ;
#10031=( BOUNDED_CURVE ( )  B_SPLINE_CURVE ( 3, ( #17960, #32977, #2234, #48022 ),
 .UNSPECIFIED., .F., .F. ) 
 B_SPLINE_CURVE_WITH_KNOTS ( ( 4, 4 ),
 ( 0.000000000000000000, 0.4074455897393655102 ),
 .UNSPECIFIED. ) 
 CURVE ( )  GEOMETRIC_REPRESENTATION_ITEM ( )  RATIONAL_B_SPLINE_CURVE ( ( 1.000000000000000000, 0.4567392136813288595, 0.3561768502900291566, 0.6983129098261007250 ) ) 
 REPRESENTATION_ITEM ( '' )  );
#10032=EDGE_CURVE ( 'NONE', #4358, #46391, #42760, .T. ) ;
#10034=CARTESIAN_POINT ( 'NONE',  ( -24.77961554291793789, -15.99297619861334674, 66.22358246620183309 ) ) ;
#10035=EDGE_CURVE ( 'NONE', #43753, #27411, #23552, .T. ) ;
#10036=EDGE_CURVE ( 'NONE', #46554, #35531, #20086, .T. ) ;
#10037=ORIENTED_EDGE ( 'NONE', *, *, #12809, .T. ) ;
#10039=CARTESIAN_POINT ( 'NONE',  ( -23.40706900507760224, -18.44293855997280929, 73.06368236814604700 ) ) ;
#10042=AXIS2_PLACEMENT_3D ( 'NONE', #2019, #40410, #5960 ) ;
#10043=CARTESIAN_POINT ( 'NONE',  ( -23.42981297399330742, -19.21767893247333348, 62.46132742258500770 ) ) ;
#10044=CARTESIAN_POINT ( 'NONE',  ( -17.42409385541300892, -14.80920654474439679, 56.49999999999994316 ) ) ;
#10045=CARTESIAN_POINT ( 'NONE',  ( -10.52215087187021325, -13.37195826583270808, 74.67817647370830514 ) ) ;
#10046=CARTESIAN_POINT ( 'NONE',  ( -12.40421236734144728, -20.31415489762336435, 68.38011531907731921 ) ) ;
#10048=CARTESIAN_POINT ( 'NONE',  ( -23.13015969901951863, -18.95476373626217281, 58.76921843841908810 ) ) ;
#10049=ORIENTED_EDGE ( 'NONE', *, *, #25936, .T. ) ;
#10050=ORIENTED_EDGE ( 'NONE', *, *, #45821, .T. ) ;
#10052=CARTESIAN_POINT ( 'NONE',  ( -23.12041803196159506, -10.00762535718595991, 66.64908106505099283 ) ) ;
#10053=CARTESIAN_POINT ( 'NONE',  ( -14.85449537034919132, -21.32098772481755944, 61.65217026632952013 ) ) ;
#10057=ORIENTED_EDGE ( 'NONE', *, *, #24352, .T. ) ;
#10058=EDGE_CURVE ( 'NONE', #32101, #18786, #14603, .T. ) ;
#10059=CARTESIAN_POINT ( 'NONE',  ( -14.86587017669673649, -21.80700303724089295, 61.74945191855038473 ) ) ;
#10061=CARTESIAN_POINT ( 'NONE',  ( -14.84764829735760649, -8.246537290690364230, 60.33468334944129197 ) ) ;
#10062=AXIS2_PLACEMENT_3D ( 'NONE', #46895, #13137, #17073 ) ;
#10063=CARTESIAN_POINT ( 'NONE',  ( -11.18327426895797494, -18.87804038469763768, 64.94045401417226060 ) ) ;
#10065=AXIS2_PLACEMENT_3D ( 'NONE', #11972, #26981, #6519 ) ;
#10066=VECTOR ( 'NONE', #45100, 1000.000000000000000 ) ;
#10067=ADVANCED_FACE ( 'NONE', ( #36777 ), #33086, .T. ) ;
#10068=FACE_OUTER_BOUND ( 'NONE', #16029, .T. ) ;
#10071=CARTESIAN_POINT ( 'NONE',  ( -16.93941734680482725, -7.775588144984237005, 74.24546186738449194 ) ) ;
#10072=FACE_OUTER_BOUND ( 'NONE', #11166, .T. ) ;
#10073=ORIENTED_EDGE ( 'NONE', *, *, #26946, .F. ) ;
#10074=CARTESIAN_POINT ( 'NONE',  ( -19.08220441618011520, -7.953150065343516317, 59.96092815196451653 ) ) ;
#10075=ORIENTED_EDGE ( 'NONE', *, *, #46856, .T. ) ;
#10076=CARTESIAN_POINT ( 'NONE',  ( -11.47236213698566054, -10.32806074475630886, 74.55389686390628867 ) ) ;
#10078=ORIENTED_EDGE ( 'NONE', *, *, #7889, .F. ) ;
#10079=CARTESIAN_POINT ( 'NONE',  ( -11.07857854458970692, -11.73724703412850801, 71.08860870961423473 ) ) ;
#10081=ORIENTED_EDGE ( 'NONE', *, *, #30101, .T. ) ;
#10082=CARTESIAN_POINT ( 'NONE',  ( -18.75616178366165698, -7.937006232909297410, 70.67068081708849547 ) ) ;
#10083=CARTESIAN_POINT ( 'NONE',  ( -19.77283897654775657, -21.87935945976245122, 65.50840285157048015 ) ) ;
#10085=EDGE_LOOP ( 'NONE', ( #44111, #9899, #42656, #36054, #44307 ) ) ;
#10086=CARTESIAN_POINT ( 'NONE',  ( -17.64006181755907932, -7.293987387894279806, 54.02312124697527906 ) ) ;
#10088=CARTESIAN_POINT ( 'NONE',  ( -23.53886599083197240, -11.30005350631630279, 70.18650949724866450 ) ) ;
#10089=FACE_OUTER_BOUND ( 'NONE', #35623, .T. ) ;
#10090=CARTESIAN_POINT ( 'NONE',  ( -22.84116833803633284, -10.28479860924217704, 59.75770304231562591 ) ) ;
#10092=ADVANCED_FACE ( 'NONE', ( #6774 ), #43686, .T. ) ;
#10094=ORIENTED_EDGE ( 'NONE', *, *, #28474, .T. ) ;
#10096=CARTESIAN_POINT ( 'NONE',  ( -21.23484681875272884, -20.74088929683185611, 69.33978048267414351 ) ) ;
#10098=VECTOR ( 'NONE', #33608, 1000.000000000000000 ) ;
#10099=CARTESIAN_POINT ( 'NONE',  ( -23.83080496556880945, -17.75212211224490133, 59.28906343887996400 ) ) ;
#10101=FACE_OUTER_BOUND ( 'NONE', #19683, .T. ) ;
#10102=VECTOR ( 'NONE', #23626, 1000.000000000000114 ) ;
#10103=CARTESIAN_POINT ( 'NONE',  ( -16.86552742978648212, -21.78694546712621616, 68.71063070142631091 ) ) ;
#10104=CARTESIAN_POINT ( 'NONE',  ( -14.81535805098777736, -7.777528402031247623, 53.89198173725363716 ) ) ;
#10109=CARTESIAN_POINT ( 'NONE',  ( -10.56265612243206498, -13.42270443805417379, 74.67817617528319829 ) ) ;
#10111=CARTESIAN_POINT ( 'NONE',  ( -14.66630222544869078, -8.320656262913125545, 63.80450889863892172 ) ) ;
#10112=CARTESIAN_POINT ( 'NONE',  ( -16.55233368891663659, -22.20803663120749505, 65.32540755232676588 ) ) ;
#10114=VERTEX_POINT ( 'NONE', #36539 ) ;
#10115=ADVANCED_FACE ( 'NONE', ( #29183 ), #48699, .T. ) ;
#10117=CARTESIAN_POINT ( 'NONE',  ( -23.68301487380630377, -11.67430220541036867, 63.25218272174556944 ) ) ;
#10118=CARTESIAN_POINT ( 'NONE',  ( -23.88493932675476472, -11.09942404494770152, 70.05244096366236306 ) ) ;
#10120=LINE ( 'NONE', #2002, #30611 ) ;
#10121=CARTESIAN_POINT ( 'NONE',  ( -22.92319755143357440, -10.39759026177046941, 63.37185995336193400 ) ) ;
#10125=CARTESIAN_POINT ( 'NONE',  ( -12.89349882295773320, -9.473050026692668268, 71.07598649106860478 ) ) ;
#10127=CARTESIAN_POINT ( 'NONE',  ( -15.75476274255337472, -8.011104503670525290, 67.36680511887003320 ) ) ;
#10128=B_SPLINE_CURVE_WITH_KNOTS ( 'NONE', 3,
 ( #27343, #37428, #7679, #766, #30086, #45343, #22687, #11596, #3723, #15761 ),
 .UNSPECIFIED., .F., .F.,
 ( 4, 2, 2, 2, 4 ),
 ( 0.000000000000000000, 0.2500000000000000000, 0.5000000000000000000, 0.7500000000000000000, 1.000000000000000000 ),
 .UNSPECIFIED. ) ;
#10131=AXIS2_PLACEMENT_3D ( 'NONE', #7458, #36968, #30109 ) ;
#10132=CIRCLE ( 'NONE', #10909, 6.999999999999999112 ) ;
#10133=ORIENTED_EDGE ( 'NONE', *, *, #3829, .T. ) ;
#10134=CARTESIAN_POINT ( 'NONE',  ( -23.93648101794248362, -17.51022725521227841, 65.95829288617392194 ) ) ;
#10135=FACE_OUTER_BOUND ( 'NONE', #36829, .T. ) ;
#10136=CARTESIAN_POINT ( 'NONE',  ( -19.26582040957177355, -21.56270631561501006, 58.52507339225701344 ) ) ;
#10137=VERTEX_POINT ( 'NONE', #26219 ) ;
#10139=CARTESIAN_POINT ( 'NONE',  ( -10.27345486655506868, -12.71824029969684844, 64.45331411623358520 ) ) ;
#10140=CARTESIAN_POINT ( 'NONE',  ( -24.36611147337434957, -16.04009697885371111, 66.07797069094537790 ) ) ;
#10142=DIRECTION ( 'NONE',  ( 0.7224352045700187519, 0.6914386272098739239, -9.340627245513716657E-09 ) ) ;
#10143=CARTESIAN_POINT ( 'NONE',  ( -22.35721049598137711, -20.39193527001060957, 62.38439161571156433 ) ) ;
#10144=DIRECTION ( 'NONE',  ( -0.06498076606345576378, -0.4424675129789833461, 0.8944271909999158554 ) ) ;
#10146=CARTESIAN_POINT ( 'NONE',  ( -16.96567540528316442, -22.24509813497291333, 72.36532000937602049 ) ) ;
#10147=CARTESIAN_POINT ( 'NONE',  ( -12.05806040642128707, -10.23620046216302448, 67.51368956197082127 ) ) ;
#10148=CARTESIAN_POINT ( 'NONE',  ( -21.65914559189701194, -18.31838547852702703, 54.07175714974879099 ) ) ;
#10150=CARTESIAN_POINT ( 'NONE',  ( -18.64167402801552242, -7.915852103407403639, 70.38570403504697026 ) ) ;
#10154=ORIENTED_EDGE ( 'NONE', *, *, #46851, .T. ) ;
#10155=CARTESIAN_POINT ( 'NONE',  ( -21.29994498387370427, -20.70774380606181708, 65.74020874375150925 ) ) ;
#10157=VERTEX_POINT ( 'NONE', #45194 ) ;
#10158=CARTESIAN_POINT ( 'NONE',  ( -24.34502428176253019, -17.56683243011407924, 66.12852677468319484 ) ) ;
#10160=CARTESIAN_POINT ( 'NONE',  ( -11.75134185092603900, -18.91115923382153596, 71.70302575940529266 ) ) ;
#10161=CARTESIAN_POINT ( 'NONE',  ( -13.22576123393696967, -9.135673809461350103, 70.99358371225501685 ) ) ;
#10162=CARTESIAN_POINT ( 'NONE',  ( -19.44222556512714917, -7.637678758653525968, 60.21738930846358073 ) ) ;
#10163=CARTESIAN_POINT ( 'NONE',  ( -14.54176669294802693, -21.67913874359843973, 58.28122557424108408 ) ) ;
#10164=( BOUNDED_CURVE ( )  B_SPLINE_CURVE ( 3, ( #43839, #28566, #43595, #21428 ),
 .UNSPECIFIED., .F., .F. ) 
 B_SPLINE_CURVE_WITH_KNOTS ( ( 4, 4 ),
 ( 0.9074455897393630677, 1.000000000000000000 ),
 .UNSPECIFIED. ) 
 CURVE ( )  GEOMETRIC_REPRESENTATION_ITEM ( )  RATIONAL_B_SPLINE_CURVE ( ( 0.6983129098260874024, 0.7760317562606933173, 0.8765941196519975165, 1.000000000000000000 ) ) 
 REPRESENTATION_ITEM ( '' )  );
#10168=PLANE ( 'NONE',  #40498 ) ;
#10169=EDGE_CURVE ( 'NONE', #47803, #29080, #25125, .T. ) ;
#10171=CARTESIAN_POINT ( 'NONE',  ( -23.70099247935880982, -17.91057002971143675, 59.07548647231428163 ) ) ;
#10172=EDGE_LOOP ( 'NONE', ( #18067, #20625, #24788, #32555, #9107 ) ) ;
#10173=FACE_OUTER_BOUND ( 'NONE', #16834, .T. ) ;
#10174=CARTESIAN_POINT ( 'NONE',  ( -15.90674806925635032, -7.920628488110523335, 70.90990109588881296 ) ) ;
#10176=AXIS2_PLACEMENT_3D ( 'NONE', #27045, #7621, #22627 ) ;
#10177=EDGE_CURVE ( 'NONE', #35577, #32087, #26711, .T. ) ;
#10178=CARTESIAN_POINT ( 'NONE',  ( -23.41977899678227004, -11.19648470850049904, 73.36193302072521760 ) ) ;
#10180=CARTESIAN_POINT ( 'NONE',  ( -21.04010602215687342, -20.80440203143702149, 69.12620543858641042 ) ) ;
#10181=CARTESIAN_POINT ( 'NONE',  ( -13.65110067086344792, -21.23324738024127356, 68.57129742521463811 ) ) ;
#10182=CARTESIAN_POINT ( 'NONE',  ( -16.51569948449359515, -21.75045648492761430, 65.24181065036900407 ) ) ;
#10183=B_SPLINE_CURVE_WITH_KNOTS ( 'NONE', 1,
 ( #34942, #1211 ),
 .UNSPECIFIED., .F., .F.,
 ( 2, 2 ),
 ( 0.000000000000000000, 1.000000000000000000 ),
 .UNSPECIFIED. ) ;
#10184=( BOUNDED_CURVE ( )  B_SPLINE_CURVE ( 3, ( #20608, #27502, #5828, #9528 ),
 .UNSPECIFIED., .F., .F. ) 
 B_SPLINE_CURVE_WITH_KNOTS ( ( 4, 4 ),
 ( 0.5000000000000000000, 0.9074455897393653991 ),
 .UNSPECIFIED. ) 
 CURVE ( )  GEOMETRIC_REPRESENTATION_ITEM ( )  RATIONAL_B_SPLINE_CURVE ( ( 1.000000000000005551, 0.4567392136813330783, 0.3561768502900267697, 0.6983129098260927314 ) ) 
 REPRESENTATION_ITEM ( '' )  );
#10186=ORIENTED_EDGE ( 'NONE', *, *, #29114, .T. ) ;
#10187=ORIENTED_EDGE ( 'NONE', *, *, #35041, .F. ) ;
#10190=FACE_OUTER_BOUND ( 'NONE', #48418, .T. ) ;
#10191=CARTESIAN_POINT ( 'NONE',  ( -11.88446955661387783, -10.44372876568607467, 67.38408161429789800 ) ) ;
#10193=( BOUNDED_CURVE ( )  B_SPLINE_CURVE ( 3, ( #20247, #13562, #31331, #46360 ),
 .UNSPECIFIED., .F., .F. ) 
 B_SPLINE_CURVE_WITH_KNOTS ( ( 4, 4 ),
 ( 0.4074455897393697290, 0.5000000000000000000 ),
 .UNSPECIFIED. ) 
 CURVE ( )  GEOMETRIC_REPRESENTATION_ITEM ( )  RATIONAL_B_SPLINE_CURVE ( ( 0.6983129098261150469, 0.7760317562607150776, 0.8765941196520095069, 0.9999999999999966693 ) ) 
 REPRESENTATION_ITEM ( '' )  );
#10194=DIRECTION ( 'NONE',  ( 0.9979768094191905359, 0.06357898915123233463, -6.487762650558261530E-18 ) ) ;
#10195=CARTESIAN_POINT ( 'NONE',  ( -15.57436938376845603, -7.592477944586329741, 70.70966202169438475 ) ) ;
#10198=CARTESIAN_POINT ( 'NONE',  ( -22.86447931068992290, -19.99836516962492183, 54.02312124697528617 ) ) ;
#10200=CARTESIAN_POINT ( 'NONE',  ( -22.83929682888979329, -10.29453308790037980, 66.55654356380499337 ) ) ;
#10201=FACE_OUTER_BOUND ( 'NONE', #11246, .T. ) ;
#10202=VERTEX_POINT ( 'NONE', #37775 ) ;
#10203=CARTESIAN_POINT ( 'NONE',  ( -17.77594298899184366, -7.367433885636743618, 60.26556189360973548 ) ) ;
#10206=ORIENTED_EDGE ( 'NONE', *, *, #47557, .T. ) ;
#10209=B_SPLINE_CURVE_WITH_KNOTS ( 'NONE', 1,
 ( #5299, #38533 ),
 .UNSPECIFIED., .F., .F.,
 ( 2, 2 ),
 ( 0.000000000000000000, 1.000000000000000000 ),
 .UNSPECIFIED. ) ;
#10210=EDGE_CURVE ( 'NONE', #43576, #37207, #35175, .T. ) ;
#10211=CARTESIAN_POINT ( 'NONE',  ( -10.69327888247252467, -16.91860816364039621, 61.24923186240393136 ) ) ;
#10214=CARTESIAN_POINT ( 'NONE',  ( -22.33161753753789469, -20.41455022152800325, 62.49085083065315160 ) ) ;
#10216=CARTESIAN_POINT ( 'NONE',  ( -21.57995947450667984, -9.113990939708573435, 70.14604673427196246 ) ) ;
#10217=CARTESIAN_POINT ( 'NONE',  ( -12.03178671929730115, -10.26761072191531277, 67.49896879719585741 ) ) ;
#10221=PLANE ( 'NONE',  #7050 ) ;
#10222=CARTESIAN_POINT ( 'NONE',  ( -12.01648161716052954, -10.28590799842451098, 67.79896869921920199 ) ) ;
#10223=VERTEX_POINT ( 'NONE', #19310 ) ;
#10225=VECTOR ( 'NONE', #17918, 1000.000000000000114 ) ;
#10229=CARTESIAN_POINT ( 'NONE',  ( -17.02791773878522719, -7.770306534664505271, 73.96018283094906565 ) ) ;
#10231=VERTEX_POINT ( 'NONE', #29918 ) ;
#10235=EDGE_CURVE ( 'NONE', #6219, #39482, #38023, .T. ) ;
#10236=CARTESIAN_POINT ( 'NONE',  ( -23.72107644662085590, -11.75175493167614427, 59.59121838756593803 ) ) ;
#10237=CARTESIAN_POINT ( 'NONE',  ( -16.00334498133122096, -7.954840756278199088, 63.95545613112251004 ) ) ;
#10241=EDGE_CURVE ( 'NONE', #18786, #26541, #5166, .T. ) ;
#10244=FACE_OUTER_BOUND ( 'NONE', #47889, .T. ) ;
#10250=CARTESIAN_POINT ( 'NONE',  ( -15.39235221195410652, -21.97689038623625635, 72.08929527613493349 ) ) ;
#10251=CARTESIAN_POINT ( 'NONE',  ( -24.87421248883078917, -14.80150407957441061, 59.36487506370225731 ) ) ;
#10252=AXIS2_PLACEMENT_3D ( 'NONE', #13364, #34813, #16085 ) ;
#10254=DIRECTION ( 'NONE',  ( 4.924618305738831318E-06, 4.007739938527551184E-06, 0.9999999999798430128 ) ) ;
#10255=ORIENTED_EDGE ( 'NONE', *, *, #40879, .F. ) ;
#10257=CARTESIAN_POINT ( 'NONE',  ( -10.43158760916531591, -13.88200553355761713, 61.21821478144431694 ) ) ;
#10258=CARTESIAN_POINT ( 'NONE',  ( -9.995738443926455830, -14.24059931954510816, 64.50308448303212572 ) ) ;
#10259=CLOSED_SHELL ( 'NONE', ( #22850, #44015, #137, #21554, #22902, #37205, #46705, #44406, #40620, #40007, #20806, #22460, #11338, #27811, #5679, #13135, #8518, #22405, #20876, #19507, #7659, #28880, #21414, #8616, #10502, #21618, #44668, #24572, #47905, #1636, #2540, #488, #5668, #32169, #18750, #28499, #22292, #22398, #35834, #9384, #42155, #6273, #24561, #16350, #38827, #44060, #32773, #27136, #18460, #34621, #48289, #16761, #22922, #34561, #18375, #17902, #29264, #47146, #21453, #45135, #3108, #28587, #33489, #44343, #18521, #10754, #35895, #26377, #38576, #7473, #19318, #25436, #16992, #40760, #34213, #32757, #47923, #48138, #17777, #28173, #16710, #3597, #25773, #1547, #34421, #3269, #42832, #28006, #44818, #20661, #7599, #4958, #11825, #15594, #42264, #20049, #42571, #21952, #31634, #37403, #2316, #37701, #23011, #22077, #29985, #36115, #14279, #39383, #10919, #38514, #26267, #23458, #24571, #265, #35438, #25966, #25868, #20825, #24419, #48500, #40344, #37964, #38512, #11438, #20991, #45091, #2798, #18262, #6423, #35649, #3000, #9702, #9410, #11441, #26855, #9791, #843, #45783, #19206, #6546, #42647, #8467, #24730, #30680, #28687, #32076, #974, #43058, #4914, #38236, #9216, #5928, #41559, #36433, #9289, #8333, #10832, #1909, #21683, #43112, #15723, #14010, #46034, #3374, #28894, #21013, #46197, #36973, #36647, #42963, #41864, #23350, #46297, #42574, #20877, #15921, #30002, #38719, #35837, #12678, #26921, #30753, #3473, #3203, #5238, #26116, #34820, #7728, #32181, #41710, #6836, #1813, #8603, #9192, #3664, #28449, #41612, #38999, #31034, #8879, #29745, #8140, #25053, #41797, #27471, #18183, #13627, #34210, #6212, #13288, #42955, #24849, #24358, #43179, #14437, #22359, #40434, #13674, #5977, #25674, #40994, #42287, #15236, #15244, #2711, #47471, #34616, #8443, #15738, #4706, #31990, #20323, #43079, #28040, #10837, #28556, #16050, #40097, #37588, #17912, #20406, #10115, #28386, #12008, #42646, #14572, #16912, #26400, #44263, #16759, #31640, #14085, #36591, #47485, #4021, #24019, #20674, #40209, #984, #2241, #37828, #40690, #23616, #22916, #33453, #3907, #28220, #4426, #25409, #5203, #19092, #15970, #38106, #43454, #15813, #33367, #5604, #17282, #43733, #19616, #14138, #46632, #20537, #32307, #17239, #13410, #17373, #45426, #20526, #12651, #9844, #11445, #18758, #39183, #17308, #24426, #40756, #35563, #45604, #41076, #22701, #43015, #32564, #25169, #45349, #17421, #13826, #36039, #18128, #15299, #47189, #22807, #20518, #6141, #29038, #28348, #8132, #24294, #29657, #15742, #31476, #29073, #43444, #47861, #12780, #3138, #31376, #13371, #13176, #21675, #20838, #23126, #27416, #24260, #39820, #2, #17023, #7493, #43318, #33323, #41454, #47852, #29395, #21471, #9435, #42033, #15452, #23088, #33235, #12534, #18633, #17313, #19910, #16258, #17717, #5529, #4767, #27437, #21005, #8194, #36930, #28450, #34148, #23737, #15428, #37296, #5320, #22981, #23674, #37622, #32595, #46710, #13253, #37708, #47598, #39343, #22037, #22372, #26029, #25459, #27716, #32662, #1665, #3758, #1849, #27210, #34012, #32341, #14658, #36316, #3553, #10666, #43687, #43032, #33954, #47338, #15916, #39466, #20400, #45242, #7979, #12982, #5982, #39774, #21789, #15870, #2909, #21211, #39740, #22348, #15401, #2438, #46290, #13431, #15315, #36107, #47466, #41643, #13946, #33047, #31773, #29518, #12215, #33577, #8798, #24229, #36927, #21421, #31159, #11952, #32313, #1258, #9585, #39414, #30269, #283, #16413, #29120, #35073, #46439, #2919, #31285, #22999, #437, #42019, #42309, #7031, #46239, #15398, #16131, #35508, #15629, #37053, #19090, #25698, #21672, #36267, #2225, #32837, #8129, #28072, #44269, #10377, #22534, #33104, #31134, #35155, #8077, #14309, #9635, #2780, #11588, #17152, #5674, #24164, #34059, #9112, #3460, #32794, #14361, #18586, #33247, #4678, #13210, #12590, #30558, #16809, #23885, #13732, #9066, #893, #21446, #46405, #4617, #17842, #31651, #7453, #32395, #22234, #13621, #6049, #31230, #27877, #25616, #39897, #32623, #45273, #10461, #2323, #4723, #27846, #6073, #277, #2532, #40439, #11047, #31618, #1638, #21344, #29015, #39361, #338, #825, #39615, #7378, #24509, #5041, #22787, #5103, #3841, #43509, #33635, #4897, #17926, #39484, #28379, #47785, #157, #43237, #47782, #23889, #556, #11883, #2424, #27951, #39750, #42018, #13181, #48630, #13567, #38591, #14552, #7859, #39118, #438, #14829, #25490, #2321, #10700, #44943, #21606, #30401, #19603, #16804, #22016, #32582, #16078, #22580, #5061, #44609, #39755, #42351, #19930, #12731, #10827, #9640, #5997, #19374, #46698, #26016, #22353, #41648, #27069, #1293, #27616, #24505, #10824, #26690, #26782, #18042, #15186, #29739, #17165, #39800, #8249, #23392, #10562, #29210, #35318, #10643, #43374, #41408, #1427, #6665, #28002, #13003, #1440, #21261, #2238, #37006, #34361, #606, #45408, #27889, #4490, #24831, #19352, #7287, #39677, #22962, #30636, #14091, #19994, #26322, #5282, #2187, #35922, #11948, #15534, #3879, #37084, #24772, #13623, #41743, #16149, #36388, #42510, #45035, #36573, #48729, #20417, #13052, #3820, #8511, #12808, #36719, #28634, #18508, #47297, #15431, #15812, #17366, #8495, #30208, #8561, #17631, #32843, #13687, #17090, #35782, #26731, #37222, #20321, #2538, #41221, #1345, #10780, #36998, #29942, #48020, #34484, #18532, #28515, #42700, #19548, #44948, #5374, #28691, #4044, #21885, #7950, #8066, #43710, #44894, #45503, #42632, #4228, #4367, #1322, #2910, #24349, #21571, #14066, #43459, #17518, #31520, #36153, #5526, #43073, #43787, #34892, #26602, #15251, #14142, #7653, #34182, #12823, #30422, #39059, #18892, #28944, #39674, #19135, #6682, #14337, #926, #13201, #6808, #9398, #33977, #11184, #8752, #43405, #31128, #29871, #19849, #46850, #22420, #40972, #38161, #36704, #31172, #48720, #11269, #45052, #10092, #10067, #10710, #23005, #945, #30715, #19437, #45427, #48378, #15074, #11388, #14965, #29880, #9129, #10318, #26321, #6669, #30023, #29056, #32933, #9430, #16315, #25192, #35374, #5393, #16154, #4049, #21065, #29362, #14971, #3408, #4878, #37659, #33137, #34593, #45210, #28364, #36522, #14418, #14667, #29063, #43869, #19986, #45373, #23940, #9823, #29180, #24861, #34334, #28172, #22267, #23206, #44795, #47380, #14489, #44329, #6142, #4917, #35312, #40686, #1411, #2185, #34849, #32126, #39419, #12063, #8740, #34500, #24995, #24560, #20606, #47606, #45758, #22796, #17646, #47192, #29187, #1639, #42633, #11788, #27204, #25990, #8743, #41235, #4586, #31020, #25828, #12758, #38522, #20550, #36675, #19167, #7413, #14386, #11532, #2050, #48130, #42433, #32028, #32973 ) ) ;
#10260=ORIENTED_EDGE ( 'NONE', *, *, #4498, .F. ) ;
#10262=( BOUNDED_CURVE ( )  B_SPLINE_CURVE ( 3, ( #44491, #30450, #10993, #14640 ),
 .UNSPECIFIED., .F., .F. ) 
 B_SPLINE_CURVE_WITH_KNOTS ( ( 4, 4 ),
 ( 0.5000000000000000000, 0.9074455897393685078 ),
 .UNSPECIFIED. ) 
 CURVE ( )  GEOMETRIC_REPRESENTATION_ITEM ( )  RATIONAL_B_SPLINE_CURVE ( ( 0.9999999999999921174, 0.4567392136813224202, 0.3561768502900321542, 0.6983129098261128265 ) ) 
 REPRESENTATION_ITEM ( '' )  );
#10263=EDGE_CURVE ( 'NONE', #12881, #25767, #40225, .T. ) ;
#10264=CARTESIAN_POINT ( 'NONE',  ( -22.78885683033217902, -10.31261690998277381, 63.26289122890993610 ) ) ;
#10266=VERTEX_POINT ( 'NONE', #38506 ) ;
#10268=DIRECTION ( 'NONE',  ( 1.590464103011092396E-07, -3.579926632912963412E-07, 0.9999999999999231726 ) ) ;
#10269=CARTESIAN_POINT ( 'NONE',  ( -23.91010245674826251, -17.57297063409389537, 62.75888927877479517 ) ) ;
#10270=ORIENTED_EDGE ( 'NONE', *, *, #12721, .F. ) ;
#10271=CARTESIAN_POINT ( 'NONE',  ( -13.72009916595086132, -20.81131062084115513, 61.40157432139535842 ) ) ;
#10272=B_SPLINE_CURVE_WITH_KNOTS ( 'NONE', 1,
 ( #10427, #2772 ),
 .UNSPECIFIED., .F., .F.,
 ( 2, 2 ),
 ( 0.000000000000000000, 1.000000000000000000 ),
 .UNSPECIFIED. ) ;
#10274=DIRECTION ( 'NONE',  ( -5.731567514496413899E-31, -1.020425574103664789E-16, -1.000000000000000000 ) ) ;
#10275=CARTESIAN_POINT ( 'NONE',  ( -24.44253391677669285, -17.31023895159264470, 73.06991310009190954 ) ) ;
#10276=CARTESIAN_POINT ( 'NONE',  ( -22.68242704663779108, -10.18794451883025154, 70.29561946466137101 ) ) ;
#10277=EDGE_LOOP ( 'NONE', ( #27575, #7237, #25909, #11918, #35859 ) ) ;
#10280=ORIENTED_EDGE ( 'NONE', *, *, #34771, .F. ) ;
#10282=FACE_OUTER_BOUND ( 'NONE', #36666, .T. ) ;
#10283=ORIENTED_EDGE ( 'NONE', *, *, #25985, .F. ) ;
#10288=B_SPLINE_CURVE_WITH_KNOTS ( 'NONE', 3,
 ( #47538, #23927, #42879, #9146, #8909, #39421, #46812, #32029, #43116, #39899 ),
 .UNSPECIFIED., .F., .F.,
 ( 4, 2, 2, 2, 4 ),
 ( 0.000000000000000000, 0.2500000000000000000, 0.5000000000000000000, 0.7500000000000000000, 1.000000000000000000 ),
 .UNSPECIFIED. ) ;
#10289=VECTOR ( 'NONE', #43254, 999.9999999999998863 ) ;
#10290=CARTESIAN_POINT ( 'NONE',  ( -10.13751350317288669, -13.25697809452625009, 74.93463578866538910 ) ) ;
#10291=CARTESIAN_POINT ( 'NONE',  ( -19.37484620200115160, -7.619050568204919216, 60.14588398245204814 ) ) ;
#10292=CARTESIAN_POINT ( 'NONE',  ( -23.81024772113315890, -18.64597811008791695, 72.94863512192290500 ) ) ;
#10293=CYLINDRICAL_SURFACE ( 'NONE', #3517, 0.1499999999999998002 ) ;
#10294=CARTESIAN_POINT ( 'NONE',  ( -22.65953014494242979, -19.53520302830625965, 72.52911954723420251 ) ) ;
#10295=VERTEX_POINT ( 'NONE', #16815 ) ;
#10296=VERTEX_POINT ( 'NONE', #20541 ) ;
#10297=EDGE_CURVE ( 'NONE', #34062, #43456, #5274, .T. ) ;
#10298=CARTESIAN_POINT ( 'NONE',  ( -10.42334066387008029, -15.64104445138816146, 61.03789045260960222 ) ) ;
#10299=AXIS2_PLACEMENT_3D ( 'NONE', #38035, #37292, #38267 ) ;
#10300=CARTESIAN_POINT ( 'NONE',  ( -17.18707620353899301, -7.362977788511615884, 70.64035839947293027 ) ) ;
#10301=PLANE ( 'NONE',  #18133 ) ;
#10302=FACE_OUTER_BOUND ( 'NONE', #18054, .T. ) ;
#10304=CARTESIAN_POINT ( 'NONE',  ( -18.54561167675666411, -7.443937692776573911, 73.97917849299003024 ) ) ;
#10306=VERTEX_POINT ( 'NONE', #46643 ) ;
#10307=CARTESIAN_POINT ( 'NONE',  ( -14.80056043599933524, -21.78207186541723317, 61.82095768364339960 ) ) ;
#10310=CARTESIAN_POINT ( 'NONE',  ( -14.47651980493331081, -8.396190447208750740, 60.47563573450432273 ) ) ;
#10312=( BOUNDED_CURVE ( )  B_SPLINE_CURVE ( 3, ( #40976, #48598, #22504, #48118 ),
 .UNSPECIFIED., .F., .F. ) 
 B_SPLINE_CURVE_WITH_KNOTS ( ( 4, 4 ),
 ( 0.000000000000000000, 0.4074455897393696735 ),
 .UNSPECIFIED. ) 
 CURVE ( )  GEOMETRIC_REPRESENTATION_ITEM ( )  RATIONAL_B_SPLINE_CURVE ( ( 1.000000000000000000, 0.4567392136813212544, 0.3561768502900263256, 0.6983129098261152690 ) ) 
 REPRESENTATION_ITEM ( '' )  );
#10314=VERTEX_POINT ( 'NONE', #27429 ) ;
#10318=ADVANCED_FACE ( 'NONE', ( #32099 ), #46147, .T. ) ;
#10319=CARTESIAN_POINT ( 'NONE',  ( -22.48964968825576705, -9.905448439006629968, 73.76689030015370463 ) ) ;
#10321=B_SPLINE_CURVE_WITH_KNOTS ( 'NONE', 3,
 ( #9260, #13416, #39773, #39535, #24286, #2348, #6040, #17358, #39293, #43729 ),
 .UNSPECIFIED., .F., .F.,
 ( 4, 2, 2, 2, 4 ),
 ( 0.000000000000000000, 0.2500000000000000000, 0.5000000000000000000, 0.7500000000000000000, 1.000000000000000000 ),
 .UNSPECIFIED. ) ;
#10322=ORIENTED_EDGE ( 'NONE', *, *, #752, .T. ) ;
#10324=( BOUNDED_SURFACE ( )  B_SPLINE_SURFACE ( 3, 1, ( 
 ( #2558, #33049 ),
 ( #17557, #36986 ),
 ( #6498, #21747 ),
 ( #29136, #6973 ),
 ( #3278, #32816 ),
 ( #25676, #48323 ),
 ( #41191, #48092 ) ),
 .UNSPECIFIED., .T., .F., .F. ) 
 B_SPLINE_SURFACE_WITH_KNOTS ( ( 4, 3, 4 ),
 ( 2, 2 ),
 ( 0.000000000000000000, 0.5000000000000000000, 1.000000000000000000 ),
 ( 0.000000000000000000, 1.000000000000000000 ),
 .UNSPECIFIED. ) 
 GEOMETRIC_REPRESENTATION_ITEM ( )  RATIONAL_B_SPLINE_SURFACE ( (
 ( 1.000000000000000000, 1.000000000000000000),
 ( 0.3333333333333335369, 0.3333333333333330373),
 ( 0.3333333333333335369, 0.3333333333333330373),
 ( 1.000000000000000000, 1.000000000000000000),
 ( 0.3333333333333333703, 0.3333333333333333703),
 ( 0.3333333333333333703, 0.3333333333333333703),
 ( 1.000000000000000000, 1.000000000000000000) ) ) 
 REPRESENTATION_ITEM ( '' )  SURFACE ( )  );
#10325=ORIENTED_EDGE ( 'NONE', *, *, #24685, .T. ) ;
#10326=CARTESIAN_POINT ( 'NONE',  ( -22.28468842640967651, -19.91619389767071269, 65.98949666203347419 ) ) ;
#10328=B_SPLINE_CURVE_WITH_KNOTS ( 'NONE', 1,
 ( #42115, #19950 ),
 .UNSPECIFIED., .F., .F.,
 ( 2, 2 ),
 ( 0.000000000000000000, 1.000000000000000000 ),
 .UNSPECIFIED. ) ;
#10329=ORIENTED_EDGE ( 'NONE', *, *, #19969, .T. ) ;
#10331=AXIS2_PLACEMENT_3D ( 'NONE', #21816, #14632, #14886 ) ;
#10332=CARTESIAN_POINT ( 'NONE',  ( -12.95250271175661183, -20.26353575427058828, 71.69165012371371404 ) ) ;
#10334=CARTESIAN_POINT ( 'NONE',  ( -22.38400322090610217, -20.36826016184844335, 62.41934579407823236 ) ) ;
#10336=CARTESIAN_POINT ( 'NONE',  ( -19.94917705995926482, -8.226604131702123013, 74.00624557436877637 ) ) ;
#10338=CARTESIAN_POINT ( 'NONE',  ( -13.53325622885376944, -21.16256470055228789, 65.17124264509627096 ) ) ;
#10339=CARTESIAN_POINT ( 'NONE',  ( -17.29268214306257434, -7.359616301281327821, 70.67691090883880634 ) ) ;
#10343=ORIENTED_EDGE ( 'NONE', *, *, #22169, .F. ) ;
#10344=VERTEX_POINT ( 'NONE', #12406 ) ;
#10345=AXIS2_PLACEMENT_3D ( 'NONE', #18199, #25846, #44334 ) ;
#10346=CARTESIAN_POINT ( 'NONE',  ( -22.48964968825576705, -9.905448439006629968, 73.76689030015370463 ) ) ;
#10347=CARTESIAN_POINT ( 'NONE',  ( -24.68275079258767235, -16.48720463981601370, 59.23837148777906236 ) ) ;
#10349=DIRECTION ( 'NONE',  ( 0.8788484374452878445, -0.3260506722428093695, 0.3483050145059469749 ) ) ;
#10352=CARTESIAN_POINT ( 'NONE',  ( -12.95651447042595095, -9.351591191262567548, 67.26453940287311184 ) ) ;
#10353=CARTESIAN_POINT ( 'NONE',  ( -23.70429433613102432, -18.81713154275495370, 69.47088838593184335 ) ) ;
#10357=CARTESIAN_POINT ( 'NONE',  ( -21.97751765269923041, -20.19167113790911827, 59.05883102620609293 ) ) ;
#10358=CARTESIAN_POINT ( 'NONE',  ( -14.10256296019058198, -8.140532706836228982, 70.84462314181931220 ) ) ;
#10361=FACE_OUTER_BOUND ( 'NONE', #35168, .T. ) ;
#10362=CARTESIAN_POINT ( 'NONE',  ( -16.57554889599778747, -22.21081103083016117, 65.41059783760971413 ) ) ;
#10365=CARTESIAN_POINT ( 'NONE',  ( -20.58212643533483543, -8.561992128821106718, 60.06798555086853497 ) ) ;
#10366=VECTOR ( 'NONE', #45829, 1000.000000000000000 ) ;
#10369=CARTESIAN_POINT ( 'NONE',  ( -11.67943375510494874, -18.89645239624664796, 68.50217487844219022 ) ) ;
#10370=ORIENTED_EDGE ( 'NONE', *, *, #44467, .T. ) ;
#10371=EDGE_CURVE ( 'NONE', #22230, #36064, #5785, .T. ) ;
#10372=CARTESIAN_POINT ( 'NONE',  ( -16.20608744287016023, -7.459440102232786529, 60.40039685254514978 ) ) ;
#10373=VECTOR ( 'NONE', #24305, 1000.000000000000114 ) ;
#10375=EDGE_CURVE ( 'NONE', #23048, #9317, #6564, .T. ) ;
#10377=ADVANCED_FACE ( 'NONE', ( #25664 ), #39726, .T. ) ;
#10378=ORIENTED_EDGE ( 'NONE', *, *, #41515, .T. ) ;
#10380=CARTESIAN_POINT ( 'NONE',  ( -22.33041860316855320, -20.41560964288588664, 62.34943852502606632 ) ) ;
#10381=CARTESIAN_POINT ( 'NONE',  ( -24.46737407909346373, -14.43901797238471474, 62.59807894131280648 ) ) ;
#10382=CARTESIAN_POINT ( 'NONE',  ( -21.94839310389095033, -8.890257795104481886, 66.85488308860405482 ) ) ;
#10383=ORIENTED_EDGE ( 'NONE', *, *, #12231, .F. ) ;
#10385=ORIENTED_EDGE ( 'NONE', *, *, #11882, .T. ) ;
#10386=CARTESIAN_POINT ( 'NONE',  ( -24.47066272824306665, -14.57993217219608972, 62.99824437345091610 ) ) ;
#10388=CARTESIAN_POINT ( 'NONE',  ( -22.29619887594318683, -17.36118473213641167, 53.49999999999995026 ) ) ;
#10389=ORIENTED_EDGE ( 'NONE', *, *, #8608, .T. ) ;
#10390=DIRECTION ( 'NONE',  ( -0.7171836970970658642, 0.6968841687240311389, -4.479616660400631173E-09 ) ) ;
#10391=CARTESIAN_POINT ( 'NONE',  ( -24.45125044792649049, -12.33277093510790579, 73.35570258362008644 ) ) ;
#10393=CARTESIAN_POINT ( 'NONE',  ( -10.75331649400429868, -16.93069871048427544, 57.68760548944693056 ) ) ;
#10396=ORIENTED_EDGE ( 'NONE', *, *, #20607, .F. ) ;
#10399=CARTESIAN_POINT ( 'NONE',  ( -13.35685195715142193, -21.05109796036597913, 61.56000367517481919 ) ) ;
#10400=FACE_OUTER_BOUND ( 'NONE', #28624, .T. ) ;
#10401=CARTESIAN_POINT ( 'NONE',  ( -24.25940922233440489, -13.08205373389642823, 63.12704356492964308 ) ) ;
#10402=EDGE_CURVE ( 'NONE', #566, #41338, #10272, .T. ) ;
#10403=VERTEX_POINT ( 'NONE', #14073 ) ;
#10405=CARTESIAN_POINT ( 'NONE',  ( -16.90447226888101895, -21.79033282223921830, 72.44926656220420114 ) ) ;
#10408=CARTESIAN_POINT ( 'NONE',  ( -24.05923365589681140, -11.41972516488058176, 66.60869825954527812 ) ) ;
#10410=CARTESIAN_POINT ( 'NONE',  ( -24.21255563026993940, -13.09477139695512449, 66.49173888256298426 ) ) ;
#10411=CARTESIAN_POINT ( 'NONE',  ( -12.00790786851990610, -10.29148984397945377, 63.91425679989585973 ) ) ;
#10412=CARTESIAN_POINT ( 'NONE',  ( -22.24723880939002996, -9.656319818818069223, 59.86604062818025795 ) ) ;
#10413=B_SPLINE_CURVE_WITH_KNOTS ( 'NONE', 3,
 ( #45999, #4884, #27517, #31212, #35621, #38840, #42788, #12254, #15937, #1899 ),
 .UNSPECIFIED., .F., .F.,
 ( 4, 2, 2, 2, 4 ),
 ( 0.6272669072878207519, 0.7522669073073100510, 0.8772669073267994611, 1.002266907346288871, 1.127266907365778170 ),
 .UNSPECIFIED. ) ;
#10415=FACE_BOUND ( 'NONE', #28422, .T. ) ;
#10416=CARTESIAN_POINT ( 'NONE',  ( -24.82842054764507367, -13.98508042741895352, 73.22933195708579035 ) ) ;
#10417=CARTESIAN_POINT ( 'NONE',  ( -10.42366004362047960, -14.81678656420000095, 74.81395567366212163 ) ) ;
#10422=EDGE_CURVE ( 'NONE', #22327, #39973, #8718, .T. ) ;
#10423=CARTESIAN_POINT ( 'NONE',  ( -10.50429924535250414, -16.15944446069506668, 71.46222527016213633 ) ) ;
#10424=CARTESIAN_POINT ( 'NONE',  ( -20.84178545912654457, -21.42902457554051310, 58.84486364983385442 ) ) ;
#10425=CARTESIAN_POINT ( 'NONE',  ( -20.00946539473887142, -8.250368680643830999, 73.87096600125035195 ) ) ;
#10426=B_SPLINE_CURVE_WITH_KNOTS ( 'NONE', 3,
 ( #27233, #4580, #34856, #38548, #1123, #46192, #15650, #20085, #45474, #42259 ),
 .UNSPECIFIED., .F., .F.,
 ( 4, 2, 2, 2, 4 ),
 ( 0.6272669072977097304, 0.7522669073147462138, 0.8772669073317826971, 1.002266907348819291, 1.127266907365855664 ),
 .UNSPECIFIED. ) ;
#10427=CARTESIAN_POINT ( 'NONE',  ( -24.47066272824306665, -14.57993217219608972, 62.99824437345091610 ) ) ;
#10428=ORIENTED_EDGE ( 'NONE', *, *, #2445, .T. ) ;
#10429=ORIENTED_EDGE ( 'NONE', *, *, #46030, .T. ) ;
#10432=CARTESIAN_POINT ( 'NONE',  ( -16.26184114368905043, -7.855670183028919062, 60.20028478909662795 ) ) ;
#10433=CARTESIAN_POINT ( 'NONE',  ( -11.77745829805909850, -9.948221969229217976, 67.68552175396945358 ) ) ;
#10434=CARTESIAN_POINT ( 'NONE',  ( -27.30749335439299585, -15.43885699713180770, 53.49999999999995026 ) ) ;
#10435=EDGE_CURVE ( 'NONE', #33004, #32745, #47246, .T. ) ;
#10436=EDGE_CURVE ( 'NONE', #20304, #41932, #25200, .T. ) ;
#10437=CARTESIAN_POINT ( 'NONE',  ( -15.59973365315860150, -7.586021664999528902, 70.71015599988244560 ) ) ;
#10438=ORIENTED_EDGE ( 'NONE', *, *, #39533, .T. ) ;
#10439=CARTESIAN_POINT ( 'NONE',  ( -21.10170628810619675, -20.76538187170625349, 65.81127219879576273 ) ) ;
#10440=PLANE ( 'NONE',  #23360 ) ;
#10442=CARTESIAN_POINT ( 'NONE',  ( -19.14414919534269899, -7.968427671776686871, 67.20072066290214252 ) ) ;
#10444=VERTEX_POINT ( 'NONE', #6486 ) ;
#10445=EDGE_CURVE ( 'NONE', #42966, #42781, #13724, .T. ) ;
#10447=CARTESIAN_POINT ( 'NONE',  ( -17.83973810966541862, -7.370757045899419602, 60.18786608788675352 ) ) ;
#10450=EDGE_LOOP ( 'NONE', ( #6322, #21787, #46013, #38643, #36669 ) ) ;
#10451=CARTESIAN_POINT ( 'NONE',  ( -20.18142963041198357, -7.888199563509442847, 73.91434887155375577 ) ) ;
#10452=EDGE_CURVE ( 'NONE', #11801, #42866, #11592, .T. ) ;
#10453=CARTESIAN_POINT ( 'NONE',  ( -23.32920216380910006, -18.57114719142387216, 72.87441430430278899 ) ) ;
#10454=( BOUNDED_CURVE ( )  B_SPLINE_CURVE ( 3, ( #13450, #36101, #6572, #47451 ),
 .UNSPECIFIED., .F., .F. ) 
 B_SPLINE_CURVE_WITH_KNOTS ( ( 4, 4 ),
 ( 0.4074455897393662318, 0.5000000000000000000 ),
 .UNSPECIFIED. ) 
 CURVE ( )  GEOMETRIC_REPRESENTATION_ITEM ( )  RATIONAL_B_SPLINE_CURVE ( ( 0.6983129098260973944, 0.7760317562607075281, 0.8765941196520100620, 1.000000000000008882 ) ) 
 REPRESENTATION_ITEM ( '' )  );
#10455=CARTESIAN_POINT ( 'NONE',  ( -15.49795884165273918, -21.59473877286356114, 68.78412844181838182 ) ) ;
#10456=ORIENTED_EDGE ( 'NONE', *, *, #19969, .F. ) ;
#10457=CARTESIAN_POINT ( 'NONE',  ( -20.00946503018472811, -8.250368534377352958, 73.72096600125085786 ) ) ;
#10458=CARTESIAN_POINT ( 'NONE',  ( -10.74932326624039014, -12.70011325730971130, 60.81356021554577751 ) ) ;
#10460=CARTESIAN_POINT ( 'NONE',  ( -11.43058294688041165, -10.38410865082031442, 74.48239070398270201 ) ) ;
#10461=ADVANCED_FACE ( 'NONE', ( #9934 ), #18019, .T. ) ;
#10462=CARTESIAN_POINT ( 'NONE',  ( -16.09168231696496676, -7.478562553351938647, 60.31373090009974902 ) ) ;
#10463=CYLINDRICAL_SURFACE ( 'NONE', #15859, 0.1499999999999991063 ) ;
#10464=ORIENTED_EDGE ( 'NONE', *, *, #42731, .F. ) ;
#10466=FACE_OUTER_BOUND ( 'NONE', #20496, .T. ) ;
#10467=CARTESIAN_POINT ( 'NONE',  ( -11.74181906717938695, -9.990828761398780955, 67.63863502377336090 ) ) ;
#10468=( BOUNDED_SURFACE ( )  B_SPLINE_SURFACE ( 3, 1, ( 
 ( #32607, #47631 ),
 ( #13864, #28910 ),
 ( #26432, #22252 ),
 ( #3294, #36751 ),
 ( #45168, #25947 ),
 ( #33802, #14340 ),
 ( #22011, #6750 ) ),
 .UNSPECIFIED., .T., .F., .F. ) 
 B_SPLINE_SURFACE_WITH_KNOTS ( ( 4, 3, 4 ),
 ( 2, 2 ),
 ( 0.000000000000000000, 0.5000000000000000000, 1.000000000000000000 ),
 ( 0.000000000000000000, 1.000000000000000000 ),
 .UNSPECIFIED. ) 
 GEOMETRIC_REPRESENTATION_ITEM ( )  RATIONAL_B_SPLINE_SURFACE ( (
 ( 1.000000000000000000, 1.000000000000000000),
 ( 0.3333333333333335369, 0.3333333333333330373),
 ( 0.3333333333333335369, 0.3333333333333330373),
 ( 1.000000000000000000, 1.000000000000000000),
 ( 0.3333333333333333703, 0.3333333333333333703),
 ( 0.3333333333333333703, 0.3333333333333333703),
 ( 1.000000000000000000, 1.000000000000000000) ) ) 
 REPRESENTATION_ITEM ( '' )  SURFACE ( )  );
#10471=FACE_OUTER_BOUND ( 'NONE', #18278, .T. ) ;
#10472=ORIENTED_EDGE ( 'NONE', *, *, #6592, .F. ) ;
#10473=ORIENTED_EDGE ( 'NONE', *, *, #31968, .T. ) ;
#10474=VERTEX_POINT ( 'NONE', #48313 ) ;
#10477=CARTESIAN_POINT ( 'NONE',  ( -16.03800433270414061, -7.947685453143400913, 63.67010977152477835 ) ) ;
#10478=CARTESIAN_POINT ( 'NONE',  ( -13.18362886651731358, -8.683667069837246899, 60.62445550483372614 ) ) ;
#10479=( BOUNDED_SURFACE ( )  B_SPLINE_SURFACE ( 3, 1, ( 
 ( #12024, #34664 ),
 ( #23841, #15694 ),
 ( #37871, #34168 ),
 ( #46241, #19894 ),
 ( #30982, #15440 ),
 ( #20132, #34900 ),
 ( #27518, #8827 ) ),
 .UNSPECIFIED., .T., .F., .F. ) 
 B_SPLINE_SURFACE_WITH_KNOTS ( ( 4, 3, 4 ),
 ( 2, 2 ),
 ( 0.000000000000000000, 0.5000000000000000000, 1.000000000000000000 ),
 ( 0.000000000000000000, 1.000000000000000000 ),
 .UNSPECIFIED. ) 
 GEOMETRIC_REPRESENTATION_ITEM ( )  RATIONAL_B_SPLINE_SURFACE ( (
 ( 1.000000000000000000, 1.000000000000000000),
 ( 0.3333333333333335369, 0.3333333333333330373),
 ( 0.3333333333333335369, 0.3333333333333330373),
 ( 1.000000000000000000, 1.000000000000000000),
 ( 0.3333333333333333703, 0.3333333333333333703),
 ( 0.3333333333333333703, 0.3333333333333333703),
 ( 1.000000000000000000, 1.000000000000000000) ) ) 
 REPRESENTATION_ITEM ( '' )  SURFACE ( )  );
#10480=ORIENTED_EDGE ( 'NONE', *, *, #48262, .T. ) ;
#10481=ORIENTED_EDGE ( 'NONE', *, *, #36881, .T. ) ;
#10483=CARTESIAN_POINT ( 'NONE',  ( -20.31649760022732565, -7.943510736669368910, 70.43595667626200907 ) ) ;
#10484=DIRECTION ( 'NONE',  ( -0.8507615431891571989, 0.5255518971808581519, 6.876821558984484920E-08 ) ) ;
#10485=EDGE_CURVE ( 'NONE', #34833, #38205, #24952, .T. ) ;
#10487=ORIENTED_EDGE ( 'NONE', *, *, #27251, .F. ) ;
#10488=EDGE_CURVE ( 'NONE', #39530, #45924, #43144, .T. ) ;
#10489=FACE_OUTER_BOUND ( 'NONE', #28890, .T. ) ;
#10491=CARTESIAN_POINT ( 'NONE',  ( -21.73662441638723308, -9.231682010981758779, 66.67622112302015580 ) ) ;
#10492=EDGE_LOOP ( 'NONE', ( #35711, #683, #853, #6850, #23560 ) ) ;
#10493=CARTESIAN_POINT ( 'NONE',  ( -23.96075626263749569, -17.45014286185010732, 66.24357239682277054 ) ) ;
#10497=CARTESIAN_POINT ( 'NONE',  ( -10.13106001268971212, -16.33070171280459704, 71.64024510068948359 ) ) ;
#10498=CARTESIAN_POINT ( 'NONE',  ( -12.45873566688477929, -9.804017486950373339, 57.10407583662104258 ) ) ;
#10501=CARTESIAN_POINT ( 'NONE',  ( -22.83095840648717711, -19.93459376977450859, 72.82895984417613988 ) ) ;
#10502=ADVANCED_FACE ( 'NONE', ( #33514 ), #17185, .T. ) ;
#10503=CARTESIAN_POINT ( 'NONE',  ( -23.07906255732286738, -9.958937815627702861, 66.72677557046061736 ) ) ;
#10504=CARTESIAN_POINT ( 'NONE',  ( -10.07803964209180414, -16.05037485348669435, 68.11734501381512530 ) ) ;
#10505=ORIENTED_EDGE ( 'NONE', *, *, #17341, .F. ) ;
#10507=DIRECTION ( 'NONE',  ( 1.411223637948141806E-06, 4.279116285847032870E-06, 0.9999999999898486758 ) ) ;
#10508=CARTESIAN_POINT ( 'NONE',  ( -10.39679176622870038, -14.24023819782134481, 64.40275955115841100 ) ) ;
#10510=CARTESIAN_POINT ( 'NONE',  ( -11.78703052381813166, -10.65887729864124189, 74.43884969850331856 ) ) ;
#10511=EDGE_LOOP ( 'NONE', ( #41011, #46638 ) ) ;
#10512=CARTESIAN_POINT ( 'NONE',  ( -10.76802635004704989, -17.14192985119425572, 57.57271792098855201 ) ) ;
#10513=CARTESIAN_POINT ( 'NONE',  ( -13.65248598864501339, -21.23405210337300630, 68.71271080785449215 ) ) ;
#10514=CARTESIAN_POINT ( 'NONE',  ( -19.37484620200115160, -7.619050568204919216, 60.14588398245204814 ) ) ;
#10516=CARTESIAN_POINT ( 'NONE',  ( -23.42604898704557925, -18.50800750300421171, 72.76928057529130456 ) ) ;
#10517=ORIENTED_EDGE ( 'NONE', *, *, #26898, .T. ) ;
#10519=CARTESIAN_POINT ( 'NONE',  ( -11.42264205816738176, -11.09470156419723708, 64.29315101522172426 ) ) ;
#10520=CARTESIAN_POINT ( 'NONE',  ( -24.34598896336966334, -16.14727844041069460, 62.89328645805750284 ) ) ;
#10521=ORIENTED_EDGE ( 'NONE', *, *, #35107, .F. ) ;
#10522=CARTESIAN_POINT ( 'NONE',  ( -9.979603264230430426, -14.52052340097724148, 68.04295441848455539 ) ) ;
#10525=ORIENTED_EDGE ( 'NONE', *, *, #34781, .T. ) ;
#10526=CARTESIAN_POINT ( 'NONE',  ( -15.03427660820159950, -21.44211488324610926, 65.12068745241758450 ) ) ;
#10528=DIRECTION ( 'NONE',  ( 0.3926557917762825145, -0.9196855055857631189, -5.808111619717074757E-09 ) ) ;
#10529=CARTESIAN_POINT ( 'NONE',  ( -20.63243265594276110, -8.084608023805090582, 63.42466202532494890 ) ) ;
#10530=CARTESIAN_POINT ( 'NONE',  ( -12.29927565234787679, -19.57981848576777040, 61.50751631702252098 ) ) ;
#10531=CARTESIAN_POINT ( 'NONE',  ( -13.14999064602648637, -9.265557826385967033, 67.37942786034257381 ) ) ;
#10532=FACE_OUTER_BOUND ( 'NONE', #26380, .T. ) ;
#10533=ORIENTED_EDGE ( 'NONE', *, *, #10646, .F. ) ;
#10534=ORIENTED_EDGE ( 'NONE', *, *, #2059, .F. ) ;
#10538=DIRECTION ( 'NONE',  ( 0.7847243476406478013, 0.6198448985189423110, -4.433022207822421914E-08 ) ) ;
#10540=CARTESIAN_POINT ( 'NONE',  ( -11.91343869374197695, -19.82283377674160718, 58.04186948019505365 ) ) ;
#10541=ORIENTED_EDGE ( 'NONE', *, *, #12174, .T. ) ;
#10546=CARTESIAN_POINT ( 'NONE',  ( -11.91343944425293522, -19.82283459374304968, 58.04187056893558605 ) ) ;
#10547=DIRECTION ( 'NONE',  ( -0.7248509490090242480, 0.6889057277456162032, -1.880377065355346998E-09 ) ) ;
#10549=ORIENTED_EDGE ( 'NONE', *, *, #21275, .T. ) ;
#10551=CARTESIAN_POINT ( 'NONE',  ( -14.60689809042303011, -8.346551666329650843, 64.08978840692947188 ) ) ;
#10553=VERTEX_POINT ( 'NONE', #18512 ) ;
#10555=CARTESIAN_POINT ( 'NONE',  ( -16.09245304043805191, -7.886071317471073705, 63.67011060592734140 ) ) ;
#10557=LINE ( 'NONE', #2441, #45653 ) ;
#10558=VERTEX_POINT ( 'NONE', #22225 ) ;
#10562=ADVANCED_FACE ( 'NONE', ( #15539 ), #8744, .T. ) ;
#10563=ORIENTED_EDGE ( 'NONE', *, *, #42418, .T. ) ;
#10564=DIRECTION ( 'NONE',  ( 0.003782665018460031406, 0.9999928456970870183, 9.532993539727310637E-09 ) ) ;
#10566=CARTESIAN_POINT ( 'NONE',  ( -20.31063677401542833, -8.430306179186672466, 70.44027317730545690 ) ) ;
#10567=ORIENTED_EDGE ( 'NONE', *, *, #41243, .F. ) ;
#10568=CARTESIAN_POINT ( 'NONE',  ( -10.89280197141400919, -11.22507430941316642, 64.33377434530349603 ) ) ;
#10569=EDGE_CURVE ( 'NONE', #43308, #22272, #18783, .T. ) ;
#10570=CARTESIAN_POINT ( 'NONE',  ( -19.67760665824181388, -21.48965406232008490, 65.75014118398131302 ) ) ;
#10571=CARTESIAN_POINT ( 'NONE',  ( -21.62445905946246327, -8.656051727655954764, 73.72411892793267896 ) ) ;
#10575=CARTESIAN_POINT ( 'NONE',  ( -12.02824346918037612, -10.34977652055329678, 67.79896853024506242 ) ) ;
#10576=CYLINDRICAL_SURFACE ( 'NONE', #43577, 0.1500000000000011879 ) ;
#10578=VERTEX_POINT ( 'NONE', #13719 ) ;
#10579=CARTESIAN_POINT ( 'NONE',  ( -22.48964968825576705, -9.905448439006629968, 73.76689030015370463 ) ) ;
#10580=CARTESIAN_POINT ( 'NONE',  ( -17.00708426123225436, -7.821638799215111071, 74.26018273346642218 ) ) ;
#10581=CARTESIAN_POINT ( 'NONE',  ( -11.01197672498281044, -17.74032467813711733, 71.85246142747087106 ) ) ;
#10583=CARTESIAN_POINT ( 'NONE',  ( -23.71751471349159601, -11.63122711669449316, 63.23746208799618529 ) ) ;
#10584=CARTESIAN_POINT ( 'NONE',  ( -14.11063322135152909, -21.03236308526469855, 72.21135587486895702 ) ) ;
#10585=CARTESIAN_POINT ( 'NONE',  ( -19.20962530548710845, -21.63318799521329083, 62.29503840543927851 ) ) ;
#10588=CARTESIAN_POINT ( 'NONE',  ( -11.75774095458083224, -19.00383931511212765, 71.68685884783835149 ) ) ;
#10589=CARTESIAN_POINT ( 'NONE',  ( -18.28991377027465504, -21.80587894173146424, 68.81514722156398989 ) ) ;
#10590=( BOUNDED_SURFACE ( )  B_SPLINE_SURFACE ( 3, 1, ( 
 ( #32435, #2141 ),
 ( #24325, #32196 ),
 ( #2388, #28502 ),
 ( #31944, #36106 ),
 ( #20632, #10275 ),
 ( #17635, #43527 ),
 ( #20864, #36351 ) ),
 .UNSPECIFIED., .T., .F., .F. ) 
 B_SPLINE_SURFACE_WITH_KNOTS ( ( 4, 3, 4 ),
 ( 2, 2 ),
 ( 0.000000000000000000, 0.5000000000000000000, 1.000000000000000000 ),
 ( 0.000000000000000000, 1.000000000000000000 ),
 .UNSPECIFIED. ) 
 GEOMETRIC_REPRESENTATION_ITEM ( )  RATIONAL_B_SPLINE_SURFACE ( (
 ( 1.000000000000000000, 1.000000000000000000),
 ( 0.3333333333333335369, 0.3333333333333330373),
 ( 0.3333333333333335369, 0.3333333333333330373),
 ( 1.000000000000000000, 1.000000000000000000),
 ( 0.3333333333333333703, 0.3333333333333333703),
 ( 0.3333333333333333703, 0.3333333333333333703),
 ( 1.000000000000000000, 1.000000000000000000) ) ) 
 REPRESENTATION_ITEM ( '' )  SURFACE ( )  );
#10592=EDGE_LOOP ( 'NONE', ( #12859, #16556, #3731, #30021, #2834 ) ) ;
#10594=ORIENTED_EDGE ( 'NONE', *, *, #9086, .T. ) ;
#10595=CARTESIAN_POINT ( 'NONE',  ( -20.58245214235086351, -8.562158453623027299, 59.91413264589528609 ) ) ;
#10597=FACE_OUTER_BOUND ( 'NONE', #38196, .T. ) ;
#10599=CARTESIAN_POINT ( 'NONE',  ( -24.30112618867181240, -13.25578303422174997, 59.64795780745660636 ) ) ;
#10601=EDGE_CURVE ( 'NONE', #36615, #14276, #23179, .T. ) ;
#10602=( BOUNDED_CURVE ( )  B_SPLINE_CURVE ( 3, ( #13899, #44708, #28942, #41237 ),
 .UNSPECIFIED., .F., .F. ) 
 B_SPLINE_CURVE_WITH_KNOTS ( ( 4, 4 ),
 ( 0.9074455897393655102, 1.000000000000000000 ),
 .UNSPECIFIED. ) 
 CURVE ( )  GEOMETRIC_REPRESENTATION_ITEM ( )  RATIONAL_B_SPLINE_CURVE ( ( 0.6983129098261073864, 0.7760317562607105257, 0.8765941196520080636, 1.000000000000000000 ) ) 
 REPRESENTATION_ITEM ( '' )  );
#10603=CARTESIAN_POINT ( 'NONE',  ( -24.46896812518309972, -12.38541668854236200, 73.40258933594091673 ) ) ;
#10604=CARTESIAN_POINT ( 'NONE',  ( -10.89280251029460622, -11.22507333849785027, 64.33377325762776877 ) ) ;
#10605=EDGE_LOOP ( 'NONE', ( #46832, #40959 ) ) ;
#10606=CARTESIAN_POINT ( 'NONE',  ( -10.12326195556307695, -13.32541703369907893, 74.86313051124790263 ) ) ;
#10607=CARTESIAN_POINT ( 'NONE',  ( -24.47999924015074669, -14.97998867148549351, 62.85729180369179403 ) ) ;
#10608=CARTESIAN_POINT ( 'NONE',  ( -12.27604185553471616, -19.62628656662749549, 58.21210303282668264 ) ) ;
#10609=ORIENTED_EDGE ( 'NONE', *, *, #23132, .F. ) ;
#10610=CARTESIAN_POINT ( 'NONE',  ( -24.11793993921729395, -12.76166543249827434, 70.07243002473258286 ) ) ;
#10612=FACE_OUTER_BOUND ( 'NONE', #43722, .T. ) ;
#10613=EDGE_CURVE ( 'NONE', #3341, #47047, #2063, .T. ) ;
#10614=DIRECTION ( 'NONE',  ( -5.854827030937197869E-31, -1.020425574103664912E-16, -1.000000000000000000 ) ) ;
#10616=CARTESIAN_POINT ( 'NONE',  ( -24.14992822999210276, -18.01341164000503525, 59.11882993461590274 ) ) ;
#10617=CARTESIAN_POINT ( 'NONE',  ( -20.05203603265719892, -8.267149239628885482, 73.72656352965896076 ) ) ;
#10618=DIRECTION ( 'NONE',  ( -1.487365705136564946E-06, 6.376425429333053644E-07, 0.9999999999986904919 ) ) ;
#10619=EDGE_CURVE ( 'NONE', #32198, #29810, #34592, .T. ) ;
#10620=CARTESIAN_POINT ( 'NONE',  ( -23.44980356754079054, -18.46889531339634871, 72.91368236442116313 ) ) ;
#10623=CARTESIAN_POINT ( 'NONE',  ( -10.47299162366406478, -15.63514707757639854, 61.33789045486464886 ) ) ;
#10625=ORIENTED_EDGE ( 'NONE', *, *, #22164, .T. ) ;
#10626=CARTESIAN_POINT ( 'NONE',  ( -12.17457826531766329, -10.10312750218776046, 64.03474096465798482 ) ) ;
#10627=CARTESIAN_POINT ( 'NONE',  ( -9.990623107247818879, -14.31192343302863179, 64.57299167182827659 ) ) ;
#10631=CARTESIAN_POINT ( 'NONE',  ( -16.02453559203015132, -22.12732798260191913, 58.47240968810538675 ) ) ;
#10635=ORIENTED_EDGE ( 'NONE', *, *, #27015, .T. ) ;
#10636=CARTESIAN_POINT ( 'NONE',  ( -24.49635653881819408, -12.46679777644911447, 73.35730153580948354 ) ) ;
#10637=CARTESIAN_POINT ( 'NONE',  ( -9.975182982828622258, -14.68140347846369131, 71.52793889455062981 ) ) ;
#10638=EDGE_LOOP ( 'NONE', ( #11210, #2864, #34456, #43625, #3175 ) ) ;
#10641=CARTESIAN_POINT ( 'NONE',  ( -21.79028809537168243, -9.273590339475653366, 63.47681654923867711 ) ) ;
#10642=CARTESIAN_POINT ( 'NONE',  ( -12.22456126456390280, -19.57467567670336450, 61.81167242413056329 ) ) ;
#10643=ADVANCED_FACE ( 'NONE', ( #35889 ), #4696, .T. ) ;
#10644=FACE_BOUND ( 'NONE', #46006, .T. ) ;
#10645=CARTESIAN_POINT ( 'NONE',  ( -12.13854904415787850, -9.558901172912655397, 57.18961277425697176 ) ) ;
#10646=EDGE_CURVE ( 'NONE', #8033, #25935, #13157, .T. ) ;
#10647=DIRECTION ( 'NONE',  ( -1.424565728495322281E-06, 1.060674514755067221E-05, -0.9999999999427338082 ) ) ;
#10648=CARTESIAN_POINT ( 'NONE',  ( -16.63927444439371683, -21.76668879618412333, 68.88487749788691872 ) ) ;
#10649=EDGE_CURVE ( 'NONE', #13987, #46068, #36136, .T. ) ;
#10650=EDGE_CURVE ( 'NONE', #30363, #24642, #14941, .T. ) ;
#10651=EDGE_CURVE ( 'NONE', #24418, #12172, #48124, .T. ) ;
#10652=EDGE_LOOP ( 'NONE', ( #21874, #7118 ) ) ;
#10654=CARTESIAN_POINT ( 'NONE',  ( -10.59656512619885227, -13.05092609425065220, 68.02360230423869325 ) ) ;
#10656=CARTESIAN_POINT ( 'NONE',  ( -13.65248598864501339, -21.23405210337300630, 68.71271080785449215 ) ) ;
#10658=VERTEX_POINT ( 'NONE', #17665 ) ;
#10661=ORIENTED_EDGE ( 'NONE', *, *, #23329, .F. ) ;
#10662=CARTESIAN_POINT ( 'NONE',  ( -17.38353765754063929, -7.359306650671737060, 67.12015974172000199 ) ) ;
#10663=CARTESIAN_POINT ( 'NONE',  ( -18.97054410961560578, -7.521390078327941708, 67.08567059339527816 ) ) ;
#10665=CARTESIAN_POINT ( 'NONE',  ( -24.61980809523442559, -12.87874405397987232, 66.46393279139718402 ) ) ;
#10666=ADVANCED_FACE ( 'NONE', ( #10771 ), #40807, .T. ) ;
#10667=CARTESIAN_POINT ( 'NONE',  ( -16.26195973558533936, -21.76306465430365122, 58.57113428431811997 ) ) ;
#10669=CARTESIAN_POINT ( 'NONE',  ( -13.53325528467554406, -21.16256411608339150, 65.17124155742401115 ) ) ;
#10670=DIRECTION ( 'NONE',  ( -5.625773302382611900E-06, -7.100530147430143890E-06, -0.9999999999589666011 ) ) ;
#10671=ORIENTED_EDGE ( 'NONE', *, *, #42354, .T. ) ;
#10672=CARTESIAN_POINT ( 'NONE',  ( -11.48484495912356707, -11.01053355528029165, 57.21463035491839122 ) ) ;
#10673=CARTESIAN_POINT ( 'NONE',  ( -12.32278866559117780, -19.67576434477648917, 61.41150688479135766 ) ) ;
#10674=ORIENTED_EDGE ( 'NONE', *, *, #14060, .T. ) ;
#10675=CARTESIAN_POINT ( 'NONE',  ( -19.57546054543010783, -21.94189796748987575, 62.03857704761023939 ) ) ;
#10678=CARTESIAN_POINT ( 'NONE',  ( -14.05371499411349845, -21.00138273984457982, 72.22607703579409133 ) ) ;
#10679=CARTESIAN_POINT ( 'NONE',  ( -24.42668993457695592, -13.99045928592870958, 73.40799407547365263 ) ) ;
#10680=( BOUNDED_SURFACE ( )  B_SPLINE_SURFACE ( 3, 1, ( 
 ( #35701, #31547 ),
 ( #13054, #9642 ),
 ( #16747, #46581 ),
 ( #12827, #13774 ),
 ( #9388, #1502 ),
 ( #27847, #39658 ),
 ( #28085, #35949 ) ),
 .UNSPECIFIED., .T., .F., .F. ) 
 B_SPLINE_SURFACE_WITH_KNOTS ( ( 4, 3, 4 ),
 ( 2, 2 ),
 ( 0.000000000000000000, 0.5000000000000000000, 1.000000000000000000 ),
 ( 0.000000000000000000, 1.000000000000000000 ),
 .UNSPECIFIED. ) 
 GEOMETRIC_REPRESENTATION_ITEM ( )  RATIONAL_B_SPLINE_SURFACE ( (
 ( 1.000000000000000000, 1.000000000000000000),
 ( 0.3333333333333335369, 0.3333333333333330373),
 ( 0.3333333333333335369, 0.3333333333333330373),
 ( 1.000000000000000000, 1.000000000000000000),
 ( 0.3333333333333333703, 0.3333333333333333703),
 ( 0.3333333333333333703, 0.3333333333333333703),
 ( 1.000000000000000000, 1.000000000000000000) ) ) 
 REPRESENTATION_ITEM ( '' )  SURFACE ( )  );
#10682=DIRECTION ( 'NONE',  ( -1.190035116827072985E-06, -1.172070119237067893E-06, -0.9999999999986051158 ) ) ;
#10685=FACE_OUTER_BOUND ( 'NONE', #37962, .T. ) ;
#10686=CARTESIAN_POINT ( 'NONE',  ( -23.70015231925135168, -18.82353928378165975, 69.47867257277708575 ) ) ;
#10687=CARTESIAN_POINT ( 'NONE',  ( -10.77549359890341485, -17.15424032507071317, 61.45743111002949632 ) ) ;
#10688=ORIENTED_EDGE ( 'NONE', *, *, #1837, .F. ) ;
#10690=CARTESIAN_POINT ( 'NONE',  ( -21.41863048803932656, -8.999699081277377388, 73.61600897546567523 ) ) ;
#10691=ORIENTED_EDGE ( 'NONE', *, *, #26112, .T. ) ;
#10694=LINE ( 'NONE', #25474, #6245 ) ;
#10695=VERTEX_POINT ( 'NONE', #2658 ) ;
#10698=VERTEX_POINT ( 'NONE', #48196 ) ;
#10700=ADVANCED_FACE ( 'NONE', ( #32690 ), #21620, .T. ) ;
#10701=ORIENTED_EDGE ( 'NONE', *, *, #38960, .T. ) ;
#10705=LINE ( 'NONE', #25722, #28313 ) ;
#10706=CARTESIAN_POINT ( 'NONE',  ( -13.26948432366006969, -9.109728530933422164, 60.32461385657482822 ) ) ;
#10710=ADVANCED_FACE ( 'NONE', ( #47714 ), #10301, .T. ) ;
#10715=ORIENTED_EDGE ( 'NONE', *, *, #36823, .F. ) ;
#10717=CARTESIAN_POINT ( 'NONE',  ( -24.37613966482678762, -15.62716692544170094, 69.64193411296469094 ) ) ;
#10718=CARTESIAN_POINT ( 'NONE',  ( -24.40836459905232303, -14.33371432994024808, 69.93658700684441953 ) ) ;
#10719=( BOUNDED_CURVE ( )  B_SPLINE_CURVE ( 3, ( #18249, #13822, #32558, #28863 ),
 .UNSPECIFIED., .F., .F. ) 
 B_SPLINE_CURVE_WITH_KNOTS ( ( 4, 4 ),
 ( 0.000000000000000000, 0.4074455897393639559 ),
 .UNSPECIFIED. ) 
 CURVE ( )  GEOMETRIC_REPRESENTATION_ITEM ( )  RATIONAL_B_SPLINE_CURVE ( ( 1.000000000000000000, 0.4567392136813391845, 0.3561768502900329869, 0.6983129098260814072 ) ) 
 REPRESENTATION_ITEM ( '' )  );
#10720=ORIENTED_EDGE ( 'NONE', *, *, #18036, .T. ) ;
#10724=CARTESIAN_POINT ( 'NONE',  ( -22.49805058420730219, -9.986866540729424813, 73.78161091687563555 ) ) ;
#10725=CARTESIAN_POINT ( 'NONE',  ( -20.35208330028754631, -8.450993137587310855, 66.78104082230152017 ) ) ;
#10727=CARTESIAN_POINT ( 'NONE',  ( -12.84615363328625648, -20.17103110633857455, 72.09181604382622766 ) ) ;
#10728=ORIENTED_EDGE ( 'NONE', *, *, #24352, .F. ) ;
#10729=CARTESIAN_POINT ( 'NONE',  ( -19.05654430117847653, -8.000564469898289843, 67.08998960197388328 ) ) ;
#10730=CARTESIAN_POINT ( 'NONE',  ( -15.39389095703113952, -21.97733419268598709, 72.23070866474378704 ) ) ;
#10731=CARTESIAN_POINT ( 'NONE',  ( -19.38312129636155134, -7.621338365550096583, 60.06754680096511834 ) ) ;
#10732=FACE_OUTER_BOUND ( 'NONE', #23094, .T. ) ;
#10735=CARTESIAN_POINT ( 'NONE',  ( -10.70566866894273161, -16.94585410378973478, 57.98760548748136756 ) ) ;
#10736=( BOUNDED_CURVE ( )  B_SPLINE_CURVE ( 3, ( #46003, #11297, #23349, #8104 ),
 .UNSPECIFIED., .F., .F. ) 
 B_SPLINE_CURVE_WITH_KNOTS ( ( 4, 4 ),
 ( 0.5000000000000000000, 0.9074455897393667314 ),
 .UNSPECIFIED. ) 
 CURVE ( )  GEOMETRIC_REPRESENTATION_ITEM ( )  RATIONAL_B_SPLINE_CURVE ( ( 1.000000000000009548, 0.4567392136813334669, 0.3561768502900239941, 0.6983129098260916212 ) ) 
 REPRESENTATION_ITEM ( '' )  );
#10737=CARTESIAN_POINT ( 'NONE',  ( -21.68499601416157674, -9.192516039336663169, 66.66149992327366647 ) ) ;
#10739=FACE_BOUND ( 'NONE', #9386, .T. ) ;
#10741=CARTESIAN_POINT ( 'NONE',  ( -10.31413044408767554, -17.03453498993188475, 57.94406477676061229 ) ) ;
#10742=CARTESIAN_POINT ( 'NONE',  ( -13.70953082315746130, -10.73489715249941057, 53.69233794759168887 ) ) ;
#10744=CARTESIAN_POINT ( 'NONE',  ( -21.64297170217681554, -9.150934564753532285, 73.74561934610416358 ) ) ;
#10745=ORIENTED_EDGE ( 'NONE', *, *, #11726, .T. ) ;
#10746=CARTESIAN_POINT ( 'NONE',  ( -10.47191904619592684, -13.98145195064897095, 61.14651201797807545 ) ) ;
#10747=VERTEX_POINT ( 'NONE', #17894 ) ;
#10748=CARTESIAN_POINT ( 'NONE',  ( -11.22844613476422460, -11.44458948612160043, 64.43409918096024569 ) ) ;
#10749=CARTESIAN_POINT ( 'NONE',  ( -23.37507359076485969, -18.49521754853151734, 69.36659925232392254 ) ) ;
#10750=VERTEX_POINT ( 'NONE', #32920 ) ;
#10751=CARTESIAN_POINT ( 'NONE',  ( -10.17289295492252599, -13.09960488110308319, 71.30804949251027836 ) ) ;
#10753=DIRECTION ( 'NONE',  ( 3.549360974554993999E-17, -6.371834667797928663E-18, -1.000000000000000000 ) ) ;
#10754=ADVANCED_FACE ( 'NONE', ( #22343 ), #48686, .T. ) ;
#10755=ORIENTED_EDGE ( 'NONE', *, *, #42325, .T. ) ;
#10756=ORIENTED_EDGE ( 'NONE', *, *, #42091, .F. ) ;
#10758=CARTESIAN_POINT ( 'NONE',  ( -23.22228500509449134, -18.82597476736437869, 69.38552271346109990 ) ) ;
#10759=CARTESIAN_POINT ( 'NONE',  ( -23.80338573481879294, -11.80731802715296297, 59.76763678108634537 ) ) ;
#10760=CARTESIAN_POINT ( 'NONE',  ( -20.75775239920833215, -8.146595409969087598, 63.56767435313065562 ) ) ;
#10761=CARTESIAN_POINT ( 'NONE',  ( -12.34924369011040923, -19.63124204235170112, 61.41295224250168872 ) ) ;
#10762=CARTESIAN_POINT ( 'NONE',  ( -20.06838235508133650, -8.265300555148282768, 66.93671294127740623 ) ) ;
#10763=AXIS2_PLACEMENT_3D ( 'NONE', #8143, #26114, #29809 ) ;
#10765=VERTEX_POINT ( 'NONE', #41297 ) ;
#10766=ORIENTED_EDGE ( 'NONE', *, *, #40833, .F. ) ;
#10767=EDGE_CURVE ( 'NONE', #26011, #37558, #22980, .T. ) ;
#10768=FACE_OUTER_BOUND ( 'NONE', #41206, .T. ) ;
#10770=CARTESIAN_POINT ( 'NONE',  ( -19.86506860716628253, -8.248529813971950730, 73.79384751630072969 ) ) ;
#10771=FACE_OUTER_BOUND ( 'NONE', #14285, .T. ) ;
#10772=CARTESIAN_POINT ( 'NONE',  ( -11.03124136535102373, -17.66077402989073875, 71.56718193465405875 ) ) ;
#10773=AXIS2_PLACEMENT_3D ( 'NONE', #40545, #41049, #2875 ) ;
#10775=EDGE_CURVE ( 'NONE', #28733, #48574, #28497, .T. ) ;
#10778=EDGE_LOOP ( 'NONE', ( #10325, #20329, #47416, #33601, #25376 ) ) ;
#10779=CARTESIAN_POINT ( 'NONE',  ( -21.94683311842353746, -20.15404798103656958, 62.42366210617201006 ) ) ;
#10780=ADVANCED_FACE ( 'NONE', ( #34382 ), #19137, .T. ) ;
#10782=CARTESIAN_POINT ( 'NONE',  ( -13.17078218117215549, -9.186392337449538203, 67.39414915108072535 ) ) ;
#10784=CARTESIAN_POINT ( 'NONE',  ( -10.48067290732983281, -16.03043740265091444, 67.97767830707738312 ) ) ;
#10785=CARTESIAN_POINT ( 'NONE',  ( -14.73514675383382055, -8.346202503743331391, 60.60530971328631722 ) ) ;
#10786=ORIENTED_EDGE ( 'NONE', *, *, #17968, .F. ) ;
#10787=CARTESIAN_POINT ( 'NONE',  ( -15.15105612103415034, -21.43000825703723322, 65.10596678909395507 ) ) ;
#10788=B_SPLINE_CURVE_WITH_KNOTS ( 'NONE', 3,
 ( #12209, #42013, #24034, #38289, #24272, #27950, #27712, #42979, #16120, #27230 ),
 .UNSPECIFIED., .F., .F.,
 ( 4, 2, 2, 2, 4 ),
 ( 0.000000000000000000, 0.2500000000000000000, 0.5000000000000000000, 0.7500000000000000000, 1.000000000000000000 ),
 .UNSPECIFIED. ) ;
#10789=CARTESIAN_POINT ( 'NONE',  ( -10.49796979654650642, -16.16706115165171198, 64.66338504953419886 ) ) ;
#10790=ORIENTED_EDGE ( 'NONE', *, *, #23986, .T. ) ;
#10791=CARTESIAN_POINT ( 'NONE',  ( -11.18189875852979043, -11.63857375077518519, 71.16031116833757153 ) ) ;
#10793=VECTOR ( 'NONE', #20372, 1000.000000000000000 ) ;
#10795=DIRECTION ( 'NONE',  ( 0.2771212459065066636, -0.9608349572466771127, -4.100231986695786665E-08 ) ) ;
#10796=CARTESIAN_POINT ( 'NONE',  ( -24.87322977116181022, -14.68525938325893065, 62.87442968679287958 ) ) ;
#10798=CARTESIAN_POINT ( 'NONE',  ( -12.79154865046270473, -8.973695691655201756, 67.49287406301634462 ) ) ;
#10799=CARTESIAN_POINT ( 'NONE',  ( -11.45924070651598470, -10.34566349473087854, 74.53910820911023905 ) ) ;
#10801=CYLINDRICAL_SURFACE ( 'NONE', #33083, 0.1500000000000081268 ) ;
#10802=AXIS2_PLACEMENT_3D ( 'NONE', #12072, #46047, #12303 ) ;
#10804=CARTESIAN_POINT ( 'NONE',  ( -11.07113446568633108, -18.70063274991032998, 61.38436695725324199 ) ) ;
#10805=CARTESIAN_POINT ( 'NONE',  ( -23.59327504554355315, -11.39630409041826198, 69.90682860766239060 ) ) ;
#10806=ORIENTED_EDGE ( 'NONE', *, *, #33872, .F. ) ;
#10807=CARTESIAN_POINT ( 'NONE',  ( -19.89714791213391365, -21.83689362560225788, 69.05765572360830618 ) ) ;
#10808=B_SPLINE_CURVE_WITH_KNOTS ( 'NONE', 3,
 ( #27856, #36201, #35712, #16990, #42886, #32519, #39666, #28821, #9650, #9396 ),
 .UNSPECIFIED., .F., .F.,
 ( 4, 2, 2, 2, 4 ),
 ( 0.000000000000000000, 0.2500000000000000000, 0.5000000000000000000, 0.7500000000000000000, 1.000000000000000000 ),
 .UNSPECIFIED. ) ;
#10809=CARTESIAN_POINT ( 'NONE',  ( -11.71918404020638427, -18.95175453447548009, 71.70158022526054253 ) ) ;
#10810=EDGE_CURVE ( 'NONE', #21395, #27235, #38416, .T. ) ;
#10811=ORIENTED_EDGE ( 'NONE', *, *, #45081, .F. ) ;
#10813=CARTESIAN_POINT ( 'NONE',  ( -22.75144419618436586, -9.600271701911582412, 73.59505825258622735 ) ) ;
#10814=CARTESIAN_POINT ( 'NONE',  ( -22.96481576609224717, -19.16891988936071556, 58.89882756593014790 ) ) ;
#10815=FACE_OUTER_BOUND ( 'NONE', #24904, .T. ) ;
#10817=CARTESIAN_POINT ( 'NONE',  ( -24.50530043060364349, -7.885727737951715888, 53.49999999999995026 ) ) ;
#10818=CARTESIAN_POINT ( 'NONE',  ( -16.92358529718788063, -21.79135155313683114, 68.92233962256314328 ) ) ;
#10819=CARTESIAN_POINT ( 'NONE',  ( -24.34502386579654498, -17.56683345968398768, 66.12852568699506151 ) ) ;
#10820=CARTESIAN_POINT ( 'NONE',  ( -16.55143150278462016, -22.20792881918157491, 65.42553161510207360 ) ) ;
#10821=ORIENTED_EDGE ( 'NONE', *, *, #25838, .T. ) ;
#10824=ADVANCED_FACE ( 'NONE', ( #34144 ), #45974, .T. ) ;
#10827=ADVANCED_FACE ( 'NONE', ( #11504 ), #8800, .T. ) ;
#10828=B_SPLINE_CURVE_WITH_KNOTS ( 'NONE', 3,
 ( #38278, #1112, #16111, #38785, #8276, #31152, #5067, #46181, #1344, #23056 ),
 .UNSPECIFIED., .F., .F.,
 ( 4, 2, 2, 2, 4 ),
 ( 0.6272669072782223187, 0.7522669073001169160, 0.8772669073220116243, 1.002266907343906333, 1.127266907365800819 ),
 .UNSPECIFIED. ) ;
#10830=ORIENTED_EDGE ( 'NONE', *, *, #10210, .F. ) ;
#10831=AXIS2_PLACEMENT_3D ( 'NONE', #43583, #10564, #32256 ) ;
#10832=ADVANCED_FACE ( 'NONE', ( #15670 ), #33910, .T. ) ;
#10837=ADVANCED_FACE ( 'NONE', ( #12233 ), #12468, .T. ) ;
#10838=ORIENTED_EDGE ( 'NONE', *, *, #9026, .T. ) ;
#10840=CARTESIAN_POINT ( 'NONE',  ( -24.48100519043057233, -12.42118325661428457, 73.34201943126451795 ) ) ;
#10843=CARTESIAN_POINT ( 'NONE',  ( -24.25486363958986757, -13.06355980472538469, 63.11792038370487035 ) ) ;
#10845=CARTESIAN_POINT ( 'NONE',  ( -24.76540239943457422, -16.07765717072269140, 66.17829646510101327 ) ) ;
#10847=CARTESIAN_POINT ( 'NONE',  ( -24.16181628213775312, -12.90510636975119674, 69.88316126822323326 ) ) ;
#10849=DIRECTION ( 'NONE',  ( 6.919810409924334203E-06, 1.067025349499717229E-05, -0.9999999999191309108 ) ) ;
#10850=CARTESIAN_POINT ( 'NONE',  ( -21.18000425931230168, -20.77541442555289919, 69.20450184740300870 ) ) ;
#10851=ORIENTED_EDGE ( 'NONE', *, *, #19794, .F. ) ;
#10852=CARTESIAN_POINT ( 'NONE',  ( -16.23831082583558327, -7.859603177651183437, 60.50028451141000119 ) ) ;
#10853=CARTESIAN_POINT ( 'NONE',  ( -20.00946503018472811, -8.250368534377352958, 73.72096600125085786 ) ) ;
#10857=VECTOR ( 'NONE', #3802, 1000.000000000000000 ) ;
#10858=EDGE_CURVE ( 'NONE', #11228, #19229, #8528, .T. ) ;
#10859=CARTESIAN_POINT ( 'NONE',  ( -23.91010245674826251, -17.57297063409389537, 62.75888927877479517 ) ) ;
#10860=CYLINDRICAL_SURFACE ( 'NONE', #35521, 0.1500000000000042966 ) ;
#10861=CARTESIAN_POINT ( 'NONE',  ( -15.68503146357154776, -7.977064754671971514, 70.75989839959960648 ) ) ;
#10863=CARTESIAN_POINT ( 'NONE',  ( -12.23301264461619553, -10.03852782535897958, 60.84446034103241630 ) ) ;
#10864=AXIS2_PLACEMENT_3D ( 'NONE', #39213, #36465, #47575 ) ;
#10865=VECTOR ( 'NONE', #19594, 1000.000000000000114 ) ;
#10866=CARTESIAN_POINT ( 'NONE',  ( -9.985622318910028383, -14.38165043598653980, 64.50148546807987771 ) ) ;
#10867=CARTESIAN_POINT ( 'NONE',  ( -22.95648371662476350, -9.819685991319531126, 70.11154895885017879 ) ) ;
#10868=DIRECTION ( 'NONE',  ( 8.226841968992228303E-06, -2.386003345919280055E-06, -0.9999999999633130132 ) ) ;
#10869=CARTESIAN_POINT ( 'NONE',  ( -10.81476112650719479, -12.49952415756758661, 60.87023803673543654 ) ) ;
#10870=CARTESIAN_POINT ( 'NONE',  ( -22.80551657591753312, -9.657165430906786696, 73.58822797253898784 ) ) ;
#10871=ORIENTED_EDGE ( 'NONE', *, *, #6521, .F. ) ;
#10873=CARTESIAN_POINT ( 'NONE',  ( -11.53435529947139315, -18.68938829637487942, 61.16221976381599745 ) ) ;
#10874=CARTESIAN_POINT ( 'NONE',  ( -17.85728874018076340, -21.84618329174708151, 61.89007996730683203 ) ) ;
#10875=ORIENTED_EDGE ( 'NONE', *, *, #25648, .F. ) ;
#10876=CARTESIAN_POINT ( 'NONE',  ( -15.34293294794334628, -7.655665426595480660, 74.25702532252046240 ) ) ;
#10878=CARTESIAN_POINT ( 'NONE',  ( -17.42409385541300892, -14.80920654474439679, 47.99999999999994316 ) ) ;
#10880=CARTESIAN_POINT ( 'NONE',  ( -20.68825345639836044, -8.112218880830354806, 63.48838406824151548 ) ) ;
#10881=CARTESIAN_POINT ( 'NONE',  ( -22.27817835350360909, -9.157512823226451104, 59.83675901011532261 ) ) ;
#10882=( BOUNDED_CURVE ( )  B_SPLINE_CURVE ( 3, ( #13632, #10211, #13143, #5555 ),
 .UNSPECIFIED., .F., .F. ) 
 B_SPLINE_CURVE_WITH_KNOTS ( ( 4, 4 ),
 ( 0.5000000000000000000, 0.9074455897393624015 ),
 .UNSPECIFIED. ) 
 CURVE ( )  GEOMETRIC_REPRESENTATION_ITEM ( )  RATIONAL_B_SPLINE_CURVE ( ( 0.9999999999999924505, 0.4567392136813328563, 0.3561768502900357625, 0.6983129098260931755 ) ) 
 REPRESENTATION_ITEM ( '' )  );
#10883=CARTESIAN_POINT ( 'NONE',  ( -11.32469277870022850, -18.34471304272907588, 58.10714594244494435 ) ) ;
#10884=CARTESIAN_POINT ( 'NONE',  ( -24.83280391540558796, -14.02581302221999593, 73.22297261464329665 ) ) ;
#10885=FACE_OUTER_BOUND ( 'NONE', #27296, .T. ) ;
#10887=ORIENTED_EDGE ( 'NONE', *, *, #12933, .T. ) ;
#10888=DIRECTION ( 'NONE',  ( 0.5652317888644005084, 0.8249321334856241084, -7.911723905263142424E-08 ) ) ;
#10889=CARTESIAN_POINT ( 'NONE',  ( -10.23610939720467528, -12.85046776639672039, 67.85337053980535416 ) ) ;
#10890=EDGE_CURVE ( 'NONE', #26171, #15132, #41800, .T. ) ;
#10891=CARTESIAN_POINT ( 'NONE',  ( -15.03781870946894905, -19.77948485407324242, 53.88362224778186516 ) ) ;
#10893=CARTESIAN_POINT ( 'NONE',  ( -10.71854902139521926, -11.56295204017805567, 71.23860870132143930 ) ) ;
#10894=CARTESIAN_POINT ( 'NONE',  ( -13.59065431704403615, -21.19813492939682220, 68.64280514999626348 ) ) ;
#10895=B_SPLINE_CURVE_WITH_KNOTS ( 'NONE', 3,
 ( #17132, #32188, #21818, #32427, #40056, #21101, #21587, #2622, #28726, #25037 ),
 .UNSPECIFIED., .F., .F.,
 ( 4, 2, 2, 2, 4 ),
 ( 0.000000000000000000, 0.2500000000000000000, 0.5000000000000000000, 0.7500000000000000000, 1.000000000000000000 ),
 .UNSPECIFIED. ) ;
#10896=CARTESIAN_POINT ( 'NONE',  ( -23.75068382698706770, -10.87373689121910658, 73.47537926597675551 ) ) ;
#10897=( BOUNDED_SURFACE ( )  B_SPLINE_SURFACE ( 3, 1, ( 
 ( #24580, #12977 ),
 ( #8581, #4635 ),
 ( #1416, #24084 ),
 ( #28259, #5130 ),
 ( #42312, #23604 ),
 ( #35630, #9309 ),
 ( #35393, #4892 ) ),
 .UNSPECIFIED., .T., .F., .F. ) 
 B_SPLINE_SURFACE_WITH_KNOTS ( ( 4, 3, 4 ),
 ( 2, 2 ),
 ( 0.000000000000000000, 0.5000000000000000000, 1.000000000000000000 ),
 ( 0.000000000000000000, 1.000000000000000000 ),
 .UNSPECIFIED. ) 
 GEOMETRIC_REPRESENTATION_ITEM ( )  RATIONAL_B_SPLINE_SURFACE ( (
 ( 1.000000000000000000, 1.000000000000000000),
 ( 0.3333333333333335369, 0.3333333333333330373),
 ( 0.3333333333333335369, 0.3333333333333330373),
 ( 1.000000000000000000, 1.000000000000000000),
 ( 0.3333333333333333703, 0.3333333333333333703),
 ( 0.3333333333333333703, 0.3333333333333333703),
 ( 1.000000000000000000, 1.000000000000000000) ) ) 
 REPRESENTATION_ITEM ( '' )  SURFACE ( )  );
#10902=VERTEX_POINT ( 'NONE', #30723 ) ;
#10903=CARTESIAN_POINT ( 'NONE',  ( -16.28536801364495545, -7.851737743193615948, 60.20028506676293034 ) ) ;
#10909=AXIS2_PLACEMENT_3D ( 'NONE', #23483, #8223, #23008 ) ;
#10910=LINE ( 'NONE', #25446, #47337 ) ;
#10911=DIRECTION ( 'NONE',  ( 0.8244078399817417191, 0.5659962132175737626, 7.627400655798535667E-08 ) ) ;
#10912=VERTEX_POINT ( 'NONE', #23320 ) ;
#10913=CARTESIAN_POINT ( 'NONE',  ( -24.36490009086193353, -15.72991820881333069, 73.11376895235396489 ) ) ;
#10914=CARTESIAN_POINT ( 'NONE',  ( -21.06494968540953749, -21.30903997076690359, 62.15825466738357363 ) ) ;
#10915=ORIENTED_EDGE ( 'NONE', *, *, #15031, .T. ) ;
#10916=CARTESIAN_POINT ( 'NONE',  ( -10.37382936219775154, -14.83089353207902228, 74.81251018390588570 ) ) ;
#10917=EDGE_CURVE ( 'NONE', #31867, #7245, #4604, .T. ) ;
#10919=ADVANCED_FACE ( 'NONE', ( #27735 ), #5096, .T. ) ;
#10921=CARTESIAN_POINT ( 'NONE',  ( -19.49109506855409180, -21.54969648977046148, 62.28031529404344013 ) ) ;
#10922=CARTESIAN_POINT ( 'NONE',  ( -27.43465133269545930, -13.44290337829342796, 54.49999999999995026 ) ) ;
#10923=CARTESIAN_POINT ( 'NONE',  ( -12.94070927391775427, -9.363776855876855265, 67.58762549400667297 ) ) ;
#10924=EDGE_CURVE ( 'NONE', #20147, #3341, #46700, .T. ) ;
#10925=EDGE_LOOP ( 'NONE', ( #16243, #5207 ) ) ;
#10926=CARTESIAN_POINT ( 'NONE',  ( -11.97152748846423265, -19.88606886789912664, 58.08715752149842615 ) ) ;
#10929=CARTESIAN_POINT ( 'NONE',  ( -10.98611580423108336, -17.68970554115635352, 67.98233349607527032 ) ) ;
#10930=ORIENTED_EDGE ( 'NONE', *, *, #17229, .F. ) ;
#10934=CARTESIAN_POINT ( 'NONE',  ( -17.95973986510568920, -21.78880545038086680, 62.17535914954028442 ) ) ;
#10936=EDGE_LOOP ( 'NONE', ( #30584, #21715, #25413, #6791, #45309 ) ) ;
#10938=CARTESIAN_POINT ( 'NONE',  ( -17.75494382041872399, -22.25186532844304921, 58.60542163939332738 ) ) ;
#10940=ORIENTED_EDGE ( 'NONE', *, *, #20553, .T. ) ;
#10941=CARTESIAN_POINT ( 'NONE',  ( -22.33376602745314798, -19.86903051493498040, 69.18890041286789483 ) ) ;
#10944=CYLINDRICAL_SURFACE ( 'NONE', #14757, 0.1499999999999990508 ) ;
#10946=CARTESIAN_POINT ( 'NONE',  ( -23.65624057141237202, -11.51332318074561911, 66.72214514605295221 ) ) ;
#10949=CARTESIAN_POINT ( 'NONE',  ( -18.37632025677473990, -22.19811156716688672, 68.91491069639255329 ) ) ;
#10954=CARTESIAN_POINT ( 'NONE',  ( -18.76558283008973049, -7.480892646508040755, 70.55563411965815135 ) ) ;
#10956=DIRECTION ( 'NONE',  ( 0.2122660683108583690, -0.9772119095896469876, 7.504255179194988334E-08 ) ) ;
#10957=CARTESIAN_POINT ( 'NONE',  ( -12.84913006811349945, -9.445038364547627907, 74.32482815461490588 ) ) ;
#10958=ORIENTED_EDGE ( 'NONE', *, *, #4285, .T. ) ;
#10961=EDGE_CURVE ( 'NONE', #18657, #28606, #24781, .T. ) ;
#10965=ORIENTED_EDGE ( 'NONE', *, *, #32047, .F. ) ;
#10966=CARTESIAN_POINT ( 'NONE',  ( -10.00731240618708462, -14.10555136595099945, 61.10316694600977172 ) ) ;
#10968=CARTESIAN_POINT ( 'NONE',  ( -18.28630064832924162, -21.80992411731310909, 72.37691179419678633 ) ) ;
#10970=ORIENTED_EDGE ( 'NONE', *, *, #41608, .T. ) ;
#10971=CARTESIAN_POINT ( 'NONE',  ( -11.19706266256277694, -11.50303319689152737, 67.63336710488009373 ) ) ;
#10972=AXIS2_PLACEMENT_3D ( 'NONE', #19919, #1686, #1924 ) ;
#10976=CARTESIAN_POINT ( 'NONE',  ( -19.56314583254387074, -21.47448964078003186, 65.76486235662434865 ) ) ;
#10979=EDGE_CURVE ( 'NONE', #16043, #26071, #41503, .T. ) ;
#10980=CARTESIAN_POINT ( 'NONE',  ( -9.990623027812100432, -14.31192454061599229, 64.57299275950818185 ) ) ;
#10981=VERTEX_POINT ( 'NONE', #39542 ) ;
#10983=CARTESIAN_POINT ( 'NONE',  ( -24.21176058185717750, -11.73806550877772459, 59.66048465809613077 ) ) ;
#10984=CARTESIAN_POINT ( 'NONE',  ( -16.06904454444675778, -7.890656075740461795, 63.67011029959335389 ) ) ;
#10985=CARTESIAN_POINT ( 'NONE',  ( -11.07857831884827604, -11.73724749328988359, 71.23860870961335934 ) ) ;
#10986=VERTEX_POINT ( 'NONE', #2114 ) ;
#10987=CARTESIAN_POINT ( 'NONE',  ( -19.49489006281195103, -21.96579734677897378, 62.15650173710307769 ) ) ;
#10988=CARTESIAN_POINT ( 'NONE',  ( -24.10584571748465521, -12.56049761727124370, 73.39225570139795707 ) ) ;
#10989=CARTESIAN_POINT ( 'NONE',  ( -18.39722185058254311, -7.818642594244027855, 70.52634850392742294 ) ) ;
#10990=ORIENTED_EDGE ( 'NONE', *, *, #35784, .T. ) ;
#10991=FACE_BOUND ( 'NONE', #7718, .T. ) ;
#10992=ORIENTED_EDGE ( 'NONE', *, *, #37390, .T. ) ;
#10993=CARTESIAN_POINT ( 'NONE',  ( -18.08661881476592015, -21.83173500943780354, 69.11514892715962333 ) ) ;
#10994=FACE_OUTER_BOUND ( 'NONE', #44730, .T. ) ;
#10997=PLANE ( 'NONE',  #30616 ) ;
#10998=ORIENTED_EDGE ( 'NONE', *, *, #10649, .T. ) ;
#11001=DIRECTION ( 'NONE',  ( -7.623677603559713149E-06, -4.209792907790860808E-06, 0.9999999999620784452 ) ) ;
#11002=CARTESIAN_POINT ( 'NONE',  ( -15.00366368785993032, -21.85518728482429296, 65.22783942216084085 ) ) ;
#11003=ORIENTED_EDGE ( 'NONE', *, *, #4473, .F. ) ;
#11004=FACE_OUTER_BOUND ( 'NONE', #11067, .T. ) ;
#11007=ORIENTED_EDGE ( 'NONE', *, *, #5206, .T. ) ;
#11009=AXIS2_PLACEMENT_3D ( 'NONE', #2498, #33228, #32303 ) ;
#11010=CARTESIAN_POINT ( 'NONE',  ( -22.86572475812252847, -14.01004878893095196, 53.49999999999995026 ) ) ;
#11012=CYLINDRICAL_SURFACE ( 'NONE', #12214, 0.1499999999999964972 ) ;
#11014=LINE ( 'NONE', #21847, #1166 ) ;
#11015=CARTESIAN_POINT ( 'NONE',  ( -17.82196845584967448, -7.369831403275952653, 60.28071967613077220 ) ) ;
#11017=ORIENTED_EDGE ( 'NONE', *, *, #538, .T. ) ;
#11018=VERTEX_POINT ( 'NONE', #35112 ) ;
#11019=CARTESIAN_POINT ( 'NONE',  ( -12.08328018599459597, -10.28419721118101293, 64.22017573579350369 ) ) ;
#11020=EDGE_CURVE ( 'NONE', #13357, #45579, #18439, .T. ) ;
#11022=CARTESIAN_POINT ( 'NONE',  ( -21.84008232946753836, -9.377762178279809291, 63.49153780852771689 ) ) ;
#11024=CARTESIAN_POINT ( 'NONE',  ( -10.38078070663892660, -14.50222156296673148, 67.85800126083267969 ) ) ;
#11027=( BOUNDED_SURFACE ( )  B_SPLINE_SURFACE ( 3, 1, ( 
 ( #25085, #9594 ),
 ( #10310, #28540 ),
 ( #25326, #32472 ),
 ( #10061, #17441 ),
 ( #24609, #28296 ),
 ( #39611, #17672 ),
 ( #32235, #32928 ) ),
 .UNSPECIFIED., .T., .F., .F. ) 
 B_SPLINE_SURFACE_WITH_KNOTS ( ( 4, 3, 4 ),
 ( 2, 2 ),
 ( 0.000000000000000000, 0.5000000000000000000, 1.000000000000000000 ),
 ( 0.000000000000000000, 1.000000000000000000 ),
 .UNSPECIFIED. ) 
 GEOMETRIC_REPRESENTATION_ITEM ( )  RATIONAL_B_SPLINE_SURFACE ( (
 ( 1.000000000000000000, 1.000000000000000000),
 ( 0.3333333333333335369, 0.3333333333333330373),
 ( 0.3333333333333335369, 0.3333333333333330373),
 ( 1.000000000000000000, 1.000000000000000000),
 ( 0.3333333333333333703, 0.3333333333333333703),
 ( 0.3333333333333333703, 0.3333333333333333703),
 ( 1.000000000000000000, 1.000000000000000000) ) ) 
 REPRESENTATION_ITEM ( '' )  SURFACE ( )  );
#11032=CARTESIAN_POINT ( 'NONE',  ( -21.18000274887674905, -20.77541536365158947, 69.05450184741354747 ) ) ;
#11034=DIRECTION ( 'NONE',  ( 1.259531062780516415E-05, -2.755480461857868066E-06, 0.9999999999168828202 ) ) ;
#11035=( BOUNDED_CURVE ( )  B_SPLINE_CURVE ( 3, ( #12162, #8468, #593, #23495 ),
 .UNSPECIFIED., .F., .F. ) 
 B_SPLINE_CURVE_WITH_KNOTS ( ( 4, 4 ),
 ( 0.5000000000000000000, 0.9074455897393631787 ),
 .UNSPECIFIED. ) 
 CURVE ( )  GEOMETRIC_REPRESENTATION_ITEM ( )  RATIONAL_B_SPLINE_CURVE ( ( 0.9999999999999987788, 0.4567392136813314685, 0.3561768502900308220, 0.6983129098260956180 ) ) 
 REPRESENTATION_ITEM ( '' )  );
#11037=CARTESIAN_POINT ( 'NONE',  ( -14.76781046749041870, -8.332642942470114278, 60.61996286262948530 ) ) ;
#11039=ORIENTED_EDGE ( 'NONE', *, *, #28820, .T. ) ;
#11040=CARTESIAN_POINT ( 'NONE',  ( -10.12790085937091078, -16.31526762935427755, 71.54726743650820708 ) ) ;
#11044=( BOUNDED_SURFACE ( )  B_SPLINE_SURFACE ( 3, 1, ( 
 ( #39725, #9933 ),
 ( #39487, #40217 ),
 ( #25199, #6485 ),
 ( #43435, #2548 ),
 ( #44176, #5766 ),
 ( #20773, #13837 ),
 ( #47607, #6717 ) ),
 .UNSPECIFIED., .T., .F., .F. ) 
 B_SPLINE_SURFACE_WITH_KNOTS ( ( 4, 3, 4 ),
 ( 2, 2 ),
 ( 0.000000000000000000, 0.5000000000000000000, 1.000000000000000000 ),
 ( 0.000000000000000000, 1.000000000000000000 ),
 .UNSPECIFIED. ) 
 GEOMETRIC_REPRESENTATION_ITEM ( )  RATIONAL_B_SPLINE_SURFACE ( (
 ( 1.000000000000000000, 1.000000000000000000),
 ( 0.3333333333333335369, 0.3333333333333330373),
 ( 0.3333333333333335369, 0.3333333333333330373),
 ( 1.000000000000000000, 1.000000000000000000),
 ( 0.3333333333333333703, 0.3333333333333333703),
 ( 0.3333333333333333703, 0.3333333333333333703),
 ( 1.000000000000000000, 1.000000000000000000) ) ) 
 REPRESENTATION_ITEM ( '' )  SURFACE ( )  );
#11045=EDGE_LOOP ( 'NONE', ( #15555, #23401 ) ) ;
#11046=CARTESIAN_POINT ( 'NONE',  ( -10.33300584886465856, -17.09388629248971370, 57.88034695574707200 ) ) ;
#11047=ADVANCED_FACE ( 'NONE', ( #35362 ), #27979, .T. ) ;
#11049=EDGE_CURVE ( 'NONE', #16961, #23554, #21442, .T. ) ;
#11050=CARTESIAN_POINT ( 'NONE',  ( -24.30048669258562555, -16.36410883687464946, 59.42332431756339162 ) ) ;
#11051=EDGE_LOOP ( 'NONE', ( #38108, #37314 ) ) ;
#11052=CARTESIAN_POINT ( 'NONE',  ( -22.14090652532222236, -20.04928072148792495, 62.51967078134249078 ) ) ;
#11053=EDGE_CURVE ( 'NONE', #40137, #38583, #30251, .T. ) ;
#11054=CARTESIAN_POINT ( 'NONE',  ( -20.20880001059865805, -8.386827409449249870, 70.55100337495873930 ) ) ;
#11055=ORIENTED_EDGE ( 'NONE', *, *, #8543, .F. ) ;
#11056=DIRECTION ( 'NONE',  ( -5.731567514496413899E-31, -1.020425574103664789E-16, -1.000000000000000000 ) ) ;
#11059=CARTESIAN_POINT ( 'NONE',  ( -18.11889358109259973, -21.82488563948435711, 65.64532159284070190 ) ) ;
#11060=CARTESIAN_POINT ( 'NONE',  ( -24.86610167639389246, -14.46236660854407674, 66.29797298380238146 ) ) ;
#11063=CARTESIAN_POINT ( 'NONE',  ( -23.73563655964320063, -11.66794921907180793, 63.25218274889858350 ) ) ;
#11066=EDGE_LOOP ( 'NONE', ( #7558, #45529 ) ) ;
#11067=EDGE_LOOP ( 'NONE', ( #17225, #34239, #24188, #9952, #4708 ) ) ;
#11068=CARTESIAN_POINT ( 'NONE',  ( -22.39254715322108780, -9.803279359720651343, 73.36672461330924477 ) ) ;
#11069=CARTESIAN_POINT ( 'NONE',  ( -24.28619334359350290, -16.42731978468327014, 59.13804568661029037 ) ) ;
#11070=CARTESIAN_POINT ( 'NONE',  ( -27.73618363589703506, -17.95286377743612505, 54.49999999999995026 ) ) ;
#11072=CARTESIAN_POINT ( 'NONE',  ( -23.21383278545907558, -10.12064720979650190, 63.11540053722242050 ) ) ;
#11073=CARTESIAN_POINT ( 'NONE',  ( -16.93761137771266689, -7.374984243389294036, 74.08205518084413654 ) ) ;
#11074=CARTESIAN_POINT ( 'NONE',  ( -14.74956200268320039, -8.338905876961694830, 63.86149019104595226 ) ) ;
#11075=ORIENTED_EDGE ( 'NONE', *, *, #19964, .T. ) ;
#11078=CARTESIAN_POINT ( 'NONE',  ( -14.03871066829747249, -8.172719617054283958, 70.91452941929576070 ) ) ;
#11080=LINE ( 'NONE', #26101, #32694 ) ;
#11081=CARTESIAN_POINT ( 'NONE',  ( -16.51211807517087493, -22.20323055888632169, 65.33290249375183123 ) ) ;
#11083=ORIENTED_EDGE ( 'NONE', *, *, #27733, .F. ) ;
#11086=CARTESIAN_POINT ( 'NONE',  ( -13.28646450387875966, -21.00477226788574114, 61.65612998380957777 ) ) ;
#11087=CARTESIAN_POINT ( 'NONE',  ( -13.82438241372512699, -21.33197126505688601, 72.04890825305675151 ) ) ;
#11092=CARTESIAN_POINT ( 'NONE',  ( -12.76547314785493192, -9.517330534081262172, 74.60450883341005124 ) ) ;
#11095=EDGE_LOOP ( 'NONE', ( #34194, #31966, #23924, #33253, #36285 ) ) ;
#11097=B_SPLINE_CURVE_WITH_KNOTS ( 'NONE', 3,
 ( #26664, #22736, #11888, #26415, #12124, #322, #30613, #34032, #558, #41922 ),
 .UNSPECIFIED., .F., .F.,
 ( 4, 2, 2, 2, 4 ),
 ( 0.1272669073657947958, 0.2522669073462836531, 0.3772669073267724826, 0.5022669073072613122, 0.6272669072877501417 ),
 .UNSPECIFIED. ) ;
#11098=CARTESIAN_POINT ( 'NONE',  ( -24.43235039625237803, -15.64544980915412431, 66.21891754810816622 ) ) ;
#11099=ORIENTED_EDGE ( 'NONE', *, *, #31025, .F. ) ;
#11100=CARTESIAN_POINT ( 'NONE',  ( -21.65477688667505518, -9.232350752012335349, 66.66149992610201025 ) ) ;
#11102=PLANE ( 'NONE',  #31465 ) ;
#11103=CARTESIAN_POINT ( 'NONE',  ( -24.40217295060720204, -14.25566147773195524, 69.95275273531336779 ) ) ;
#11105=CARTESIAN_POINT ( 'NONE',  ( -10.38360249164154325, -14.43747963625415309, 67.87272197508832505 ) ) ;
#11107=EDGE_CURVE ( 'NONE', #3454, #2663, #32989, .T. ) ;
#11109=VECTOR ( 'NONE', #26503, 1000.000000000000114 ) ;
#11110=CARTESIAN_POINT ( 'NONE',  ( -17.64597108892888500, -21.80612737151159664, 58.68936778192047399 ) ) ;
#11112=CARTESIAN_POINT ( 'NONE',  ( -24.47535868512742496, -14.65268306083313199, 66.59781357586173556 ) ) ;
#11114=DIRECTION ( 'NONE',  ( -0.2466764125338440639, -0.9690979039805150963, 7.162324212089591066E-08 ) ) ;
#11115=ORIENTED_EDGE ( 'NONE', *, *, #27340, .F. ) ;
#11117=CARTESIAN_POINT ( 'NONE',  ( -16.91093646999636135, -22.24163895736238317, 72.28826323766482176 ) ) ;
#11118=LINE ( 'NONE', #48050, #40018 ) ;
#11121=CARTESIAN_POINT ( 'NONE',  ( -16.19813999035177687, -21.75179513556690480, 58.28585572029250983 ) ) ;
#11122=CARTESIAN_POINT ( 'NONE',  ( -22.81570869814190772, -9.667889350279351035, 73.58137470877635167 ) ) ;
#11123=ORIENTED_EDGE ( 'NONE', *, *, #18050, .F. ) ;
#11124=ORIENTED_EDGE ( 'NONE', *, *, #10263, .T. ) ;
#11125=CARTESIAN_POINT ( 'NONE',  ( -16.90447120769729494, -21.79033274870119641, 72.18159849112339543 ) ) ;
#11126=CARTESIAN_POINT ( 'NONE',  ( -14.84918562769068018, -8.299994025627823291, 57.04137321387239723 ) ) ;
#11127=EDGE_LOOP ( 'NONE', ( #43749, #9745, #16519, #46490, #674 ) ) ;
#11128=DIRECTION ( 'NONE',  ( 6.385196549736874992E-06, -5.147825522337142951E-06, 0.9999999999663644612 ) ) ;
#11130=CARTESIAN_POINT ( 'NONE',  ( -11.86838218109940790, -9.845554053733961197, 64.14419007574942100 ) ) ;
#11131=FACE_OUTER_BOUND ( 'NONE', #35157, .T. ) ;
#11132=EDGE_CURVE ( 'NONE', #38153, #46391, #46263, .T. ) ;
#11134=DIRECTION ( 'NONE',  ( 2.117869074558178593E-07, 2.255668799892331646E-07, 0.9999999999999520384 ) ) ;
#11135=CARTESIAN_POINT ( 'NONE',  ( -24.68275054790482770, -16.48720572190336853, 59.23837039904986312 ) ) ;
#11136=CARTESIAN_POINT ( 'NONE',  ( -18.75147246090708109, -7.478239630221399814, 70.53101348938672288 ) ) ;
#11137=VERTEX_POINT ( 'NONE', #6780 ) ;
#11139=CARTESIAN_POINT ( 'NONE',  ( -11.32469211327616065, -18.34471187850051166, 57.95714594245092854 ) ) ;
#11141=B_SPLINE_CURVE_WITH_KNOTS ( 'NONE', 3,
 ( #47108, #9448, #31356, #8724, #31117, #13349, #28402, #1558, #35040, #5758 ),
 .UNSPECIFIED., .F., .F.,
 ( 4, 2, 2, 2, 4 ),
 ( 0.000000000000000000, 0.2500000000000000000, 0.5000000000000000000, 0.7500000000000000000, 1.000000000000000000 ),
 .UNSPECIFIED. ) ;
#11144=CARTESIAN_POINT ( 'NONE',  ( -24.27033198218900978, -13.12649362337911718, 62.83264177274070050 ) ) ;
#11145=CARTESIAN_POINT ( 'NONE',  ( -13.93897074462874919, -20.93787812888889377, 68.74153005185598886 ) ) ;
#11148=VERTEX_POINT ( 'NONE', #37276 ) ;
#11149=B_SPLINE_CURVE_WITH_KNOTS ( 'NONE', 1,
 ( #5273, #23505 ),
 .UNSPECIFIED., .F., .F.,
 ( 2, 2 ),
 ( 0.000000000000000000, 1.000000000000000000 ),
 .UNSPECIFIED. ) ;
#11152=EDGE_LOOP ( 'NONE', ( #47329, #14900, #36931, #44090, #25450 ) ) ;
#11153=CARTESIAN_POINT ( 'NONE',  ( -17.42403923091872642, -7.359153445762296464, 67.12765421629525520 ) ) ;
#11155=CARTESIAN_POINT ( 'NONE',  ( -12.81450527785482230, -9.474959380418823685, 74.61923006088066757 ) ) ;
#11158=LINE ( 'NONE', #6732, #17510 ) ;
#11160=DIRECTION ( 'NONE',  ( 0.4156784896208475244, 0.1649587623211671294, 0.8944271909999157444 ) ) ;
#11161=VECTOR ( 'NONE', #11887, 1000.000000000000114 ) ;
#11162=CARTESIAN_POINT ( 'NONE',  ( -17.55304533075025475, -7.360155577183800979, 63.68910541025692140 ) ) ;
#11163=ORIENTED_EDGE ( 'NONE', *, *, #4016, .T. ) ;
#11165=CARTESIAN_POINT ( 'NONE',  ( -12.21883005507435271, -20.13911453956916375, 64.96700631603125942 ) ) ;
#11166=EDGE_LOOP ( 'NONE', ( #42160, #38100, #8342, #45215, #31624 ) ) ;
#11167=DIRECTION ( 'NONE',  ( 3.549360974554993999E-17, -6.371834667797928663E-18, -1.000000000000000000 ) ) ;
#11168=CARTESIAN_POINT ( 'NONE',  ( -15.02609155194205393, -8.232647636148229253, 57.14999999999994884 ) ) ;
#11169=DIRECTION ( 'NONE',  ( -0.7224352045700189739, -0.6914386272098739239, 9.340627272150576816E-09 ) ) ;
#11170=ORIENTED_EDGE ( 'NONE', *, *, #26663, .T. ) ;
#11171=CARTESIAN_POINT ( 'NONE',  ( -20.19651366439481421, -7.894145410699936249, 73.84379675463323167 ) ) ;
#11176=DIRECTION ( 'NONE',  ( -0.5729733056696844073, 0.8195740302071247152, 7.403245352187747277E-08 ) ) ;
#11179=CARTESIAN_POINT ( 'NONE',  ( -9.979935309495182594, -14.51290508331406670, 68.05074287064346095 ) ) ;
#11180=CARTESIAN_POINT ( 'NONE',  ( -24.47217469393258327, -14.64471774706559515, 62.86296487297660462 ) ) ;
#11181=CARTESIAN_POINT ( 'NONE',  ( -11.42622172434740158, -18.51434208396348069, 61.42710833180511543 ) ) ;
#11182=CARTESIAN_POINT ( 'NONE',  ( -17.91840021365262814, -21.79173196354552644, 62.17535923606572368 ) ) ;
#11183=B_SPLINE_CURVE_WITH_KNOTS ( 'NONE', 3,
 ( #18368, #40538, #18121, #10749, #14172, #25054, #33374, #28978, #33138, #29227 ),
 .UNSPECIFIED., .F., .F.,
 ( 4, 2, 2, 2, 4 ),
 ( 0.000000000000000000, 0.2500000000000000000, 0.5000000000000000000, 0.7500000000000000000, 1.000000000000000000 ),
 .UNSPECIFIED. ) ;
#11184=ADVANCED_FACE ( 'NONE', ( #17602 ), #18196, .T. ) ;
#11188=CARTESIAN_POINT ( 'NONE',  ( -17.70014646425873295, -22.25421675543054789, 58.52836462438737897 ) ) ;
#11189=DIRECTION ( 'NONE',  ( 0.1261685609230672744, 0.9920088176193796459, 5.058037262945178220E-08 ) ) ;
#11190=ORIENTED_EDGE ( 'NONE', *, *, #16936, .F. ) ;
#11191=CARTESIAN_POINT ( 'NONE',  ( -11.33876662530985513, -19.10724307639906883, 68.33876836528679632 ) ) ;
#11192=EDGE_CURVE ( 'NONE', #13199, #23558, #34846, .T. ) ;
#11196=CARTESIAN_POINT ( 'NONE',  ( -18.37786432726835883, -21.79469297182707521, 69.10042588711679912 ) ) ;
#11197=( BOUNDED_CURVE ( )  B_SPLINE_CURVE ( 3, ( #36677, #7174, #36448, #44128 ),
 .UNSPECIFIED., .F., .F. ) 
 B_SPLINE_CURVE_WITH_KNOTS ( ( 4, 4 ),
 ( 4.712388980384689674, 4.921828490624009511 ),
 .UNSPECIFIED. ) 
 CURVE ( )  GEOMETRIC_REPRESENTATION_ITEM ( )  RATIONAL_B_SPLINE_CURVE ( ( 1.000000000000000000, 0.9963479302455154896, 0.9963479302455154896, 1.000000000000000000 ) ) 
 REPRESENTATION_ITEM ( '' )  );
#11198=B_SPLINE_CURVE_WITH_KNOTS ( 'NONE', 1,
 ( #13831, #32568 ),
 .UNSPECIFIED., .F., .F.,
 ( 2, 2 ),
 ( 0.000000000000000000, 1.000000000000000000 ),
 .UNSPECIFIED. ) ;
#11199=CARTESIAN_POINT ( 'NONE',  ( -23.44663229712023877, -18.37710346651732962, 73.04902823781205257 ) ) ;
#11201=VERTEX_POINT ( 'NONE', #8021 ) ;
#11203=CARTESIAN_POINT ( 'NONE',  ( -12.83553897491427342, -8.939779468292423203, 67.53976116287044817 ) ) ;
#11205=CARTESIAN_POINT ( 'NONE',  ( -15.55171241031346696, -7.598245096497682205, 70.79485117658632021 ) ) ;
#11207=CARTESIAN_POINT ( 'NONE',  ( -13.38575581802539993, -9.030060914960570173, 60.72478133471773987 ) ) ;
#11208=EDGE_CURVE ( 'NONE', #29545, #20111, #17823, .T. ) ;
#11209=ORIENTED_EDGE ( 'NONE', *, *, #32345, .T. ) ;
#11210=ORIENTED_EDGE ( 'NONE', *, *, #3491, .T. ) ;
#11212=B_SPLINE_CURVE_WITH_KNOTS ( 'NONE', 1,
 ( #34587, #18849 ),
 .UNSPECIFIED., .F., .F.,
 ( 2, 2 ),
 ( 0.000000000000000000, 1.000000000000000000 ),
 .UNSPECIFIED. ) ;
#11213=CARTESIAN_POINT ( 'NONE',  ( -21.33694466872984918, -9.004932385753821933, 73.90128753631783809 ) ) ;
#11214=CARTESIAN_POINT ( 'NONE',  ( -13.76849323099554567, -20.83774554052356009, 65.27156739751333703 ) ) ;
#11217=ORIENTED_EDGE ( 'NONE', *, *, #19995, .T. ) ;
#11220=CARTESIAN_POINT ( 'NONE',  ( -11.21783104652298846, -18.93062367394879431, 64.93202350587574756 ) ) ;
#11221=VERTEX_POINT ( 'NONE', #11213 ) ;
#11222=CARTESIAN_POINT ( 'NONE',  ( -24.47217469780904153, -14.64471797168181233, 63.01296487297644688 ) ) ;
#11224=CARTESIAN_POINT ( 'NONE',  ( -22.27695970603427966, -9.156476278077038344, 59.97817131676683999 ) ) ;
#11225=CARTESIAN_POINT ( 'NONE',  ( -24.83668925967022290, -14.06191770065747981, 73.26238150409892569 ) ) ;
#11226=CARTESIAN_POINT ( 'NONE',  ( -24.39669641284641699, -17.43334540211986550, 69.52065623779036230 ) ) ;
#11227=CARTESIAN_POINT ( 'NONE',  ( -9.991237185789255904, -14.30336124839046263, 64.49465555223780200 ) ) ;
#11228=VERTEX_POINT ( 'NONE', #41734 ) ;
#11229=CARTESIAN_POINT ( 'NONE',  ( -10.83541799943766293, -17.32598710976732903, 61.04254427365582103 ) ) ;
#11230=CARTESIAN_POINT ( 'NONE',  ( -22.78151503426583702, -19.98625364524674097, 72.75905110386234753 ) ) ;
#11231=DIRECTION ( 'NONE',  ( -8.419732596317119940E-06, 4.907637675873463559E-06, 0.9999999999525115424 ) ) ;
#11233=CARTESIAN_POINT ( 'NONE',  ( -10.37394849890712401, -14.76283852923608286, 71.61310637325181006 ) ) ;
#11235=CARTESIAN_POINT ( 'NONE',  ( -10.73038759976291878, -11.53849795754883623, 71.28199172907763170 ) ) ;
#11236=FACE_BOUND ( 'NONE', #26065, .T. ) ;
#11238=EDGE_LOOP ( 'NONE', ( #22031, #7072, #15647, #44775, #43956 ) ) ;
#11239=DIRECTION ( 'NONE',  ( -8.262539633966638414E-06, 9.998826072665628149E-07, 0.9999999999653652605 ) ) ;
#11241=CARTESIAN_POINT ( 'NONE',  ( -24.42122136640115571, -14.60445272614867562, 63.01296493458807646 ) ) ;
#11242=EDGE_CURVE ( 'NONE', #2922, #10698, #19820, .T. ) ;
#11243=CARTESIAN_POINT ( 'NONE',  ( -15.95707318215220205, -7.504986700048139170, 63.85506303619484214 ) ) ;
#11246=EDGE_LOOP ( 'NONE', ( #18284, #28091, #5391, #37052, #48149 ) ) ;
#11247=CARTESIAN_POINT ( 'NONE',  ( -22.78678303852979425, -9.565966637465477262, 53.49999999999994316 ) ) ;
#11249=CARTESIAN_POINT ( 'NONE',  ( -14.54749350918765671, -8.372447261038937327, 64.07506791522041567 ) ) ;
#11251=CARTESIAN_POINT ( 'NONE',  ( -21.48052744822966531, -21.05892743585564375, 72.71101825924023387 ) ) ;
#11252=CARTESIAN_POINT ( 'NONE',  ( -11.00662809167565470, -17.60509476157276865, 68.32395370577452809 ) ) ;
#11253=ORIENTED_EDGE ( 'NONE', *, *, #21753, .T. ) ;
#11254=ORIENTED_EDGE ( 'NONE', *, *, #3076, .F. ) ;
#11255=ORIENTED_EDGE ( 'NONE', *, *, #28655, .T. ) ;
#11256=CARTESIAN_POINT ( 'NONE',  ( -15.39388989008627995, -21.97733388496078177, 72.23070757706680922 ) ) ;
#11257=CARTESIAN_POINT ( 'NONE',  ( -24.39403702774331606, -17.44049340399234893, 69.52844358061491903 ) ) ;
#11258=CARTESIAN_POINT ( 'NONE',  ( -20.24919536711601964, -8.341303680600599790, 63.46688622775676691 ) ) ;
#11259=CARTESIAN_POINT ( 'NONE',  ( -24.23307633429531194, -12.98099662095383344, 66.30806553712001516 ) ) ;
#11263=EDGE_CURVE ( 'NONE', #36043, #39613, #21663, .T. ) ;
#11265=ORIENTED_EDGE ( 'NONE', *, *, #38935, .F. ) ;
#11266=CARTESIAN_POINT ( 'NONE',  ( -17.56717618076180187, -7.360494862701306928, 63.73552352176282909 ) ) ;
#11267=EDGE_CURVE ( 'NONE', #700, #44129, #2588, .T. ) ;
#11269=ADVANCED_FACE ( 'NONE', ( #24242 ), #28168, .T. ) ;
#11270=CARTESIAN_POINT ( 'NONE',  ( -22.48987839669337419, -20.27190899980916328, 65.81147567037690749 ) ) ;
#11271=CARTESIAN_POINT ( 'NONE',  ( -21.84008380685302342, -9.377763380601791710, 63.19153780853375935 ) ) ;
#11273=DIRECTION ( 'NONE',  ( -0.3478314405900310158, -0.9375570856950865561, 0.000000000000000000 ) ) ;
#11274=ORIENTED_EDGE ( 'NONE', *, *, #28985, .F. ) ;
#11276=ORIENTED_EDGE ( 'NONE', *, *, #26052, .F. ) ;
#11277=CARTESIAN_POINT ( 'NONE',  ( -16.07504252742545603, -21.67928465087502232, 58.51415545652290717 ) ) ;
#11278=CARTESIAN_POINT ( 'NONE',  ( -11.61908885153752813, -23.53148341178916425, 53.49999999999995026 ) ) ;
#11281=ORIENTED_EDGE ( 'NONE', *, *, #39533, .F. ) ;
#11282=CARTESIAN_POINT ( 'NONE',  ( -23.37999588001404661, -18.58199455739222827, 69.57899840282863124 ) ) ;
#11283=DIRECTION ( 'NONE',  ( 1.209056813000714825E-06, 5.657077699801570473E-07, 0.9999999999991090460 ) ) ;
#11284=CARTESIAN_POINT ( 'NONE',  ( -21.59308387932192730, -9.186008246182964854, 66.67652394132250038 ) ) ;
#11285=EDGE_CURVE ( 'NONE', #25938, #8282, #30164, .T. ) ;
#11287=CARTESIAN_POINT ( 'NONE',  ( -10.37462439815953275, -14.89569326811688832, 74.94778901494476031 ) ) ;
#11289=CARTESIAN_POINT ( 'NONE',  ( -23.88368001943721453, -17.64091657838220328, 66.35845829618112646 ) ) ;
#11292=VERTEX_POINT ( 'NONE', #28417 ) ;
#11293=CARTESIAN_POINT ( 'NONE',  ( -9.975020038748654727, -14.69173609724344054, 71.47782692972722884 ) ) ;
#11294=CARTESIAN_POINT ( 'NONE',  ( -24.87307799990805535, -14.67875618097862045, 62.83579567226647811 ) ) ;
#11295=ORIENTED_EDGE ( 'NONE', *, *, #15829, .T. ) ;
#11297=CARTESIAN_POINT ( 'NONE',  ( -11.08849928128054430, -11.70861240866882547, 74.65019981390956616 ) ) ;
#11298=FACE_OUTER_BOUND ( 'NONE', #21036, .T. ) ;
#11299=EDGE_CURVE ( 'NONE', #3450, #5029, #38324, .T. ) ;
#11301=FACE_OUTER_BOUND ( 'NONE', #14392, .T. ) ;
#11303=CARTESIAN_POINT ( 'NONE',  ( -10.93882922636242583, -17.44414199431199819, 68.09721938813615338 ) ) ;
#11304=EDGE_LOOP ( 'NONE', ( #37409, #20821 ) ) ;
#11305=CARTESIAN_POINT ( 'NONE',  ( -17.33262245845742910, -7.759502110702281463, 67.30567542699309058 ) ) ;
#11306=B_SPLINE_CURVE_WITH_KNOTS ( 'NONE', 1,
 ( #35550, #46406 ),
 .UNSPECIFIED., .F., .F.,
 ( 2, 2 ),
 ( 0.000000000000000000, 1.000000000000000000 ),
 .UNSPECIFIED. ) ;
#11307=CARTESIAN_POINT ( 'NONE',  ( -23.59327504554355315, -11.39630409041826020, 69.90682860766239060 ) ) ;
#11308=DIRECTION ( 'NONE',  ( -0.9118114225829224706, -0.4106092176842892627, -5.589476761700638069E-08 ) ) ;
#11310=ORIENTED_EDGE ( 'NONE', *, *, #9953, .T. ) ;
#11313=CARTESIAN_POINT ( 'NONE',  ( -23.46647660864419294, -19.16733412182131246, 62.39760931945144051 ) ) ;
#11314=ORIENTED_EDGE ( 'NONE', *, *, #5429, .F. ) ;
#11316=CARTESIAN_POINT ( 'NONE',  ( -24.82750207115152463, -13.97654542584719373, 73.30766806548945169 ) ) ;
#11317=( BOUNDED_CURVE ( )  B_SPLINE_CURVE ( 3, ( #39437, #12839, #42662, #39184 ),
 .UNSPECIFIED., .F., .F. ) 
 B_SPLINE_CURVE_WITH_KNOTS ( ( 4, 4 ),
 ( 0.5000000000000000000, 0.9074455897393687298 ),
 .UNSPECIFIED. ) 
 CURVE ( )  GEOMETRIC_REPRESENTATION_ITEM ( )  RATIONAL_B_SPLINE_CURVE ( ( 1.000000000000003775, 0.4567392136813261949, 0.3561768502900253264, 0.6983129098261054990 ) ) 
 REPRESENTATION_ITEM ( '' )  );
#11318=CARTESIAN_POINT ( 'NONE',  ( -11.55673057814116333, -10.21815940138198009, 71.01247170384147012 ) ) ;
#11321=CARTESIAN_POINT ( 'NONE',  ( -10.44202790750644461, -14.30845231023897846, 64.38803863533676974 ) ) ;
#11323=EDGE_CURVE ( 'NONE', #39442, #38153, #31146, .T. ) ;
#11324=CARTESIAN_POINT ( 'NONE',  ( -18.59601872632196518, -7.856991649524070809, 73.85536540707786912 ) ) ;
#11325=CARTESIAN_POINT ( 'NONE',  ( -10.52215087187021325, -13.37195826583270808, 74.67817647370830514 ) ) ;
#11326=( BOUNDED_CURVE ( )  B_SPLINE_CURVE ( 3, ( #20144, #42573, #27774, #16678 ),
 .UNSPECIFIED., .F., .F. ) 
 B_SPLINE_CURVE_WITH_KNOTS ( ( 4, 4 ),
 ( 0.000000000000000000, 0.4074455897393671755 ),
 .UNSPECIFIED. ) 
 CURVE ( )  GEOMETRIC_REPRESENTATION_ITEM ( )  RATIONAL_B_SPLINE_CURVE ( ( 1.000000000000000000, 0.4567392136813245296, 0.3561768502900275468, 0.6983129098261091627 ) ) 
 REPRESENTATION_ITEM ( '' )  );
#11327=ORIENTED_EDGE ( 'NONE', *, *, #17446, .F. ) ;
#11328=EDGE_CURVE ( 'NONE', #12343, #2068, #46827, .T. ) ;
#11329=EDGE_CURVE ( 'NONE', #15253, #897, #26412, .T. ) ;
#11330=ORIENTED_EDGE ( 'NONE', *, *, #17222, .T. ) ;
#11332=CARTESIAN_POINT ( 'NONE',  ( -15.38564177817468526, -21.97495498498005162, 72.15237147290109476 ) ) ;
#11333=CARTESIAN_POINT ( 'NONE',  ( -17.03575403388767384, -5.365376231199011414, 53.49999999999995026 ) ) ;
#11334=ORIENTED_EDGE ( 'NONE', *, *, #7016, .F. ) ;
#11335=CARTESIAN_POINT ( 'NONE',  ( -23.57564663096156821, -11.46866237256667986, 66.43716952005193832 ) ) ;
#11336=( BOUNDED_SURFACE ( )  B_SPLINE_SURFACE ( 3, 1, ( 
 ( #8757, #23774 ),
 ( #5054, #46661 ),
 ( #5293, #20064 ),
 ( #20309, #12907 ),
 ( #35316, #27931 ),
 ( #32372, #32123 ),
 ( #36744, #40465 ) ),
 .UNSPECIFIED., .T., .F., .F. ) 
 B_SPLINE_SURFACE_WITH_KNOTS ( ( 4, 3, 4 ),
 ( 2, 2 ),
 ( 0.000000000000000000, 0.5000000000000000000, 1.000000000000000000 ),
 ( 0.000000000000000000, 1.000000000000000000 ),
 .UNSPECIFIED. ) 
 GEOMETRIC_REPRESENTATION_ITEM ( )  RATIONAL_B_SPLINE_SURFACE ( (
 ( 1.000000000000000000, 1.000000000000000000),
 ( 0.3333333333333335369, 0.3333333333333330373),
 ( 0.3333333333333335369, 0.3333333333333330373),
 ( 1.000000000000000000, 1.000000000000000000),
 ( 0.3333333333333333703, 0.3333333333333333703),
 ( 0.3333333333333333703, 0.3333333333333333703),
 ( 1.000000000000000000, 1.000000000000000000) ) ) 
 REPRESENTATION_ITEM ( '' )  SURFACE ( )  );
#11337=LINE ( 'NONE', #3956, #7625 ) ;
#11338=ADVANCED_FACE ( 'NONE', ( #20549 ), #12888, .T. ) ;
#11339=VECTOR ( 'NONE', #19785, 1000.000000000000227 ) ;
#11341=CARTESIAN_POINT ( 'NONE',  ( -21.84103824432629892, -20.31425616591354455, 62.37872033649042436 ) ) ;
#11345=CARTESIAN_POINT ( 'NONE',  ( -19.23170823189057543, -21.62663761134119156, 62.40992444795293892 ) ) ;
#11346=CARTESIAN_POINT ( 'NONE',  ( -20.52762626839951210, -8.534807245883811788, 63.61121513079540080 ) ) ;
#11348=CARTESIAN_POINT ( 'NONE',  ( -17.22281210278579167, -7.361840297529252730, 70.60540404266352255 ) ) ;
#11351=CARTESIAN_POINT ( 'NONE',  ( -21.35069750557218526, -21.14061989791981944, 69.19416854129514149 ) ) ;
#11352=CARTESIAN_POINT ( 'NONE',  ( -24.20836943865575464, -17.88934756284849215, 62.66016244028183024 ) ) ;
#11353=CARTESIAN_POINT ( 'NONE',  ( -10.51883074965326870, -17.60604944894409130, 68.25868426185122928 ) ) ;
#11354=VERTEX_POINT ( 'NONE', #42943 ) ;
#11355=CARTESIAN_POINT ( 'NONE',  ( -16.19589554557147792, -7.461143648330228473, 60.35028476078848314 ) ) ;
#11356=CARTESIAN_POINT ( 'NONE',  ( -10.38752013045322009, -14.36951432065623635, 64.67331771650336236 ) ) ;
#11357=CARTESIAN_POINT ( 'NONE',  ( -18.24855905490383279, -21.76054561525072373, 65.57205495431095699 ) ) ;
#11362=VERTEX_POINT ( 'NONE', #38760 ) ;
#11363=CARTESIAN_POINT ( 'NONE',  ( -11.15620858584903807, -11.58171791265060691, 67.91864592172348125 ) ) ;
#11364=CARTESIAN_POINT ( 'NONE',  ( -14.95042625923249702, -8.260719279109913771, 57.14999999999994884 ) ) ;
#11365=VERTEX_POINT ( 'NONE', #46650 ) ;
#11366=CARTESIAN_POINT ( 'NONE',  ( -21.01123855637963089, -20.87838213191899683, 65.58453944497207999 ) ) ;
#11367=CARTESIAN_POINT ( 'NONE',  ( -23.34481533081060434, -18.63641918517796370, 69.44371984263474928 ) ) ;
#11368=CARTESIAN_POINT ( 'NONE',  ( -14.45223855097109578, -8.412213402796462347, 70.82137677761178907 ) ) ;
#11370=CARTESIAN_POINT ( 'NONE',  ( -11.13733870171179596, -11.61806121328042174, 67.90392505421056057 ) ) ;
#11373=FACE_OUTER_BOUND ( 'NONE', #24291, .T. ) ;
#11375=EDGE_CURVE ( 'NONE', #44310, #40803, #32496, .T. ) ;
#11376=CARTESIAN_POINT ( 'NONE',  ( -20.33143355559478138, -8.386436920021669295, 67.07544311258112657 ) ) ;
#11377=CARTESIAN_POINT ( 'NONE',  ( -15.63656756482722443, -8.039962711168056941, 74.30815578088962070 ) ) ;
#11381=CARTESIAN_POINT ( 'NONE',  ( -10.63726236355470078, -16.73075914568876144, 57.77940687674663423 ) ) ;
#11386=ORIENTED_EDGE ( 'NONE', *, *, #38662, .F. ) ;
#11387=CARTESIAN_POINT ( 'NONE',  ( -23.53769205375521167, -19.06701183966639945, 65.98535978091517507 ) ) ;
#11388=ADVANCED_FACE ( 'NONE', ( #21744 ), #39978, .T. ) ;
#11389=FACE_OUTER_BOUND ( 'NONE', #34804, .T. ) ;
#11390=EDGE_CURVE ( 'NONE', #46448, #32393, #1348, .T. ) ;
#11391=CARTESIAN_POINT ( 'NONE',  ( -13.60238289842206072, -8.884932333444998775, 57.26967755503795132 ) ) ;
#11392=CARTESIAN_POINT ( 'NONE',  ( -17.77594409791816688, -7.367433943401969998, 60.26556080592736464 ) ) ;
#11394=CARTESIAN_POINT ( 'NONE',  ( -23.11979735578276163, -10.00689463417326053, 66.73520565964795992 ) ) ;
#11395=CYLINDRICAL_SURFACE ( 'NONE', #34377, 0.1500000000000059897 ) ;
#11396=EDGE_LOOP ( 'NONE', ( #40627, #44077, #12011, #19609, #1024 ) ) ;
#11399=ORIENTED_EDGE ( 'NONE', *, *, #34830, .F. ) ;
#11400=CARTESIAN_POINT ( 'NONE',  ( -11.14868235907462335, -10.79371162966233832, 57.37049761327430275 ) ) ;
#11403=CARTESIAN_POINT ( 'NONE',  ( -22.53655473247544805, -20.22829521909097394, 65.88917159596024931 ) ) ;
#11406=CARTESIAN_POINT ( 'NONE',  ( -11.90843004312087494, -10.41235542147202153, 74.73885506873732254 ) ) ;
#11407=CARTESIAN_POINT ( 'NONE',  ( -10.55151165865014384, -17.68520938540437371, 68.28217272534745064 ) ) ;
#11408=ORIENTED_EDGE ( 'NONE', *, *, #39997, .F. ) ;
#11409=CARTESIAN_POINT ( 'NONE',  ( -11.71918404020638427, -18.95175453447547653, 71.70158022526054253 ) ) ;
#11411=CARTESIAN_POINT ( 'NONE',  ( -20.49170831689750472, -8.461258797198503601, 63.59649424907593129 ) ) ;
#11412=CARTESIAN_POINT ( 'NONE',  ( -23.37999588001404661, -18.58199455739222827, 69.57899840282863124 ) ) ;
#11413=CARTESIAN_POINT ( 'NONE',  ( -16.14669044099090556, -7.469368122434191903, 60.33881929519913712 ) ) ;
#11417=DIRECTION ( 'NONE',  ( -0.3478314405900307382, -0.9375570856950865561, 0.000000000000000000 ) ) ;
#11418=CARTESIAN_POINT ( 'NONE',  ( -14.79551189520038967, -8.264331297124348552, 64.20467431377564083 ) ) ;
#11420=CARTESIAN_POINT ( 'NONE',  ( -18.39027086422678536, -7.876143750135766730, 74.06737643580208896 ) ) ;
#11421=CARTESIAN_POINT ( 'NONE',  ( -22.52510384832546109, -10.01533137145497676, 73.78161092902590212 ) ) ;
#11422=CARTESIAN_POINT ( 'NONE',  ( -18.46801905451614090, -7.836623195388690455, 74.12592262855558545 ) ) ;
#11424=VERTEX_POINT ( 'NONE', #48090 ) ;
#11426=CARTESIAN_POINT ( 'NONE',  ( -18.39951368268757648, -22.19516171751901368, 69.00010101991060196 ) ) ;
#11429=B_SPLINE_CURVE_WITH_KNOTS ( 'NONE', 3,
 ( #25061, #32680, #48424, #14653, #13708, #6344, #43780, #29475, #29719, #47700 ),
 .UNSPECIFIED., .F., .F.,
 ( 4, 2, 2, 2, 4 ),
 ( 0.000000000000000000, 0.2500000000000000000, 0.5000000000000000000, 0.7500000000000000000, 1.000000000000000000 ),
 .UNSPECIFIED. ) ;
#11430=CARTESIAN_POINT ( 'NONE',  ( -14.39270346209745988, -8.498217395175695188, 70.95787461648006911 ) ) ;
#11431=CARTESIAN_POINT ( 'NONE',  ( -10.89013669529741790, -17.45722423822778779, 68.10281702760276801 ) ) ;
#11432=CARTESIAN_POINT ( 'NONE',  ( -15.48563737764182591, -8.027819004131977465, 70.49500973495348433 ) ) ;
#11435=EDGE_LOOP ( 'NONE', ( #637, #30964, #29585, #15767, #32272 ) ) ;
#11438=ADVANCED_FACE ( 'NONE', ( #32360 ), #28290, .T. ) ;
#11440=CARTESIAN_POINT ( 'NONE',  ( -11.68672710392437608, -10.05669134056747005, 67.68392285705759548 ) ) ;
#11441=ADVANCED_FACE ( 'NONE', ( #2779 ), #36164, .T. ) ;
#11442=( BOUNDED_CURVE ( )  B_SPLINE_CURVE ( 3, ( #28875, #5761, #32349, #9699 ),
 .UNSPECIFIED., .F., .F. ) 
 B_SPLINE_CURVE_WITH_KNOTS ( ( 4, 4 ),
 ( 1.570796326794896780, 1.780235837034217505 ),
 .UNSPECIFIED. ) 
 CURVE ( )  GEOMETRIC_REPRESENTATION_ITEM ( )  RATIONAL_B_SPLINE_CURVE ( ( 1.000000000000000000, 0.9963479302455154896, 0.9963479302455154896, 1.000000000000000000 ) ) 
 REPRESENTATION_ITEM ( '' )  );
#11444=B_SPLINE_CURVE_WITH_KNOTS ( 'NONE', 3,
 ( #47370, #43183, #27911, #42934, #47114, #38990, #39485, #17545, #28409, #13835 ),
 .UNSPECIFIED., .F., .F.,
 ( 4, 2, 2, 2, 4 ),
 ( 0.1272669073658669048, 0.2522669073463478795, 0.3772669073268288820, 0.5022669073073098289, 0.6272669072877907759 ),
 .UNSPECIFIED. ) ;
#11445=ADVANCED_FACE ( 'NONE', ( #11389 ), #2814, .T. ) ;
#11446=CARTESIAN_POINT ( 'NONE',  ( -16.13263948075386978, -7.878200451182638453, 63.68483172840383588 ) ) ;
#11447=CARTESIAN_POINT ( 'NONE',  ( -11.93522140360746242, -14.45952210441258678, 54.07175714974879099 ) ) ;
#11449=CARTESIAN_POINT ( 'NONE',  ( -11.56806251476610115, -18.73522173559940995, 65.03234934376791898 ) ) ;
#11451=VERTEX_POINT ( 'NONE', #8425 ) ;
#11452=( BOUNDED_SURFACE ( )  B_SPLINE_SURFACE ( 3, 1, ( 
 ( #6588, #21609 ),
 ( #32905, #14180 ),
 ( #29234, #44273 ),
 ( #10526, #25532 ),
 ( #21842, #36836 ),
 ( #18131, #3122 ),
 ( #23078, #26765 ) ),
 .UNSPECIFIED., .T., .F., .F. ) 
 B_SPLINE_SURFACE_WITH_KNOTS ( ( 4, 3, 4 ),
 ( 2, 2 ),
 ( 0.000000000000000000, 0.5000000000000000000, 1.000000000000000000 ),
 ( 0.000000000000000000, 1.000000000000000000 ),
 .UNSPECIFIED. ) 
 GEOMETRIC_REPRESENTATION_ITEM ( )  RATIONAL_B_SPLINE_SURFACE ( (
 ( 1.000000000000000000, 1.000000000000000000),
 ( 0.3333333333333335369, 0.3333333333333330373),
 ( 0.3333333333333335369, 0.3333333333333330373),
 ( 1.000000000000000000, 1.000000000000000000),
 ( 0.3333333333333333703, 0.3333333333333333703),
 ( 0.3333333333333333703, 0.3333333333333333703),
 ( 1.000000000000000000, 1.000000000000000000) ) ) 
 REPRESENTATION_ITEM ( '' )  SURFACE ( )  );
#11454=( BOUNDED_CURVE ( )  B_SPLINE_CURVE ( 3, ( #46718, #42297, #23832, #38834 ),
 .UNSPECIFIED., .F., .F. ) 
 B_SPLINE_CURVE_WITH_KNOTS ( ( 4, 4 ),
 ( 0.5000000000000000000, 0.9074455897393605142 ),
 .UNSPECIFIED. ) 
 CURVE ( )  GEOMETRIC_REPRESENTATION_ITEM ( )  RATIONAL_B_SPLINE_CURVE ( ( 0.9999999999999941158, 0.4567392136813325232, 0.3561768502900345412, 0.6983129098260937306 ) ) 
 REPRESENTATION_ITEM ( '' )  );
#11456=CARTESIAN_POINT ( 'NONE',  ( -13.01353397724842154, -8.804979801064929390, 64.09441804368185558 ) ) ;
#11457=CARTESIAN_POINT ( 'NONE',  ( -10.11824970337647223, -16.26811690260224452, 71.56254994910038647 ) ) ;
#11458=CARTESIAN_POINT ( 'NONE',  ( -12.52591642561268515, -9.195683996340104471, 74.50418400381258266 ) ) ;
#11459=CARTESIAN_POINT ( 'NONE',  ( -18.16972350937645686, -22.22180848762789296, 65.54520937023384874 ) ) ;
#11461=CARTESIAN_POINT ( 'NONE',  ( -13.28405640107581220, -24.63958226071216728, 54.49999999999995026 ) ) ;
#11462=FACE_OUTER_BOUND ( 'NONE', #6721, .T. ) ;
#11463=CARTESIAN_POINT ( 'NONE',  ( -20.10157833785231674, -8.341446982617696904, 70.26602821964115719 ) ) ;
#11464=CARTESIAN_POINT ( 'NONE',  ( -24.31456749111805848, -16.04512898536875198, 66.07941623514170715 ) ) ;
#11465=VERTEX_POINT ( 'NONE', #11155 ) ;
#11466=CARTESIAN_POINT ( 'NONE',  ( -10.52422430310768320, -17.61911375464911700, 68.21226508126260057 ) ) ;
#11468=CARTESIAN_POINT ( 'NONE',  ( -10.73412848974934874, -11.53077067998621175, 71.20365450754333381 ) ) ;
#11469=( BOUNDED_CURVE ( )  B_SPLINE_CURVE ( 3, ( #21634, #13501, #28544, #35665 ),
 .UNSPECIFIED., .F., .F. ) 
 B_SPLINE_CURVE_WITH_KNOTS ( ( 4, 4 ),
 ( 0.000000000000000000, 0.4074455897393634562 ),
 .UNSPECIFIED. ) 
 CURVE ( )  GEOMETRIC_REPRESENTATION_ITEM ( )  RATIONAL_B_SPLINE_CURVE ( ( 1.000000000000000000, 0.4567392136813352432, 0.3561768502900315436, 0.6983129098260888457 ) ) 
 REPRESENTATION_ITEM ( '' )  );
#11471=FACE_BOUND ( 'NONE', #30499, .T. ) ;
#11474=CARTESIAN_POINT ( 'NONE',  ( -13.17849012079414095, -20.93114571188291961, 58.23924207018498578 ) ) ;
#11476=CARTESIAN_POINT ( 'NONE',  ( -24.42218830102925509, -14.64588410380239480, 62.71296487252168816 ) ) ;
#11477=CARTESIAN_POINT ( 'NONE',  ( -21.08681864223905578, -8.776014225774568800, 73.75695571861821520 ) ) ;
#11479=CARTESIAN_POINT ( 'NONE',  ( -10.11857101092534528, -16.26968670661729632, 71.70396332877544410 ) ) ;
#11482=CARTESIAN_POINT ( 'NONE',  ( -16.99415041099795332, -7.769321291326151346, 70.37547239324983650 ) ) ;
#11483=EDGE_CURVE ( 'NONE', #17387, #2275, #17216, .T. ) ;
#11484=CARTESIAN_POINT ( 'NONE',  ( -14.35020019311386719, -8.022098033332648370, 63.90323595109556720 ) ) ;
#11486=CARTESIAN_POINT ( 'NONE',  ( -13.53684336123755472, -20.63065685511644887, 58.15535990049952630 ) ) ;
#11487=B_SPLINE_CURVE_WITH_KNOTS ( 'NONE', 3,
 ( #7691, #777, #22705, #41652, #30828, #37697, #3735, #11861, #34490, #3988 ),
 .UNSPECIFIED., .F., .F.,
 ( 4, 2, 2, 2, 4 ),
 ( 0.1272669073658512784, 0.2522669073463361111, 0.3772669073268208884, 0.5022669073073057211, 0.6272669072877905538 ),
 .UNSPECIFIED. ) ;
#11488=ORIENTED_EDGE ( 'NONE', *, *, #12947, .T. ) ;
#11489=EDGE_LOOP ( 'NONE', ( #24579, #12220, #37965, #3311, #26362 ) ) ;
#11492=CYLINDRICAL_SURFACE ( 'NONE', #7657, 0.1499999999999949984 ) ;
#11493=CARTESIAN_POINT ( 'NONE',  ( -19.30706890485013005, -22.01740903849647069, 58.64011989901568711 ) ) ;
#11494=CARTESIAN_POINT ( 'NONE',  ( -20.49170831689750827, -8.461258797198503601, 63.59649424907591708 ) ) ;
#11496=CARTESIAN_POINT ( 'NONE',  ( -16.19814381282456495, -21.75179583453235210, 58.58585572026735377 ) ) ;
#11499=ORIENTED_EDGE ( 'NONE', *, *, #10651, .F. ) ;
#11500=VERTEX_POINT ( 'NONE', #319 ) ;
#11501=CARTESIAN_POINT ( 'NONE',  ( -11.98246295270348050, -15.60836430055780610, 53.49999999999995026 ) ) ;
#11502=CARTESIAN_POINT ( 'NONE',  ( -13.87531073599090448, -8.258727944021641676, 74.39943442283376385 ) ) ;
#11503=B_SPLINE_CURVE_WITH_KNOTS ( 'NONE', 1,
 ( #7823, #30713 ),
 .UNSPECIFIED., .F., .F.,
 ( 2, 2 ),
 ( 0.000000000000000000, 1.000000000000000000 ),
 .UNSPECIFIED. ) ;
#11504=FACE_OUTER_BOUND ( 'NONE', #9873, .T. ) ;
#11506=ORIENTED_EDGE ( 'NONE', *, *, #48681, .T. ) ;
#11508=VECTOR ( 'NONE', #30802, 1000.000000000000000 ) ;
#11510=ORIENTED_EDGE ( 'NONE', *, *, #15800, .T. ) ;
#11512=CARTESIAN_POINT ( 'NONE',  ( -20.03282965983824226, -21.84088468745754597, 53.89198173725360874 ) ) ;
#11514=CARTESIAN_POINT ( 'NONE',  ( -10.43949455435184603, -13.84896052950683298, 57.46297163929641982 ) ) ;
#11516=B_SPLINE_CURVE_WITH_KNOTS ( 'NONE', 3,
 ( #26556, #7617, #14228, #3168, #15209, #10566, #41579, #6868, #11054, #37123 ),
 .UNSPECIFIED., .F., .F.,
 ( 4, 2, 2, 2, 4 ),
 ( 0.000000000000000000, 0.2500000000000000000, 0.5000000000000000000, 0.7500000000000000000, 1.000000000000000000 ),
 .UNSPECIFIED. ) ;
#11518=CARTESIAN_POINT ( 'NONE',  ( -20.35888297561835003, -7.961606991444354797, 70.45111537669373547 ) ) ;
#11519=CARTESIAN_POINT ( 'NONE',  ( -14.68149645524703928, -8.368787582623010479, 60.39284412189408613 ) ) ;
#11520=ORIENTED_EDGE ( 'NONE', *, *, #7541, .F. ) ;
#11521=CARTESIAN_POINT ( 'NONE',  ( -10.43429035678604500, -13.88957849880590700, 57.44825060447983844 ) ) ;
#11523=CARTESIAN_POINT ( 'NONE',  ( -10.41921500249975807, -15.63170790598816140, 64.92260423241262401 ) ) ;
#11524=CARTESIAN_POINT ( 'NONE',  ( -24.29205067375949056, -17.69794899492463713, 66.13012485676826202 ) ) ;
#11525=EDGE_LOOP ( 'NONE', ( #2385, #9017, #27037, #23304, #5445 ) ) ;
#11526=DIRECTION ( 'NONE',  ( -3.913797937844888413E-06, -1.965591629113562018E-06, -0.9999999999904092274 ) ) ;
#11528=ORIENTED_EDGE ( 'NONE', *, *, #8919, .F. ) ;
#11529=DIRECTION ( 'NONE',  ( 0.04287186434519785205, 0.9990805789562556827, -2.806673972535358096E-09 ) ) ;
#11530=CARTESIAN_POINT ( 'NONE',  ( -24.72694788909437236, -16.28301151488813403, 62.70833397083087846 ) ) ;
#11532=ADVANCED_FACE ( 'NONE', ( #26656 ), #77, .T. ) ;
#11535=CARTESIAN_POINT ( 'NONE',  ( -24.14679772577363437, -12.68507108172156883, 70.05770892828130059 ) ) ;
#11536=CARTESIAN_POINT ( 'NONE',  ( -18.54310121003094736, -22.17474206275902660, 72.39236802054413999 ) ) ;
#11537=ORIENTED_EDGE ( 'NONE', *, *, #39795, .T. ) ;
#11538=CARTESIAN_POINT ( 'NONE',  ( -22.23348325011687976, -19.89560912233985590, 66.00421727876722855 ) ) ;
#11539=CARTESIAN_POINT ( 'NONE',  ( -11.46189391869686958, -11.14137219122531697, 57.22405587208396582 ) ) ;
#11541=FACE_OUTER_BOUND ( 'NONE', #25483, .T. ) ;
#11542=AXIS2_PLACEMENT_3D ( 'NONE', #23135, #45549, #27057 ) ;
#11543=CARTESIAN_POINT ( 'NONE',  ( -21.47456293661849713, -9.038556783377254433, 70.41660404402310292 ) ) ;
#11545=VERTEX_POINT ( 'NONE', #22731 ) ;
#11546=CARTESIAN_POINT ( 'NONE',  ( -22.80992488001626128, -10.33718742043409122, 66.55798901525795941 ) ) ;
#11547=CARTESIAN_POINT ( 'NONE',  ( -10.69964535969413433, -11.60199994243103028, 71.26577769276515539 ) ) ;
#11550=( BOUNDED_CURVE ( )  B_SPLINE_CURVE ( 3, ( #12160, #1073, #16072, #4522 ),
 .UNSPECIFIED., .F., .F. ) 
 B_SPLINE_CURVE_WITH_KNOTS ( ( 4, 4 ),
 ( 1.675516081914546707, 1.780235837034217505 ),
 .UNSPECIFIED. ) 
 CURVE ( )  GEOMETRIC_REPRESENTATION_ITEM ( )  RATIONAL_B_SPLINE_CURVE ( ( 1.000000000000000000, 0.9990863565030491111, 0.9990863565030491111, 1.000000000000000000 ) ) 
 REPRESENTATION_ITEM ( '' )  );
#11553=FACE_OUTER_BOUND ( 'NONE', #18846, .T. ) ;
#11554=DIRECTION ( 'NONE',  ( -0.8604039311673230550, -0.5096126717731922495, 7.110477544621476444E-08 ) ) ;
#11555=LINE ( 'NONE', #28023, #34983 ) ;
#11556=CARTESIAN_POINT ( 'NONE',  ( -9.975266540682891758, -14.95048458752718545, 74.93632366797223199 ) ) ;
#11557=ORIENTED_EDGE ( 'NONE', *, *, #28985, .T. ) ;
#11558=CARTESIAN_POINT ( 'NONE',  ( -10.43125849979191955, -13.91324152291312366, 57.74825034919034294 ) ) ;
#11560=CARTESIAN_POINT ( 'NONE',  ( -10.03807673793979838, -13.83450552870046479, 57.55550895888026020 ) ) ;
#11562=EDGE_LOOP ( 'NONE', ( #21592, #38526, #10930, #37191, #12292 ) ) ;
#11564=EDGE_CURVE ( 'NONE', #33331, #1365, #17898, .T. ) ;
#11566=CARTESIAN_POINT ( 'NONE',  ( -10.64823572114831585, -13.04561703115311566, 71.31901764264975441 ) ) ;
#11568=DIRECTION ( 'NONE',  ( -5.731567514496413899E-31, -1.020425574103664789E-16, -1.000000000000000000 ) ) ;
#11570=CARTESIAN_POINT ( 'NONE',  ( -11.54484398236026799, -18.70636738123116061, 61.48530584391141929 ) ) ;
#11573=FACE_OUTER_BOUND ( 'NONE', #40374, .T. ) ;
#11574=ORIENTED_EDGE ( 'NONE', *, *, #759, .T. ) ;
#11575=CARTESIAN_POINT ( 'NONE',  ( -10.78898398081525301, -17.19290454168847404, 61.44271037915215317 ) ) ;
#11578=CARTESIAN_POINT ( 'NONE',  ( -23.00454255336054743, -10.50046069577333441, 59.88731295783226471 ) ) ;
#11579=ORIENTED_EDGE ( 'NONE', *, *, #45578, .T. ) ;
#11580=CARTESIAN_POINT ( 'NONE',  ( -17.53144728931050977, -7.808750373270764378, 67.09209771269890155 ) ) ;
#11581=EDGE_CURVE ( 'NONE', #6378, #4829, #39556, .T. ) ;
#11582=ORIENTED_EDGE ( 'NONE', *, *, #40147, .T. ) ;
#11583=CARTESIAN_POINT ( 'NONE',  ( -15.02405691534179688, -8.340062653448301333, 75.49999999999994316 ) ) ;
#11585=ORIENTED_EDGE ( 'NONE', *, *, #216, .T. ) ;
#11586=CARTESIAN_POINT ( 'NONE',  ( -17.59331746331979929, -7.761237803891376075, 63.55057029381061540 ) ) ;
#11587=EDGE_CURVE ( 'NONE', #32492, #5613, #23095, .T. ) ;
#11588=ADVANCED_FACE ( 'NONE', ( #20226 ), #23709, .T. ) ;
#11589=CARTESIAN_POINT ( 'NONE',  ( -24.28579947082789303, -13.18942387424446316, 62.84736316175410309 ) ) ;
#11591=DIRECTION ( 'NONE',  ( 0.6105870317843965500, 0.7919491628991826015, -6.540688078241514573E-08 ) ) ;
#11592=( BOUNDED_CURVE ( )  B_SPLINE_CURVE ( 3, ( #14545, #14317, #6961, #43680 ),
 .UNSPECIFIED., .F., .F. ) 
 B_SPLINE_CURVE_WITH_KNOTS ( ( 4, 4 ),
 ( 0.5000000000000000000, 0.9074455897393657322 ),
 .UNSPECIFIED. ) 
 CURVE ( )  GEOMETRIC_REPRESENTATION_ITEM ( )  RATIONAL_B_SPLINE_CURVE ( ( 1.000000000000009326, 0.4567392136813359649, 0.3561768502900252154, 0.6983129098260869583 ) ) 
 REPRESENTATION_ITEM ( '' )  );
#11593=CARTESIAN_POINT ( 'NONE',  ( -14.25068859620041017, -8.513811488652077486, 70.72957628655862550 ) ) ;
#11595=ORIENTED_EDGE ( 'NONE', *, *, #29115, .F. ) ;
#11596=CARTESIAN_POINT ( 'NONE',  ( -10.43689247203059267, -14.38509032613565530, 64.67338506919912788 ) ) ;
#11597=CARTESIAN_POINT ( 'NONE',  ( -13.21599742097365038, -20.46930908964682416, 58.46138952334620598 ) ) ;
#11598=EDGE_CURVE ( 'NONE', #44533, #3166, #4737, .T. ) ;
#11600=CARTESIAN_POINT ( 'NONE',  ( -10.70566838141854404, -16.94585318031169763, 57.83760548748448116 ) ) ;
#11601=CARTESIAN_POINT ( 'NONE',  ( -22.84886471163500588, -9.702775354051940582, 73.59665661135821324 ) ) ;
#11602=EDGE_LOOP ( 'NONE', ( #462, #7937, #2165, #38914, #17821 ) ) ;
#11604=CARTESIAN_POINT ( 'NONE',  ( -21.40186815114211782, -9.048699395220948460, 73.88512259465339582 ) ) ;
#11607=CARTESIAN_POINT ( 'NONE',  ( -24.11267623503602664, -17.03798637408549155, 73.17776260608479788 ) ) ;
#11609=CARTESIAN_POINT ( 'NONE',  ( -11.65817609178158065, -18.77836167696750636, 64.93810149108783492 ) ) ;
#11610=CARTESIAN_POINT ( 'NONE',  ( -17.20139249542113191, -7.812750000685961815, 70.49035839633111777 ) ) ;
#11611=CARTESIAN_POINT ( 'NONE',  ( -23.59416455813390101, -18.98475620612148518, 65.96242875894608915 ) ) ;
#11612=( BOUNDED_CURVE ( )  B_SPLINE_CURVE ( 3, ( #22938, #26128, #26614, #41140 ),
 .UNSPECIFIED., .F., .F. ) 
 B_SPLINE_CURVE_WITH_KNOTS ( ( 4, 4 ),
 ( 0.5000000000000000000, 0.9074455897393642889 ),
 .UNSPECIFIED. ) 
 CURVE ( )  GEOMETRIC_REPRESENTATION_ITEM ( )  RATIONAL_B_SPLINE_CURVE ( ( 1.000000000000009104, 0.4567392136813325232, 0.3561768502900241051, 0.6983129098260936196 ) ) 
 REPRESENTATION_ITEM ( '' )  );
#11616=CARTESIAN_POINT ( 'NONE',  ( -19.24190894175819366, -7.584296403803404196, 63.54593838833191910 ) ) ;
#11617=EDGE_CURVE ( 'NONE', #30363, #24642, #37812, .T. ) ;
#11619=CARTESIAN_POINT ( 'NONE',  ( -16.36834455927873222, -22.18410795223847387, 61.94063518049016182 ) ) ;
#11620=AXIS2_PLACEMENT_3D ( 'NONE', #44312, #18924, #25577 ) ;
#11622=CARTESIAN_POINT ( 'NONE',  ( -10.46944733747312917, -15.96661384539355133, 67.99239968927004441 ) ) ;
#11625=ORIENTED_EDGE ( 'NONE', *, *, #41319, .T. ) ;
#11628=EDGE_LOOP ( 'NONE', ( #25185, #26338, #44454, #13420, #43539 ) ) ;
#11631=DIRECTION ( 'NONE',  ( -5.731567514496413899E-31, -1.020425574103664789E-16, -1.000000000000000000 ) ) ;
#11632=FACE_OUTER_BOUND ( 'NONE', #48423, .T. ) ;
#11633=ORIENTED_EDGE ( 'NONE', *, *, #27277, .F. ) ;
#11634=CARTESIAN_POINT ( 'NONE',  ( -13.41301606045583128, -21.08813317394188758, 65.17284274790917209 ) ) ;
#11635=VECTOR ( 'NONE', #14750, 999.9999999999998863 ) ;
#11636=CARTESIAN_POINT ( 'NONE',  ( -17.56018945634354722, -7.360327109558735259, 63.67244293056884175 ) ) ;
#11637=VERTEX_POINT ( 'NONE', #34765 ) ;
#11638=CARTESIAN_POINT ( 'NONE',  ( -10.63004074901718532, -12.92571453866564823, 67.75304464120749515 ) ) ;
#11639=CARTESIAN_POINT ( 'NONE',  ( -20.69509153224808173, -8.115601224564374050, 63.49616927690831858 ) ) ;
#11640=CIRCLE ( 'NONE', #686, 7.500000000000002665 ) ;
#11642=ORIENTED_EDGE ( 'NONE', *, *, #40833, .T. ) ;
#11643=CARTESIAN_POINT ( 'NONE',  ( -10.37095245282503342, -14.72771709220537240, 68.06620091705121922 ) ) ;
#11644=DIRECTION ( 'NONE',  ( -0.2479245821708705444, -0.9687793358424813261, 9.885672099568325381E-17 ) ) ;
#11645=CARTESIAN_POINT ( 'NONE',  ( -12.12786991918758339, -13.32596279628197600, 54.07175714974879099 ) ) ;
#11646=ORIENTED_EDGE ( 'NONE', *, *, #46819, .F. ) ;
#11647=CARTESIAN_POINT ( 'NONE',  ( -19.64493811714022087, -21.44926310044305851, 69.04555521092800063 ) ) ;
#11648=EDGE_CURVE ( 'NONE', #10296, #26347, #6676, .T. ) ;
#11649=CARTESIAN_POINT ( 'NONE',  ( -23.04402284766838349, -19.06632961612601918, 59.16938527523783620 ) ) ;
#11650=B_SPLINE_CURVE_WITH_KNOTS ( 'NONE', 3,
 ( #10531, #39835, #13943, #44041, #13713, #47954, #28756, #35643, #46981, #1926 ),
 .UNSPECIFIED., .F., .F.,
 ( 4, 2, 2, 2, 4 ),
 ( 0.000000000000000000, 0.2500000000000000000, 0.5000000000000000000, 0.7500000000000000000, 1.000000000000000000 ),
 .UNSPECIFIED. ) ;
#11651=AXIS2_PLACEMENT_3D ( 'NONE', #33009, #14291, #10868 ) ;
#11654=ORIENTED_EDGE ( 'NONE', *, *, #11242, .T. ) ;
#11655=CARTESIAN_POINT ( 'NONE',  ( -24.69852180232685157, -16.41745880042978101, 59.30827708941524889 ) ) ;
#11656=CARTESIAN_POINT ( 'NONE',  ( -10.99582178678916833, -11.91441492378913480, 74.85840195586327184 ) ) ;
#11659=CARTESIAN_POINT ( 'NONE',  ( -23.91468471116454708, -11.15204413962362828, 70.09221953707209707 ) ) ;
#11660=EDGE_CURVE ( 'NONE', #17355, #16961, #14714, .T. ) ;
#11661=EDGE_CURVE ( 'NONE', #23333, #47654, #31740, .T. ) ;
#11662=CARTESIAN_POINT ( 'NONE',  ( -22.17130234749883044, -20.55096496926394778, 58.87947491310501391 ) ) ;
#11664=EDGE_LOOP ( 'NONE', ( #1195, #9184 ) ) ;
#11665=EDGE_CURVE ( 'NONE', #42290, #48213, #12707, .T. ) ;
#11668=EDGE_LOOP ( 'NONE', ( #2166, #41367, #23327, #47134, #26423 ) ) ;
#11672=VERTEX_POINT ( 'NONE', #20486 ) ;
#11673=CARTESIAN_POINT ( 'NONE',  ( -18.32857756213031664, -22.20418371868804996, 68.93019407337365578 ) ) ;
#11674=CARTESIAN_POINT ( 'NONE',  ( -19.93798644100873574, -21.82225466599480157, 69.08482476138111394 ) ) ;
#11677=ORIENTED_EDGE ( 'NONE', *, *, #12140, .F. ) ;
#11682=CARTESIAN_POINT ( 'NONE',  ( -24.80663772805713307, -15.80987445113336776, 69.72581619873751890 ) ) ;
#11683=CARTESIAN_POINT ( 'NONE',  ( -15.74783386771837890, -7.961078896070159061, 70.62461975990308360 ) ) ;
#11684=CARTESIAN_POINT ( 'NONE',  ( -13.56513943501515840, -8.968887331962283938, 57.25502341335112533 ) ) ;
#11686=AXIS2_PLACEMENT_3D ( 'NONE', #19345, #23296, #11975 ) ;
#11687=VERTEX_POINT ( 'NONE', #28356 ) ;
#11688=ORIENTED_EDGE ( 'NONE', *, *, #35447, .F. ) ;
#11690=CARTESIAN_POINT ( 'NONE',  ( -20.31649760022732565, -7.943510736669368910, 70.43595667626200907 ) ) ;
#11694=B_SPLINE_CURVE_WITH_KNOTS ( 'NONE', 3,
 ( #22743, #4748, #15075, #19772, #11897, #15810, #4496, #11165, #30864, #26917 ),
 .UNSPECIFIED., .F., .F.,
 ( 4, 2, 2, 2, 4 ),
 ( 0.6272669072876895235, 0.7522669073072305590, 0.8772669073267717055, 1.002266907346312852, 1.127266907365853887 ),
 .UNSPECIFIED. ) ;
#11696=CARTESIAN_POINT ( 'NONE',  ( -20.78299823145727387, -8.610459808214880439, 59.85597358678664648 ) ) ;
#11697=CARTESIAN_POINT ( 'NONE',  ( -24.42401644153718721, -14.84212863923847081, 59.24300237020570137 ) ) ;
#11701=CARTESIAN_POINT ( 'NONE',  ( -23.00382349513648350, -19.03821702553108253, 62.58236827718467765 ) ) ;
#11702=ORIENTED_EDGE ( 'NONE', *, *, #8206, .F. ) ;
#11703=CARTESIAN_POINT ( 'NONE',  ( -21.94242186726961208, -9.397052521110282441, 60.00699132926281010 ) ) ;
#11704=CARTESIAN_POINT ( 'NONE',  ( -18.50931870666621037, -21.77518001355031529, 72.28510940651260341 ) ) ;
#11705=CARTESIAN_POINT ( 'NONE',  ( -18.60148480518915548, -7.908490531605076868, 74.12447901480395274 ) ) ;
#11706=DIRECTION ( 'NONE',  ( 0.6380325334150297456, -0.7700094066334507437, 1.806162864933161516E-16 ) ) ;
#11707=EDGE_CURVE ( 'NONE', #32753, #14163, #253, .T. ) ;
#11708=ORIENTED_EDGE ( 'NONE', *, *, #14758, .T. ) ;
#11709=B_SPLINE_CURVE_WITH_KNOTS ( 'NONE', 1,
 ( #22051, #22531 ),
 .UNSPECIFIED., .F., .F.,
 ( 2, 2 ),
 ( 0.000000000000000000, 1.000000000000000000 ),
 .UNSPECIFIED. ) ;
#11710=DIRECTION ( 'NONE',  ( 0.3224496555704363665, 0.8691421305882583992, -0.3749909018349775192 ) ) ;
#11711=VECTOR ( 'NONE', #44206, 1000.000000000000114 ) ;
#11712=CARTESIAN_POINT ( 'NONE',  ( -24.68759284454203851, -16.46579109868681812, 59.22358191938879202 ) ) ;
#11713=FACE_OUTER_BOUND ( 'NONE', #44786, .T. ) ;
#11714=CARTESIAN_POINT ( 'NONE',  ( -24.49266415654671292, -17.16299127166918126, 73.02189535998635961 ) ) ;
#11716=CARTESIAN_POINT ( 'NONE',  ( -19.50843993236927432, -21.96177808838975665, 62.11008241541560437 ) ) ;
#11718=AXIS2_PLACEMENT_3D ( 'NONE', #25410, #2518, #48287 ) ;
#11719=CARTESIAN_POINT ( 'NONE',  ( -23.48344415125163565, -18.41350569598871090, 73.04896097104848707 ) ) ;
#11720=CARTESIAN_POINT ( 'NONE',  ( -12.79725882921341373, -20.12850138265567068, 72.10653676770067477 ) ) ;
#11722=ORIENTED_EDGE ( 'NONE', *, *, #22600, .T. ) ;
#11723=CARTESIAN_POINT ( 'NONE',  ( -17.79084007069931417, -7.768752218527304798, 60.38060768310334225 ) ) ;
#11724=CARTESIAN_POINT ( 'NONE',  ( -18.34656657831649085, -21.80233790260681204, 65.34532039249234003 ) ) ;
#11725=CARTESIAN_POINT ( 'NONE',  ( -23.04635137988585214, -19.07596084359022726, 65.96822594231640835 ) ) ;
#11726=EDGE_CURVE ( 'NONE', #35202, #313, #34221, .T. ) ;
#11727=CARTESIAN_POINT ( 'NONE',  ( -21.31115985637654120, -8.927249709250721921, 73.88656608925673197 ) ) ;
#11728=ORIENTED_EDGE ( 'NONE', *, *, #405, .T. ) ;
#11733=CARTESIAN_POINT ( 'NONE',  ( -19.00548271871079464, -7.528979306145422434, 67.05071780787497460 ) ) ;
#11734=CARTESIAN_POINT ( 'NONE',  ( -19.81920524125959560, -24.16823983354497685, 54.50428052266512680 ) ) ;
#11735=CARTESIAN_POINT ( 'NONE',  ( -11.93195840498443516, -10.38844327383712773, 70.98365212470247343 ) ) ;
#11737=EDGE_CURVE ( 'NONE', #17592, #38583, #15472, .T. ) ;
#11738=CARTESIAN_POINT ( 'NONE',  ( -10.95381465013825206, -17.48043978162002077, 68.39721944380028162 ) ) ;
#11739=ORIENTED_EDGE ( 'NONE', *, *, #17645, .F. ) ;
#11740=ORIENTED_EDGE ( 'NONE', *, *, #36457, .T. ) ;
#11741=VERTEX_POINT ( 'NONE', #21203 ) ;
#11742=CARTESIAN_POINT ( 'NONE',  ( -15.14815771252334820, -21.49015593068176244, 72.19008430323151515 ) ) ;
#11744=CARTESIAN_POINT ( 'NONE',  ( -21.21846785720043727, -20.69168585734932719, 69.06952566980361041 ) ) ;
#11747=( BOUNDED_CURVE ( )  B_SPLINE_CURVE ( 3, ( #32389, #28683, #36301, #25241 ),
 .UNSPECIFIED., .F., .F. ) 
 B_SPLINE_CURVE_WITH_KNOTS ( ( 4, 4 ),
 ( 0.9074455897393632897, 1.000000000000000000 ),
 .UNSPECIFIED. ) 
 CURVE ( )  GEOMETRIC_REPRESENTATION_ITEM ( )  RATIONAL_B_SPLINE_CURVE ( ( 0.6983129098260791867, 0.7760317562606862118, 0.8765941196519931866, 1.000000000000000000 ) ) 
 REPRESENTATION_ITEM ( '' )  );
#11748=CARTESIAN_POINT ( 'NONE',  ( -10.39923015370485260, -17.29004932004441031, 61.35017275334070064 ) ) ;
#11749=CARTESIAN_POINT ( 'NONE',  ( -14.16804751454036726, -8.612086832270765768, 74.21571240128525915 ) ) ;
#11750=CARTESIAN_POINT ( 'NONE',  ( -10.51251092892767325, -16.19956264364908449, 71.44750414188726495 ) ) ;
#11751=ORIENTED_EDGE ( 'NONE', *, *, #13012, .F. ) ;
#11752=ORIENTED_EDGE ( 'NONE', *, *, #5206, .F. ) ;
#11753=CARTESIAN_POINT ( 'NONE',  ( -12.03835690272354597, -15.98895779851376631, 53.69233794759168887 ) ) ;
#11754=CARTESIAN_POINT ( 'NONE',  ( -22.51947191901838963, -20.24425718459050572, 65.80398109777289051 ) ) ;
#11755=VECTOR ( 'NONE', #15213, 1000.000000000000114 ) ;
#11756=CARTESIAN_POINT ( 'NONE',  ( -10.50673402251998390, -15.88996810048886488, 68.20597793203801018 ) ) ;
#11757=CARTESIAN_POINT ( 'NONE',  ( -23.69928304873747038, -18.82488403301566038, 69.33726028187463442 ) ) ;
#11758=ORIENTED_EDGE ( 'NONE', *, *, #23410, .T. ) ;
#11759=( BOUNDED_SURFACE ( )  B_SPLINE_SURFACE ( 3, 1, ( 
 ( #35968, #47789 ),
 ( #6671, #24907 ),
 ( #6189, #43878 ),
 ( #7172, #32990 ),
 ( #48032, #33976 ),
 ( #44356, #14270 ),
 ( #26607, #18221 ) ),
 .UNSPECIFIED., .T., .F., .F. ) 
 B_SPLINE_SURFACE_WITH_KNOTS ( ( 4, 3, 4 ),
 ( 2, 2 ),
 ( 0.000000000000000000, 0.5000000000000000000, 1.000000000000000000 ),
 ( 0.000000000000000000, 1.000000000000000000 ),
 .UNSPECIFIED. ) 
 GEOMETRIC_REPRESENTATION_ITEM ( )  RATIONAL_B_SPLINE_SURFACE ( (
 ( 1.000000000000000000, 1.000000000000000000),
 ( 0.3333333333333335369, 0.3333333333333330373),
 ( 0.3333333333333335369, 0.3333333333333330373),
 ( 1.000000000000000000, 1.000000000000000000),
 ( 0.3333333333333333703, 0.3333333333333333703),
 ( 0.3333333333333333703, 0.3333333333333333703),
 ( 1.000000000000000000, 1.000000000000000000) ) ) 
 REPRESENTATION_ITEM ( '' )  SURFACE ( )  );
#11761=( BOUNDED_CURVE ( )  B_SPLINE_CURVE ( 3, ( #45325, #25865, #14500, #34214 ),
 .UNSPECIFIED., .F., .F. ) 
 B_SPLINE_CURVE_WITH_KNOTS ( ( 4, 4 ),
 ( 0.5000000000000000000, 0.9074455897393687298 ),
 .UNSPECIFIED. ) 
 CURVE ( )  GEOMETRIC_REPRESENTATION_ITEM ( )  RATIONAL_B_SPLINE_CURVE ( ( 1.000000000000004219, 0.4567392136813255288, 0.3561768502900249378, 0.6983129098261068313 ) ) 
 REPRESENTATION_ITEM ( '' )  );
#11763=AXIS2_PLACEMENT_3D ( 'NONE', #46793, #28328, #9623 ) ;
#11764=VERTEX_POINT ( 'NONE', #17722 ) ;
#11765=CARTESIAN_POINT ( 'NONE',  ( -16.12973315643056793, -21.68894210253334975, 58.56969077390900225 ) ) ;
#11766=CARTESIAN_POINT ( 'NONE',  ( -12.10487669921564446, -20.02548830339394925, 61.44032727821130635 ) ) ;
#11767=CARTESIAN_POINT ( 'NONE',  ( -15.26068139326780226, -21.46662260714567694, 68.57592932306751266 ) ) ;
#11770=ORIENTED_EDGE ( 'NONE', *, *, #38313, .T. ) ;
#11772=( BOUNDED_CURVE ( )  B_SPLINE_CURVE ( 3, ( #46169, #22804, #8499, #41751 ),
 .UNSPECIFIED., .F., .F. ) 
 B_SPLINE_CURVE_WITH_KNOTS ( ( 4, 4 ),
 ( 0.4074455897393650661, 0.5000000000000000000 ),
 .UNSPECIFIED. ) 
 CURVE ( )  GEOMETRIC_REPRESENTATION_ITEM ( )  RATIONAL_B_SPLINE_CURVE ( ( 0.6983129098260983936, 0.7760317562607078612, 0.8765941196520097289, 1.000000000000007772 ) ) 
 REPRESENTATION_ITEM ( '' )  );
#11773=CARTESIAN_POINT ( 'NONE',  ( -10.64854695470030599, -12.86019059820356780, 64.55364013863997741 ) ) ;
#11775=ORIENTED_EDGE ( 'NONE', *, *, #30232, .F. ) ;
#11776=CARTESIAN_POINT ( 'NONE',  ( -15.55171133418867235, -7.598245370416885969, 70.79485226425863686 ) ) ;
#11780=FACE_OUTER_BOUND ( 'NONE', #32019, .T. ) ;
#11781=ORIENTED_EDGE ( 'NONE', *, *, #36272, .T. ) ;
#11782=CARTESIAN_POINT ( 'NONE',  ( -18.18338144371267617, -21.81849904615365432, 65.63060065626805795 ) ) ;
#11783=CARTESIAN_POINT ( 'NONE',  ( -23.84607668508775902, -11.89174505508500523, 63.04398307482357922 ) ) ;
#11785=CARTESIAN_POINT ( 'NONE',  ( -24.38756562526642213, -15.91227465074931935, 66.34852784166324113 ) ) ;
#11786=CARTESIAN_POINT ( 'NONE',  ( -18.24929096724884658, -21.81104555038653103, 68.82986815895560540 ) ) ;
#11787=CARTESIAN_POINT ( 'NONE',  ( -10.96069643151774109, -18.51437482595545347, 57.92219192461608657 ) ) ;
#11788=ADVANCED_FACE ( 'NONE', ( #44114 ), #21916, .T. ) ;
#11790=ORIENTED_EDGE ( 'NONE', *, *, #29379, .T. ) ;
#11791=DIRECTION ( 'NONE',  ( -0.8705373987491421550, 0.4921022631314296847, -4.758021987662797425E-08 ) ) ;
#11792=EDGE_CURVE ( 'NONE', #5421, #37170, #6062, .T. ) ;
#11793=CARTESIAN_POINT ( 'NONE',  ( -16.27008412796014625, -7.904986034540439022, 60.20028479263386600 ) ) ;
#11794=CARTESIAN_POINT ( 'NONE',  ( -11.42427419758796603, -11.20335516203438075, 57.31789115431045190 ) ) ;
#11796=CARTESIAN_POINT ( 'NONE',  ( -17.13503149044196761, -7.764836982087094164, 70.77563787455143540 ) ) ;
#11797=AXIS2_PLACEMENT_3D ( 'NONE', #26519, #30472, #44763 ) ;
#11798=EDGE_CURVE ( 'NONE', #19293, #32931, #31440, .T. ) ;
#11799=CARTESIAN_POINT ( 'NONE',  ( -23.29054614595685635, -19.40156175341775580, 59.04557170734604199 ) ) ;
#11800=ORIENTED_EDGE ( 'NONE', *, *, #48385, .F. ) ;
#11801=VERTEX_POINT ( 'NONE', #40618 ) ;
#11803=FACE_OUTER_BOUND ( 'NONE', #24406, .T. ) ;
#11804=CARTESIAN_POINT ( 'NONE',  ( -23.42532394183187705, -19.22384306421519184, 62.46911594462533657 ) ) ;
#11808=CARTESIAN_POINT ( 'NONE',  ( -11.55573855159262386, -10.21941529800896653, 71.15388400389697665 ) ) ;
#11809=CARTESIAN_POINT ( 'NONE',  ( -23.88368001943721453, -17.64091657838220328, 66.35845829618112646 ) ) ;
#11811=ORIENTED_EDGE ( 'NONE', *, *, #32166, .T. ) ;
#11812=FACE_OUTER_BOUND ( 'NONE', #37002, .T. ) ;
#11813=CARTESIAN_POINT ( 'NONE',  ( -15.58636089855801110, -7.589425593079765164, 70.75989837095031021 ) ) ;
#11814=CARTESIAN_POINT ( 'NONE',  ( -15.09544305450467760, -21.46351983957133669, 65.40596681500470311 ) ) ;
#11816=EDGE_LOOP ( 'NONE', ( #27106, #44018, #23822, #30270, #33391 ) ) ;
#11817=EDGE_CURVE ( 'NONE', #20357, #29883, #7881, .T. ) ;
#11818=ORIENTED_EDGE ( 'NONE', *, *, #35791, .T. ) ;
#11819=EDGE_CURVE ( 'NONE', #8067, #44791, #41919, .T. ) ;
#11820=CARTESIAN_POINT ( 'NONE',  ( -19.87969377733951859, -21.36436553174173270, 69.19822862580041090 ) ) ;
#11821=CYLINDRICAL_SURFACE ( 'NONE', #42592, 0.1500000000000009104 ) ;
#11825=ADVANCED_FACE ( 'NONE', ( #26108 ), #45083, .T. ) ;
#11826=ORIENTED_EDGE ( 'NONE', *, *, #10601, .T. ) ;
#11828=CARTESIAN_POINT ( 'NONE',  ( -13.11378388673462148, -9.291622923581300597, 70.95998485332185624 ) ) ;
#11829=LINE ( 'NONE', #37661, #8419 ) ;
#11830=ORIENTED_EDGE ( 'NONE', *, *, #2708, .T. ) ;
#11831=CIRCLE ( 'NONE', #29121, 6.999999999999999112 ) ;
#11833=CARTESIAN_POINT ( 'NONE',  ( -14.01837044221388595, -8.636059239884618322, 74.48482605064899076 ) ) ;
#11836=ORIENTED_EDGE ( 'NONE', *, *, #34768, .F. ) ;
#11838=DIRECTION ( 'NONE',  ( -6.059369603295153624E-06, 3.309764060044371102E-06, 0.9999999999761648439 ) ) ;
#11840=CARTESIAN_POINT ( 'NONE',  ( -24.43112999227502513, -15.58634490091466951, 73.00303748142292193 ) ) ;
#11841=CARTESIAN_POINT ( 'NONE',  ( -10.13784000599894597, -13.25541019000276499, 74.79322239981686948 ) ) ;
#11844=B_SPLINE_CURVE_WITH_KNOTS ( 'NONE', 3,
 ( #8279, #37554, #30934, #48655, #14897, #18864, #29957, #33875, #26499, #38284 ),
 .UNSPECIFIED., .F., .F.,
 ( 4, 2, 2, 2, 4 ),
 ( 0.000000000000000000, 0.2500000000000000000, 0.5000000000000000000, 0.7500000000000000000, 1.000000000000000000 ),
 .UNSPECIFIED. ) ;
#11845=CARTESIAN_POINT ( 'NONE',  ( -17.82745659574447927, -7.820727410278355940, 60.08060779106381233 ) ) ;
#11846=( BOUNDED_CURVE ( )  B_SPLINE_CURVE ( 3, ( #10853, #44364, #10617, #40641 ),
 .UNSPECIFIED., .F., .F. ) 
 B_SPLINE_CURVE_WITH_KNOTS ( ( 4, 4 ),
 ( 0.4074455897393681747, 0.5000000000000000000 ),
 .UNSPECIFIED. ) 
 CURVE ( )  GEOMETRIC_REPRESENTATION_ITEM ( )  RATIONAL_B_SPLINE_CURVE ( ( 0.6983129098260796308, 0.7760317562606730002, 0.8765941196519756451, 0.9999999999999783507 ) ) 
 REPRESENTATION_ITEM ( '' )  );
#11847=CARTESIAN_POINT ( 'NONE',  ( -22.27236978094073550, -9.152572242100493582, 59.82897054759915534 ) ) ;
#11848=CARTESIAN_POINT ( 'NONE',  ( -13.35550429318260512, -8.568184490765622385, 57.15463139269148485 ) ) ;
#11849=ORIENTED_EDGE ( 'NONE', *, *, #23132, .T. ) ;
#11850=CARTESIAN_POINT ( 'NONE',  ( -13.55325570056783491, -20.70509005021970594, 57.93161203092463296 ) ) ;
#11854=CARTESIAN_POINT ( 'NONE',  ( -16.02413508665766528, -7.899451961642459885, 63.96451206367848386 ) ) ;
#11856=EDGE_LOOP ( 'NONE', ( #4351, #47648, #39779, #3643, #12852 ) ) ;
#11857=EDGE_CURVE ( 'NONE', #19458, #14528, #27182, .T. ) ;
#11858=CARTESIAN_POINT ( 'NONE',  ( -18.53202070066404517, -7.846807721809618386, 73.84064401782792686 ) ) ;
#11859=CARTESIAN_POINT ( 'NONE',  ( -23.94755663202570517, -8.431048274511610430, 54.44843099904676365 ) ) ;
#11861=CARTESIAN_POINT ( 'NONE',  ( -21.04510527405784970, -21.32003654990205987, 62.31460175905966992 ) ) ;
#11862=CARTESIAN_POINT ( 'NONE',  ( -15.22116837037893866, -21.50650591823945845, 68.59065000974109694 ) ) ;
#11864=CARTESIAN_POINT ( 'NONE',  ( -17.27965087796144061, -7.810258999111470146, 70.50652427083761609 ) ) ;
#11865=CARTESIAN_POINT ( 'NONE',  ( -14.22586362203780652, -8.080537296073694975, 67.30329176109222544 ) ) ;
#11866=CARTESIAN_POINT ( 'NONE',  ( -11.26201241829012822, -11.37794026804562009, 68.03353368067536167 ) ) ;
#11867=VECTOR ( 'NONE', #448, 1000.000000000000114 ) ;
#11869=CARTESIAN_POINT ( 'NONE',  ( -10.02759501504927186, -15.70053000738341709, 61.13765413890485689 ) ) ;
#11872=CARTESIAN_POINT ( 'NONE',  ( -16.45566506110110438, -21.79267588865899086, 62.04095995016087528 ) ) ;
#11874=CARTESIAN_POINT ( 'NONE',  ( -12.71689648175658149, -19.99233235212643223, 71.91726715478147014 ) ) ;
#11875=CARTESIAN_POINT ( 'NONE',  ( -23.82284107231174630, -10.99348899561931781, 73.61839243124092036 ) ) ;
#11877=ORIENTED_EDGE ( 'NONE', *, *, #34087, .F. ) ;
#11879=CARTESIAN_POINT ( 'NONE',  ( -20.16542227925740249, -21.73660035250202327, 72.44832829956453679 ) ) ;
#11880=ORIENTED_EDGE ( 'NONE', *, *, #3403, .F. ) ;
#11881=EDGE_CURVE ( 'NONE', #1976, #31856, #7223, .T. ) ;
#11882=EDGE_CURVE ( 'NONE', #24162, #15992, #24225, .T. ) ;
#11883=ADVANCED_FACE ( 'NONE', ( #33707 ), #26709, .T. ) ;
#11884=CARTESIAN_POINT ( 'NONE',  ( -21.35673258969865174, -10.96416394607318701, 54.07175714974879099 ) ) ;
#11885=B_SPLINE_CURVE_WITH_KNOTS ( 'NONE', 1,
 ( #5066, #11971 ),
 .UNSPECIFIED., .F., .F.,
 ( 2, 2 ),
 ( 0.000000000000000000, 1.000000000000000000 ),
 .UNSPECIFIED. ) ;
#11887=DIRECTION ( 'NONE',  ( -0.5497669574358330369, 0.8353180786453389128, 7.898837271846008747E-08 ) ) ;
#11888=CARTESIAN_POINT ( 'NONE',  ( -16.07923611736888603, -22.13698717359939039, 58.42552246658256365 ) ) ;
#11890=VECTOR ( 'NONE', #41582, 1000.000000000000227 ) ;
#11891=CARTESIAN_POINT ( 'NONE',  ( -13.76968405657925487, -21.30219918833402204, 72.11263056552699879 ) ) ;
#11893=ORIENTED_EDGE ( 'NONE', *, *, #1997, .T. ) ;
#11894=( BOUNDED_SURFACE ( )  B_SPLINE_SURFACE ( 3, 1, ( 
 ( #25469, #28918 ),
 ( #21051, #2335 ),
 ( #21772, #40258 ),
 ( #13152, #47639 ),
 ( #39522, #17814 ),
 ( #24989, #6522 ),
 ( #13874, #2580 ) ),
 .UNSPECIFIED., .T., .F., .F. ) 
 B_SPLINE_SURFACE_WITH_KNOTS ( ( 4, 3, 4 ),
 ( 2, 2 ),
 ( 0.000000000000000000, 0.5000000000000000000, 1.000000000000000000 ),
 ( 0.000000000000000000, 1.000000000000000000 ),
 .UNSPECIFIED. ) 
 GEOMETRIC_REPRESENTATION_ITEM ( )  RATIONAL_B_SPLINE_SURFACE ( (
 ( 1.000000000000000000, 1.000000000000000000),
 ( 0.3333333333333335369, 0.3333333333333330373),
 ( 0.3333333333333335369, 0.3333333333333330373),
 ( 1.000000000000000000, 1.000000000000000000),
 ( 0.3333333333333333703, 0.3333333333333333703),
 ( 0.3333333333333333703, 0.3333333333333333703),
 ( 1.000000000000000000, 1.000000000000000000) ) ) 
 REPRESENTATION_ITEM ( '' )  SURFACE ( )  );
#11895=CARTESIAN_POINT ( 'NONE',  ( -10.82281284296662527, -12.48008513829669575, 57.62857332801928578 ) ) ;
#11897=CARTESIAN_POINT ( 'NONE',  ( -12.25935330346987051, -20.17854375260402477, 64.98862157977991671 ) ) ;
#11899=B_SPLINE_CURVE_WITH_KNOTS ( 'NONE', 1,
 ( #40714, #26195 ),
 .UNSPECIFIED., .F., .F.,
 ( 2, 2 ),
 ( 0.000000000000000000, 1.000000000000000000 ),
 .UNSPECIFIED. ) ;
#11900=CARTESIAN_POINT ( 'NONE',  ( -11.11596100489605199, -10.84561087226838794, 57.40891979410004353 ) ) ;
#11901=CARTESIAN_POINT ( 'NONE',  ( -17.11809369177854379, -21.86054179209348192, 68.85127668957714775 ) ) ;
#11902=CARTESIAN_POINT ( 'NONE',  ( -23.42532328873747005, -19.22384396101403681, 62.46911485589509994 ) ) ;
#11903=ORIENTED_EDGE ( 'NONE', *, *, #36367, .F. ) ;
#11905=EDGE_CURVE ( 'NONE', #3501, #27387, #21392, .T. ) ;
#11907=B_SPLINE_CURVE_WITH_KNOTS ( 'NONE', 3,
 ( #12650, #24233, #31853, #38751, #1312, #45911, #12168, #38247, #39239, #5519 ),
 .UNSPECIFIED., .F., .F.,
 ( 4, 2, 2, 2, 4 ),
 ( 0.1272669073658447836, 0.2522669073463343903, 0.3772669073268239970, 0.5022669073073136037, 0.6272669072878032104 ),
 .UNSPECIFIED. ) ;
#11910=VERTEX_POINT ( 'NONE', #23643 ) ;
#11911=CARTESIAN_POINT ( 'NONE',  ( -24.38391064099431915, -14.06024038319858960, 73.42271507915008044 ) ) ;
#11912=LINE ( 'NONE', #4508, #11339 ) ;
#11913=( BOUNDED_CURVE ( )  B_SPLINE_CURVE ( 3, ( #20796, #5295, #9957, #12675 ),
 .UNSPECIFIED., .F., .F. ) 
 B_SPLINE_CURVE_WITH_KNOTS ( ( 4, 4 ),
 ( 0.9074455897393701731, 1.000000000000000000 ),
 .UNSPECIFIED. ) 
 CURVE ( )  GEOMETRIC_REPRESENTATION_ITEM ( )  RATIONAL_B_SPLINE_CURVE ( ( 0.6983129098261042778, 0.7760317562607079722, 0.8765941196520065093, 1.000000000000000000 ) ) 
 REPRESENTATION_ITEM ( '' )  );
#11914=CARTESIAN_POINT ( 'NONE',  ( -23.92296941035127844, -11.16669991615614066, 70.08549063249201083 ) ) ;
#11918=ORIENTED_EDGE ( 'NONE', *, *, #47095, .T. ) ;
#11920=CARTESIAN_POINT ( 'NONE',  ( -21.57995947450667984, -9.113990939708573435, 70.14604673427196246 ) ) ;
#11921=CARTESIAN_POINT ( 'NONE',  ( -15.75283589881223278, -7.548994832054173543, 67.32502661251716347 ) ) ;
#11922=ORIENTED_EDGE ( 'NONE', *, *, #44238, .T. ) ;
#11923=CARTESIAN_POINT ( 'NONE',  ( -24.38756562526642213, -15.91227465074931935, 66.34852784166324113 ) ) ;
#11924=CARTESIAN_POINT ( 'NONE',  ( -12.78399838166839686, -20.05042309268234391, 68.40945562133974533 ) ) ;
#11925=CARTESIAN_POINT ( 'NONE',  ( -18.62860737289870983, -7.457144689169211027, 74.09710349057253609 ) ) ;
#11926=ORIENTED_EDGE ( 'NONE', *, *, #216, .F. ) ;
#11927=DIRECTION ( 'NONE',  ( -0.6380325334150243055, 0.7700094066334552956, 2.346882832748419528E-17 ) ) ;
#11928=CYLINDRICAL_SURFACE ( 'NONE', #41446, 0.1500000000000022704 ) ;
#11929=VECTOR ( 'NONE', #23036, 1000.000000000000114 ) ;
#11930=CARTESIAN_POINT ( 'NONE',  ( -14.86627107493491984, -7.811969877679347363, 56.96504568426624360 ) ) ;
#11935=CARTESIAN_POINT ( 'NONE',  ( -17.42409385541300892, -14.80920654474439502, 77.49999999999994316 ) ) ;
#11937=CARTESIAN_POINT ( 'NONE',  ( -13.51671022627207286, -9.001178471081288990, 57.04255703468526661 ) ) ;
#11938=ORIENTED_EDGE ( 'NONE', *, *, #45775, .T. ) ;
#11939=VERTEX_POINT ( 'NONE', #5405 ) ;
#11941=EDGE_CURVE ( 'NONE', #17754, #1223, #34761, .T. ) ;
#11942=EDGE_CURVE ( 'NONE', #22030, #17855, #4251, .T. ) ;
#11943=CARTESIAN_POINT ( 'NONE',  ( -19.11145865927416310, -7.964113456900453691, 63.43089235103783352 ) ) ;
#11944=CARTESIAN_POINT ( 'NONE',  ( -10.45452924831652375, -14.15584214187167511, 60.91821260770957025 ) ) ;
#11948=ADVANCED_FACE ( 'NONE', ( #9344 ), #28038, .T. ) ;
#11949=CARTESIAN_POINT ( 'NONE',  ( -18.06139463723319949, -21.83834701327926808, 58.56120650458878174 ) ) ;
#11950=DIRECTION ( 'NONE',  ( 0.8604039311673230550, 0.5096126717731923605, -7.110477545283408869E-08 ) ) ;
#11952=ADVANCED_FACE ( 'NONE', ( #24362 ), #981, .T. ) ;
#11953=CARTESIAN_POINT ( 'NONE',  ( -19.81804402429900236, -8.174913897241847138, 73.60608030023824710 ) ) ;
#11954=CARTESIAN_POINT ( 'NONE',  ( -14.97188219925329378, -8.199429090594037461, 56.99999999999994316 ) ) ;
#11955=VERTEX_POINT ( 'NONE', #20665 ) ;
#11956=DIRECTION ( 'NONE',  ( 1.259531062780516415E-05, -2.755480461857868066E-06, 0.9999999999168828202 ) ) ;
#11957=ORIENTED_EDGE ( 'NONE', *, *, #46088, .F. ) ;
#11958=CARTESIAN_POINT ( 'NONE',  ( -23.46260449798628045, -11.17067817067885649, 73.51193301756617871 ) ) ;
#11959=CARTESIAN_POINT ( 'NONE',  ( -15.05225219112592860, -21.44840536712413126, 65.11156449207337005 ) ) ;
#11960=CARTESIAN_POINT ( 'NONE',  ( -18.71757194967216975, -7.929750632967406787, 70.37068030597254165 ) ) ;
#11961=CARTESIAN_POINT ( 'NONE',  ( -10.66160605790631344, -13.00123564105898666, 68.03832347539896830 ) ) ;
#11964=ORIENTED_EDGE ( 'NONE', *, *, #39878, .F. ) ;
#11965=CARTESIAN_POINT ( 'NONE',  ( -17.58740562021222686, -21.86528886929834670, 62.01968736857112674 ) ) ;
#11966=CARTESIAN_POINT ( 'NONE',  ( -24.69662841158067579, -16.42583212380900903, 59.22994102966119101 ) ) ;
#11969=ORIENTED_EDGE ( 'NONE', *, *, #9497, .T. ) ;
#11971=CARTESIAN_POINT ( 'NONE',  ( -23.25757785049868787, -10.17517560731475967, 63.18690593950643120 ) ) ;
#11972=CARTESIAN_POINT ( 'NONE',  ( -24.19391819315973180, -11.69922608242822726, 59.63235732785043552 ) ) ;
#11975=DIRECTION ( 'NONE',  ( 1.053901171194056067E-05, -6.708308827411335869E-06, 0.9999999999219638669 ) ) ;
#11977=CARTESIAN_POINT ( 'NONE',  ( -20.35208330028754631, -8.450993137587310855, 66.78104082230152017 ) ) ;
#11981=ORIENTED_EDGE ( 'NONE', *, *, #39347, .F. ) ;
#11982=LINE ( 'NONE', #34607, #40773 ) ;
#11983=DIRECTION ( 'NONE',  ( -5.731567514496413899E-31, -1.020425574103664789E-16, -1.000000000000000000 ) ) ;
#11985=CARTESIAN_POINT ( 'NONE',  ( -20.16518531629159838, -8.309878794262091972, 66.78104051650225870 ) ) ;
#11986=ORIENTED_EDGE ( 'NONE', *, *, #45007, .T. ) ;
#11987=ORIENTED_EDGE ( 'NONE', *, *, #39342, .F. ) ;
#11988=ORIENTED_EDGE ( 'NONE', *, *, #35107, .T. ) ;
#11989=DIRECTION ( 'NONE',  ( 2.331190576225089612E-06, -8.511884079520847478E-06, 0.9999999999610567070 ) ) ;
#11990=CARTESIAN_POINT ( 'NONE',  ( -21.94915715192368921, -8.890837417924517538, 66.76875849712446609 ) ) ;
#11992=CARTESIAN_POINT ( 'NONE',  ( -10.38655970317176802, -17.25373507390027328, 61.35754318564477927 ) ) ;
#11993=CARTESIAN_POINT ( 'NONE',  ( -13.65684165595416921, -8.849801312179289781, 56.98439896120441261 ) ) ;
#11994=CARTESIAN_POINT ( 'NONE',  ( -22.78262153964987036, -19.98509753430224833, 72.90046450679021461 ) ) ;
#11996=ORIENTED_EDGE ( 'NONE', *, *, #10619, .F. ) ;
#11997=CARTESIAN_POINT ( 'NONE',  ( -17.52853272358826686, -7.759682304905023642, 63.83584969886392457 ) ) ;
#11999=CARTESIAN_POINT ( 'NONE',  ( -10.00073915290244564, -14.17087342314384735, 64.57459177551746166 ) ) ;
#12001=CARTESIAN_POINT ( 'NONE',  ( -20.78299823145727387, -8.610459808214880439, 59.85597358678664648 ) ) ;
#12005=ORIENTED_EDGE ( 'NONE', *, *, #32649, .F. ) ;
#12006=DIRECTION ( 'NONE',  ( 0.7971031148784507581, -0.6038432116460915600, 6.916509187980650173E-08 ) ) ;
#12007=CARTESIAN_POINT ( 'NONE',  ( -15.44183219577975130, -21.52267352039123338, 68.76696128071972680 ) ) ;
#12008=ADVANCED_FACE ( 'NONE', ( #6846 ), #11027, .T. ) ;
#12010=EDGE_CURVE ( 'NONE', #48202, #6672, #18341, .T. ) ;
#12011=ORIENTED_EDGE ( 'NONE', *, *, #19343, .F. ) ;
#12013=B_SPLINE_CURVE_WITH_KNOTS ( 'NONE', 3,
 ( #48495, #18449, #37153, #14729, #36431, #48021, #18696, #44112, #14257, #33215 ),
 .UNSPECIFIED., .F., .F.,
 ( 4, 2, 2, 2, 4 ),
 ( 0.1272669073658215244, 0.2522669073463236211, 0.3772669073268256623, 0.5022669073073278145, 0.6272669072878298557 ),
 .UNSPECIFIED. ) ;
#12014=CARTESIAN_POINT ( 'NONE',  ( -11.67943375510494697, -18.89645239624664441, 68.50217487844219022 ) ) ;
#12015=CARTESIAN_POINT ( 'NONE',  ( -12.10481839165579565, -9.592984239578061789, 57.13289628414671739 ) ) ;
#12017=CARTESIAN_POINT ( 'NONE',  ( -22.53429313110963861, -9.952421254863265787, 73.78161091678163075 ) ) ;
#12020=EDGE_LOOP ( 'NONE', ( #29780, #42985, #21889, #1425, #1004 ) ) ;
#12021=FACE_OUTER_BOUND ( 'NONE', #30793, .T. ) ;
#12022=ORIENTED_EDGE ( 'NONE', *, *, #44073, .T. ) ;
#12023=LINE ( 'NONE', #8572, #651 ) ;
#12024=CARTESIAN_POINT ( 'NONE',  ( -14.91112529534803066, -8.221969756899694559, 57.13527940342243028 ) ) ;
#12025=ORIENTED_EDGE ( 'NONE', *, *, #37190, .F. ) ;
#12026=DIRECTION ( 'NONE',  ( -0.9918916210775228226, -0.1270866320121812332, 6.503929234589264523E-08 ) ) ;
#12027=LINE ( 'NONE', #27039, #24778 ) ;
#12029=ORIENTED_EDGE ( 'NONE', *, *, #1712, .F. ) ;
#12030=CARTESIAN_POINT ( 'NONE',  ( -11.28210193903344560, -11.34791643573311859, 64.15441847699383970 ) ) ;
#12031=( BOUNDED_SURFACE ( )  B_SPLINE_SURFACE ( 3, 1, ( 
 ( #27276, #42304 ),
 ( #19893, #16170 ),
 ( #46238, #12497 ),
 ( #13685, #16901 ),
 ( #39568, #29218 ),
 ( #28967, #21356 ),
 ( #25043, #24800 ) ),
 .UNSPECIFIED., .T., .F., .F. ) 
 B_SPLINE_SURFACE_WITH_KNOTS ( ( 4, 3, 4 ),
 ( 2, 2 ),
 ( 0.000000000000000000, 0.5000000000000000000, 1.000000000000000000 ),
 ( 0.000000000000000000, 1.000000000000000000 ),
 .UNSPECIFIED. ) 
 GEOMETRIC_REPRESENTATION_ITEM ( )  RATIONAL_B_SPLINE_SURFACE ( (
 ( 1.000000000000000000, 1.000000000000000000),
 ( 0.3333333333333335369, 0.3333333333333330373),
 ( 0.3333333333333335369, 0.3333333333333330373),
 ( 1.000000000000000000, 1.000000000000000000),
 ( 0.3333333333333333703, 0.3333333333333333703),
 ( 0.3333333333333333703, 0.3333333333333333703),
 ( 1.000000000000000000, 1.000000000000000000) ) ) 
 REPRESENTATION_ITEM ( '' )  SURFACE ( )  );
#12032=CARTESIAN_POINT ( 'NONE',  ( -16.41803040986462037, -7.880257286500736313, 60.31101663054752748 ) ) ;
#12033=CARTESIAN_POINT ( 'NONE',  ( -11.96084830514426400, -9.743959610980004626, 60.74413522332266524 ) ) ;
#12034=VERTEX_POINT ( 'NONE', #13243 ) ;
#12035=CARTESIAN_POINT ( 'NONE',  ( -12.86353962931362283, -9.432586330540292607, 74.33395128836551180 ) ) ;
#12036=LINE ( 'NONE', #3419, #17250 ) ;
#12037=ORIENTED_EDGE ( 'NONE', *, *, #17868, .F. ) ;
#12039=CARTESIAN_POINT ( 'NONE',  ( -24.84793640206982701, -14.18443463346696909, 69.83770693398628282 ) ) ;
#12040=CARTESIAN_POINT ( 'NONE',  ( -10.71315705494743753, -11.57408983106119216, 71.18837245568840899 ) ) ;
#12043=CARTESIAN_POINT ( 'NONE',  ( -12.40380818233537141, -19.68739593843253033, 61.69678633575567517 ) ) ;
#12045=DIRECTION ( 'NONE',  ( 6.023555219429074381E-06, -1.003033500007733605E-05, 0.9999999999315545285 ) ) ;
#12047=( BOUNDED_CURVE ( )  B_SPLINE_CURVE ( 3, ( #40084, #14186, #5870, #29241 ),
 .UNSPECIFIED., .F., .F. ) 
 B_SPLINE_CURVE_WITH_KNOTS ( ( 4, 4 ),
 ( 0.000000000000000000, 0.4074455897393628456 ),
 .UNSPECIFIED. ) 
 CURVE ( )  GEOMETRIC_REPRESENTATION_ITEM ( )  RATIONAL_B_SPLINE_CURVE ( ( 1.000000000000000000, 0.4567392136813396841, 0.3561768502900331534, 0.6983129098260804080 ) ) 
 REPRESENTATION_ITEM ( '' )  );
#12048=DIRECTION ( 'NONE',  ( 0.9904243694481096316, 0.1380563957348939774, 6.973877024228147881E-08 ) ) ;
#12049=ORIENTED_EDGE ( 'NONE', *, *, #32047, .T. ) ;
#12050=EDGE_LOOP ( 'NONE', ( #197, #37974, #31577, #2250, #48097 ) ) ;
#12051=CARTESIAN_POINT ( 'NONE',  ( -10.40651916427681023, -14.13340035957373075, 61.21821274675264846 ) ) ;
#12053=VECTOR ( 'NONE', #40468, 1000.000000000000000 ) ;
#12054=CARTESIAN_POINT ( 'NONE',  ( -10.02995815481606634, -13.89786978184575794, 57.63320425522585566 ) ) ;
#12055=ORIENTED_EDGE ( 'NONE', *, *, #2685, .T. ) ;
#12056=( BOUNDED_CURVE ( )  B_SPLINE_CURVE ( 3, ( #35610, #1887, #10257, #21091 ),
 .UNSPECIFIED., .F., .F. ) 
 B_SPLINE_CURVE_WITH_KNOTS ( ( 4, 4 ),
 ( 0.5000000000000000000, 0.9074455897393668424 ),
 .UNSPECIFIED. ) 
 CURVE ( )  GEOMETRIC_REPRESENTATION_ITEM ( )  RATIONAL_B_SPLINE_CURVE ( ( 1.000000000000003109, 0.4567392136813368531, 0.3561768502900296562, 0.6983129098260851819 ) ) 
 REPRESENTATION_ITEM ( '' )  );
#12057=ORIENTED_EDGE ( 'NONE', *, *, #24511, .F. ) ;
#12058=FACE_OUTER_BOUND ( 'NONE', #40317, .T. ) ;
#12059=CARTESIAN_POINT ( 'NONE',  ( -17.59331746709300148, -7.761237804004919916, 63.70057029381062819 ) ) ;
#12060=EDGE_CURVE ( 'NONE', #1531, #21712, #31890, .T. ) ;
#12061=CARTESIAN_POINT ( 'NONE',  ( -14.98986966776551988, -21.85036012251616810, 65.29870846104924453 ) ) ;
#12062=CARTESIAN_POINT ( 'NONE',  ( -22.94085434386056832, -9.802298134861713308, 70.19673941016031904 ) ) ;
#12063=ADVANCED_FACE ( 'NONE', ( #36618 ), #44295, .T. ) ;
#12064=ORIENTED_EDGE ( 'NONE', *, *, #9392, .T. ) ;
#12065=B_SPLINE_CURVE_WITH_KNOTS ( 'NONE', 1,
 ( #33326, #41471 ),
 .UNSPECIFIED., .F., .F.,
 ( 2, 2 ),
 ( 0.000000000000000000, 1.000000000000000000 ),
 .UNSPECIFIED. ) ;
#12066=CARTESIAN_POINT ( 'NONE',  ( -13.05823872554153908, -9.336963863356308124, 70.86542013787308747 ) ) ;
#12067=EDGE_CURVE ( 'NONE', #15704, #26298, #32698, .T. ) ;
#12068=CARTESIAN_POINT ( 'NONE',  ( -24.45288365649568618, -15.45035942066159862, 69.68874360283344060 ) ) ;
#12069=ORIENTED_EDGE ( 'NONE', *, *, #43510, .T. ) ;
#12070=CARTESIAN_POINT ( 'NONE',  ( -11.17842666812006769, -10.74653426074781848, 57.39558607234117460 ) ) ;
#12072=CARTESIAN_POINT ( 'NONE',  ( -11.08591710707173839, -18.72456284283582661, 61.42710830429783186 ) ) ;
#12073=ORIENTED_EDGE ( 'NONE', *, *, #8727, .F. ) ;
#12074=CARTESIAN_POINT ( 'NONE',  ( -12.26730668522635526, -19.62818085036556681, 65.01107574152555912 ) ) ;
#12075=EDGE_CURVE ( 'NONE', #10295, #34444, #19813, .T. ) ;
#12076=VERTEX_POINT ( 'NONE', #20902 ) ;
#12084=DIRECTION ( 'NONE',  ( -0.9729319276368276759, -0.2310918955413239773, 6.827553174175007530E-08 ) ) ;
#12085=CARTESIAN_POINT ( 'NONE',  ( -22.24151848281995214, -9.126331139912949197, 59.82147588101616265 ) ) ;
#12086=ORIENTED_EDGE ( 'NONE', *, *, #40612, .F. ) ;
#12088=DIRECTION ( 'NONE',  ( 0.8398192074808118468, 0.5428661886195297326, 7.907900705247677662E-08 ) ) ;
#12090=CARTESIAN_POINT ( 'NONE',  ( -18.38376433957202849, -21.74317146278215773, 68.83017111679792777 ) ) ;
#12095=DIRECTION ( 'NONE',  ( 0.8875028193683940358, 0.4608022847308269609, -4.020963237754318724E-08 ) ) ;
#12096=CARTESIAN_POINT ( 'NONE',  ( -12.36794907275616850, -19.72224022788673636, 61.54678633597969650 ) ) ;
#12098=CARTESIAN_POINT ( 'NONE',  ( -10.00747521095153303, -15.51449648374953050, 57.61146884931378054 ) ) ;
#12099=CARTESIAN_POINT ( 'NONE',  ( -15.47894645291934523, -21.58867816219044755, 68.46104220717563749 ) ) ;
#12101=CARTESIAN_POINT ( 'NONE',  ( -28.05267866845275293, -15.70886298607290499, 54.49999999999995026 ) ) ;
#12103=CARTESIAN_POINT ( 'NONE',  ( -14.48548941065490148, -8.400516866317895293, 67.27447142263336843 ) ) ;
#12104=CARTESIAN_POINT ( 'NONE',  ( -10.82867469351122836, -11.34449526142513598, 67.73369307302053244 ) ) ;
#12105=ORIENTED_EDGE ( 'NONE', *, *, #5632, .F. ) ;
#12106=DIRECTION ( 'NONE',  ( -5.731567514496413899E-31, -1.020425574103664789E-16, -1.000000000000000000 ) ) ;
#12107=CARTESIAN_POINT ( 'NONE',  ( -13.38462506958126319, -20.58719851387657940, 58.04650077714654088 ) ) ;
#12109=CARTESIAN_POINT ( 'NONE',  ( -12.80044372018415189, -20.06500349168936737, 72.10653684543767383 ) ) ;
#12110=CARTESIAN_POINT ( 'NONE',  ( -16.03289554736505806, -7.947204745776725865, 67.32934463618931886 ) ) ;
#12112=ORIENTED_EDGE ( 'NONE', *, *, #41587, .F. ) ;
#12116=ORIENTED_EDGE ( 'NONE', *, *, #7655, .T. ) ;
#12117=CARTESIAN_POINT ( 'NONE',  ( -12.01937617657256041, -9.681437477770858280, 60.72064570034685715 ) ) ;
#12119=CARTESIAN_POINT ( 'NONE',  ( -10.40511033146429831, -14.11732416830307280, 57.33336190745325212 ) ) ;
#12123=CARTESIAN_POINT ( 'NONE',  ( -11.23918011089898705, -11.53084126649161512, 64.22170027535517534 ) ) ;
#12124=CARTESIAN_POINT ( 'NONE',  ( -16.08649462381330864, -22.13826890709367845, 58.46398360678714567 ) ) ;
#12125=ORIENTED_EDGE ( 'NONE', *, *, #46941, .F. ) ;
#12126=EDGE_CURVE ( 'NONE', #30297, #2344, #964, .T. ) ;
#12128=EDGE_CURVE ( 'NONE', #41672, #40331, #41813, .T. ) ;
#12129=CARTESIAN_POINT ( 'NONE',  ( -19.37616744185158879, -21.99900390342548206, 58.71002665166666645 ) ) ;
#12131=FACE_OUTER_BOUND ( 'NONE', #7502, .T. ) ;
#12132=CARTESIAN_POINT ( 'NONE',  ( -13.84336496337389022, -20.88234202223394931, 68.46184952764561160 ) ) ;
#12135=CARTESIAN_POINT ( 'NONE',  ( -12.52738813637484405, -19.88632359053370990, 61.39678650461756604 ) ) ;
#12136=CARTESIAN_POINT ( 'NONE',  ( -24.00897149951030940, -12.43446728902662457, 73.43328766012302822 ) ) ;
#12138=CYLINDRICAL_SURFACE ( 'NONE', #28598, 0.1499999999999990508 ) ;
#12139=CARTESIAN_POINT ( 'NONE',  ( -17.87364429212824390, -21.79475623858289168, 58.51439479403251909 ) ) ;
#12140=EDGE_CURVE ( 'NONE', #12494, #35872, #3625, .T. ) ;
#12141=DIRECTION ( 'NONE',  ( 3.549360974554993999E-17, -6.371834667797928663E-18, -1.000000000000000000 ) ) ;
#12142=CARTESIAN_POINT ( 'NONE',  ( -24.04021708909630206, -12.36549076622675791, 73.12736853451067986 ) ) ;
#12143=CARTESIAN_POINT ( 'NONE',  ( -24.37947642869176690, -14.01903517687732759, 73.42271482001694949 ) ) ;
#12144=CARTESIAN_POINT ( 'NONE',  ( -14.60783717270099835, -21.70648693424663378, 58.35113322083577003 ) ) ;
#12145=EDGE_CURVE ( 'NONE', #38602, #3056, #48397, .T. ) ;
#12147=CARTESIAN_POINT ( 'NONE',  ( -20.88427521310116575, -20.89426873771111559, 62.12973820747942000 ) ) ;
#12148=CARTESIAN_POINT ( 'NONE',  ( -10.48723240375378829, -15.75052704102940915, 64.52388266229672809 ) ) ;
#12153=ORIENTED_EDGE ( 'NONE', *, *, #37682, .F. ) ;
#12155=CARTESIAN_POINT ( 'NONE',  ( -10.47928406297145720, -17.50635424218827296, 64.76592889887460558 ) ) ;
#12156=ORIENTED_EDGE ( 'NONE', *, *, #15217, .T. ) ;
#12157=CARTESIAN_POINT ( 'NONE',  ( -23.36565744117094923, -18.61087216430447455, 65.82389142905810786 ) ) ;
#12158=CARTESIAN_POINT ( 'NONE',  ( -10.63173029587417595, -17.86977651231121911, 71.75992364232735099 ) ) ;
#12159=CARTESIAN_POINT ( 'NONE',  ( -23.21283044961208830, -10.11939778159179859, 63.25681392212788268 ) ) ;
#12160=CARTESIAN_POINT ( 'NONE',  ( -20.03282965983824226, -21.84088468745754597, 53.89198173725360874 ) ) ;
#12162=CARTESIAN_POINT ( 'NONE',  ( -10.37599212182869124, -14.63324797960940593, 71.34254748307667171 ) ) ;
#12163=CARTESIAN_POINT ( 'NONE',  ( -24.42401643431037073, -14.84212902100172293, 59.54300237020546405 ) ) ;
#12166=CARTESIAN_POINT ( 'NONE',  ( -16.99415041099795332, -7.769321291326151346, 70.37547239324983650 ) ) ;
#12167=CARTESIAN_POINT ( 'NONE',  ( -23.69044173319201363, -11.56146079933792237, 59.63803016077844177 ) ) ;
#12168=CARTESIAN_POINT ( 'NONE',  ( -24.55128148229147911, -12.63992024488134902, 69.97254205454612475 ) ) ;
#12172=VERTEX_POINT ( 'NONE', #34089 ) ;
#12174=EDGE_CURVE ( 'NONE', #23522, #42856, #377, .T. ) ;
#12175=CARTESIAN_POINT ( 'NONE',  ( -22.75539019595754908, -10.19575032747719412, 66.82710158566565894 ) ) ;
#12176=CARTESIAN_POINT ( 'NONE',  ( -23.34903492872366115, -11.08148469299992378, 73.43481278317960914 ) ) ;
#12177=CARTESIAN_POINT ( 'NONE',  ( -16.94458633259734270, -7.374567983260779336, 74.14513688882354359 ) ) ;
#12178=( BOUNDED_CURVE ( )  B_SPLINE_CURVE ( 3, ( #23860, #35874, #28749, #43541 ),
 .UNSPECIFIED., .F., .F. ) 
 B_SPLINE_CURVE_WITH_KNOTS ( ( 4, 4 ),
 ( 0.5000000000000000000, 0.9074455897393589598 ),
 .UNSPECIFIED. ) 
 CURVE ( )  GEOMETRIC_REPRESENTATION_ITEM ( )  RATIONAL_B_SPLINE_CURVE ( ( 0.9999999999999803491, 0.4567392136813388515, 0.3561768502900464761, 0.6983129098260818513 ) ) 
 REPRESENTATION_ITEM ( '' )  );
#12181=CARTESIAN_POINT ( 'NONE',  ( -17.66159697976433307, -21.85550285805611637, 58.42025434932890704 ) ) ;
#12182=CARTESIAN_POINT ( 'NONE',  ( -15.39388989008627995, -21.97733388496078177, 72.23070757706680922 ) ) ;
#12183=CARTESIAN_POINT ( 'NONE',  ( -20.18941521006531303, -7.891347330600439136, 73.83601268700121523 ) ) ;
#12184=CARTESIAN_POINT ( 'NONE',  ( -24.76540239943457422, -16.07765717072269140, 66.17829646510101327 ) ) ;
#12185=ORIENTED_EDGE ( 'NONE', *, *, #46776, .T. ) ;
#12186=CARTESIAN_POINT ( 'NONE',  ( -22.44011750557629270, -19.69186611616677851, 69.40091412993344022 ) ) ;
#12187=( BOUNDED_SURFACE ( )  B_SPLINE_SURFACE ( 3, 1, ( 
 ( #3498, #37958 ),
 ( #4245, #33512 ),
 ( #44397, #19256 ),
 ( #48559, #46087 ),
 ( #30842, #19751 ),
 ( #27369, #1256 ),
 ( #46584, #12348 ) ),
 .UNSPECIFIED., .T., .F., .F. ) 
 B_SPLINE_SURFACE_WITH_KNOTS ( ( 4, 3, 4 ),
 ( 2, 2 ),
 ( 0.000000000000000000, 0.5000000000000000000, 1.000000000000000000 ),
 ( 0.000000000000000000, 1.000000000000000000 ),
 .UNSPECIFIED. ) 
 GEOMETRIC_REPRESENTATION_ITEM ( )  RATIONAL_B_SPLINE_SURFACE ( (
 ( 1.000000000000000000, 1.000000000000000000),
 ( 0.3333333333333335369, 0.3333333333333330373),
 ( 0.3333333333333335369, 0.3333333333333330373),
 ( 1.000000000000000000, 1.000000000000000000),
 ( 0.3333333333333333703, 0.3333333333333333703),
 ( 0.3333333333333333703, 0.3333333333333333703),
 ( 1.000000000000000000, 1.000000000000000000) ) ) 
 REPRESENTATION_ITEM ( '' )  SURFACE ( )  );
#12189=ORIENTED_EDGE ( 'NONE', *, *, #19406, .F. ) ;
#12190=CARTESIAN_POINT ( 'NONE',  ( -12.39983768287018329, -19.75505771991250725, 61.69118872147407018 ) ) ;
#12191=CARTESIAN_POINT ( 'NONE',  ( -19.46797834413568040, -22.79580085574647441, 53.49999999999995026 ) ) ;
#12192=ORIENTED_EDGE ( 'NONE', *, *, #20935, .F. ) ;
#12193=CARTESIAN_POINT ( 'NONE',  ( -18.10844610942486099, -22.22787712852580455, 65.48498797171305341 ) ) ;
#12195=DIRECTION ( 'NONE',  ( 6.291559634385637730E-07, -1.530398238691524640E-06, 0.9999999999986310950 ) ) ;
#12198=VERTEX_POINT ( 'NONE', #30426 ) ;
#12201=CARTESIAN_POINT ( 'NONE',  ( -23.34299683607928699, -18.64475395501998278, 73.17857113406003577 ) ) ;
#12202=CARTESIAN_POINT ( 'NONE',  ( -10.40860991809309155, -15.50898095412354571, 57.85320721669017985 ) ) ;
#12205=CARTESIAN_POINT ( 'NONE',  ( -11.38872272660762164, -18.35547376437386191, 57.80714557486621885 ) ) ;
#12209=CARTESIAN_POINT ( 'NONE',  ( -12.05483428091225129, -10.31798718066989551, 67.49896870046983111 ) ) ;
#12210=ORIENTED_EDGE ( 'NONE', *, *, #17983, .F. ) ;
#12212=EDGE_LOOP ( 'NONE', ( #24017, #27100 ) ) ;
#12214=AXIS2_PLACEMENT_3D ( 'NONE', #19128, #48674, #34135 ) ;
#12215=ADVANCED_FACE ( 'NONE', ( #38024 ), #46559, .T. ) ;
#12217=FACE_BOUND ( 'NONE', #9329, .T. ) ;
#12218=VERTEX_POINT ( 'NONE', #17314 ) ;
#12220=ORIENTED_EDGE ( 'NONE', *, *, #14116, .F. ) ;
#12222=CYLINDRICAL_SURFACE ( 'NONE', #36708, 0.1499999999999963030 ) ;
#12224=CARTESIAN_POINT ( 'NONE',  ( -16.50454646563301964, -22.20232569423288282, 65.34069100801451668 ) ) ;
#12227=CARTESIAN_POINT ( 'NONE',  ( -19.43397249051689357, -8.102278120859530475, 60.07166125860918271 ) ) ;
#12229=ORIENTED_EDGE ( 'NONE', *, *, #33788, .F. ) ;
#12231=EDGE_CURVE ( 'NONE', #26697, #25255, #29524, .T. ) ;
#12232=CARTESIAN_POINT ( 'NONE',  ( -10.39679176622870038, -14.24023819782134304, 64.40275955115841100 ) ) ;
#12233=FACE_OUTER_BOUND ( 'NONE', #19216, .T. ) ;
#12237=VERTEX_POINT ( 'NONE', #20055 ) ;
#12238=DIRECTION ( 'NONE',  ( -3.840742979682813137E-07, 4.934726756126598837E-06, -0.9999999999877504653 ) ) ;
#12239=CARTESIAN_POINT ( 'NONE',  ( -15.29809632361469873, -21.47854941203162937, 68.57592918283285144 ) ) ;
#12240=CARTESIAN_POINT ( 'NONE',  ( -17.39761456938454742, -7.809256627251312644, 67.32039592144390383 ) ) ;
#12241=EDGE_LOOP ( 'NONE', ( #37015, #46072, #45398, #27348, #40729 ) ) ;
#12242=CARTESIAN_POINT ( 'NONE',  ( -11.63855245876247935, -18.75048069921609439, 68.23306329961977212 ) ) ;
#12243=B_SPLINE_CURVE_WITH_KNOTS ( 'NONE', 3,
 ( #43622, #24667, #25143, #36437, #2719, #17726, #32754, #47781, #14020, #9882 ),
 .UNSPECIFIED., .F., .F.,
 ( 4, 2, 2, 2, 4 ),
 ( 0.000000000000000000, 0.2500000000000000000, 0.5000000000000000000, 0.7500000000000000000, 1.000000000000000000 ),
 .UNSPECIFIED. ) ;
#12245=FACE_OUTER_BOUND ( 'NONE', #11664, .T. ) ;
#12248=CARTESIAN_POINT ( 'NONE',  ( -10.44551236293470353, -15.36195525749487345, 57.58409439150996434 ) ) ;
#12251=ORIENTED_EDGE ( 'NONE', *, *, #42481, .T. ) ;
#12252=DIRECTION ( 'NONE',  ( 2.200805972648249745E-07, 3.006001593475220059E-06, 0.9999999999954577445 ) ) ;
#12253=ORIENTED_EDGE ( 'NONE', *, *, #33662, .F. ) ;
#12254=CARTESIAN_POINT ( 'NONE',  ( -9.975237612755753602, -14.67793925367211116, 71.42808438716600961 ) ) ;
#12255=CARTESIAN_POINT ( 'NONE',  ( -22.04114742393716142, -9.481025248639417313, 59.73643293354757589 ) ) ;
#12258=CYLINDRICAL_SURFACE ( 'NONE', #14001, 0.1500000000000038802 ) ;
#12259=CARTESIAN_POINT ( 'NONE',  ( -23.81768783790253252, -11.95822662118994373, 59.49852322759251422 ) ) ;
#12262=CARTESIAN_POINT ( 'NONE',  ( -9.990623027812100432, -14.31192454061599229, 64.57299275950818185 ) ) ;
#12263=CARTESIAN_POINT ( 'NONE',  ( -15.13554010266625482, -21.89904150877020328, 68.76931220517136012 ) ) ;
#12264=CARTESIAN_POINT ( 'NONE',  ( -19.65950609550678152, -21.49557518541719148, 65.75926423743261751 ) ) ;
#12265=CARTESIAN_POINT ( 'NONE',  ( -10.89657400502345830, -17.34179108361152544, 68.28648913934780751 ) ) ;
#12266=ORIENTED_EDGE ( 'NONE', *, *, #23913, .T. ) ;
#12267=CARTESIAN_POINT ( 'NONE',  ( -16.07630405233268434, -7.886179812623181462, 67.55496168274575552 ) ) ;
#12268=EDGE_CURVE ( 'NONE', #34163, #48033, #19497, .T. ) ;
#12269=EDGE_CURVE ( 'NONE', #18224, #36615, #31864, .T. ) ;
#12272=EDGE_LOOP ( 'NONE', ( #41893, #13881 ) ) ;
#12273=EDGE_CURVE ( 'NONE', #14369, #14223, #11306, .T. ) ;
#12274=CARTESIAN_POINT ( 'NONE',  ( -24.85298803532284850, -14.24811622150979673, 69.76001114652854085 ) ) ;
#12278=EDGE_CURVE ( 'NONE', #43778, #40803, #24001, .T. ) ;
#12280=CARTESIAN_POINT ( 'NONE',  ( -12.20309422964675150, -20.12380354524033521, 64.98179449731530610 ) ) ;
#12281=CARTESIAN_POINT ( 'NONE',  ( -9.974806312911359996, -14.91297370499342989, 74.89755268075251138 ) ) ;
#12282=AXIS2_PLACEMENT_3D ( 'NONE', #8634, #38898, #37924 ) ;
#12285=ORIENTED_EDGE ( 'NONE', *, *, #33187, .T. ) ;
#12286=CARTESIAN_POINT ( 'NONE',  ( -21.94239175829699207, -20.22099772874085488, 59.06442899522711087 ) ) ;
#12288=CARTESIAN_POINT ( 'NONE',  ( -13.82689732469268229, -20.87277619789260186, 68.47097268802275494 ) ) ;
#12289=CARTESIAN_POINT ( 'NONE',  ( -19.61601503992405071, -21.50980213996393786, 65.76486213821364402 ) ) ;
#12290=CARTESIAN_POINT ( 'NONE',  ( -18.76558392140857023, -7.480892851696864021, 70.55563303198719893 ) ) ;
#12292=ORIENTED_EDGE ( 'NONE', *, *, #23675, .F. ) ;
#12293=DIRECTION ( 'NONE',  ( 1.371992797150048625E-08, -1.272593384837864910E-06, 0.9999999999991900923 ) ) ;
#12294=CARTESIAN_POINT ( 'NONE',  ( -23.56879427660422266, -11.34691063241640130, 73.77682139093690239 ) ) ;
#12297=VERTEX_POINT ( 'NONE', #5040 ) ;
#12298=CARTESIAN_POINT ( 'NONE',  ( -10.52991759648590531, -16.02177972226642311, 68.27767831073917648 ) ) ;
#12301=CARTESIAN_POINT ( 'NONE',  ( -11.63929734443426867, -10.76555703936739938, 57.35336384308645563 ) ) ;
#12302=( BOUNDED_CURVE ( )  B_SPLINE_CURVE ( 3, ( #13585, #37196, #14530, #32790 ),
 .UNSPECIFIED., .F., .F. ) 
 B_SPLINE_CURVE_WITH_KNOTS ( ( 4, 4 ),
 ( 0.9074455897393730597, 1.000000000000000000 ),
 .UNSPECIFIED. ) 
 CURVE ( )  GEOMETRIC_REPRESENTATION_ITEM ( )  RATIONAL_B_SPLINE_CURVE ( ( 0.6983129098261336987, 0.7760317562607332853, 0.8765941196520220524, 1.000000000000000000 ) ) 
 REPRESENTATION_ITEM ( '' )  );
#12303=DIRECTION ( 'NONE',  ( 5.888300609747748832E-06, 9.662809622277729834E-06, -0.9999999999359791003 ) ) ;
#12305=ORIENTED_EDGE ( 'NONE', *, *, #28308, .T. ) ;
#12306=CARTESIAN_POINT ( 'NONE',  ( -20.33799833967064075, -7.952690384846734517, 70.35076722350379441 ) ) ;
#12307=AXIS2_PLACEMENT_3D ( 'NONE', #16444, #46260, #20646 ) ;
#12308=AXIS2_PLACEMENT_3D ( 'NONE', #45316, #46038, #8619 ) ;
#12309=ORIENTED_EDGE ( 'NONE', *, *, #15457, .T. ) ;
#12310=DIRECTION ( 'NONE',  ( 1.143861049860740968E-05, -2.837703139598260652E-06, 0.9999999999305527743 ) ) ;
#12311=CARTESIAN_POINT ( 'NONE',  ( -11.06572510127579356, -10.92528991087847068, 57.32247810849851533 ) ) ;
#12312=ORIENTED_EDGE ( 'NONE', *, *, #42830, .T. ) ;
#12313=CARTESIAN_POINT ( 'NONE',  ( -24.46828707212341669, -14.45681828193256280, 70.06763959435293998 ) ) ;
#12314=EDGE_CURVE ( 'NONE', #22864, #7039, #9223, .T. ) ;
#12315=CARTESIAN_POINT ( 'NONE',  ( -10.28038339137012258, -12.69496154482620121, 64.46824888007303400 ) ) ;
#12317=CARTESIAN_POINT ( 'NONE',  ( -12.02400249370662522, -10.35258068100519324, 71.15820205995147774 ) ) ;
#12319=CARTESIAN_POINT ( 'NONE',  ( -22.21277271144190379, -9.101880927996923276, 59.88204583602121289 ) ) ;
#12320=DIRECTION ( 'NONE',  ( -0.3303050442826436228, 0.9438742382973701606, 3.829623549872328137E-09 ) ) ;
#12321=ORIENTED_EDGE ( 'NONE', *, *, #34830, .T. ) ;
#12324=CARTESIAN_POINT ( 'NONE',  ( -10.76216126260078987, -17.12512740823429525, 65.04228012599854480 ) ) ;
#12326=CARTESIAN_POINT ( 'NONE',  ( -12.96596342764269139, -9.347744029417796696, 71.14925352873375175 ) ) ;
#12327=FACE_OUTER_BOUND ( 'NONE', #39644, .T. ) ;
#12328=VERTEX_POINT ( 'NONE', #5281 ) ;
#12329=ORIENTED_EDGE ( 'NONE', *, *, #48471, .T. ) ;
#12331=B_SPLINE_CURVE_WITH_KNOTS ( 'NONE', 3,
 ( #18593, #41505, #10504, #3346, #29949, #18351, #22551, #7305, #3096, #3585 ),
 .UNSPECIFIED., .F., .F.,
 ( 4, 2, 2, 2, 4 ),
 ( 0.1272669073657954342, 0.2522669073488127967, 0.3772669073318302146, 0.5022669073148475771, 0.6272669072978649396 ),
 .UNSPECIFIED. ) ;
#12332=CARTESIAN_POINT ( 'NONE',  ( -21.33694466872984918, -9.004932385753821933, 73.90128753631783809 ) ) ;
#12333=ORIENTED_EDGE ( 'NONE', *, *, #12145, .F. ) ;
#12336=CARTESIAN_POINT ( 'NONE',  ( -20.73950801051994119, -8.137571121906521654, 63.41147264556233409 ) ) ;
#12337=EDGE_CURVE ( 'NONE', #4669, #31415, #43392, .T. ) ;
#12338=CARTESIAN_POINT ( 'NONE',  ( -19.60046790782316251, -21.46228069541063732, 65.46486213989528835 ) ) ;
#12339=CARTESIAN_POINT ( 'NONE',  ( -14.73037927113499812, -8.285490617698924254, 67.40407820626249702 ) ) ;
#12340=CARTESIAN_POINT ( 'NONE',  ( -12.21223302309773651, -10.13625172099550475, 60.75021366515743182 ) ) ;
#12341=CARTESIAN_POINT ( 'NONE',  ( -20.49170831689750472, -8.461258797198503601, 63.59649424907593129 ) ) ;
#12342=( BOUNDED_CURVE ( )  B_SPLINE_CURVE ( 3, ( #41496, #23282, #45701, #7785 ),
 .UNSPECIFIED., .F., .F. ) 
 B_SPLINE_CURVE_WITH_KNOTS ( ( 4, 4 ),
 ( 0.5000000000000000000, 0.9074455897393670645 ),
 .UNSPECIFIED. ) 
 CURVE ( )  GEOMETRIC_REPRESENTATION_ITEM ( )  RATIONAL_B_SPLINE_CURVE ( ( 1.000000000000019540, 0.4567392136813334114, 0.3561768502900171107, 0.6983129098260917322 ) ) 
 REPRESENTATION_ITEM ( '' )  );
#12343=VERTEX_POINT ( 'NONE', #43198 ) ;
#12345=CARTESIAN_POINT ( 'NONE',  ( -22.47245519635065492, -19.73066437834766873, 72.65872596779033188 ) ) ;
#12346=CARTESIAN_POINT ( 'NONE',  ( -22.96375064570672819, -10.44813988596692411, 63.08658113699938497 ) ) ;
#12348=CARTESIAN_POINT ( 'NONE',  ( -11.82099749022622426, -9.899105802180386604, 64.21409645106085406 ) ) ;
#12353=CARTESIAN_POINT ( 'NONE',  ( -20.03518388220226143, -21.78744935781895009, 72.59133997248245862 ) ) ;
#12354=ORIENTED_EDGE ( 'NONE', *, *, #40281, .F. ) ;
#12356=CARTESIAN_POINT ( 'NONE',  ( -18.50846021547567233, -7.843058547566564620, 74.14064372603324671 ) ) ;
#12357=AXIS2_PLACEMENT_3D ( 'NONE', #41249, #48383, #11956 ) ;
#12358=EDGE_LOOP ( 'NONE', ( #33894, #21089 ) ) ;
#12360=CARTESIAN_POINT ( 'NONE',  ( -18.30911350570762153, -7.811336752399037131, 74.04884132303362776 ) ) ;
#12362=CARTESIAN_POINT ( 'NONE',  ( -15.94320239998165967, -7.507703417504081322, 63.80864474281522547 ) ) ;
#12363=CARTESIAN_POINT ( 'NONE',  ( -23.82261068186806696, -17.64831283868447542, 62.77360983446511966 ) ) ;
#12366=EDGE_CURVE ( 'NONE', #15929, #42340, #33281, .T. ) ;
#12367=CARTESIAN_POINT ( 'NONE',  ( -23.59327504554355315, -11.39630409041826020, 69.90682860766239060 ) ) ;
#12369=LINE ( 'NONE', #26675, #20535 ) ;
#12370=CARTESIAN_POINT ( 'NONE',  ( -16.71219989829967645, -22.22520177033091926, 68.81065352759269160 ) ) ;
#12373=CARTESIAN_POINT ( 'NONE',  ( -10.45994342254983778, -13.68936021814239012, 57.54005269860393668 ) ) ;
#12374=CARTESIAN_POINT ( 'NONE',  ( -14.25068859620041017, -8.513811488652077486, 70.72957628655862550 ) ) ;
#12376=CARTESIAN_POINT ( 'NONE',  ( -10.49754805884589004, -17.55449835891870691, 68.28377192865846723 ) ) ;
#12377=CARTESIAN_POINT ( 'NONE',  ( -24.36823009493971171, -13.92613870693967293, 73.19559539736981435 ) ) ;
#12378=DIRECTION ( 'NONE',  ( 1.261798975490001659E-05, -2.391811517362266964E-06, 0.9999999999175328558 ) ) ;
#12380=VECTOR ( 'NONE', #219, 1000.000000000000114 ) ;
#12381=FACE_OUTER_BOUND ( 'NONE', #29272, .T. ) ;
#12383=CARTESIAN_POINT ( 'NONE',  ( -22.23351441301664622, -19.96811234597608120, 69.58906588434240348 ) ) ;
#12385=VERTEX_POINT ( 'NONE', #29135 ) ;
#12387=CARTESIAN_POINT ( 'NONE',  ( -14.03276184351355127, -20.98997801200527391, 71.92607724353423748 ) ) ;
#12388=CARTESIAN_POINT ( 'NONE',  ( -24.28316357868862241, -16.20676250134670582, 59.23218348001186939 ) ) ;
#12391=CARTESIAN_POINT ( 'NONE',  ( -10.77430091989677408, -12.46723135102848090, 57.62297568056796848 ) ) ;
#12394=CARTESIAN_POINT ( 'NONE',  ( -24.34138173484706158, -16.17068648017255583, 62.59328676670276792 ) ) ;
#12396=CARTESIAN_POINT ( 'NONE',  ( -24.40668608927523309, -14.31499747486667573, 66.25580842628600919 ) ) ;
#12397=DIRECTION ( 'NONE',  ( -1.006957036272130273E-05, 6.253991260048532259E-06, 0.9999999999297456421 ) ) ;
#12398=EDGE_CURVE ( 'NONE', #40297, #3376, #29873, .T. ) ;
#12399=CARTESIAN_POINT ( 'NONE',  ( -16.55451525393793233, -12.46531383050667863, 47.99999999999994316 ) ) ;
#12400=ORIENTED_EDGE ( 'NONE', *, *, #2359, .F. ) ;
#12402=EDGE_CURVE ( 'NONE', #35636, #18401, #28316, .T. ) ;
#12405=CARTESIAN_POINT ( 'NONE',  ( -24.46479343890040425, -14.44719913075708995, 66.48292729247951627 ) ) ;
#12406=CARTESIAN_POINT ( 'NONE',  ( -22.78678303852979425, -9.565966637465477262, 53.49999999999994316 ) ) ;
#12408=VERTEX_POINT ( 'NONE', #6731 ) ;
#12410=CARTESIAN_POINT ( 'NONE',  ( -22.94085434386056832, -9.802298134861713308, 70.19673941016031904 ) ) ;
#12412=CARTESIAN_POINT ( 'NONE',  ( -14.03870967672415304, -8.172720116890397790, 70.91453050697840865 ) ) ;
#12413=EDGE_CURVE ( 'NONE', #36713, #11687, #26568, .T. ) ;
#12418=EDGE_CURVE ( 'NONE', #36238, #2574, #6972, .T. ) ;
#12419=CARTESIAN_POINT ( 'NONE',  ( -17.72634068467203505, -21.85272461955047874, 58.70553378267869249 ) ) ;
#12420=CARTESIAN_POINT ( 'NONE',  ( -17.16915267636370146, -4.372400222636961153, 54.49999999999995026 ) ) ;
#12423=ORIENTED_EDGE ( 'NONE', *, *, #14551, .T. ) ;
#12424=CARTESIAN_POINT ( 'NONE',  ( -22.39933173914730702, -19.73341662423927190, 69.18920472232342433 ) ) ;
#12425=VECTOR ( 'NONE', #299, 1000.000000000000114 ) ;
#12426=CARTESIAN_POINT ( 'NONE',  ( -24.26711730922272281, -13.09851334671752632, 59.57087637770133171 ) ) ;
#12427=ORIENTED_EDGE ( 'NONE', *, *, #3044, .F. ) ;
#12428=CARTESIAN_POINT ( 'NONE',  ( -12.38457195078649598, -19.73934731251468477, 61.69678635356166296 ) ) ;
#12429=CARTESIAN_POINT ( 'NONE',  ( -20.35208293893518672, -8.450992964911224092, 67.08104082230126153 ) ) ;
#12430=VERTEX_POINT ( 'NONE', #25206 ) ;
#12432=CARTESIAN_POINT ( 'NONE',  ( -21.94239013569476171, -20.22099906679998327, 58.76442899523448204 ) ) ;
#12433=CARTESIAN_POINT ( 'NONE',  ( -24.03160971261424805, -17.26750559640275640, 69.71339792588547368 ) ) ;
#12434=CARTESIAN_POINT ( 'NONE',  ( -19.30272045617997634, -8.014115550771091279, 59.96092997145632353 ) ) ;
#12436=CARTESIAN_POINT ( 'NONE',  ( -10.33271527364436082, -17.09297260451290867, 57.79422236154066184 ) ) ;
#12437=CARTESIAN_POINT ( 'NONE',  ( -17.75585263246644985, -22.25182633040162372, 58.50529758609160069 ) ) ;
#12439=CARTESIAN_POINT ( 'NONE',  ( -18.37786432726835883, -21.79469297182707521, 69.10042588711679912 ) ) ;
#12442=DIRECTION ( 'NONE',  ( -6.919810407550069512E-06, -1.067025350021132924E-05, 0.9999999999191310218 ) ) ;
#12446=VERTEX_POINT ( 'NONE', #36985 ) ;
#12449=CARTESIAN_POINT ( 'NONE',  ( -13.14999064602648637, -9.265557826385967033, 67.37942786034257381 ) ) ;
#12450=ORIENTED_EDGE ( 'NONE', *, *, #13071, .F. ) ;
#12451=CARTESIAN_POINT ( 'NONE',  ( -19.97164249076357478, -21.81019033462135326, 69.11977790463622284 ) ) ;
#12453=FACE_BOUND ( 'NONE', #8399, .T. ) ;
#12456=ORIENTED_EDGE ( 'NONE', *, *, #12549, .T. ) ;
#12459=CARTESIAN_POINT ( 'NONE',  ( -11.60006209888454443, -10.16330164164447325, 71.08397698276321819 ) ) ;
#12460=( BOUNDED_CURVE ( )  B_SPLINE_CURVE ( 3, ( #33481, #17743, #44603, #14040 ),
 .UNSPECIFIED., .F., .F. ) 
 B_SPLINE_CURVE_WITH_KNOTS ( ( 4, 4 ),
 ( 0.5000000000000000000, 0.9074455897393702841 ),
 .UNSPECIFIED. ) 
 CURVE ( )  GEOMETRIC_REPRESENTATION_ITEM ( )  RATIONAL_B_SPLINE_CURVE ( ( 1.000000000000006661, 0.4567392136813283043, 0.3561768502900239941, 0.6983129098261012802 ) ) 
 REPRESENTATION_ITEM ( '' )  );
#12461=CARTESIAN_POINT ( 'NONE',  ( -21.27276468869498416, -8.962107285475900298, 73.61631126181501372 ) ) ;
#12462=CARTESIAN_POINT ( 'NONE',  ( -10.61641583932764910, -11.78277314028518319, 74.74335662173743344 ) ) ;
#12463=CARTESIAN_POINT ( 'NONE',  ( -16.32745258320347759, -21.77369344365219561, 61.77040269689842944 ) ) ;
#12465=ORIENTED_EDGE ( 'NONE', *, *, #40310, .F. ) ;
#12467=LINE ( 'NONE', #38568, #17321 ) ;
#12468=CYLINDRICAL_SURFACE ( 'NONE', #26813, 0.1499999999999998834 ) ;
#12469=CARTESIAN_POINT ( 'NONE',  ( -17.42409385541300892, -14.80920654474439324, 56.49999999999994316 ) ) ;
#12470=VERTEX_POINT ( 'NONE', #44648 ) ;
#12472=( BOUNDED_CURVE ( )  B_SPLINE_CURVE ( 3, ( #46735, #13208, #9069, #20635 ),
 .UNSPECIFIED., .F., .F. ) 
 B_SPLINE_CURVE_WITH_KNOTS ( ( 4, 4 ),
 ( 0.9074455897393662873, 1.000000000000000000 ),
 .UNSPECIFIED. ) 
 CURVE ( )  GEOMETRIC_REPRESENTATION_ITEM ( )  RATIONAL_B_SPLINE_CURVE ( ( 0.6983129098260957290, 0.7760317562607005337, 0.8765941196520019574, 1.000000000000000000 ) ) 
 REPRESENTATION_ITEM ( '' )  );
#12474=EDGE_LOOP ( 'NONE', ( #14443, #45831, #45823, #8018 ) ) ;
#12475=EDGE_CURVE ( 'NONE', #43128, #17100, #10910, .T. ) ;
#12476=EDGE_CURVE ( 'NONE', #28650, #44593, #40090, .T. ) ;
#12477=CARTESIAN_POINT ( 'NONE',  ( -14.80056147340629380, -21.78207226143426922, 61.82095877133116346 ) ) ;
#12480=FACE_OUTER_BOUND ( 'NONE', #18505, .T. ) ;
#12482=ORIENTED_EDGE ( 'NONE', *, *, #37278, .F. ) ;
#12483=CARTESIAN_POINT ( 'NONE',  ( -15.39388989008627995, -21.97733388496078177, 72.23070757706680922 ) ) ;
#12485=VECTOR ( 'NONE', #38704, 999.9999999999998863 ) ;
#12487=CARTESIAN_POINT ( 'NONE',  ( -23.78676187654788521, -10.93361199230012559, 73.54688693628270357 ) ) ;
#12488=CARTESIAN_POINT ( 'NONE',  ( -22.83578998848691199, -19.92954559311242235, 72.76587817586035101 ) ) ;
#12489=ORIENTED_EDGE ( 'NONE', *, *, #39975, .T. ) ;
#12490=VECTOR ( 'NONE', #45947, 1000.000000000000114 ) ;
#12493=CARTESIAN_POINT ( 'NONE',  ( -20.10953249554714262, -7.859859036490854045, 73.88130001012858372 ) ) ;
#12494=VERTEX_POINT ( 'NONE', #22476 ) ;
#12496=VERTEX_POINT ( 'NONE', #26661 ) ;
#12497=CARTESIAN_POINT ( 'NONE',  ( -14.99555751708010121, -21.85235056220836469, 65.14950770721691242 ) ) ;
#12499=EDGE_LOOP ( 'NONE', ( #21277, #24710, #45320, #24050, #45063 ) ) ;
#12500=CARTESIAN_POINT ( 'NONE',  ( -16.18802525292456096, -21.75305063948447426, 62.17057002965735535 ) ) ;
#12501=CARTESIAN_POINT ( 'NONE',  ( -10.81170448216924740, -12.36318809540519048, 57.34329390664808557 ) ) ;
#12502=EDGE_CURVE ( 'NONE', #14825, #39482, #15799, .T. ) ;
#12503=CARTESIAN_POINT ( 'NONE',  ( -10.56492483649129710, -13.18000429128331774, 71.50828586225090078 ) ) ;
#12504=FACE_OUTER_BOUND ( 'NONE', #31192, .T. ) ;
#12505=VERTEX_POINT ( 'NONE', #557 ) ;
#12506=CARTESIAN_POINT ( 'NONE',  ( -24.21013527259002629, -17.88545513683227384, 59.11723130990997532 ) ) ;
#12507=CARTESIAN_POINT ( 'NONE',  ( -20.64758772760614036, -8.594144261551539543, 63.53951371574645179 ) ) ;
#12509=CARTESIAN_POINT ( 'NONE',  ( -22.28399030946148329, -9.162456282157330989, 59.84454312193096825 ) ) ;
#12512=CARTESIAN_POINT ( 'NONE',  ( -24.72860576188992709, -16.27458831476113943, 62.78667002183767210 ) ) ;
#12513=VERTEX_POINT ( 'NONE', #27142 ) ;
#12514=ORIENTED_EDGE ( 'NONE', *, *, #21062, .T. ) ;
#12515=CARTESIAN_POINT ( 'NONE',  ( -13.01482893870565682, -8.804038099563683772, 63.95300575187839343 ) ) ;
#12516=EDGE_CURVE ( 'NONE', #1995, #8331, #14430, .T. ) ;
#12517=CARTESIAN_POINT ( 'NONE',  ( -11.03161394367693049, -18.63672047605813376, 57.92059234540772650 ) ) ;
#12519=CARTESIAN_POINT ( 'NONE',  ( -12.35460334350678480, -9.982084953531975557, 57.16223665588471192 ) ) ;
#12521=CARTESIAN_POINT ( 'NONE',  ( -23.30282330091471366, -18.60927750845715067, 69.29371984660140527 ) ) ;
#12524=VERTEX_POINT ( 'NONE', #23455 ) ;
#12525=ORIENTED_EDGE ( 'NONE', *, *, #1771, .T. ) ;
#12526=CARTESIAN_POINT ( 'NONE',  ( -10.64577699202231287, -11.71757285455929853, 74.67344842241411129 ) ) ;
#12529=VECTOR ( 'NONE', #3797, 1000.000000000000114 ) ;
#12530=FACE_OUTER_BOUND ( 'NONE', #13264, .T. ) ;
#12532=EDGE_LOOP ( 'NONE', ( #15736, #18352, #18717, #31507, #18919 ) ) ;
#12533=EDGE_CURVE ( 'NONE', #6805, #21796, #45379, .T. ) ;
#12534=ADVANCED_FACE ( 'NONE', ( #18775 ), #4018, .F. ) ;
#12536=FACE_OUTER_BOUND ( 'NONE', #38813, .T. ) ;
#12538=CARTESIAN_POINT ( 'NONE',  ( -15.79779810604033408, -7.538871719435400465, 67.34018486351625654 ) ) ;
#12539=ORIENTED_EDGE ( 'NONE', *, *, #47400, .T. ) ;
#12540=CARTESIAN_POINT ( 'NONE',  ( -13.10125976363765332, -9.301846226610548385, 71.07755262771341620 ) ) ;
#12542=EDGE_CURVE ( 'NONE', #15202, #48304, #41260, .T. ) ;
#12545=EDGE_CURVE ( 'NONE', #37822, #48265, #21313, .T. ) ;
#12547=( BOUNDED_CURVE ( )  B_SPLINE_CURVE ( 3, ( #23922, #47296, #39415, #20468 ),
 .UNSPECIFIED., .F., .F. ) 
 B_SPLINE_CURVE_WITH_KNOTS ( ( 4, 4 ),
 ( 0.5000000000000000000, 0.9074455897393658432 ),
 .UNSPECIFIED. ) 
 CURVE ( )  GEOMETRIC_REPRESENTATION_ITEM ( )  RATIONAL_B_SPLINE_CURVE ( ( 0.9999999999999861222, 0.4567392136813359649, 0.3561768502900413691, 0.6983129098260872913 ) ) 
 REPRESENTATION_ITEM ( '' )  );
#12548=CARTESIAN_POINT ( 'NONE',  ( -11.14029015952437263, -10.80702246001832023, 57.46549161190092292 ) ) ;
#12549=EDGE_CURVE ( 'NONE', #36492, #300, #11317, .T. ) ;
#12554=ORIENTED_EDGE ( 'NONE', *, *, #40667, .T. ) ;
#12555=DIRECTION ( 'NONE',  ( -0.2466764125338440639, -0.9690979039805150963, 7.162324212089591066E-08 ) ) ;
#12556=CARTESIAN_POINT ( 'NONE',  ( -21.08681864223905578, -8.776014225774568800, 73.75695571861821520 ) ) ;
#12558=CARTESIAN_POINT ( 'NONE',  ( -24.26499744607890818, -17.75976858747020160, 62.65856309191605789 ) ) ;
#12559=CYLINDRICAL_SURFACE ( 'NONE', #24246, 0.1499999999999964140 ) ;
#12562=CARTESIAN_POINT ( 'NONE',  ( -24.06787342886325121, -18.28917680027896608, 54.27966884056654351 ) ) ;
#12563=AXIS2_PLACEMENT_3D ( 'NONE', #3181, #37137, #48478 ) ;
#12564=B_SPLINE_CURVE_WITH_KNOTS ( 'NONE', 3,
 ( #25172, #29838, #22201, #10869, #14048, #13813, #29342, #18484, #37188, #48053 ),
 .UNSPECIFIED., .F., .F.,
 ( 4, 2, 2, 2, 4 ),
 ( 0.000000000000000000, 0.2500000000000000000, 0.5000000000000000000, 0.7500000000000000000, 1.000000000000000000 ),
 .UNSPECIFIED. ) ;
#12565=CARTESIAN_POINT ( 'NONE',  ( -10.62638924718675248, -11.76062588693173794, 74.75828993396721955 ) ) ;
#12566=PLANE ( 'NONE',  #47069 ) ;
#12570=CARTESIAN_POINT ( 'NONE',  ( -14.98927377128279304, -8.246306944878789125, 56.49999999999994316 ) ) ;
#12571=CARTESIAN_POINT ( 'NONE',  ( -24.61022370753789090, -12.84395140709443162, 66.40272499809746876 ) ) ;
#12572=CARTESIAN_POINT ( 'NONE',  ( -20.69990174146486694, -20.99685511590434217, 62.34301292963910157 ) ) ;
#12574=VERTEX_POINT ( 'NONE', #28105 ) ;
#12575=DIRECTION ( 'NONE',  ( -0.8875028193683940358, -0.4608022847308269609, 4.020963237607658939E-08 ) ) ;
#12576=DIRECTION ( 'NONE',  ( 0.6621635203543605463, 0.7493593746073505812, 2.316976118889565779E-08 ) ) ;
#12577=ORIENTED_EDGE ( 'NONE', *, *, #13609, .T. ) ;
#12578=CARTESIAN_POINT ( 'NONE',  ( -22.58763249286555208, -20.18056880150341215, 65.81766459098905386 ) ) ;
#12579=DIRECTION ( 'NONE',  ( 2.403795750412638671E-06, 2.069898558110202305E-06, 0.9999999999949686913 ) ) ;
#12581=CARTESIAN_POINT ( 'NONE',  ( -10.42462062184586635, -14.89508117765250361, 75.09778901762284420 ) ) ;
#12582=CARTESIAN_POINT ( 'NONE',  ( -10.63483670088760924, -17.87674068094334245, 71.75213521449022380 ) ) ;
#12583=CARTESIAN_POINT ( 'NONE',  ( -10.89237721494850142, -17.47219765205588615, 71.86718162093610829 ) ) ;
#12585=CARTESIAN_POINT ( 'NONE',  ( -22.65122241358830024, -10.07311426451252956, 66.75002127378915873 ) ) ;
#12587=AXIS2_PLACEMENT_3D ( 'NONE', #30745, #5612, #12252 ) ;
#12588=CARTESIAN_POINT ( 'NONE',  ( -12.27729925481933471, -9.991218852276041673, 60.55918086709623083 ) ) ;
#12589=CARTESIAN_POINT ( 'NONE',  ( -12.56076107774658723, -9.694232635630330108, 74.47489936300191005 ) ) ;
#12590=ADVANCED_FACE ( 'NONE', ( #23942 ), #38705, .T. ) ;
#12595=EDGE_CURVE ( 'NONE', #37558, #44222, #1769, .T. ) ;
#12597=CARTESIAN_POINT ( 'NONE',  ( -24.07263600646086132, -12.61902678358097063, 69.88128981831194153 ) ) ;
#12598=VECTOR ( 'NONE', #21734, 1000.000000000000114 ) ;
#12599=( BOUNDED_SURFACE ( )  B_SPLINE_SURFACE ( 3, 1, ( 
 ( #4160, #26072 ),
 ( #41827, #33668 ),
 ( #19159, #34167 ),
 ( #15693, #8101 ),
 ( #48711, #37365 ),
 ( #4384, #38104 ),
 ( #30510, #34405 ) ),
 .UNSPECIFIED., .T., .F., .F. ) 
 B_SPLINE_SURFACE_WITH_KNOTS ( ( 4, 3, 4 ),
 ( 2, 2 ),
 ( 0.000000000000000000, 0.5000000000000000000, 1.000000000000000000 ),
 ( 0.000000000000000000, 1.000000000000000000 ),
 .UNSPECIFIED. ) 
 GEOMETRIC_REPRESENTATION_ITEM ( )  RATIONAL_B_SPLINE_SURFACE ( (
 ( 1.000000000000000000, 1.000000000000000000),
 ( 0.3333333333333335369, 0.3333333333333330373),
 ( 0.3333333333333335369, 0.3333333333333330373),
 ( 1.000000000000000000, 1.000000000000000000),
 ( 0.3333333333333333703, 0.3333333333333333703),
 ( 0.3333333333333333703, 0.3333333333333333703),
 ( 1.000000000000000000, 1.000000000000000000) ) ) 
 REPRESENTATION_ITEM ( '' )  SURFACE ( )  );
#12602=FACE_OUTER_BOUND ( 'NONE', #22502, .T. ) ;
#12606=CARTESIAN_POINT ( 'NONE',  ( -10.63794491530182640, -17.88370890602386609, 71.74435113740163672 ) ) ;
#12608=EDGE_CURVE ( 'NONE', #39039, #7306, #38858, .T. ) ;
#12609=EDGE_LOOP ( 'NONE', ( #968, #42057 ) ) ;
#12611=( BOUNDED_CURVE ( )  B_SPLINE_CURVE ( 3, ( #1747, #24155, #35941, #38921 ),
 .UNSPECIFIED., .F., .F. ) 
 B_SPLINE_CURVE_WITH_KNOTS ( ( 4, 4 ),
 ( 0.4074455897393705062, 0.5000000000000000000 ),
 .UNSPECIFIED. ) 
 CURVE ( )  GEOMETRIC_REPRESENTATION_ITEM ( )  RATIONAL_B_SPLINE_CURVE ( ( 0.6983129098261044998, 0.7760317562607099706, 0.8765941196520091738, 1.000000000000003109 ) ) 
 REPRESENTATION_ITEM ( '' )  );
#12612=CARTESIAN_POINT ( 'NONE',  ( -10.58350140945814744, -13.32355762376674768, 71.43501841499802651 ) ) ;
#12613=ORIENTED_EDGE ( 'NONE', *, *, #39616, .T. ) ;
#12614=CYLINDRICAL_SURFACE ( 'NONE', #75, 0.1499999999999973577 ) ;
#12615=CARTESIAN_POINT ( 'NONE',  ( -16.45013838383832550, -21.79965580723203189, 68.83993634381745608 ) ) ;
#12616=CARTESIAN_POINT ( 'NONE',  ( -19.42896739221782809, -21.56812523091048206, 62.29503644570711174 ) ) ;
#12619=CARTESIAN_POINT ( 'NONE',  ( -22.27985548098255109, -20.46033401586769429, 58.87787560672637710 ) ) ;
#12620=AXIS2_PLACEMENT_3D ( 'NONE', #28964, #6568, #36565 ) ;
#12621=EDGE_CURVE ( 'NONE', #17138, #3477, #4405, .T. ) ;
#12622=CARTESIAN_POINT ( 'NONE',  ( -14.53530919737752924, -21.67646582726403182, 58.34430615535840303 ) ) ;
#12627=( BOUNDED_CURVE ( )  B_SPLINE_CURVE ( 3, ( #22581, #37577, #1133, #46452 ),
 .UNSPECIFIED., .F., .F. ) 
 B_SPLINE_CURVE_WITH_KNOTS ( ( 4, 4 ),
 ( 0.5000000000000000000, 0.9074455897393668424 ),
 .UNSPECIFIED. ) 
 CURVE ( )  GEOMETRIC_REPRESENTATION_ITEM ( )  RATIONAL_B_SPLINE_CURVE ( ( 0.9999999999999977796, 0.4567392136813193115, 0.3561768502900270472, 0.6983129098261184886 ) ) 
 REPRESENTATION_ITEM ( '' )  );
#12632=VERTEX_POINT ( 'NONE', #31318 ) ;
#12633=CARTESIAN_POINT ( 'NONE',  ( -10.42544315765747420, -13.95862937692757555, 57.74265221125428837 ) ) ;
#12635=EDGE_LOOP ( 'NONE', ( #41031, #30639, #13782, #30137, #40673 ) ) ;
#12636=FACE_OUTER_BOUND ( 'NONE', #40251, .T. ) ;
#12637=CARTESIAN_POINT ( 'NONE',  ( -15.01040879766030223, -21.85754770930110880, 65.24450189717120452 ) ) ;
#12639=CARTESIAN_POINT ( 'NONE',  ( -16.17130706675677132, -22.15324536104840547, 58.46302426628946591 ) ) ;
#12640=CARTESIAN_POINT ( 'NONE',  ( -22.62394951084894146, -10.04809318868971424, 70.29706442286226320 ) ) ;
#12641=CARTESIAN_POINT ( 'NONE',  ( -21.31115985637654120, -8.927249709250720144, 73.88656608925673197 ) ) ;
#12642=ORIENTED_EDGE ( 'NONE', *, *, #21237, .T. ) ;
#12643=CARTESIAN_POINT ( 'NONE',  ( -13.35550429318260512, -8.568184490765622385, 57.15463139269148485 ) ) ;
#12645=CARTESIAN_POINT ( 'NONE',  ( -12.23301264461619553, -10.03852782535897958, 60.84446034103241630 ) ) ;
#12646=EDGE_LOOP ( 'NONE', ( #10970, #34606 ) ) ;
#12648=CARTESIAN_POINT ( 'NONE',  ( -18.52137898189696230, -22.17812618198155761, 72.42477605357316861 ) ) ;
#12649=CARTESIAN_POINT ( 'NONE',  ( -23.85748962928175132, -11.92509172808648543, 59.49707787073156595 ) ) ;
#12650=CARTESIAN_POINT ( 'NONE',  ( -24.55871722839809834, -12.66422925090921225, 69.88747596251579353 ) ) ;
#12651=ADVANCED_FACE ( 'NONE', ( #12602 ), #3094, .T. ) ;
#12652=CARTESIAN_POINT ( 'NONE',  ( -21.73098984888145679, -8.730191469543168381, 70.31627926275058371 ) ) ;
#12654=ORIENTED_EDGE ( 'NONE', *, *, #45154, .T. ) ;
#12655=VERTEX_POINT ( 'NONE', #35002 ) ;
#12657=VECTOR ( 'NONE', #13721, 1000.000000000000000 ) ;
#12658=CARTESIAN_POINT ( 'NONE',  ( -24.40658449907487793, -15.78251210865724907, 69.53307488410803217 ) ) ;
#12659=CARTESIAN_POINT ( 'NONE',  ( -17.72612443559818018, -7.765381109175947927, 60.36588690973874094 ) ) ;
#12661=CARTESIAN_POINT ( 'NONE',  ( -24.31561971792381982, -17.63961254754600816, 66.12169969450457074 ) ) ;
#12662=ORIENTED_EDGE ( 'NONE', *, *, #44201, .F. ) ;
#12665=FACE_OUTER_BOUND ( 'NONE', #504, .T. ) ;
#12667=EDGE_LOOP ( 'NONE', ( #45907, #38084, #17334, #7349, #19064 ) ) ;
#12668=CARTESIAN_POINT ( 'NONE',  ( -24.21013527259002629, -17.88545513683227384, 59.11723130990997532 ) ) ;
#12669=CARTESIAN_POINT ( 'NONE',  ( -17.15681863660994821, -7.812702811906586220, 74.07091344620687323 ) ) ;
#12670=ORIENTED_EDGE ( 'NONE', *, *, #37212, .F. ) ;
#12671=EDGE_CURVE ( 'NONE', #16961, #8530, #36730, .T. ) ;
#12672=CARTESIAN_POINT ( 'NONE',  ( -13.35819042472069107, -21.05197888995676436, 61.70141705377209007 ) ) ;
#12673=CARTESIAN_POINT ( 'NONE',  ( -15.03427660820159772, -21.44211488324610571, 65.12068745241758450 ) ) ;
#12675=CARTESIAN_POINT ( 'NONE',  ( -10.50893933415051507, -13.43540278197273885, 74.96345540680638919 ) ) ;
#12677=DIRECTION ( 'NONE',  ( -0.9710973231077276724, 0.2386838684389876730, -7.431671637556418335E-08 ) ) ;
#12678=ADVANCED_FACE ( 'NONE', ( #39672 ), #8160, .T. ) ;
#12680=CARTESIAN_POINT ( 'NONE',  ( -21.78783678618839303, -8.770877803870156697, 70.38778484029896276 ) ) ;
#12681=CARTESIAN_POINT ( 'NONE',  ( -22.50978241177926975, -19.61935080069436665, 72.64400553400905380 ) ) ;
#12682=ORIENTED_EDGE ( 'NONE', *, *, #28776, .F. ) ;
#12683=CARTESIAN_POINT ( 'NONE',  ( -10.31595651221557830, -17.04027680973078063, 57.79486398785477519 ) ) ;
#12685=CARTESIAN_POINT ( 'NONE',  ( -23.73684003905821527, -18.76684476618103403, 72.95023626440647035 ) ) ;
#12686=FACE_BOUND ( 'NONE', #32713, .T. ) ;
#12689=CARTESIAN_POINT ( 'NONE',  ( -24.39763799706551950, -15.84669482609578317, 69.54779622430706354 ) ) ;
#12691=DIRECTION ( 'NONE',  ( 0.02400335114476204179, -0.9997118780597843424, -1.529429985666831130E-10 ) ) ;
#12692=ORIENTED_EDGE ( 'NONE', *, *, #34781, .F. ) ;
#12693=CARTESIAN_POINT ( 'NONE',  ( -10.67763251680271175, -12.94209746246583492, 64.34124149314979491 ) ) ;
#12694=ORIENTED_EDGE ( 'NONE', *, *, #34274, .T. ) ;
#12695=B_SPLINE_CURVE_WITH_KNOTS ( 'NONE', 3,
 ( #5060, #38531, #35800, #16841, #42241, #46423, #27936, #31644, #35072, #20069 ),
 .UNSPECIFIED., .F., .F.,
 ( 4, 2, 2, 2, 4 ),
 ( 0.6272669072877483654, 0.7522669073072711932, 0.8772669073267939099, 1.002266907346316627, 1.127266907365839455 ),
 .UNSPECIFIED. ) ;
#12696=CARTESIAN_POINT ( 'NONE',  ( -11.14372862008015019, -11.71776470779160917, 67.80967772160084905 ) ) ;
#12697=CARTESIAN_POINT ( 'NONE',  ( -22.88419851978063591, -10.42888047092867865, 63.07185995612697837 ) ) ;
#12699=AXIS2_PLACEMENT_3D ( 'NONE', #29685, #19328, #3837 ) ;
#12700=CARTESIAN_POINT ( 'NONE',  ( -15.28291166272247992, -21.52618791248891128, 68.87592918174580348 ) ) ;
#12701=EDGE_CURVE ( 'NONE', #26903, #48665, #40626, .T. ) ;
#12702=FACE_BOUND ( 'NONE', #37905, .T. ) ;
#12703=VERTEX_POINT ( 'NONE', #29072 ) ;
#12704=ORIENTED_EDGE ( 'NONE', *, *, #11049, .F. ) ;
#12706=CARTESIAN_POINT ( 'NONE',  ( -17.91610874870965020, -22.24302035646641684, 62.13181838639658139 ) ) ;
#12707=CIRCLE ( 'NONE', #25296, 0.4000000000000006883 ) ;
#12708=CARTESIAN_POINT ( 'NONE',  ( -23.16117746674104438, -18.90708040007733359, 62.63934749780565880 ) ) ;
#12712=CARTESIAN_POINT ( 'NONE',  ( -10.75331705403316818, -16.93070056221711184, 57.98760548944069626 ) ) ;
#12713=ORIENTED_EDGE ( 'NONE', *, *, #8010, .F. ) ;
#12714=ORIENTED_EDGE ( 'NONE', *, *, #47249, .T. ) ;
#12716=VECTOR ( 'NONE', #29638, 1000.000000000000000 ) ;
#12719=DIRECTION ( 'NONE',  ( -2.209513405570979834E-06, 7.769005115158032304E-07, 0.9999999999972571940 ) ) ;
#12721=EDGE_CURVE ( 'NONE', #16722, #30190, #25340, .T. ) ;
#12725=CARTESIAN_POINT ( 'NONE',  ( -16.55627334167764175, -21.80933031065637806, 68.99560815001524361 ) ) ;
#12727=PLANE ( 'NONE',  #22087 ) ;
#12729=B_SPLINE_CURVE_WITH_KNOTS ( 'NONE', 3,
 ( #10616, #32539, #28610, #17740, #17508, #7180, #36937, #14277, #44135, #6918 ),
 .UNSPECIFIED., .F., .F.,
 ( 4, 2, 2, 2, 4 ),
 ( 0.1272669073658429240, 0.2522669073463211231, 0.3772669073267993500, 0.5022669073072775214, 0.6272669072877556928 ),
 .UNSPECIFIED. ) ;
#12730=FACE_OUTER_BOUND ( 'NONE', #29878, .T. ) ;
#12731=ADVANCED_FACE ( 'NONE', ( #6906 ), #2720, .T. ) ;
#12732=CARTESIAN_POINT ( 'NONE',  ( -10.65715545825994681, -16.81507633650918976, 61.30175972107676330 ) ) ;
#12733=CARTESIAN_POINT ( 'NONE',  ( -10.42608517478068109, -14.63970064516040637, 68.08473508565809595 ) ) ;
#12737=CARTESIAN_POINT ( 'NONE',  ( -12.23220206747518013, -19.57856285391799034, 58.22682373937800548 ) ) ;
#12738=CARTESIAN_POINT ( 'NONE',  ( -19.22781571947377444, -4.195962512586791426, 54.61912878955446615 ) ) ;
#12740=VERTEX_POINT ( 'NONE', #28597 ) ;
#12747=CARTESIAN_POINT ( 'NONE',  ( -20.19838274129777389, -21.29432534982823810, 72.61298750797109847 ) ) ;
#12748=CARTESIAN_POINT ( 'NONE',  ( -14.22441497990486958, -8.081217732231424478, 67.44470516081543110 ) ) ;
#12749=DIRECTION ( 'NONE',  ( -5.104528445087193737E-07, -5.317498825627977299E-07, -0.9999999999997284394 ) ) ;
#12750=ORIENTED_EDGE ( 'NONE', *, *, #4935, .F. ) ;
#12751=CARTESIAN_POINT ( 'NONE',  ( -23.83080496556880945, -17.75212211224490133, 59.28906343887996400 ) ) ;
#12752=CARTESIAN_POINT ( 'NONE',  ( -20.66207812730969096, -8.601311705287542964, 63.50048569590220637 ) ) ;
#12753=( BOUNDED_CURVE ( )  B_SPLINE_CURVE ( 3, ( #22621, #36882, #232, #30020 ),
 .UNSPECIFIED., .F., .F. ) 
 B_SPLINE_CURVE_WITH_KNOTS ( ( 4, 4 ),
 ( 0.4074455897393681747, 0.5000000000000000000 ),
 .UNSPECIFIED. ) 
 CURVE ( )  GEOMETRIC_REPRESENTATION_ITEM ( )  RATIONAL_B_SPLINE_CURVE ( ( 0.6983129098261053880, 0.7760317562607254027, 0.8765941196520283807, 1.000000000000026201 ) ) 
 REPRESENTATION_ITEM ( '' )  );
#12754=CARTESIAN_POINT ( 'NONE',  ( -23.85820194903862657, -17.69173191509663567, 62.48833042115954584 ) ) ;
#12755=EDGE_CURVE ( 'NONE', #13527, #32027, #43087, .T. ) ;
#12758=ADVANCED_FACE ( 'NONE', ( #44351 ), #29872, .T. ) ;
#12759=CARTESIAN_POINT ( 'NONE',  ( -24.72421832269116138, -16.29687976975823460, 62.75475226558750563 ) ) ;
#12763=ORIENTED_EDGE ( 'NONE', *, *, #35430, .T. ) ;
#12764=CARTESIAN_POINT ( 'NONE',  ( -23.65513889391139557, -11.50482878637529716, 62.83729622335476961 ) ) ;
#12765=CARTESIAN_POINT ( 'NONE',  ( -20.00855069579964862, -21.31476573450181888, 72.70478738568573362 ) ) ;
#12768=CARTESIAN_POINT ( 'NONE',  ( -12.39491807234433551, -9.940094850350357447, 57.37470223362350907 ) ) ;
#12770=CARTESIAN_POINT ( 'NONE',  ( -24.27033198218900978, -13.12649362337911718, 62.83264177274070050 ) ) ;
#12771=( BOUNDED_CURVE ( )  B_SPLINE_CURVE ( 3, ( #32351, #6716, #39723, #17546 ),
 .UNSPECIFIED., .F., .F. ) 
 B_SPLINE_CURVE_WITH_KNOTS ( ( 4, 4 ),
 ( 0.9074455897393625126, 1.000000000000000000 ),
 .UNSPECIFIED. ) 
 CURVE ( )  GEOMETRIC_REPRESENTATION_ITEM ( )  RATIONAL_B_SPLINE_CURVE ( ( 0.6983129098260738576, 0.7760317562606816599, 0.8765941196519904111, 1.000000000000000000 ) ) 
 REPRESENTATION_ITEM ( '' )  );
#12772=CARTESIAN_POINT ( 'NONE',  ( -13.88634980723361778, -21.36569984987395188, 72.03269384293926691 ) ) ;
#12773=ORIENTED_EDGE ( 'NONE', *, *, #25234, .T. ) ;
#12774=ORIENTED_EDGE ( 'NONE', *, *, #28829, .F. ) ;
#12775=CARTESIAN_POINT ( 'NONE',  ( -10.96024275427387984, -11.10349598290784989, 60.79230391164892211 ) ) ;
#12777=DIRECTION ( 'NONE',  ( 0.3636930986378153485, 0.9315188296557532777, -1.850371886801397451E-09 ) ) ;
#12780=ADVANCED_FACE ( 'NONE', ( #7408 ), #7658, .F. ) ;
#12782=CARTESIAN_POINT ( 'NONE',  ( -14.91623309787384066, -21.82459129695467581, 65.26743172979871588 ) ) ;
#12784=VERTEX_POINT ( 'NONE', #48504 ) ;
#12785=CARTESIAN_POINT ( 'NONE',  ( -24.81734138798520561, -15.73308575106217511, 69.64652101300646336 ) ) ;
#12786=ORIENTED_EDGE ( 'NONE', *, *, #7105, .F. ) ;
#12787=CARTESIAN_POINT ( 'NONE',  ( -22.63063519912030941, -20.13802011715040052, 69.35230721051679836 ) ) ;
#12789=ORIENTED_EDGE ( 'NONE', *, *, #45645, .F. ) ;
#12791=ORIENTED_EDGE ( 'NONE', *, *, #13134, .F. ) ;
#12792=DIRECTION ( 'NONE',  ( -0.9893874368562762811, 0.1453014101478983522, -3.604276813338691349E-17 ) ) ;
#12793=CARTESIAN_POINT ( 'NONE',  ( -18.60463909989377385, -22.16515503909319307, 72.32864992405023941 ) ) ;
#12794=ORIENTED_EDGE ( 'NONE', *, *, #35644, .T. ) ;
#12795=CARTESIAN_POINT ( 'NONE',  ( -15.18638434861223452, -8.119849305256630956, 57.14999999999947278 ) ) ;
#12798=EDGE_LOOP ( 'NONE', ( #42476, #38044, #20992, #10821, #16314, #48407, #43343 ) ) ;
#12799=CARTESIAN_POINT ( 'NONE',  ( -17.82745577869553699, -7.820727362736762167, 60.38060779106270104 ) ) ;
#12800=CARTESIAN_POINT ( 'NONE',  ( -19.24035349434955577, -7.583912967164861740, 63.68735177183580021 ) ) ;
#12801=CARTESIAN_POINT ( 'NONE',  ( -16.45566506110110083, -21.79267588865899086, 62.04095995016087528 ) ) ;
#12803=CARTESIAN_POINT ( 'NONE',  ( -24.10584571748465521, -12.56049761727124370, 73.39225570139795707 ) ) ;
#12805=CARTESIAN_POINT ( 'NONE',  ( -23.46260370332431933, -11.17067683354235719, 73.66193301755811262 ) ) ;
#12807=CARTESIAN_POINT ( 'NONE',  ( -12.26730668522635526, -19.62818085036556681, 65.01107574152555912 ) ) ;
#12808=ADVANCED_FACE ( 'NONE', ( #11573 ), #23260, .T. ) ;
#12809=EDGE_CURVE ( 'NONE', #40331, #3004, #9457, .T. ) ;
#12810=VECTOR ( 'NONE', #26971, 1000.000000000000000 ) ;
#12811=VERTEX_POINT ( 'NONE', #4428 ) ;
#12812=ORIENTED_EDGE ( 'NONE', *, *, #3325, .T. ) ;
#12814=CARTESIAN_POINT ( 'NONE',  ( -21.46381135070672386, -20.59674881067212127, 69.21017043924877044 ) ) ;
#12815=ORIENTED_EDGE ( 'NONE', *, *, #41804, .T. ) ;
#12816=CARTESIAN_POINT ( 'NONE',  ( -24.34865124180699070, -15.83455620839685452, 66.13612870751769890 ) ) ;
#12817=DIRECTION ( 'NONE',  ( 0.6478992145799702396, -0.7617260713318518839, 1.927832152310587483E-08 ) ) ;
#12820=CARTESIAN_POINT ( 'NONE',  ( -11.12219343327886811, -17.98741664779230121, 71.72285496256920112 ) ) ;
#12821=CARTESIAN_POINT ( 'NONE',  ( -10.95917937052863422, -17.62195967018737619, 71.58190244267143498 ) ) ;
#12822=ORIENTED_EDGE ( 'NONE', *, *, #37535, .T. ) ;
#12823=ADVANCED_FACE ( 'NONE', ( #41619 ), #19447, .T. ) ;
#12824=EDGE_CURVE ( 'NONE', #28108, #22354, #11829, .T. ) ;
#12825=B_SPLINE_CURVE_WITH_KNOTS ( 'NONE', 3,
 ( #25151, #47791, #18223, #28835, #10847, #36215, #25870, #32992, #6913, #10610 ),
 .UNSPECIFIED., .F., .F.,
 ( 4, 2, 2, 2, 4 ),
 ( 0.000000000000000000, 0.2500000000000000000, 0.5000000000000000000, 0.7500000000000000000, 1.000000000000000000 ),
 .UNSPECIFIED. ) ;
#12826=CARTESIAN_POINT ( 'NONE',  ( -22.58588533274201282, -20.18224782263116523, 69.36073240021890740 ) ) ;
#12827=CARTESIAN_POINT ( 'NONE',  ( -19.17437844398820346, -7.979623566120205957, 63.44561363416070776 ) ) ;
#12828=CARTESIAN_POINT ( 'NONE',  ( -23.21283114448125673, -10.11939864774917908, 63.25681283445349123 ) ) ;
#12829=CARTESIAN_POINT ( 'NONE',  ( -12.58002129225892674, -9.148929240056048684, 74.43427715830415536 ) ) ;
#12830=CARTESIAN_POINT ( 'NONE',  ( -21.46447785953442278, -9.092825438250168091, 70.13132491419585790 ) ) ;
#12831=EDGE_LOOP ( 'NONE', ( #3775, #10472, #39736, #35678 ) ) ;
#12832=VERTEX_POINT ( 'NONE', #15000 ) ;
#12834=EDGE_CURVE ( 'NONE', #24853, #18111, #34883, .T. ) ;
#12836=CARTESIAN_POINT ( 'NONE',  ( -20.03075563493810307, -21.35977203713853712, 72.69918973885827995 ) ) ;
#12837=ORIENTED_EDGE ( 'NONE', *, *, #270, .T. ) ;
#12838=CARTESIAN_POINT ( 'NONE',  ( -10.43656091707388534, -14.37069178587375973, 67.92970350560246118 ) ) ;
#12839=CARTESIAN_POINT ( 'NONE',  ( -22.68978555823764864, -10.11602685316156780, 73.57341092052691067 ) ) ;
#12841=ORIENTED_EDGE ( 'NONE', *, *, #824, .T. ) ;
#12842=CARTESIAN_POINT ( 'NONE',  ( -14.65765131015531253, -21.78034674156931061, 54.27966884056655061 ) ) ;
#12843=CARTESIAN_POINT ( 'NONE',  ( -19.43748438392636402, -21.56872497219108098, 58.41018533341049590 ) ) ;
#12844=EDGE_LOOP ( 'NONE', ( #39490, #5323, #4930, #47671, #30927 ) ) ;
#12846=EDGE_LOOP ( 'NONE', ( #23529, #16590, #1528, #26762, #40975 ) ) ;
#12847=CARTESIAN_POINT ( 'NONE',  ( -23.56138404952065812, -11.33988834032952830, 70.19210750372964469 ) ) ;
#12851=CARTESIAN_POINT ( 'NONE',  ( -18.91460061187875397, -21.70800071742875303, 58.66940498489888256 ) ) ;
#12852=ORIENTED_EDGE ( 'NONE', *, *, #7906, .F. ) ;
#12853=CARTESIAN_POINT ( 'NONE',  ( -24.40658499505740053, -15.78250870199476807, 69.83307488408829045 ) ) ;
#12856=CARTESIAN_POINT ( 'NONE',  ( -16.20683845212634111, -21.70255763714999020, 58.58585572420326315 ) ) ;
#12857=CARTESIAN_POINT ( 'NONE',  ( -10.45529269445903253, -15.48619349139875467, 61.14862166396536480 ) ) ;
#12858=CARTESIAN_POINT ( 'NONE',  ( -10.40174263535760524, -17.29725023780839166, 61.34238537770443855 ) ) ;
#12859=ORIENTED_EDGE ( 'NONE', *, *, #18273, .F. ) ;
#12861=CARTESIAN_POINT ( 'NONE',  ( -11.97490362423377164, -10.33561459433851404, 67.78424783647008667 ) ) ;
#12862=CARTESIAN_POINT ( 'NONE',  ( -23.04402284766838349, -19.06632961612601918, 59.16938527523783620 ) ) ;
#12864=CARTESIAN_POINT ( 'NONE',  ( -14.19711780326422712, -21.02108897209633298, 72.15280992966681595 ) ) ;
#12866=EDGE_CURVE ( 'NONE', #5991, #47078, #11337, .T. ) ;
#12867=EDGE_LOOP ( 'NONE', ( #4455, #6325, #13111, #22762, #16008 ) ) ;
#12868=CARTESIAN_POINT ( 'NONE',  ( -10.43125849979191955, -13.91324152291312366, 57.74825034919034294 ) ) ;
#12869=DIRECTION ( 'NONE',  ( 0.7224352045700187519, 0.6914386272098739239, -9.340627245513716657E-09 ) ) ;
#12870=ORIENTED_EDGE ( 'NONE', *, *, #20609, .F. ) ;
#12871=B_SPLINE_CURVE_WITH_KNOTS ( 'NONE', 3,
 ( #55, #23194, #41166, #15526, #15284, #22456, #4465, #37703, #26155, #15778 ),
 .UNSPECIFIED., .F., .F.,
 ( 4, 2, 2, 2, 4 ),
 ( 0.6272669072877858909, 0.7522669073072849599, 0.8772669073267839179, 1.002266907346282876, 1.127266907365781945 ),
 .UNSPECIFIED. ) ;
#12872=CARTESIAN_POINT ( 'NONE',  ( -24.42668993457695592, -13.99045928592870780, 73.40799407547365263 ) ) ;
#12873=CARTESIAN_POINT ( 'NONE',  ( -10.64203103149789698, -13.07586850037579040, 67.75334752786112347 ) ) ;
#12874=CARTESIAN_POINT ( 'NONE',  ( -23.03380641475053281, -9.905658051014942345, 66.65526928932193584 ) ) ;
#12875=CARTESIAN_POINT ( 'NONE',  ( -23.21760288594795441, -10.12534664246260441, 63.26460134184395656 ) ) ;
#12876=CARTESIAN_POINT ( 'NONE',  ( -16.91855014848012928, -22.24212009645463439, 72.28047803099305213 ) ) ;
#12879=EDGE_CURVE ( 'NONE', #2353, #41372, #45378, .T. ) ;
#12880=CARTESIAN_POINT ( 'NONE',  ( -19.05927265761716072, -8.002745927047119068, 63.43089191541108107 ) ) ;
#12881=VERTEX_POINT ( 'NONE', #11366 ) ;
#12882=AXIS2_PLACEMENT_3D ( 'NONE', #41945, #42187, #12378 ) ;
#12883=CARTESIAN_POINT ( 'NONE',  ( -18.52160066619603995, -22.17809164712859271, 72.44657480731611088 ) ) ;
#12884=EDGE_CURVE ( 'NONE', #12524, #3450, #39635, .T. ) ;
#12885=EDGE_CURVE ( 'NONE', #11741, #39260, #39918, .T. ) ;
#12886=CARTESIAN_POINT ( 'NONE',  ( -23.46018882259003036, -11.26354882964838033, 73.37809979709153652 ) ) ;
#12887=CARTESIAN_POINT ( 'NONE',  ( -10.37497030826117417, -14.69804335084345581, 71.32782692816427073 ) ) ;
#12888=( BOUNDED_SURFACE ( )  B_SPLINE_SURFACE ( 3, 1, ( 
 ( #2061, #20051 ),
 ( #43443, #13121 ),
 ( #16335, #31374 ),
 ( #27919, #5530 ),
 ( #24729, #31130 ),
 ( #42468, #24492 ),
 ( #13369, #39731 ) ),
 .UNSPECIFIED., .T., .F., .F. ) 
 B_SPLINE_SURFACE_WITH_KNOTS ( ( 4, 3, 4 ),
 ( 2, 2 ),
 ( 0.000000000000000000, 0.5000000000000000000, 1.000000000000000000 ),
 ( 0.000000000000000000, 1.000000000000000000 ),
 .UNSPECIFIED. ) 
 GEOMETRIC_REPRESENTATION_ITEM ( )  RATIONAL_B_SPLINE_SURFACE ( (
 ( 1.000000000000000000, 1.000000000000000000),
 ( 0.3333333333333335369, 0.3333333333333330373),
 ( 0.3333333333333335369, 0.3333333333333330373),
 ( 1.000000000000000000, 1.000000000000000000),
 ( 0.3333333333333333703, 0.3333333333333333703),
 ( 0.3333333333333333703, 0.3333333333333333703),
 ( 1.000000000000000000, 1.000000000000000000) ) ) 
 REPRESENTATION_ITEM ( '' )  SURFACE ( )  );
#12890=EDGE_LOOP ( 'NONE', ( #27698, #35629, #38709, #47515, #10383 ) ) ;
#12894=CARTESIAN_POINT ( 'NONE',  ( -19.23866564181064831, -21.62168251543363695, 58.82507384655653482 ) ) ;
#12895=FACE_OUTER_BOUND ( 'NONE', #43660, .T. ) ;
#12896=( BOUNDED_CURVE ( )  B_SPLINE_CURVE ( 3, ( #19848, #34848, #27946, #8773 ),
 .UNSPECIFIED., .F., .F. ) 
 B_SPLINE_CURVE_WITH_KNOTS ( ( 4, 4 ),
 ( 0.000000000000000000, 0.4074455897393631787 ),
 .UNSPECIFIED. ) 
 CURVE ( )  GEOMETRIC_REPRESENTATION_ITEM ( )  RATIONAL_B_SPLINE_CURVE ( ( 1.000000000000000000, 0.4567392136813412939, 0.3561768502900337641, 0.6983129098260774104 ) ) 
 REPRESENTATION_ITEM ( '' )  );
#12898=CARTESIAN_POINT ( 'NONE',  ( -13.97495002277310583, -20.90053183151249172, 68.47127524766125362 ) ) ;
#12899=CARTESIAN_POINT ( 'NONE',  ( -10.44916082259176093, -15.83527127794237543, 64.80771589743309846 ) ) ;
#12902=CARTESIAN_POINT ( 'NONE',  ( -21.73662441638722953, -9.231682010981758779, 66.67622112302015580 ) ) ;
#12903=CARTESIAN_POINT ( 'NONE',  ( -21.18000576974785787, -20.77541348745421246, 69.35450184739246993 ) ) ;
#12906=ORIENTED_EDGE ( 'NONE', *, *, #12595, .F. ) ;
#12907=CARTESIAN_POINT ( 'NONE',  ( -10.31364544024427410, -17.03300993871772562, 57.80265247535063367 ) ) ;
#12908=CARTESIAN_POINT ( 'NONE',  ( -10.02613496734058351, -15.68824233352117403, 61.18789043449853438 ) ) ;
#12909=VERTEX_POINT ( 'NONE', #7938 ) ;
#12910=CARTESIAN_POINT ( 'NONE',  ( -10.43972881942000086, -15.77115500203794873, 64.52243715390834211 ) ) ;
#12911=AXIS2_PLACEMENT_3D ( 'NONE', #12803, #32264, #43350 ) ;
#12912=DIRECTION ( 'NONE',  ( -2.846534185458051278E-06, -1.189262794577403004E-05, -0.9999999999252313643 ) ) ;
#12914=CARTESIAN_POINT ( 'NONE',  ( -12.50766613833180330, -19.86205114983803455, 64.86674886870797252 ) ) ;
#12915=CARTESIAN_POINT ( 'NONE',  ( -22.50979607835742158, -19.61933652539927309, 72.94400553403978904 ) ) ;
#12916=ORIENTED_EDGE ( 'NONE', *, *, #35977, .T. ) ;
#12917=CARTESIAN_POINT ( 'NONE',  ( -18.67529344402863956, -22.15414776727839907, 72.39855560065855400 ) ) ;
#12918=DIRECTION ( 'NONE',  ( -2.191687988502693051E-06, 1.258878959409210278E-05, 0.9999999999183594168 ) ) ;
#12919=CARTESIAN_POINT ( 'NONE',  ( -24.10556926794565413, -12.55028678686139898, 69.65754220287278997 ) ) ;
#12921=B_SPLINE_CURVE_WITH_KNOTS ( 'NONE', 1,
 ( #48360, #26701 ),
 .UNSPECIFIED., .F., .F.,
 ( 2, 2 ),
 ( 0.000000000000000000, 1.000000000000000000 ),
 .UNSPECIFIED. ) ;
#12922=FACE_OUTER_BOUND ( 'NONE', #23464, .T. ) ;
#12923=ORIENTED_EDGE ( 'NONE', *, *, #4163, .F. ) ;
#12924=DIRECTION ( 'NONE',  ( -0.3478314405900307937, -0.9375570856950865561, 0.000000000000000000 ) ) ;
#12926=CARTESIAN_POINT ( 'NONE',  ( -14.92764441971231726, -21.34891144748960201, 61.93600440564248544 ) ) ;
#12928=DIRECTION ( 'NONE',  ( 0.5820088206811424580, -0.8131824719270214219, 7.019974882119937445E-08 ) ) ;
#12929=FACE_BOUND ( 'NONE', #33914, .T. ) ;
#12931=ORIENTED_EDGE ( 'NONE', *, *, #48449, .T. ) ;
#12933=EDGE_CURVE ( 'NONE', #29013, #14217, #29846, .T. ) ;
#12934=EDGE_CURVE ( 'NONE', #12832, #33156, #44982, .T. ) ;
#12935=CARTESIAN_POINT ( 'NONE',  ( -14.90981281861414587, -21.39562369906352757, 61.78600440604535748 ) ) ;
#12936=CARTESIAN_POINT ( 'NONE',  ( -10.39693166811831304, -15.37990016280386740, 57.58264896457095006 ) ) ;
#12940=ORIENTED_EDGE ( 'NONE', *, *, #42220, .F. ) ;
#12942=EDGE_CURVE ( 'NONE', #17100, #18739, #19476, .T. ) ;
#12946=CYLINDRICAL_SURFACE ( 'NONE', #44903, 0.1500000000000007716 ) ;
#12947=EDGE_CURVE ( 'NONE', #14347, #9986, #43630, .T. ) ;
#12949=ORIENTED_EDGE ( 'NONE', *, *, #2452, .T. ) ;
#12950=CARTESIAN_POINT ( 'NONE',  ( -10.08052675126636721, -16.06451543208143917, 68.09272439531302723 ) ) ;
#12951=CARTESIAN_POINT ( 'NONE',  ( -10.91015311220344053, -11.19381230364907864, 64.29882037057124933 ) ) ;
#12952=CARTESIAN_POINT ( 'NONE',  ( -17.35619151017142769, -7.809413324447545435, 67.02039598641979978 ) ) ;
#12954=LINE ( 'NONE', #39315, #16348 ) ;
#12955=B_SPLINE_CURVE_WITH_KNOTS ( 'NONE', 1,
 ( #29725, #27002 ),
 .UNSPECIFIED., .F., .F.,
 ( 2, 2 ),
 ( 0.000000000000000000, 1.000000000000000000 ),
 .UNSPECIFIED. ) ;
#12956=CARTESIAN_POINT ( 'NONE',  ( -10.42477179210370686, -17.36325313327283482, 61.27087820301521504 ) ) ;
#12957=CARTESIAN_POINT ( 'NONE',  ( -10.98142154448249208, -12.07205956039035399, 74.66726427164191193 ) ) ;
#12958=CARTESIAN_POINT ( 'NONE',  ( -22.28468842640968006, -19.91619389767071269, 65.98949666203347419 ) ) ;
#12960=CARTESIAN_POINT ( 'NONE',  ( -24.43362369560107794, -14.05489154181400124, 73.27271507725298250 ) ) ;
#12961=EDGE_CURVE ( 'NONE', #48574, #28733, #11487, .T. ) ;
#12962=CARTESIAN_POINT ( 'NONE',  ( -23.75972628784533569, -10.79550978475969991, 54.27966884056655061 ) ) ;
#12963=CARTESIAN_POINT ( 'NONE',  ( -12.41100344835299474, -20.32040484475852082, 68.51374354841996706 ) ) ;
#12965=CARTESIAN_POINT ( 'NONE',  ( -10.40245588357037043, -14.17414831712846990, 61.20349182037644198 ) ) ;
#12967=AXIS2_PLACEMENT_3D ( 'NONE', #18379, #14920, #18135 ) ;
#12968=CARTESIAN_POINT ( 'NONE',  ( -19.17247849636888901, -7.567181371456696226, 63.61584626116109575 ) ) ;
#12969=CARTESIAN_POINT ( 'NONE',  ( -20.19231683483797113, -8.325423577284544407, 70.55100341277886855 ) ) ;
#12971=DIRECTION ( 'NONE',  ( 1.424565731581784133E-06, -1.060674514654238452E-05, 0.9999999999427338082 ) ) ;
#12972=LINE ( 'NONE', #28501, #23196 ) ;
#12976=ORIENTED_EDGE ( 'NONE', *, *, #24687, .F. ) ;
#12977=CARTESIAN_POINT ( 'NONE',  ( -10.63483670088760924, -17.87674068094334245, 71.75213521449022380 ) ) ;
#12979=CARTESIAN_POINT ( 'NONE',  ( -13.71293426195967413, -21.26916566922604801, 68.64120525947689089 ) ) ;
#12980=CARTESIAN_POINT ( 'NONE',  ( -23.42083229484411788, -19.23001078651488172, 62.47690011599960513 ) ) ;
#12982=ADVANCED_FACE ( 'NONE', ( #23428 ), #44689, .T. ) ;
#12984=CARTESIAN_POINT ( 'NONE',  ( -11.53435529947139315, -18.68938829637487942, 61.16221976381599745 ) ) ;
#12985=ORIENTED_EDGE ( 'NONE', *, *, #3066, .F. ) ;
#12987=CARTESIAN_POINT ( 'NONE',  ( -20.10876870628512592, -21.27392007786688666, 72.51364836102385425 ) ) ;
#12989=CARTESIAN_POINT ( 'NONE',  ( -11.15651104234136781, -18.05456883900698983, 57.95147637344698666 ) ) ;
#12993=CARTESIAN_POINT ( 'NONE',  ( -19.78161167002369325, -21.87648970866461440, 65.64203102478617780 ) ) ;
#12994=CARTESIAN_POINT ( 'NONE',  ( -23.04402284766838349, -19.06632961612601918, 59.16938527523783620 ) ) ;
#12995=ORIENTED_EDGE ( 'NONE', *, *, #17828, .F. ) ;
#12996=ORIENTED_EDGE ( 'NONE', *, *, #37471, .T. ) ;
#12998=CARTESIAN_POINT ( 'NONE',  ( -10.61707248396235315, -11.78131495581930999, 74.60194320761131337 ) ) ;
#13000=CARTESIAN_POINT ( 'NONE',  ( -21.96934083826521444, -20.13288636094451789, 58.77945318984681933 ) ) ;
#13001=CARTESIAN_POINT ( 'NONE',  ( -20.64578759472022540, -21.08007238041850684, 58.64475173743925751 ) ) ;
#13003=ADVANCED_FACE ( 'NONE', ( #16974 ), #1228, .T. ) ;
#13004=CARTESIAN_POINT ( 'NONE',  ( -11.06587071220225660, -11.88109531467702773, 71.16148941250592941 ) ) ;
#13006=B_SPLINE_CURVE_WITH_KNOTS ( 'NONE', 1,
 ( #11920, #8457 ),
 .UNSPECIFIED., .F., .F.,
 ( 2, 2 ),
 ( 0.000000000000000000, 1.000000000000000000 ),
 .UNSPECIFIED. ) ;
#13009=CARTESIAN_POINT ( 'NONE',  ( -15.62914763455529332, -21.57516310569510054, 72.23678623017254097 ) ) ;
#13010=LINE ( 'NONE', #5406, #40591 ) ;
#13011=( BOUNDED_SURFACE ( )  B_SPLINE_SURFACE ( 3, 1, ( 
 ( #15960, #22392 ),
 ( #23370, #482 ),
 ( #26331, #23139 ),
 ( #15717, #37896 ),
 ( #14980, #37386 ),
 ( #30774, #26578 ),
 ( #38129, #4406 ) ),
 .UNSPECIFIED., .T., .F., .F. ) 
 B_SPLINE_SURFACE_WITH_KNOTS ( ( 4, 3, 4 ),
 ( 2, 2 ),
 ( 0.000000000000000000, 0.5000000000000000000, 1.000000000000000000 ),
 ( 0.000000000000000000, 1.000000000000000000 ),
 .UNSPECIFIED. ) 
 GEOMETRIC_REPRESENTATION_ITEM ( )  RATIONAL_B_SPLINE_SURFACE ( (
 ( 1.000000000000000000, 1.000000000000000000),
 ( 0.3333333333333335369, 0.3333333333333330373),
 ( 0.3333333333333335369, 0.3333333333333330373),
 ( 1.000000000000000000, 1.000000000000000000),
 ( 0.3333333333333333703, 0.3333333333333333703),
 ( 0.3333333333333333703, 0.3333333333333333703),
 ( 1.000000000000000000, 1.000000000000000000) ) ) 
 REPRESENTATION_ITEM ( '' )  SURFACE ( )  );
#13012=EDGE_CURVE ( 'NONE', #39661, #43615, #47348, .T. ) ;
#13013=ORIENTED_EDGE ( 'NONE', *, *, #29269, .T. ) ;
#13014=EDGE_CURVE ( 'NONE', #25854, #1499, #32676, .T. ) ;
#13015=CARTESIAN_POINT ( 'NONE',  ( -23.58371808145649950, -11.48100254794470310, 69.96381055508895486 ) ) ;
#13018=CARTESIAN_POINT ( 'NONE',  ( -17.84575570470781258, -7.371070506658266908, 60.33706685437874739 ) ) ;
#13019=CARTESIAN_POINT ( 'NONE',  ( -22.68104036972259507, -20.08820309574320362, 69.36692159779713052 ) ) ;
#13021=( BOUNDED_CURVE ( )  B_SPLINE_CURVE ( 3, ( #37623, #46011, #12264, #26816 ),
 .UNSPECIFIED., .F., .F. ) 
 B_SPLINE_CURVE_WITH_KNOTS ( ( 4, 4 ),
 ( 0.9074455897393673975, 1.000000000000000000 ),
 .UNSPECIFIED. ) 
 CURVE ( )  GEOMETRIC_REPRESENTATION_ITEM ( )  RATIONAL_B_SPLINE_CURVE ( ( 0.6983129098261030565, 0.7760317562607068620, 0.8765941196520058432, 1.000000000000000000 ) ) 
 REPRESENTATION_ITEM ( '' )  );
#13023=B_SPLINE_CURVE_WITH_KNOTS ( 'NONE', 1,
 ( #33925, #37605 ),
 .UNSPECIFIED., .F., .F.,
 ( 2, 2 ),
 ( 0.000000000000000000, 1.000000000000000000 ),
 .UNSPECIFIED. ) ;
#13024=CARTESIAN_POINT ( 'NONE',  ( -13.17078218117215549, -9.186392337449538203, 67.39414915108072535 ) ) ;
#13025=ORIENTED_EDGE ( 'NONE', *, *, #19904, .F. ) ;
#13027=CYLINDRICAL_SURFACE ( 'NONE', #45507, 0.1499999999999984401 ) ;
#13030=CARTESIAN_POINT ( 'NONE',  ( -12.64201450438284624, -19.99346662158319887, 72.22142341168820678 ) ) ;
#13031=ORIENTED_EDGE ( 'NONE', *, *, #16274, .T. ) ;
#13032=CARTESIAN_POINT ( 'NONE',  ( -21.06635048418738165, -21.30826373965517817, 62.29966805574095901 ) ) ;
#13033=CARTESIAN_POINT ( 'NONE',  ( -14.79922921121938195, -7.836842249070715916, 57.03495322699122738 ) ) ;
#13035=EDGE_LOOP ( 'NONE', ( #10533, #25830, #2928, #40089, #13937 ) ) ;
#13036=CARTESIAN_POINT ( 'NONE',  ( -24.18037300165767434, -17.94870813986570113, 59.18873840842728384 ) ) ;
#13037=( BOUNDED_CURVE ( )  B_SPLINE_CURVE ( 3, ( #91, #41196, #12132, #807 ),
 .UNSPECIFIED., .F., .F. ) 
 B_SPLINE_CURVE_WITH_KNOTS ( ( 4, 4 ),
 ( 0.4074455897393615689, 0.5000000000000000000 ),
 .UNSPECIFIED. ) 
 CURVE ( )  GEOMETRIC_REPRESENTATION_ITEM ( )  RATIONAL_B_SPLINE_CURVE ( ( 0.6983129098260865142, 0.7760317562606893205, 0.8765941196519929646, 0.9999999999999950040 ) ) 
 REPRESENTATION_ITEM ( '' )  );
#13039=CARTESIAN_POINT ( 'NONE',  ( -24.76961015134066102, -16.05258769581026002, 66.26336133875032885 ) ) ;
#13040=EDGE_LOOP ( 'NONE', ( #8574, #10992, #12916, #48404, #33301 ) ) ;
#13041=ORIENTED_EDGE ( 'NONE', *, *, #40709, .T. ) ;
#13043=PLANE ( 'NONE',  #13178 ) ;
#13044=ORIENTED_EDGE ( 'NONE', *, *, #34654, .T. ) ;
#13048=CARTESIAN_POINT ( 'NONE',  ( -13.03317698800707802, -8.790695117698408723, 64.10935296935409156 ) ) ;
#13049=CARTESIAN_POINT ( 'NONE',  ( -22.48114103837971101, -19.64927616005747879, 72.64400547034465205 ) ) ;
#13052=ADVANCED_FACE ( 'NONE', ( #9138 ), #6284, .T. ) ;
#13053=FACE_OUTER_BOUND ( 'NONE', #41126, .T. ) ;
#13054=CARTESIAN_POINT ( 'NONE',  ( -18.78584198798900928, -7.883846953673406155, 63.58656136513857149 ) ) ;
#13055=CARTESIAN_POINT ( 'NONE',  ( -22.88264614489240856, -10.34704276773305764, 63.35713876973677827 ) ) ;
#13056=CARTESIAN_POINT ( 'NONE',  ( -12.86353962931362283, -9.432586330540292607, 74.33395128836551180 ) ) ;
#13057=CARTESIAN_POINT ( 'NONE',  ( -13.45042104576995889, -20.57396378630483369, 61.62719528072427266 ) ) ;
#13058=EDGE_LOOP ( 'NONE', ( #26669, #25019, #1840, #16972, #11633 ) ) ;
#13059=ORIENTED_EDGE ( 'NONE', *, *, #12721, .T. ) ;
#13060=ORIENTED_EDGE ( 'NONE', *, *, #11942, .F. ) ;
#13062=CARTESIAN_POINT ( 'NONE',  ( -18.92057809895272058, -7.919864474132484844, 66.90071783790342863 ) ) ;
#13063=CARTESIAN_POINT ( 'NONE',  ( -20.04849592361258104, -21.35284569240296548, 72.69006679631317525 ) ) ;
#13064=ORIENTED_EDGE ( 'NONE', *, *, #48070, .T. ) ;
#13065=EDGE_CURVE ( 'NONE', #29117, #15587, #16323, .T. ) ;
#13066=CARTESIAN_POINT ( 'NONE',  ( -10.43656090296491179, -14.37069206989541392, 68.08629950323120283 ) ) ;
#13069=CARTESIAN_POINT ( 'NONE',  ( -9.994877497295997060, -15.37525289974553289, 57.75448116320448833 ) ) ;
#13071=EDGE_CURVE ( 'NONE', #936, #25681, #36445, .T. ) ;
#13073=CARTESIAN_POINT ( 'NONE',  ( -11.32469277870022850, -18.34471304272907588, 58.10714594244493725 ) ) ;
#13074=FACE_OUTER_BOUND ( 'NONE', #33793, .T. ) ;
#13075=VERTEX_POINT ( 'NONE', #21186 ) ;
#13082=CARTESIAN_POINT ( 'NONE',  ( -11.68672710392437608, -10.05669134056747005, 67.68392285705759548 ) ) ;
#13085=CARTESIAN_POINT ( 'NONE',  ( -24.42401512807229125, -14.72416121340251571, 62.99679879080087375 ) ) ;
#13086=CARTESIAN_POINT ( 'NONE',  ( -24.08271688320076720, -11.46738811444140538, 63.11251657512028146 ) ) ;
#13088=CARTESIAN_POINT ( 'NONE',  ( -10.46375309629256201, -15.55739590339904233, 61.32172507360417057 ) ) ;
#13091=CARTESIAN_POINT ( 'NONE',  ( -23.80521486491402428, -10.96423656519770340, 73.51193299235829670 ) ) ;
#13092=CARTESIAN_POINT ( 'NONE',  ( -11.84412991438031248, -19.03588838109888570, 71.70188265515885462 ) ) ;
#13094=CARTESIAN_POINT ( 'NONE',  ( -23.19948571119275726, -18.85291137746749968, 65.83861571032234394 ) ) ;
#13096=EDGE_CURVE ( 'NONE', #38891, #19754, #19163, .T. ) ;
#13097=ORIENTED_EDGE ( 'NONE', *, *, #11107, .T. ) ;
#13098=CARTESIAN_POINT ( 'NONE',  ( -16.48446094845526488, -7.818459999738816002, 60.29208735039289735 ) ) ;
#13099=CARTESIAN_POINT ( 'NONE',  ( -24.42398663107514523, -15.65075326911586906, 73.01775867260030850 ) ) ;
#13100=ORIENTED_EDGE ( 'NONE', *, *, #29970, .F. ) ;
#13101=CARTESIAN_POINT ( 'NONE',  ( -21.99178428503402216, -9.439038574390064440, 60.02171213140444195 ) ) ;
#13102=CARTESIAN_POINT ( 'NONE',  ( -23.49945856589985027, -11.21686614839013885, 66.57781614479455357 ) ) ;
#13103=CARTESIAN_POINT ( 'NONE',  ( -12.63116919492461854, -9.104687665260810192, 70.96270001146038453 ) ) ;
#13104=FACE_OUTER_BOUND ( 'NONE', #1044, .T. ) ;
#13105=PLANE ( 'NONE',  #37596 ) ;
#13107=CARTESIAN_POINT ( 'NONE',  ( -12.10973142303912908, -9.588019877982702610, 57.19597242491963840 ) ) ;
#13110=CARTESIAN_POINT ( 'NONE',  ( -23.70099262725067746, -17.91056972029587513, 59.23208246994288118 ) ) ;
#13111=ORIENTED_EDGE ( 'NONE', *, *, #9237, .T. ) ;
#13112=CARTESIAN_POINT ( 'NONE',  ( -17.15134141312287852, -7.364115244199362920, 70.67531166753866501 ) ) ;
#13113=( BOUNDED_CURVE ( )  B_SPLINE_CURVE ( 3, ( #23070, #16377, #27474, #38059 ),
 .UNSPECIFIED., .F., .F. ) 
 B_SPLINE_CURVE_WITH_KNOTS ( ( 4, 4 ),
 ( 0.000000000000000000, 0.4074455897393672310 ),
 .UNSPECIFIED. ) 
 CURVE ( )  GEOMETRIC_REPRESENTATION_ITEM ( )  RATIONAL_B_SPLINE_CURVE ( ( 1.000000000000000000, 0.4567392136813307468, 0.3561768502900298783, 0.6983129098260973944 ) ) 
 REPRESENTATION_ITEM ( '' )  );
#13114=CARTESIAN_POINT ( 'NONE',  ( -23.49719401221368642, -11.32496260901646856, 73.47266466796968132 ) ) ;
#13116=CARTESIAN_POINT ( 'NONE',  ( -10.75774562132040479, -12.66857536220184777, 64.45763188802062871 ) ) ;
#13118=ORIENTED_EDGE ( 'NONE', *, *, #44769, .T. ) ;
#13120=CARTESIAN_POINT ( 'NONE',  ( -10.91566558191575531, -17.52836192114708425, 64.83559378099900528 ) ) ;
#13121=CARTESIAN_POINT ( 'NONE',  ( -15.28303595616968913, -7.672713470548185200, 74.19330299898706471 ) ) ;
#13122=CARTESIAN_POINT ( 'NONE',  ( -11.55573855159262386, -10.21941529800896653, 71.15388400389697665 ) ) ;
#13123=CARTESIAN_POINT ( 'NONE',  ( -24.44839783832460967, -14.20609194633158623, 69.94715494824646385 ) ) ;
#13124=EDGE_CURVE ( 'NONE', #40875, #6404, #19503, .T. ) ;
#13127=CARTESIAN_POINT ( 'NONE',  ( -19.35269785843539125, -22.00525528091193195, 58.72496154332668539 ) ) ;
#13128=CARTESIAN_POINT ( 'NONE',  ( -24.39459507417318562, -17.43899346222085711, 69.66985698250167047 ) ) ;
#13130=CARTESIAN_POINT ( 'NONE',  ( -23.83080496556880945, -17.75212211224490133, 59.28906343887996400 ) ) ;
#13131=CARTESIAN_POINT ( 'NONE',  ( -16.16523928603239924, -21.74967706772850207, 62.05568406594436226 ) ) ;
#13132=AXIS2_PLACEMENT_3D ( 'NONE', #18376, #45485, #26271 ) ;
#13133=ORIENTED_EDGE ( 'NONE', *, *, #29378, .F. ) ;
#13134=EDGE_CURVE ( 'NONE', #24440, #43669, #41484, .T. ) ;
#13135=ADVANCED_FACE ( 'NONE', ( #10815 ), #13528, .T. ) ;
#13136=CARTESIAN_POINT ( 'NONE',  ( -19.23866243364646422, -21.62168334911581269, 58.52507384657483414 ) ) ;
#13137=DIRECTION ( 'NONE',  ( 0.7800143876985550229, -0.6257615799833393666, 5.505484597913564244E-08 ) ) ;
#13140=DIRECTION ( 'NONE',  ( -3.964551025433374905E-06, -2.747358590626761473E-07, 0.9999999999921033167 ) ) ;
#13143=CARTESIAN_POINT ( 'NONE',  ( -10.69226473215256590, -16.91570156256109669, 61.45743193859061648 ) ) ;
#13144=CARTESIAN_POINT ( 'NONE',  ( -24.71334378318632830, -13.26952680650525274, 59.47772536435775947 ) ) ;
#13145=ORIENTED_EDGE ( 'NONE', *, *, #9280, .T. ) ;
#13146=CARTESIAN_POINT ( 'NONE',  ( -14.40524399388063514, -8.438208624349055498, 67.55975084334407654 ) ) ;
#13147=CARTESIAN_POINT ( 'NONE',  ( -24.37683854932038585, -15.97618581480151434, 66.21324926630431662 ) ) ;
#13148=CARTESIAN_POINT ( 'NONE',  ( -21.36489517220793743, -8.963474395264050543, 73.75128753236120360 ) ) ;
#13149=CARTESIAN_POINT ( 'NONE',  ( -11.60526899143904345, -18.79015832504765626, 68.23161775275829655 ) ) ;
#13150=CARTESIAN_POINT ( 'NONE',  ( -21.63336539757928634, -9.153348366551478321, 66.94677872351418557 ) ) ;
#13151=EDGE_CURVE ( 'NONE', #45924, #27231, #332, .T. ) ;
#13152=CARTESIAN_POINT ( 'NONE',  ( -16.71957921250844592, -21.82421608262117729, 68.71032757591046902 ) ) ;
#13153=EDGE_LOOP ( 'NONE', ( #23802, #24318 ) ) ;
#13154=CARTESIAN_POINT ( 'NONE',  ( -13.86149102995237037, -8.266187410065942487, 74.30616366049129340 ) ) ;
#13155=CARTESIAN_POINT ( 'NONE',  ( -20.12398138731996511, -21.75278012861551247, 72.60489934222226793 ) ) ;
#13156=CARTESIAN_POINT ( 'NONE',  ( -13.41327373486474883, -20.54621981236622830, 58.04650078084816300 ) ) ;
#13157=( BOUNDED_CURVE ( )  B_SPLINE_CURVE ( 3, ( #13233, #28286, #39602, #21139 ),
 .UNSPECIFIED., .F., .F. ) 
 B_SPLINE_CURVE_WITH_KNOTS ( ( 4, 4 ),
 ( 0.4074455897393602921, 0.5000000000000000000 ),
 .UNSPECIFIED. ) 
 CURVE ( )  GEOMETRIC_REPRESENTATION_ITEM ( )  RATIONAL_B_SPLINE_CURVE ( ( 0.6983129098260720813, 0.7760317562606737773, 0.8765941196519813072, 0.9999999999999900080 ) ) 
 REPRESENTATION_ITEM ( '' )  );
#13158=ORIENTED_EDGE ( 'NONE', *, *, #35096, .T. ) ;
#13160=ORIENTED_EDGE ( 'NONE', *, *, #39737, .T. ) ;
#13164=AXIS2_PLACEMENT_3D ( 'NONE', #22299, #29442, #33856 ) ;
#13165=CARTESIAN_POINT ( 'NONE',  ( -23.75261229635691862, -11.81743247384379991, 59.76770420102489823 ) ) ;
#13166=CARTESIAN_POINT ( 'NONE',  ( -17.36778503871311230, -7.359366238864594401, 67.21313763515482265 ) ) ;
#13169=( BOUNDED_CURVE ( )  B_SPLINE_CURVE ( 3, ( #5629, #20639, #35634, #31952 ),
 .UNSPECIFIED., .F., .F. ) 
 B_SPLINE_CURVE_WITH_KNOTS ( ( 4, 4 ),
 ( 0.5000000000000000000, 0.9074455897393722825 ),
 .UNSPECIFIED. ) 
 CURVE ( )  GEOMETRIC_REPRESENTATION_ITEM ( )  RATIONAL_B_SPLINE_CURVE ( ( 0.9999999999999791278, 0.4567392136813193115, 0.3561768502900400923, 0.6983129098261189327 ) ) 
 REPRESENTATION_ITEM ( '' )  );
#13170=EDGE_LOOP ( 'NONE', ( #10073, #20002 ) ) ;
#13171=ORIENTED_EDGE ( 'NONE', *, *, #591, .T. ) ;
#13173=CARTESIAN_POINT ( 'NONE',  ( -13.85393650630732054, -8.270265118416840977, 74.38450092284953996 ) ) ;
#13176=ADVANCED_FACE ( 'NONE', ( #43846 ), #14243, .F. ) ;
#13178=AXIS2_PLACEMENT_3D ( 'NONE', #28806, #43844, #28074 ) ;
#13179=ORIENTED_EDGE ( 'NONE', *, *, #41129, .F. ) ;
#13181=ADVANCED_FACE ( 'NONE', ( #25359 ), #6884, .T. ) ;
#13183=CARTESIAN_POINT ( 'NONE',  ( -11.64235247690698749, -18.84330696305777408, 68.51689631558762983 ) ) ;
#13186=DIRECTION ( 'NONE',  ( 3.298726456874245264E-06, -1.683524832386861475E-06, -0.9999999999931420414 ) ) ;
#13187=CARTESIAN_POINT ( 'NONE',  ( -16.20683845212634111, -21.70255763714999020, 58.58585572420326315 ) ) ;
#13189=EDGE_CURVE ( 'NONE', #22471, #45412, #16793, .T. ) ;
#13190=EDGE_LOOP ( 'NONE', ( #41093, #30734 ) ) ;
#13192=CARTESIAN_POINT ( 'NONE',  ( -11.07857831884827604, -11.73724749328988359, 71.23860870961335934 ) ) ;
#13193=EDGE_CURVE ( 'NONE', #32966, #48033, #14974, .T. ) ;
#13194=CARTESIAN_POINT ( 'NONE',  ( -22.93054552543627977, -10.40195957496224644, 66.95671006072360854 ) ) ;
#13195=DIRECTION ( 'NONE',  ( 7.381188785182666071E-06, 5.670466977913946987E-06, 0.9999999999566818731 ) ) ;
#13197=CYLINDRICAL_SURFACE ( 'NONE', #19731, 0.1500000000000050460 ) ;
#13198=AXIS2_PLACEMENT_3D ( 'NONE', #46002, #1663, #27038 ) ;
#13199=VERTEX_POINT ( 'NONE', #3426 ) ;
#13200=CARTESIAN_POINT ( 'NONE',  ( -14.66404237506551311, -7.889278293989088198, 60.42722112806361423 ) ) ;
#13201=ADVANCED_FACE ( 'NONE', ( #8119 ), #41594, .T. ) ;
#13203=CARTESIAN_POINT ( 'NONE',  ( -10.98557813051190024, -17.68114236276378293, 71.56718193507128944 ) ) ;
#13205=CARTESIAN_POINT ( 'NONE',  ( -13.60894707410760240, -8.877133421815647907, 60.85439169328856934 ) ) ;
#13208=CARTESIAN_POINT ( 'NONE',  ( -13.40417755890050699, -20.60086790338396057, 58.34650048655475274 ) ) ;
#13209=AXIS2_PLACEMENT_3D ( 'NONE', #45112, #15509, #33488 ) ;
#13210=ADVANCED_FACE ( 'NONE', ( #7138 ), #37139, .T. ) ;
#13212=CARTESIAN_POINT ( 'NONE',  ( -15.29626560849200878, -8.084834557582363246, 73.96496852212565898 ) ) ;
#13213=VERTEX_POINT ( 'NONE', #245 ) ;
#13214=( BOUNDED_CURVE ( )  B_SPLINE_CURVE ( 3, ( #25226, #43706, #6267, #9729 ),
 .UNSPECIFIED., .F., .F. ) 
 B_SPLINE_CURVE_WITH_KNOTS ( ( 4, 4 ),
 ( 0.000000000000000000, 0.4074455897393638448 ),
 .UNSPECIFIED. ) 
 CURVE ( )  GEOMETRIC_REPRESENTATION_ITEM ( )  RATIONAL_B_SPLINE_CURVE ( ( 1.000000000000000000, 0.4567392136813241965, 0.3561768502900274358, 0.6983129098261096068 ) ) 
 REPRESENTATION_ITEM ( '' )  );
#13215=CARTESIAN_POINT ( 'NONE',  ( -11.06796828401846078, -18.69550736580278993, 61.53356777548469125 ) ) ;
#13216=EDGE_LOOP ( 'NONE', ( #47726, #33416 ) ) ;
#13217=ORIENTED_EDGE ( 'NONE', *, *, #47404, .F. ) ;
#13218=CARTESIAN_POINT ( 'NONE',  ( -24.08907123645992243, -11.48026457312919391, 63.13713595337925000 ) ) ;
#13219=CARTESIAN_POINT ( 'NONE',  ( -20.10940917962770769, -21.27365406404410564, 72.59582005363583335 ) ) ;
#13223=CARTESIAN_POINT ( 'NONE',  ( -12.79725882921341551, -20.12850138265567068, 72.10653676770067477 ) ) ;
#13224=B_SPLINE_CURVE_WITH_KNOTS ( 'NONE', 3,
 ( #11100, #24, #48511, #19454, #34461, #18467, #4207, #30071, #45094, #33470 ),
 .UNSPECIFIED., .F., .F.,
 ( 4, 2, 2, 2, 4 ),
 ( 0.000000000000000000, 0.2500000000000000000, 0.5000000000000000000, 0.7500000000000000000, 1.000000000000000000 ),
 .UNSPECIFIED. ) ;
#13226=CARTESIAN_POINT ( 'NONE',  ( -10.53028993777715883, -16.28642212234895226, 71.73278239416407587 ) ) ;
#13227=CARTESIAN_POINT ( 'NONE',  ( -13.90630441925721250, -21.37656106130631173, 72.06461169531037569 ) ) ;
#13228=ORIENTED_EDGE ( 'NONE', *, *, #27195, .T. ) ;
#13229=ORIENTED_EDGE ( 'NONE', *, *, #38282, .T. ) ;
#13230=CARTESIAN_POINT ( 'NONE',  ( -11.32522400900782067, -11.27219014254736074, 60.96413645226084554 ) ) ;
#13232=AXIS2_PLACEMENT_3D ( 'NONE', #10861, #11114, #36686 ) ;
#13233=CARTESIAN_POINT ( 'NONE',  ( -11.42622084110231029, -18.51434063454204093, 61.27710833181470917 ) ) ;
#13234=FACE_OUTER_BOUND ( 'NONE', #46972, .T. ) ;
#13240=VERTEX_POINT ( 'NONE', #41846 ) ;
#13241=DIRECTION ( 'NONE',  ( 0.4433615477241706904, -0.8963428685495450354, 2.661652803430218851E-08 ) ) ;
#13242=CARTESIAN_POINT ( 'NONE',  ( -10.21393201348709212, -12.93341964037237091, 67.89865688031065361 ) ) ;
#13243=CARTESIAN_POINT ( 'NONE',  ( -10.98557813051190202, -17.68114236276378293, 71.56718193507127523 ) ) ;
#13244=FACE_OUTER_BOUND ( 'NONE', #16108, .T. ) ;
#13245=B_SPLINE_CURVE_WITH_KNOTS ( 'NONE', 1,
 ( #29579, #40417 ),
 .UNSPECIFIED., .F., .F.,
 ( 2, 2 ),
 ( 0.000000000000000000, 1.000000000000000000 ),
 .UNSPECIFIED. ) ;
#13247=CARTESIAN_POINT ( 'NONE',  ( -11.64547064851736202, -18.85300969848255193, 64.63218190802510321 ) ) ;
#13248=CARTESIAN_POINT ( 'NONE',  ( -13.53325528467554406, -21.16256411608339150, 65.17124155742401115 ) ) ;
#13252=LINE ( 'NONE', #29270, #28094 ) ;
#13253=ADVANCED_FACE ( 'NONE', ( #34427 ), #18430, .F. ) ;
#13254=CARTESIAN_POINT ( 'NONE',  ( -14.78597691548102411, -7.841758819152822468, 56.98853511513466685 ) ) ;
#13257=DIRECTION ( 'NONE',  ( -0.05202058437830281434, 0.9986460127597465153, -1.657953767072174380E-08 ) ) ;
#13259=FACE_OUTER_BOUND ( 'NONE', #17409, .T. ) ;
#13261=CARTESIAN_POINT ( 'NONE',  ( -10.27563016671317619, -12.71093163253470237, 64.46110259866301817 ) ) ;
#13264=EDGE_LOOP ( 'NONE', ( #9091, #23742, #27695, #30631, #30360 ) ) ;
#13265=CARTESIAN_POINT ( 'NONE',  ( -12.02400285154091897, -10.35258023360360369, 71.07966224361382501 ) ) ;
#13267=CARTESIAN_POINT ( 'NONE',  ( -19.45281838860202228, -9.697037067072804106, 54.07175714974879099 ) ) ;
#13272=FACE_OUTER_BOUND ( 'NONE', #32001, .T. ) ;
#13274=CARTESIAN_POINT ( 'NONE',  ( -23.80321451250838649, -17.81075939459467961, 59.00378417737415049 ) ) ;
#13276=VERTEX_POINT ( 'NONE', #4180 ) ;
#13277=CARTESIAN_POINT ( 'NONE',  ( -10.77303329795002895, -12.62668660113453178, 60.79853568451941470 ) ) ;
#13278=CARTESIAN_POINT ( 'NONE',  ( -18.57335281209669731, -21.76520412651811043, 72.57038810541313012 ) ) ;
#13280=CARTESIAN_POINT ( 'NONE',  ( -24.33438471898804778, -15.92705986081045744, 66.06324874090134358 ) ) ;
#13281=CARTESIAN_POINT ( 'NONE',  ( -23.25590038356622102, -18.77701127317174112, 62.56226639404914636 ) ) ;
#13284=CARTESIAN_POINT ( 'NONE',  ( -23.82366785274684418, -10.99486113721019009, 73.47697904737684382 ) ) ;
#13286=CARTESIAN_POINT ( 'NONE',  ( -10.63418523514201652, -17.87528017975677130, 71.61072290056861789 ) ) ;
#13288=ADVANCED_FACE ( 'NONE', ( #30040 ), #24555, .T. ) ;
#13289=ORIENTED_EDGE ( 'NONE', *, *, #15489, .F. ) ;
#13291=CARTESIAN_POINT ( 'NONE',  ( -24.48495216189764534, -12.43291116107568861, 73.39225569044465658 ) ) ;
#13292=CARTESIAN_POINT ( 'NONE',  ( -13.51031689544038805, -20.61338442564125728, 61.80029829250916151 ) ) ;
#13293=( BOUNDED_CURVE ( )  B_SPLINE_CURVE ( 3, ( #32266, #29525, #2925, #29040 ),
 .UNSPECIFIED., .F., .F. ) 
 B_SPLINE_CURVE_WITH_KNOTS ( ( 4, 4 ),
 ( 0.9074455897393689519, 1.000000000000000000 ),
 .UNSPECIFIED. ) 
 CURVE ( )  GEOMETRIC_REPRESENTATION_ITEM ( )  RATIONAL_B_SPLINE_CURVE ( ( 0.6983129098261018353, 0.7760317562607057518, 0.8765941196520051770, 1.000000000000000000 ) ) 
 REPRESENTATION_ITEM ( '' )  );
#13296=ORIENTED_EDGE ( 'NONE', *, *, #30967, .F. ) ;
#13297=CARTESIAN_POINT ( 'NONE',  ( -17.65810221059773610, -7.762793303104815301, 63.56529088875731759 ) ) ;
#13300=CARTESIAN_POINT ( 'NONE',  ( -21.70317610893864924, -9.269322718887449852, 63.41827076980987954 ) ) ;
#13301=( BOUNDED_SURFACE ( )  B_SPLINE_SURFACE ( 3, 1, ( 
 ( #46161, #46890 ),
 ( #4805, #39011 ),
 ( #867, #34580 ),
 ( #12902, #38260 ),
 ( #1328, #8494 ),
 ( #24009, #9228 ),
 ( #38768, #5287 ) ),
 .UNSPECIFIED., .T., .F., .F. ) 
 B_SPLINE_SURFACE_WITH_KNOTS ( ( 4, 3, 4 ),
 ( 2, 2 ),
 ( 0.000000000000000000, 0.5000000000000000000, 1.000000000000000000 ),
 ( 0.000000000000000000, 1.000000000000000000 ),
 .UNSPECIFIED. ) 
 GEOMETRIC_REPRESENTATION_ITEM ( )  RATIONAL_B_SPLINE_SURFACE ( (
 ( 1.000000000000000000, 1.000000000000000000),
 ( 0.3333333333333335369, 0.3333333333333330373),
 ( 0.3333333333333335369, 0.3333333333333330373),
 ( 1.000000000000000000, 1.000000000000000000),
 ( 0.3333333333333333703, 0.3333333333333333703),
 ( 0.3333333333333333703, 0.3333333333333333703),
 ( 1.000000000000000000, 1.000000000000000000) ) ) 
 REPRESENTATION_ITEM ( '' )  SURFACE ( )  );
#13302=EDGE_LOOP ( 'NONE', ( #23631, #27053 ) ) ;
#13303=( BOUNDED_SURFACE ( )  B_SPLINE_SURFACE ( 3, 1, ( 
 ( #7779, #30671 ),
 ( #3832, #41986 ),
 ( #38258, #45206 ),
 ( #4547, #12184 ),
 ( #27201, #8492 ),
 ( #33592, #48632 ),
 ( #44970, #41246 ) ),
 .UNSPECIFIED., .T., .F., .F. ) 
 B_SPLINE_SURFACE_WITH_KNOTS ( ( 4, 3, 4 ),
 ( 2, 2 ),
 ( 0.000000000000000000, 0.5000000000000000000, 1.000000000000000000 ),
 ( 0.000000000000000000, 1.000000000000000000 ),
 .UNSPECIFIED. ) 
 GEOMETRIC_REPRESENTATION_ITEM ( )  RATIONAL_B_SPLINE_SURFACE ( (
 ( 1.000000000000000000, 1.000000000000000000),
 ( 0.3333333333333335369, 0.3333333333333330373),
 ( 0.3333333333333335369, 0.3333333333333330373),
 ( 1.000000000000000000, 1.000000000000000000),
 ( 0.3333333333333333703, 0.3333333333333333703),
 ( 0.3333333333333333703, 0.3333333333333333703),
 ( 1.000000000000000000, 1.000000000000000000) ) ) 
 REPRESENTATION_ITEM ( '' )  SURFACE ( )  );
#13306=CARTESIAN_POINT ( 'NONE',  ( -16.18458696102261385, -7.463033837898945144, 60.40017247762416019 ) ) ;
#13308=ORIENTED_EDGE ( 'NONE', *, *, #34768, .T. ) ;
#13310=AXIS2_PLACEMENT_3D ( 'NONE', #15832, #34797, #27409 ) ;
#13311=CARTESIAN_POINT ( 'NONE',  ( -12.56699215081136600, -20.45835600996747417, 71.92840931458714238 ) ) ;
#13313=CARTESIAN_POINT ( 'NONE',  ( -21.96667192285332604, -8.904124347047575938, 66.80116649577588817 ) ) ;
#13314=B_SPLINE_CURVE_WITH_KNOTS ( 'NONE', 3,
 ( #32061, #47083, #8937, #42907, #13324, #38959, #20249, #1532, #16539, #46611 ),
 .UNSPECIFIED., .F., .F.,
 ( 4, 2, 2, 2, 4 ),
 ( 0.6272669072977246074, 0.7522669073147544294, 0.8772669073317842514, 1.002266907348813962, 1.127266907365843895 ),
 .UNSPECIFIED. ) ;
#13315=VERTEX_POINT ( 'NONE', #23367 ) ;
#13316=CARTESIAN_POINT ( 'NONE',  ( -13.52595587147657596, -21.15804559846413824, 65.09290550380976015 ) ) ;
#13317=( BOUNDED_CURVE ( )  B_SPLINE_CURVE ( 3, ( #29951, #3348, #14393, #11233 ),
 .UNSPECIFIED., .F., .F. ) 
 B_SPLINE_CURVE_WITH_KNOTS ( ( 4, 4 ),
 ( 0.9074455897393632897, 1.000000000000000000 ),
 .UNSPECIFIED. ) 
 CURVE ( )  GEOMETRIC_REPRESENTATION_ITEM ( )  RATIONAL_B_SPLINE_CURVE ( ( 0.6983129098260950629, 0.7760317562606999786, 0.8765941196520016243, 1.000000000000000000 ) ) 
 REPRESENTATION_ITEM ( '' )  );
#13318=ORIENTED_EDGE ( 'NONE', *, *, #41790, .F. ) ;
#13319=CARTESIAN_POINT ( 'NONE',  ( -11.90871160445621868, -19.81768789853573054, 58.10495117216805738 ) ) ;
#13321=EDGE_CURVE ( 'NONE', #46319, #40340, #29557, .T. ) ;
#13322=FACE_OUTER_BOUND ( 'NONE', #9047, .T. ) ;
#13323=ORIENTED_EDGE ( 'NONE', *, *, #37392, .F. ) ;
#13324=CARTESIAN_POINT ( 'NONE',  ( -24.26779606828610270, -17.75336464367330080, 62.59548250328385421 ) ) ;
#13325=CARTESIAN_POINT ( 'NONE',  ( -24.70163917427996481, -16.40367249003021755, 59.26185880907539882 ) ) ;
#13328=CARTESIAN_POINT ( 'NONE',  ( -14.78754716229542865, -8.270772359302402066, 60.31996282000578447 ) ) ;
#13331=ORIENTED_EDGE ( 'NONE', *, *, #28474, .F. ) ;
#13332=CARTESIAN_POINT ( 'NONE',  ( -14.99687845949598319, -8.186362001186598292, 60.41176252006127356 ) ) ;
#13334=CYLINDRICAL_SURFACE ( 'NONE', #38413, 0.1500000000000028533 ) ;
#13335=DIRECTION ( 'NONE',  ( 0.8967515337576289491, -0.4425343904188010491, 9.546469656967252871E-09 ) ) ;
#13342=CARTESIAN_POINT ( 'NONE',  ( -9.973354012397450674, -14.79738236791871664, 71.44127436690867228 ) ) ;
#13343=CARTESIAN_POINT ( 'NONE',  ( -10.13226805943771858, -16.33660356775173739, 71.49104427242312454 ) ) ;
#13344=CARTESIAN_POINT ( 'NONE',  ( -14.58888777286794358, -8.408946862453658966, 64.08978847350323349 ) ) ;
#13345=CARTESIAN_POINT ( 'NONE',  ( -14.72778340125292651, -21.32322296975913645, 58.46617885012762628 ) ) ;
#13346=CARTESIAN_POINT ( 'NONE',  ( -23.78676187654788521, -10.93361199230012559, 73.54688693628270357 ) ) ;
#13347=ORIENTED_EDGE ( 'NONE', *, *, #40612, .T. ) ;
#13349=CARTESIAN_POINT ( 'NONE',  ( -23.76773510245185506, -11.84597926658418565, 63.14145293063592845 ) ) ;
#13352=LINE ( 'NONE', #31357, #26522 ) ;
#13353=CARTESIAN_POINT ( 'NONE',  ( -23.74125327615269754, -17.82500477549296036, 59.00378426403860033 ) ) ;
#13355=EDGE_CURVE ( 'NONE', #25477, #10558, #6778, .T. ) ;
#13357=VERTEX_POINT ( 'NONE', #1922 ) ;
#13359=CARTESIAN_POINT ( 'NONE',  ( -15.90376647335224192, -7.921387445786724157, 70.70170099352583293 ) ) ;
#13360=AXIS2_PLACEMENT_3D ( 'NONE', #20764, #32799, #29116 ) ;
#13362=CARTESIAN_POINT ( 'NONE',  ( -21.15336504700141163, -20.73310185707507713, 69.05450185101547333 ) ) ;
#13364=CARTESIAN_POINT ( 'NONE',  ( -10.12541953518153370, -16.30314513718451508, 71.59750380059928432 ) ) ;
#13365=ORIENTED_EDGE ( 'NONE', *, *, #25374, .T. ) ;
#13366=ORIENTED_EDGE ( 'NONE', *, *, #33378, .T. ) ;
#13368=CARTESIAN_POINT ( 'NONE',  ( -10.78898398081525301, -17.19290454168847404, 61.44271037915215317 ) ) ;
#13369=CARTESIAN_POINT ( 'NONE',  ( -15.43182990062313742, -8.046249867383863830, 74.36513541778452918 ) ) ;
#13370=CARTESIAN_POINT ( 'NONE',  ( -14.23620588414828880, -8.577105282884037507, 70.72957618505992627 ) ) ;
#13371=ADVANCED_FACE ( 'NONE', ( #31724 ), #39350, .F. ) ;
#13373=EDGE_LOOP ( 'NONE', ( #14681, #37541 ) ) ;
#13374=AXIS2_PLACEMENT_3D ( 'NONE', #36626, #14448, #26548 ) ;
#13375=CARTESIAN_POINT ( 'NONE',  ( -21.02145776008824996, -20.81426181449660717, 65.58453904424985126 ) ) ;
#13377=CARTESIAN_POINT ( 'NONE',  ( -10.83683315258895519, -12.44108567723101899, 57.32857332099802505 ) ) ;
#13379=PLANE ( 'NONE',  #21799 ) ;
#13382=ORIENTED_EDGE ( 'NONE', *, *, #240, .F. ) ;
#13384=CARTESIAN_POINT ( 'NONE',  ( -10.00731240618708462, -14.10555136595099945, 61.10316694600977172 ) ) ;
#13386=CARTESIAN_POINT ( 'NONE',  ( -12.32158608955787393, -9.943909642237139579, 60.57390139315987909 ) ) ;
#13390=CARTESIAN_POINT ( 'NONE',  ( -14.99706828511980916, -21.85287925006270626, 65.29092110561946072 ) ) ;
#13392=CARTESIAN_POINT ( 'NONE',  ( -22.28468842640967651, -19.91619389767071269, 65.98949666203347419 ) ) ;
#13393=CARTESIAN_POINT ( 'NONE',  ( -11.22844613476422282, -11.44458948612160221, 64.43409918096024569 ) ) ;
#13394=CARTESIAN_POINT ( 'NONE',  ( -21.52726260838264949, -9.076274878514672295, 70.13132538915753855 ) ) ;
#13395=CARTESIAN_POINT ( 'NONE',  ( -24.84449963183508459, -13.71944596863515464, 54.27966884056654351 ) ) ;
#13397=CARTESIAN_POINT ( 'NONE',  ( -20.18792757799173287, -7.890760935853403879, 73.97742500291465717 ) ) ;
#13398=DIRECTION ( 'NONE',  ( 2.403795750412638671E-06, 2.069898558110202305E-06, 0.9999999999949686913 ) ) ;
#13400=PLANE ( 'NONE',  #36729 ) ;
#13402=CARTESIAN_POINT ( 'NONE',  ( -13.87451016560426353, -8.259160067131549710, 74.29931037044663356 ) ) ;
#13403=( BOUNDED_SURFACE ( )  B_SPLINE_SURFACE ( 3, 1, ( 
 ( #13825, #25421 ),
 ( #33023, #21720 ),
 ( #18749, #28866 ),
 ( #17764, #10881 ),
 ( #10412, #7206 ),
 ( #18252, #33260 ),
 ( #33502, #6473 ) ),
 .UNSPECIFIED., .T., .F., .F. ) 
 B_SPLINE_SURFACE_WITH_KNOTS ( ( 4, 3, 4 ),
 ( 2, 2 ),
 ( 0.000000000000000000, 0.5000000000000000000, 1.000000000000000000 ),
 ( 0.000000000000000000, 1.000000000000000000 ),
 .UNSPECIFIED. ) 
 GEOMETRIC_REPRESENTATION_ITEM ( )  RATIONAL_B_SPLINE_SURFACE ( (
 ( 1.000000000000000000, 1.000000000000000000),
 ( 0.3333333333333335369, 0.3333333333333330373),
 ( 0.3333333333333335369, 0.3333333333333330373),
 ( 1.000000000000000000, 1.000000000000000000),
 ( 0.3333333333333333703, 0.3333333333333333703),
 ( 0.3333333333333333703, 0.3333333333333333703),
 ( 1.000000000000000000, 1.000000000000000000) ) ) 
 REPRESENTATION_ITEM ( '' )  SURFACE ( )  );
#13404=CARTESIAN_POINT ( 'NONE',  ( -14.22441497990486958, -8.081217732231424478, 67.44470516081543110 ) ) ;
#13406=ORIENTED_EDGE ( 'NONE', *, *, #385, .T. ) ;
#13407=CARTESIAN_POINT ( 'NONE',  ( -19.90583630033073703, -21.83377919204098205, 69.19128392610542733 ) ) ;
#13408=AXIS2_PLACEMENT_3D ( 'NONE', #21329, #10484, #43988 ) ;
#13409=ORIENTED_EDGE ( 'NONE', *, *, #16145, .F. ) ;
#13410=ADVANCED_FACE ( 'NONE', ( #4905 ), #5988, .T. ) ;
#13412=ORIENTED_EDGE ( 'NONE', *, *, #31188, .F. ) ;
#13413=ORIENTED_EDGE ( 'NONE', *, *, #1877, .T. ) ;
#13415=CARTESIAN_POINT ( 'NONE',  ( -18.75808540593367368, -7.479482988535800736, 70.54784884510475251 ) ) ;
#13416=CARTESIAN_POINT ( 'NONE',  ( -23.17271708368352634, -18.80356169263502508, 65.82389479710441549 ) ) ;
#13417=CARTESIAN_POINT ( 'NONE',  ( -10.99582121268164414, -11.91441617825094923, 74.70840195586961840 ) ) ;
#13420=ORIENTED_EDGE ( 'NONE', *, *, #18893, .T. ) ;
#13421=VERTEX_POINT ( 'NONE', #8350 ) ;
#13422=EDGE_CURVE ( 'NONE', #2461, #19324, #47950, .T. ) ;
#13425=CARTESIAN_POINT ( 'NONE',  ( -20.54786284059405688, -21.13826946137156781, 62.25904375309657723 ) ) ;
#13427=CARTESIAN_POINT ( 'NONE',  ( -11.75774308769439180, -19.00384223356172697, 71.98685884781657762 ) ) ;
#13429=B_SPLINE_CURVE_WITH_KNOTS ( 'NONE', 1,
 ( #18258, #11135 ),
 .UNSPECIFIED., .F., .F.,
 ( 2, 2 ),
 ( 0.000000000000000000, 1.000000000000000000 ),
 .UNSPECIFIED. ) ;
#13431=ADVANCED_FACE ( 'NONE', ( #32681 ), #16036, .T. ) ;
#13432=DIRECTION ( 'NONE',  ( 0.8743548079231423520, 0.4852872034802500623, -5.778319183281911236E-08 ) ) ;
#13434=CARTESIAN_POINT ( 'NONE',  ( -24.41553149706675896, -15.71832598455623398, 69.81835354388927328 ) ) ;
#13435=ORIENTED_EDGE ( 'NONE', *, *, #1762, .F. ) ;
#13436=CARTESIAN_POINT ( 'NONE',  ( -21.84079884060555088, -9.314189094968263305, 63.34153755726884327 ) ) ;
#13437=CARTESIAN_POINT ( 'NONE',  ( -22.40388508455290761, -9.889599135513202910, 73.70834494508456203 ) ) ;
#13438=CARTESIAN_POINT ( 'NONE',  ( -20.94465790601859467, -8.243431112063134947, 59.95629843672877257 ) ) ;
#13439=CARTESIAN_POINT ( 'NONE',  ( -22.48430662296557614, -20.27711519517875516, 65.81926411519917508 ) ) ;
#13440=AXIS2_PLACEMENT_3D ( 'NONE', #36110, #13458, #25295 ) ;
#13441=ORIENTED_EDGE ( 'NONE', *, *, #33523, .T. ) ;
#13443=( BOUNDED_SURFACE ( )  B_SPLINE_SURFACE ( 3, 1, ( 
 ( #13944, #29481 ),
 ( #28995, #22099 ),
 ( #10294, #21613 ),
 ( #7340, #32911 ),
 ( #44765, #36600 ),
 ( #34375, #11994 ),
 ( #41793, #26772 ) ),
 .UNSPECIFIED., .T., .F., .F. ) 
 B_SPLINE_SURFACE_WITH_KNOTS ( ( 4, 3, 4 ),
 ( 2, 2 ),
 ( 0.000000000000000000, 0.5000000000000000000, 1.000000000000000000 ),
 ( 0.000000000000000000, 1.000000000000000000 ),
 .UNSPECIFIED. ) 
 GEOMETRIC_REPRESENTATION_ITEM ( )  RATIONAL_B_SPLINE_SURFACE ( (
 ( 1.000000000000000000, 1.000000000000000000),
 ( 0.3333333333333335369, 0.3333333333333330373),
 ( 0.3333333333333335369, 0.3333333333333330373),
 ( 1.000000000000000000, 1.000000000000000000),
 ( 0.3333333333333333703, 0.3333333333333333703),
 ( 0.3333333333333333703, 0.3333333333333333703),
 ( 1.000000000000000000, 1.000000000000000000) ) ) 
 REPRESENTATION_ITEM ( '' )  SURFACE ( )  );
#13444=CARTESIAN_POINT ( 'NONE',  ( -23.03380641475053281, -9.905658051014942345, 66.65526928932193584 ) ) ;
#13445=CARTESIAN_POINT ( 'NONE',  ( -21.05063378830672249, -20.85509781831549958, 65.87894135078376223 ) ) ;
#13447=CARTESIAN_POINT ( 'NONE',  ( -21.92090081525502399, -20.24368645090660124, 62.53439249721748183 ) ) ;
#13450=CARTESIAN_POINT ( 'NONE',  ( -13.43921731646364925, -8.993429882417945720, 60.43950277494440826 ) ) ;
#13451=CARTESIAN_POINT ( 'NONE',  ( -9.975093131592752016, -14.93635113986534257, 74.98274190467411415 ) ) ;
#13455=CARTESIAN_POINT ( 'NONE',  ( -16.94618458872839994, -7.374472604449730184, 74.00372349603880195 ) ) ;
#13456=CARTESIAN_POINT ( 'NONE',  ( -22.68242755436546076, -10.18794509063480547, 70.02795139357954213 ) ) ;
#13458=DIRECTION ( 'NONE',  ( 0.8547111024021492032, 0.5191039697695417621, 7.472447835916433805E-08 ) ) ;
#13459=AXIS2_PLACEMENT_3D ( 'NONE', #39120, #8863, #38641 ) ;
#13461=CARTESIAN_POINT ( 'NONE',  ( -24.17966087195022595, -11.66819065304315117, 59.52589827039258097 ) ) ;
#13462=CARTESIAN_POINT ( 'NONE',  ( -10.10502314809590274, -16.20379097455708006, 68.09112436593052564 ) ) ;
#13463=VERTEX_POINT ( 'NONE', #28518 ) ;
#13464=LINE ( 'NONE', #25527, #26310 ) ;
#13465=( BOUNDED_SURFACE ( )  B_SPLINE_SURFACE ( 3, 1, ( 
 ( #48339, #17803 ),
 ( #47628, #37239 ),
 ( #18047, #43952 ),
 ( #40711, #21762 ),
 ( #22005, #21290 ),
 ( #7246, #3523 ),
 ( #26192, #22249 ) ),
 .UNSPECIFIED., .T., .F., .F. ) 
 B_SPLINE_SURFACE_WITH_KNOTS ( ( 4, 3, 4 ),
 ( 2, 2 ),
 ( 0.000000000000000000, 0.5000000000000000000, 1.000000000000000000 ),
 ( 0.000000000000000000, 1.000000000000000000 ),
 .UNSPECIFIED. ) 
 GEOMETRIC_REPRESENTATION_ITEM ( )  RATIONAL_B_SPLINE_SURFACE ( (
 ( 1.000000000000000000, 1.000000000000000000),
 ( 0.3333333333333335369, 0.3333333333333330373),
 ( 0.3333333333333335369, 0.3333333333333330373),
 ( 1.000000000000000000, 1.000000000000000000),
 ( 0.3333333333333333703, 0.3333333333333333703),
 ( 0.3333333333333333703, 0.3333333333333333703),
 ( 1.000000000000000000, 1.000000000000000000) ) ) 
 REPRESENTATION_ITEM ( '' )  SURFACE ( )  );
#13466=CARTESIAN_POINT ( 'NONE',  ( -12.04811195874215812, -10.23604714248314629, 60.71485379904431312 ) ) ;
#13467=EDGE_CURVE ( 'NONE', #5874, #37436, #8026, .T. ) ;
#13469=ORIENTED_EDGE ( 'NONE', *, *, #40896, .F. ) ;
#13470=CARTESIAN_POINT ( 'NONE',  ( -14.25466281091639686, -21.11075775427102030, 71.92607504337564706 ) ) ;
#13471=CARTESIAN_POINT ( 'NONE',  ( -10.83536383905390998, -17.31742040078651357, 64.62739380450889826 ) ) ;
#13472=CARTESIAN_POINT ( 'NONE',  ( -13.12744695462171407, -20.89546087334666069, 58.30296024829184631 ) ) ;
#13475=CARTESIAN_POINT ( 'NONE',  ( -12.62463572719220828, -19.97835019563962788, 72.10653721712196784 ) ) ;
#13476=CARTESIAN_POINT ( 'NONE',  ( -12.34924355347848035, -19.63124190001923708, 61.68062031358459052 ) ) ;
#13477=CARTESIAN_POINT ( 'NONE',  ( -12.80135276601915528, -20.13603490024450693, 68.22168825917964341 ) ) ;
#13478=CARTESIAN_POINT ( 'NONE',  ( -16.69790031487229243, -22.22389832459700898, 68.83527298580068532 ) ) ;
#13480=ORIENTED_EDGE ( 'NONE', *, *, #23328, .F. ) ;
#13481=EDGE_CURVE ( 'NONE', #15587, #41843, #21086, .T. ) ;
#13483=CARTESIAN_POINT ( 'NONE',  ( -24.82475139314513868, -15.66597149415626156, 73.11808456017074320 ) ) ;
#13488=CARTESIAN_POINT ( 'NONE',  ( -13.77528250856571645, -8.773395728905704516, 57.38456636527085664 ) ) ;
#13489=CARTESIAN_POINT ( 'NONE',  ( -20.88128654865952427, -21.40856141908871635, 58.68829242887799325 ) ) ;
#13490=EDGE_CURVE ( 'NONE', #1995, #1905, #23273, .T. ) ;
#13493=CARTESIAN_POINT ( 'NONE',  ( -18.11396434131172128, -21.77512919714542150, 65.34532159443909904 ) ) ;
#13496=CARTESIAN_POINT ( 'NONE',  ( -10.06841751317020872, -15.99566775706410482, 68.16423218926057359 ) ) ;
#13497=VECTOR ( 'NONE', #2782, 1000.000000000000000 ) ;
#13498=ORIENTED_EDGE ( 'NONE', *, *, #9521, .T. ) ;
#13501=CARTESIAN_POINT ( 'NONE',  ( -10.71342319306032564, -12.63657128681412800, 57.53677342537894646 ) ) ;
#13503=CARTESIAN_POINT ( 'NONE',  ( -14.85912063279003092, -7.814622674645058886, 56.95725833468153354 ) ) ;
#13504=DIRECTION ( 'NONE',  ( -0.1206048672277665601, 0.4306442452895119510, 0.8944271909999156334 ) ) ;
#13505=VERTEX_POINT ( 'NONE', #17882 ) ;
#13506=CARTESIAN_POINT ( 'NONE',  ( -20.95199127080493895, -20.85531950328408612, 65.58453983063536441 ) ) ;
#13509=CARTESIAN_POINT ( 'NONE',  ( -11.29876324976417123, -19.04990965798615221, 68.41027957156066464 ) ) ;
#13511=CARTESIAN_POINT ( 'NONE',  ( -18.50162202296811742, -21.72577595440482057, 72.28510940981611554 ) ) ;
#13512=CARTESIAN_POINT ( 'NONE',  ( -12.56051219783612538, -20.45271961000943861, 71.85007761110178137 ) ) ;
#13515=DIRECTION ( 'NONE',  ( 0.9997277805376393323, -0.02333162706040292980, -9.101776391673710038E-09 ) ) ;
#13516=EDGE_CURVE ( 'NONE', #11148, #47795, #9144, .T. ) ;
#13517=CARTESIAN_POINT ( 'NONE',  ( -24.47654139670598994, -14.67568567259567303, 66.48292734092783007 ) ) ;
#13518=CARTESIAN_POINT ( 'NONE',  ( -16.29760782986628342, -22.17363506107604110, 61.87072849596245305 ) ) ;
#13519=ORIENTED_EDGE ( 'NONE', *, *, #33107, .T. ) ;
#13521=LINE ( 'NONE', #4118, #39275 ) ;
#13522=CARTESIAN_POINT ( 'NONE',  ( -23.29871437377730814, -10.22635856038569990, 59.71548043103533843 ) ) ;
#13524=ORIENTED_EDGE ( 'NONE', *, *, #25240, .T. ) ;
#13527=VERTEX_POINT ( 'NONE', #6345 ) ;
#13528=CYLINDRICAL_SURFACE ( 'NONE', #21769, 0.1500000000000057399 ) ;
#13529=CARTESIAN_POINT ( 'NONE',  ( -19.27094073640459015, -21.56284686256307381, 62.18430764133905342 ) ) ;
#13532=CARTESIAN_POINT ( 'NONE',  ( -24.25002676646741051, -16.58726329047720327, 59.42332704469328064 ) ) ;
#13533=CARTESIAN_POINT ( 'NONE',  ( -16.01003035779492834, -7.894338788008341545, 70.75422978485266867 ) ) ;
#13535=CARTESIAN_POINT ( 'NONE',  ( -20.66848101912799862, -8.549761622307151754, 60.12653141481577990 ) ) ;
#13536=CARTESIAN_POINT ( 'NONE',  ( -13.06519849244570430, -8.767408624477393886, 64.01672394663651744 ) ) ;
#13538=B_SPLINE_CURVE_WITH_KNOTS ( 'NONE', 3,
 ( #11458, #26481, #30437, #23046, #7786, #41752, #19330, #37797, #34337, #45702 ),
 .UNSPECIFIED., .F., .F.,
 ( 4, 2, 2, 2, 4 ),
 ( 0.6272669072877815610, 0.7522669073072951740, 0.8772669073268086759, 1.002266907346322178, 1.127266907365835902 ),
 .UNSPECIFIED. ) ;
#13539=PLANE ( 'NONE',  #41347 ) ;
#13540=CARTESIAN_POINT ( 'NONE',  ( -10.48085350821551742, -13.91959267249018950, 57.44825035245948186 ) ) ;
#13541=EDGE_CURVE ( 'NONE', #9944, #32131, #16172, .T. ) ;
#13542=EDGE_LOOP ( 'NONE', ( #715, #30868, #4020, #20642, #33195 ) ) ;
#13545=CARTESIAN_POINT ( 'NONE',  ( -17.92858306677455715, -7.769287621248931686, 63.69489771833700331 ) ) ;
#13546=CARTESIAN_POINT ( 'NONE',  ( -22.53890663478593481, -10.03013475771905760, 70.08466598210137022 ) ) ;
#13547=CARTESIAN_POINT ( 'NONE',  ( -10.01440787728688520, -14.03439562150409969, 61.03325889150411143 ) ) ;
#13553=ORIENTED_EDGE ( 'NONE', *, *, #17654, .T. ) ;
#13554=CARTESIAN_POINT ( 'NONE',  ( -11.29219319990544079, -18.28864530752396433, 57.82186711835544912 ) ) ;
#13555=CARTESIAN_POINT ( 'NONE',  ( -24.46146587544552276, -14.38248120490118609, 66.46820668217904426 ) ) ;
#13557=EDGE_LOOP ( 'NONE', ( #29413, #23710 ) ) ;
#13559=EDGE_LOOP ( 'NONE', ( #2284, #40000 ) ) ;
#13560=CARTESIAN_POINT ( 'NONE',  ( -24.87417961795293664, -14.80849281899037884, 59.42795564617806292 ) ) ;
#13562=CARTESIAN_POINT ( 'NONE',  ( -10.41125311197691694, -14.08592688229884970, 60.91821313097471347 ) ) ;
#13563=ORIENTED_EDGE ( 'NONE', *, *, #31060, .F. ) ;
#13565=CARTESIAN_POINT ( 'NONE',  ( -20.18028783932825476, -21.73079638842835948, 72.56512126044646038 ) ) ;
#13567=ADVANCED_FACE ( 'NONE', ( #22330 ), #29720, .T. ) ;
#13568=CARTESIAN_POINT ( 'NONE',  ( -20.01548349435434204, -21.36955285994420706, 69.14302430453618342 ) ) ;
#13570=CARTESIAN_POINT ( 'NONE',  ( -19.15858190565953123, -8.027436205280443104, 60.18766296741227961 ) ) ;
#13573=CARTESIAN_POINT ( 'NONE',  ( -23.46260529264823802, -11.17067950781535579, 73.36193301757424479 ) ) ;
#13574=CYLINDRICAL_SURFACE ( 'NONE', #18817, 0.1499999999999991618 ) ;
#13575=DIRECTION ( 'NONE',  ( -1.184681380772507928E-05, -1.827615836447136132E-06, 0.9999999999281563579 ) ) ;
#13581=CARTESIAN_POINT ( 'NONE',  ( -24.43827367352892210, -15.52193379869737377, 73.28831629023289906 ) ) ;
#13582=ORIENTED_EDGE ( 'NONE', *, *, #20851, .F. ) ;
#13583=CARTESIAN_POINT ( 'NONE',  ( -23.49605051889219709, -11.22618518380361152, 73.37665428612797314 ) ) ;
#13584=CARTESIAN_POINT ( 'NONE',  ( -10.66160677810301038, -13.00123309306513697, 67.73832347541063825 ) ) ;
#13585=CARTESIAN_POINT ( 'NONE',  ( -14.05371499411350023, -21.00138273984457982, 72.22607703579409133 ) ) ;
#13587=CARTESIAN_POINT ( 'NONE',  ( -11.82205746763155041, -9.897907871467767293, 64.07268414109491061 ) ) ;
#13589=( BOUNDED_SURFACE ( )  B_SPLINE_SURFACE ( 3, 1, ( 
 ( #12640, #26939 ),
 ( #27662, #5256 ),
 ( #42927, #23979 ),
 ( #9199, #34301 ),
 ( #24218, #25420 ),
 ( #35757, #9920 ),
 ( #2282, #28147 ) ),
 .UNSPECIFIED., .T., .F., .F. ) 
 B_SPLINE_SURFACE_WITH_KNOTS ( ( 4, 3, 4 ),
 ( 2, 2 ),
 ( 0.000000000000000000, 0.5000000000000000000, 1.000000000000000000 ),
 ( 0.000000000000000000, 1.000000000000000000 ),
 .UNSPECIFIED. ) 
 GEOMETRIC_REPRESENTATION_ITEM ( )  RATIONAL_B_SPLINE_SURFACE ( (
 ( 1.000000000000000000, 1.000000000000000000),
 ( 0.3333333333333335369, 0.3333333333333330373),
 ( 0.3333333333333335369, 0.3333333333333330373),
 ( 1.000000000000000000, 1.000000000000000000),
 ( 0.3333333333333333703, 0.3333333333333333703),
 ( 0.3333333333333333703, 0.3333333333333333703),
 ( 1.000000000000000000, 1.000000000000000000) ) ) 
 REPRESENTATION_ITEM ( '' )  SURFACE ( )  );
#13594=CARTESIAN_POINT ( 'NONE',  ( -14.87342360121920315, -7.809316307502902177, 56.97283086062095236 ) ) ;
#13597=CARTESIAN_POINT ( 'NONE',  ( -13.24891125353284949, -8.638936510823443271, 60.56233416867657127 ) ) ;
#13598=CARTESIAN_POINT ( 'NONE',  ( -22.91296630721855720, -15.15889098507616950, 54.07175714974879099 ) ) ;
#13600=( BOUNDED_CURVE ( )  B_SPLINE_CURVE ( 3, ( #7676, #38408, #45106, #37933 ),
 .UNSPECIFIED., .F., .F. ) 
 B_SPLINE_CURVE_WITH_KNOTS ( ( 4, 4 ),
 ( 0.9074455897393690629, 1.000000000000000000 ),
 .UNSPECIFIED. ) 
 CURVE ( )  GEOMETRIC_REPRESENTATION_ITEM ( )  RATIONAL_B_SPLINE_CURVE ( ( 0.6983129098261066092, 0.7760317562607099706, 0.8765941196520077305, 1.000000000000000000 ) ) 
 REPRESENTATION_ITEM ( '' )  );
#13601=DIRECTION ( 'NONE',  ( 7.652304183832323392E-06, 2.165757503891338892E-06, 0.9999999999683758523 ) ) ;
#13602=( BOUNDED_CURVE ( )  B_SPLINE_CURVE ( 3, ( #7018, #48132, #6772, #37269 ),
 .UNSPECIFIED., .F., .F. ) 
 B_SPLINE_CURVE_WITH_KNOTS ( ( 4, 4 ),
 ( 1.570796326794896780, 1.780235837034217505 ),
 .UNSPECIFIED. ) 
 CURVE ( )  GEOMETRIC_REPRESENTATION_ITEM ( )  RATIONAL_B_SPLINE_CURVE ( ( 1.000000000000000000, 0.9963479302455154896, 0.9963479302455154896, 1.000000000000000000 ) ) 
 REPRESENTATION_ITEM ( '' )  );
#13606=EDGE_CURVE ( 'NONE', #3011, #32538, #13812, .T. ) ;
#13607=DIRECTION ( 'NONE',  ( -0.5652317888644005084, -0.8249321334856241084, 7.911723905267715079E-08 ) ) ;
#13608=VECTOR ( 'NONE', #4811, 1000.000000000000114 ) ;
#13609=EDGE_CURVE ( 'NONE', #32577, #23164, #26120, .T. ) ;
#13610=CARTESIAN_POINT ( 'NONE',  ( -24.03066126544255354, -17.12310022511010388, 69.48627920760770849 ) ) ;
#13611=EDGE_CURVE ( 'NONE', #14012, #14322, #42648, .T. ) ;
#13612=( BOUNDED_CURVE ( )  B_SPLINE_CURVE ( 3, ( #24016, #28433, #9724, #24742 ),
 .UNSPECIFIED., .F., .F. ) 
 B_SPLINE_CURVE_WITH_KNOTS ( ( 4, 4 ),
 ( 0.000000000000000000, 0.4074455897279072869 ),
 .UNSPECIFIED. ) 
 CURVE ( )  GEOMETRIC_REPRESENTATION_ITEM ( )  RATIONAL_B_SPLINE_CURVE ( ( 1.000000000000000000, 0.4567392136965981453, 0.3561768502956821347, 0.6983129097972519128 ) ) 
 REPRESENTATION_ITEM ( '' )  );
#13613=B_SPLINE_CURVE_WITH_KNOTS ( 'NONE', 3,
 ( #7426, #25401, #37424, #18727, #25882, #32774, #14511, #40412, #6683, #48044 ),
 .UNSPECIFIED., .F., .F.,
 ( 4, 2, 2, 2, 4 ),
 ( 0.6272669072877967711, 0.7522669073073094959, 0.8772669073268222206, 1.002266907346335056, 1.127266907365847670 ),
 .UNSPECIFIED. ) ;
#13614=CARTESIAN_POINT ( 'NONE',  ( -15.87557863975121464, -7.931372594209567417, 67.14007279017359053 ) ) ;
#13615=CARTESIAN_POINT ( 'NONE',  ( -24.43362379028604536, -14.05489247495133753, 73.12271507725591846 ) ) ;
#13617=CARTESIAN_POINT ( 'NONE',  ( -13.18362795047878144, -8.683667697493742565, 60.62445659250467145 ) ) ;
#13618=CARTESIAN_POINT ( 'NONE',  ( -12.41315146567208139, -9.850077947585075933, 57.08935532239182464 ) ) ;
#13619=EDGE_LOOP ( 'NONE', ( #30892, #30914, #47739, #43239, #38796 ) ) ;
#13620=DIRECTION ( 'NONE',  ( 6.816999858124113439E-06, 9.113320815582587851E-06, 0.9999999999352379154 ) ) ;
#13621=ADVANCED_FACE ( 'NONE', ( #7570 ), #23079, .T. ) ;
#13623=ADVANCED_FACE ( 'NONE', ( #190 ), #41220, .T. ) ;
#13626=CARTESIAN_POINT ( 'NONE',  ( -11.39216336840796373, -18.45920852072106300, 61.29182966166492719 ) ) ;
#13627=ADVANCED_FACE ( 'NONE', ( #7080 ), #11492, .T. ) ;
#13629=EDGE_CURVE ( 'NONE', #13641, #4739, #44117, .T. ) ;
#13630=CARTESIAN_POINT ( 'NONE',  ( -13.92250310594754303, -20.92831230454754987, 68.75065321223313219 ) ) ;
#13632=CARTESIAN_POINT ( 'NONE',  ( -10.74628672884880132, -17.07053172313825939, 61.17215199736627795 ) ) ;
#13633=CARTESIAN_POINT ( 'NONE',  ( -11.09396220476197037, -17.79742230095041577, 71.75821477588401365 ) ) ;
#13635=CARTESIAN_POINT ( 'NONE',  ( -10.40277084706750621, -15.44444119821074679, 57.86792809062919218 ) ) ;
#13636=CARTESIAN_POINT ( 'NONE',  ( -24.55871690389112061, -12.66422819002857558, 69.88747705124970366 ) ) ;
#13637=CARTESIAN_POINT ( 'NONE',  ( -19.75993683595673289, -21.46115599289353781, 68.94042252247996316 ) ) ;
#13638=CARTESIAN_POINT ( 'NONE',  ( -10.78271008354229465, -17.17492318853433986, 61.45183338995374811 ) ) ;
#13640=FACE_OUTER_BOUND ( 'NONE', #28559, .T. ) ;
#13641=VERTEX_POINT ( 'NONE', #11010 ) ;
#13642=CARTESIAN_POINT ( 'NONE',  ( -11.10300703817161327, -10.86615712478015539, 57.39398594787093089 ) ) ;
#13643=CARTESIAN_POINT ( 'NONE',  ( -13.30358754779367025, -20.46953698742588301, 58.11820441233432177 ) ) ;
#13644=VERTEX_POINT ( 'NONE', #48672 ) ;
#13646=ORIENTED_EDGE ( 'NONE', *, *, #5072, .F. ) ;
#13647=EDGE_CURVE ( 'NONE', #19673, #8437, #34133, .T. ) ;
#13648=ORIENTED_EDGE ( 'NONE', *, *, #23952, .T. ) ;
#13649=ORIENTED_EDGE ( 'NONE', *, *, #24754, .F. ) ;
#13650=FACE_OUTER_BOUND ( 'NONE', #12474, .T. ) ;
#13651=CARTESIAN_POINT ( 'NONE',  ( -22.66727108289645543, -10.09628893573625064, 70.01178520457129650 ) ) ;
#13652=B_SPLINE_CURVE_WITH_KNOTS ( 'NONE', 1,
 ( #33327, #26707 ),
 .UNSPECIFIED., .F., .F.,
 ( 2, 2 ),
 ( 0.000000000000000000, 1.000000000000000000 ),
 .UNSPECIFIED. ) ;
#13655=ORIENTED_EDGE ( 'NONE', *, *, #2791, .T. ) ;
#13657=EDGE_CURVE ( 'NONE', #16737, #11137, #17913, .T. ) ;
#13658=EDGE_CURVE ( 'NONE', #20248, #44249, #8295, .T. ) ;
#13661=VECTOR ( 'NONE', #12928, 999.9999999999998863 ) ;
#13663=FACE_OUTER_BOUND ( 'NONE', #21185, .T. ) ;
#13666=B_SPLINE_CURVE_WITH_KNOTS ( 'NONE', 3,
 ( #1080, #8241, #12648, #12883, #8472, #38988, #1311, #31614, #46392, #34560 ),
 .UNSPECIFIED., .F., .F.,
 ( 4, 2, 2, 2, 4 ),
 ( 0.1272669073657735350, 0.2522669073462773248, 0.3772669073267810314, 0.5022669073072848489, 0.6272669072877885554 ),
 .UNSPECIFIED. ) ;
#13667=ORIENTED_EDGE ( 'NONE', *, *, #4646, .F. ) ;
#13668=CARTESIAN_POINT ( 'NONE',  ( -12.41315160057549960, -9.850077812919039388, 57.23935532239169532 ) ) ;
#13670=ORIENTED_EDGE ( 'NONE', *, *, #24110, .T. ) ;
#13671=FACE_OUTER_BOUND ( 'NONE', #15137, .T. ) ;
#13674=ADVANCED_FACE ( 'NONE', ( #26999 ), #5711, .T. ) ;
#13675=CARTESIAN_POINT ( 'NONE',  ( -19.24829632005326019, -7.991050106228435368, 67.04504941182814548 ) ) ;
#13678=( BOUNDED_SURFACE ( )  B_SPLINE_SURFACE ( 3, 1, ( 
 ( #15250, #30314 ),
 ( #19943, #46773 ),
 ( #43072, #4681 ),
 ( #30797, #19704 ),
 ( #12301, #12070 ),
 ( #28046, #12548 ),
 ( #38892, #19451 ) ),
 .UNSPECIFIED., .T., .F., .F. ) 
 B_SPLINE_SURFACE_WITH_KNOTS ( ( 4, 3, 4 ),
 ( 2, 2 ),
 ( 0.000000000000000000, 0.5000000000000000000, 1.000000000000000000 ),
 ( 0.000000000000000000, 1.000000000000000000 ),
 .UNSPECIFIED. ) 
 GEOMETRIC_REPRESENTATION_ITEM ( )  RATIONAL_B_SPLINE_SURFACE ( (
 ( 1.000000000000000000, 1.000000000000000000),
 ( 0.3333333333333335369, 0.3333333333333330373),
 ( 0.3333333333333335369, 0.3333333333333330373),
 ( 1.000000000000000000, 1.000000000000000000),
 ( 0.3333333333333333703, 0.3333333333333333703),
 ( 0.3333333333333333703, 0.3333333333333333703),
 ( 1.000000000000000000, 1.000000000000000000) ) ) 
 REPRESENTATION_ITEM ( '' )  SURFACE ( )  );
#13680=CARTESIAN_POINT ( 'NONE',  ( -10.44157451558128358, -15.80814149404359981, 68.06948097726898084 ) ) ;
#13681=ORIENTED_EDGE ( 'NONE', *, *, #21011, .F. ) ;
#13682=DIRECTION ( 'NONE',  ( -4.734277553319870270E-07, 1.363385191780837012E-06, 0.9999999999989586108 ) ) ;
#13683=FACE_OUTER_BOUND ( 'NONE', #43141, .T. ) ;
#13684=ORIENTED_EDGE ( 'NONE', *, *, #14822, .T. ) ;
#13685=CARTESIAN_POINT ( 'NONE',  ( -15.03427660820159950, -21.44211488324610926, 65.12068745241758450 ) ) ;
#13687=ADVANCED_FACE ( 'NONE', ( #16387 ), #12222, .T. ) ;
#13688=CARTESIAN_POINT ( 'NONE',  ( -9.975950761882481643, -15.00625170120774321, 74.91123542948268721 ) ) ;
#13689=B_SPLINE_CURVE_WITH_KNOTS ( 'NONE', 1,
 ( #42727, #13384 ),
 .UNSPECIFIED., .F., .F.,
 ( 2, 2 ),
 ( 0.000000000000000000, 1.000000000000000000 ),
 .UNSPECIFIED. ) ;
#13691=DIRECTION ( 'NONE',  ( 6.291559634385637730E-07, -1.530398238691524640E-06, 0.9999999999986310950 ) ) ;
#13692=PLANE ( 'NONE',  #42835 ) ;
#13695=EDGE_LOOP ( 'NONE', ( #42580, #24740 ) ) ;
#13697=CARTESIAN_POINT ( 'NONE',  ( -19.04725004413522882, -7.538051835607980422, 67.07884570001746738 ) ) ;
#13698=DIRECTION ( 'NONE',  ( -0.9345716196833626643, 0.3557750520798445559, 2.412542607589989711E-09 ) ) ;
#13699=ORIENTED_EDGE ( 'NONE', *, *, #18088, .F. ) ;
#13700=CARTESIAN_POINT ( 'NONE',  ( -23.97576963128622651, -17.42270779624378108, 62.47360993958987763 ) ) ;
#13702=CARTESIAN_POINT ( 'NONE',  ( -24.25486363958986757, -13.06355980472538292, 63.11792038370487035 ) ) ;
#13705=ORIENTED_EDGE ( 'NONE', *, *, #30019, .T. ) ;
#13706=ORIENTED_EDGE ( 'NONE', *, *, #22841, .F. ) ;
#13708=CARTESIAN_POINT ( 'NONE',  ( -15.55273166284925246, -8.063985742959628666, 70.71875758216351926 ) ) ;
#13709=CARTESIAN_POINT ( 'NONE',  ( -10.02491569571532715, -15.67798101985274073, 61.23800248293585469 ) ) ;
#13710=CARTESIAN_POINT ( 'NONE',  ( -23.42532328873747005, -19.22384396101403681, 62.46911485589509994 ) ) ;
#13712=CARTESIAN_POINT ( 'NONE',  ( -11.33476867595667770, -19.10151316506851416, 68.40185013497388411 ) ) ;
#13713=CARTESIAN_POINT ( 'NONE',  ( -13.03244867582903943, -9.358201799085602346, 67.48828719236378504 ) ) ;
#13714=CARTESIAN_POINT ( 'NONE',  ( -16.71219879347879100, -22.22520166962337740, 68.81065243885818461 ) ) ;
#13715=ORIENTED_EDGE ( 'NONE', *, *, #33182, .T. ) ;
#13716=EDGE_LOOP ( 'NONE', ( #45980, #38731 ) ) ;
#13718=CARTESIAN_POINT ( 'NONE',  ( -19.85066507975247063, -8.243252523173408619, 73.91199902895934315 ) ) ;
#13719=CARTESIAN_POINT ( 'NONE',  ( -21.36489355414517632, -8.963473290115421932, 73.90128753234840531 ) ) ;
#13720=CARTESIAN_POINT ( 'NONE',  ( -10.97672171568423671, -17.53854784295387503, 71.79547974970954272 ) ) ;
#13721=DIRECTION ( 'NONE',  ( 3.549360974554993999E-17, -6.371834667797928663E-18, -1.000000000000000000 ) ) ;
#13724=B_SPLINE_CURVE_WITH_KNOTS ( 'NONE', 3,
 ( #25434, #2296, #17779, #17303, #40445, #32353, #47372, #28648, #39971, #32807 ),
 .UNSPECIFIED., .F., .F.,
 ( 4, 2, 2, 2, 4 ),
 ( 0.000000000000000000, 0.2500000000000000000, 0.5000000000000000000, 0.7500000000000000000, 1.000000000000000000 ),
 .UNSPECIFIED. ) ;
#13725=CARTESIAN_POINT ( 'NONE',  ( -12.66750632023469514, -20.01285372994693290, 68.63657439664891058 ) ) ;
#13726=CARTESIAN_POINT ( 'NONE',  ( -14.42683419600288985, -8.428067575814651491, 67.55975083869262221 ) ) ;
#13727=CARTESIAN_POINT ( 'NONE',  ( -11.17067368074822120, -18.85886670308036273, 64.88673749957456494 ) ) ;
#13728=( BOUNDED_CURVE ( )  B_SPLINE_CURVE ( 3, ( #5895, #10555, #18167, #29020 ),
 .UNSPECIFIED., .F., .F. ) 
 B_SPLINE_CURVE_WITH_KNOTS ( ( 4, 4 ),
 ( 0.4074455897393691739, 0.5000000000000000000 ),
 .UNSPECIFIED. ) 
 CURVE ( )  GEOMETRIC_REPRESENTATION_ITEM ( )  RATIONAL_B_SPLINE_CURVE ( ( 0.6983129098260982826, 0.7760317562607088604, 0.8765941196520110612, 1.000000000000009548 ) ) 
 REPRESENTATION_ITEM ( '' )  );
#13729=ORIENTED_EDGE ( 'NONE', *, *, #27618, .F. ) ;
#13730=CARTESIAN_POINT ( 'NONE',  ( -10.59456938016190541, -16.34492539027162650, 71.52038324560433580 ) ) ;
#13731=CARTESIAN_POINT ( 'NONE',  ( -12.73501256528857617, -9.611849834345010279, 74.42808954951277656 ) ) ;
#13732=ADVANCED_FACE ( 'NONE', ( #4591 ), #22378, .T. ) ;
#13735=CARTESIAN_POINT ( 'NONE',  ( -12.14425506381237341, -10.13739722748950811, 64.32914326607962607 ) ) ;
#13736=ORIENTED_EDGE ( 'NONE', *, *, #9551, .T. ) ;
#13738=( BOUNDED_CURVE ( )  B_SPLINE_CURVE ( 3, ( #8137, #46534, #20167, #30546 ),
 .UNSPECIFIED., .F., .F. ) 
 B_SPLINE_CURVE_WITH_KNOTS ( ( 4, 4 ),
 ( 0.000000000000000000, 0.4074455897393669535 ),
 .UNSPECIFIED. ) 
 CURVE ( )  GEOMETRIC_REPRESENTATION_ITEM ( )  RATIONAL_B_SPLINE_CURVE ( ( 1.000000000000000000, 0.4567392136813293035, 0.3561768502900293232, 0.6983129098261000589 ) ) 
 REPRESENTATION_ITEM ( '' )  );
#13739=ORIENTED_EDGE ( 'NONE', *, *, #27206, .F. ) ;
#13741=EDGE_CURVE ( 'NONE', #12408, #47772, #4842, .T. ) ;
#13743=CARTESIAN_POINT ( 'NONE',  ( -19.25584931519960463, -7.587732789139183254, 63.57055898488500389 ) ) ;
#13750=EDGE_CURVE ( 'NONE', #27631, #14412, #42812, .T. ) ;
#13752=CARTESIAN_POINT ( 'NONE',  ( -20.10030204730919223, -21.76202525863913451, 72.51983304728076973 ) ) ;
#13753=VERTEX_POINT ( 'NONE', #7455 ) ;
#13754=CARTESIAN_POINT ( 'NONE',  ( -13.46024608985845994, -21.11736968229694611, 65.12595554403661424 ) ) ;
#13755=CARTESIAN_POINT ( 'NONE',  ( -17.08147026401541524, -7.366339275741904835, 70.60380589010705421 ) ) ;
#13757=CARTESIAN_POINT ( 'NONE',  ( -23.34189317711797429, -10.28335673940103590, 59.64557479084083269 ) ) ;
#13758=EDGE_CURVE ( 'NONE', #13276, #22004, #47425, .T. ) ;
#13760=ORIENTED_EDGE ( 'NONE', *, *, #30299, .F. ) ;
#13762=CARTESIAN_POINT ( 'NONE',  ( -23.81387519531508445, -18.64000541993103610, 72.88555444462819821 ) ) ;
#13763=CARTESIAN_POINT ( 'NONE',  ( -24.23813412381375088, -12.99935709875259526, 66.31718868320673721 ) ) ;
#13765=CARTESIAN_POINT ( 'NONE',  ( -20.73640204290083489, -8.136034802137729116, 63.51132713554439846 ) ) ;
#13767=CARTESIAN_POINT ( 'NONE',  ( -23.59778322581706789, -11.38860327479983603, 63.10785482661193413 ) ) ;
#13768=CARTESIAN_POINT ( 'NONE',  ( -13.76968405657925487, -21.30219918833402204, 72.11263056552699879 ) ) ;
#13769=CARTESIAN_POINT ( 'NONE',  ( -12.41631181157024066, -9.915882637312337877, 60.66991079537774567 ) ) ;
#13770=AXIS2_PLACEMENT_3D ( 'NONE', #32400, #47419, #20824 ) ;
#13771=EDGE_LOOP ( 'NONE', ( #33078, #9023 ) ) ;
#13772=FACE_OUTER_BOUND ( 'NONE', #17064, .T. ) ;
#13773=VECTOR ( 'NONE', #5080, 1000.000000000000341 ) ;
#13774=CARTESIAN_POINT ( 'NONE',  ( -19.24190786459753610, -7.584296138276666710, 63.54593947706258206 ) ) ;
#13775=CARTESIAN_POINT ( 'NONE',  ( -24.47432067347917695, -14.77756146504815327, 59.52828185648635184 ) ) ;
#13776=DIRECTION ( 'NONE',  ( -0.8507615431891570879, 0.5255518971808580408, 6.876821558984483597E-08 ) ) ;
#13777=EDGE_LOOP ( 'NONE', ( #16716, #19045, #40274, #26511, #29823 ) ) ;
#13778=ORIENTED_EDGE ( 'NONE', *, *, #28776, .T. ) ;
#13779=CARTESIAN_POINT ( 'NONE',  ( -24.47999924015074669, -14.97998867148549351, 62.85729180369179403 ) ) ;
#13782=ORIENTED_EDGE ( 'NONE', *, *, #28710, .F. ) ;
#13784=CARTESIAN_POINT ( 'NONE',  ( -23.75797280549784318, -17.78947120508452429, 59.30378417803890301 ) ) ;
#13785=EDGE_CURVE ( 'NONE', #16929, #15929, #15746, .T. ) ;
#13786=ORIENTED_EDGE ( 'NONE', *, *, #31263, .T. ) ;
#13788=CARTESIAN_POINT ( 'NONE',  ( -12.23220172533775063, -19.57856247689574403, 57.92682373937842044 ) ) ;
#13789=CARTESIAN_POINT ( 'NONE',  ( -22.98865756656685022, -9.855479763439479512, 70.12683098403445570 ) ) ;
#13790=ORIENTED_EDGE ( 'NONE', *, *, #25703, .T. ) ;
#13791=DIRECTION ( 'NONE',  ( -0.4468359692653126602, 0.01837434545035235636, 0.8944271909999157444 ) ) ;
#13792=AXIS2_PLACEMENT_3D ( 'NONE', #40382, #21673, #40865 ) ;
#13793=ORIENTED_EDGE ( 'NONE', *, *, #26722, .F. ) ;
#13796=DIRECTION ( 'NONE',  ( -1.006957036272130273E-05, 6.253991260048532259E-06, 0.9999999999297456421 ) ) ;
#13798=LINE ( 'NONE', #48276, #21515 ) ;
#13799=DIRECTION ( 'NONE',  ( 0.5589780652556124441, -0.8291824422665291516, 7.938832475108296738E-08 ) ) ;
#13802=EDGE_CURVE ( 'NONE', #44542, #43576, #7588, .T. ) ;
#13803=CARTESIAN_POINT ( 'NONE',  ( -14.57821615407322291, -8.355182602927943236, 60.52816311995014331 ) ) ;
#13805=CARTESIAN_POINT ( 'NONE',  ( -19.14472750395669465, -8.023971105352707411, 60.06978972629352853 ) ) ;
#13808=CARTESIAN_POINT ( 'NONE',  ( -24.67073143307269589, -13.07968201635391914, 62.97230848449754603 ) ) ;
#13809=CARTESIAN_POINT ( 'NONE',  ( -22.69143476767070311, -20.07792998486722880, 69.29605258592428640 ) ) ;
#13810=CARTESIAN_POINT ( 'NONE',  ( -13.35818949714929360, -21.05197827947291955, 61.70141596610112344 ) ) ;
#13811=EDGE_CURVE ( 'NONE', #47972, #19236, #30888, .T. ) ;
#13812=B_SPLINE_CURVE_WITH_KNOTS ( 'NONE', 1,
 ( #37573, #33896 ),
 .UNSPECIFIED., .F., .F.,
 ( 2, 2 ),
 ( 0.000000000000000000, 1.000000000000000000 ),
 .UNSPECIFIED. ) ;
#13813=CARTESIAN_POINT ( 'NONE',  ( -10.81980138738203223, -12.48416433311569129, 60.98780598612082571 ) ) ;
#13816=EDGE_LOOP ( 'NONE', ( #16952, #13917 ) ) ;
#13817=CARTESIAN_POINT ( 'NONE',  ( -21.63336539757928634, -9.153348366551478321, 66.94677872351418557 ) ) ;
#13818=CARTESIAN_POINT ( 'NONE',  ( -24.84033948030421968, -15.52542097194404569, 73.11648385888869939 ) ) ;
#13820=CARTESIAN_POINT ( 'NONE',  ( -15.49415775405465645, -8.028509947901662613, 74.37985659017797957 ) ) ;
#13821=CARTESIAN_POINT ( 'NONE',  ( -17.65006842549283306, -20.30456235612523841, 53.49899999999994549 ) ) ;
#13822=CARTESIAN_POINT ( 'NONE',  ( -12.66943518016813996, -20.01945279446396952, 65.07494931179483899 ) ) ;
#13823=CARTESIAN_POINT ( 'NONE',  ( -14.58890586778976584, -8.408938977662566927, 63.78978847347087111 ) ) ;
#13824=CARTESIAN_POINT ( 'NONE',  ( -19.62595585458452163, -8.103479577873935469, 60.10526007146324901 ) ) ;
#13825=CARTESIAN_POINT ( 'NONE',  ( -21.94242186726961208, -9.397052521110282441, 60.00699132926281010 ) ) ;
#13826=ADVANCED_FACE ( 'NONE', ( #13650 ), #2821, .F. ) ;
#13827=DIRECTION ( 'NONE',  ( 0.4439273849576848563, 0.8960627639203804229, 1.004702157337987228E-17 ) ) ;
#13828=FACE_OUTER_BOUND ( 'NONE', #25677, .T. ) ;
#13830=CARTESIAN_POINT ( 'NONE',  ( -11.46167752593530942, -19.27618730729482266, 71.80873093914522087 ) ) ;
#13831=CARTESIAN_POINT ( 'NONE',  ( -20.95545100651803594, -20.91135505560678354, 65.59926067308570907 ) ) ;
#13832=EDGE_LOOP ( 'NONE', ( #3639, #15910, #11007, #17724, #29496 ) ) ;
#13833=DIRECTION ( 'NONE',  ( 0.8394943004421988597, -0.3114503813636535501, 0.4452504682462422592 ) ) ;
#13834=CARTESIAN_POINT ( 'NONE',  ( -11.54077142481382268, -18.60227312804761723, 61.34998797001519932 ) ) ;
#13835=CARTESIAN_POINT ( 'NONE',  ( -10.40127070788197017, -12.32249518151173895, 57.51352764219546998 ) ) ;
#13836=CARTESIAN_POINT ( 'NONE',  ( -24.18037300165767434, -17.94870813986570113, 59.18873840842728384 ) ) ;
#13837=CARTESIAN_POINT ( 'NONE',  ( -10.73343087151675590, -11.53221169192942597, 71.34506790255136366 ) ) ;
#13838=ORIENTED_EDGE ( 'NONE', *, *, #31669, .F. ) ;
#13839=AXIS2_PLACEMENT_3D ( 'NONE', #1158, #31203, #5108 ) ;
#13841=AXIS2_PLACEMENT_3D ( 'NONE', #14798, #19996, #23212 ) ;
#13843=CARTESIAN_POINT ( 'NONE',  ( -24.01131036459814183, -17.17762702439318900, 69.42842272742100818 ) ) ;
#13845=B_SPLINE_CURVE_WITH_KNOTS ( 'NONE', 1,
 ( #11324, #27067 ),
 .UNSPECIFIED., .F., .F.,
 ( 2, 2 ),
 ( 0.000000000000000000, 1.000000000000000000 ),
 .UNSPECIFIED. ) ;
#13846=CARTESIAN_POINT ( 'NONE',  ( -24.61986767591916347, -12.87896034533829237, 66.44213403754470448 ) ) ;
#13847=CARTESIAN_POINT ( 'NONE',  ( -15.99552465959851233, -21.71601670177824417, 58.70074462513652236 ) ) ;
#13848=ORIENTED_EDGE ( 'NONE', *, *, #47434, .F. ) ;
#13849=CARTESIAN_POINT ( 'NONE',  ( -11.00778200170179133, -11.02323315455921815, 60.77862143039379106 ) ) ;
#13850=CARTESIAN_POINT ( 'NONE',  ( -21.13453391143521287, -20.81317186429504673, 62.27038425631170782 ) ) ;
#13851=B_SPLINE_CURVE_WITH_KNOTS ( 'NONE', 3,
 ( #17407, #40311, #32439, #47462, #13697, #43772, #10026, #44264, #25052, #2633 ),
 .UNSPECIFIED., .F., .F.,
 ( 4, 2, 2, 2, 4 ),
 ( 0.1272669073658256045, 0.2522669073463177924, 0.3772669073268100082, 0.5022669073073021684, 0.6272669072877943286 ),
 .UNSPECIFIED. ) ;
#13852=ORIENTED_EDGE ( 'NONE', *, *, #39426, .T. ) ;
#13853=CARTESIAN_POINT ( 'NONE',  ( -18.92057448382017526, -7.919863665830076727, 67.20071783788056052 ) ) ;
#13854=CARTESIAN_POINT ( 'NONE',  ( -18.31357640787765462, -21.80286941108919763, 68.81514702304139064 ) ) ;
#13856=CARTESIAN_POINT ( 'NONE',  ( -11.08846142298070880, -18.82290330472913098, 54.27966884056657904 ) ) ;
#13857=LINE ( 'NONE', #36511, #37556 ) ;
#13859=CARTESIAN_POINT ( 'NONE',  ( -11.94599784085152372, -19.85827745584209580, 58.02658751082835664 ) ) ;
#13860=EDGE_CURVE ( 'NONE', #17712, #43339, #48529, .T. ) ;
#13861=CARTESIAN_POINT ( 'NONE',  ( -24.39459507417318562, -17.43899346222085711, 69.66985698250167047 ) ) ;
#13862=( BOUNDED_CURVE ( )  B_SPLINE_CURVE ( 3, ( #41349, #26584, #27065, #37646 ),
 .UNSPECIFIED., .F., .F. ) 
 B_SPLINE_CURVE_WITH_KNOTS ( ( 4, 4 ),
 ( 0.4074455897393670645, 0.5000000000000000000 ),
 .UNSPECIFIED. ) 
 CURVE ( )  GEOMETRIC_REPRESENTATION_ITEM ( )  RATIONAL_B_SPLINE_CURVE ( ( 0.6983129098260947298, 0.7760317562606947606, 0.8765941196519950740, 0.9999999999999923395 ) ) 
 REPRESENTATION_ITEM ( '' )  );
#13864=CARTESIAN_POINT ( 'NONE',  ( -22.19982498210932675, -20.00606685933203366, 58.92009921125114857 ) ) ;
#13865=ORIENTED_EDGE ( 'NONE', *, *, #41740, .F. ) ;
#13866=CARTESIAN_POINT ( 'NONE',  ( -22.38280345442485242, -20.36932031849321589, 62.27793240076999126 ) ) ;
#13867=CARTESIAN_POINT ( 'NONE',  ( -24.18470913683765389, -12.80901137141652768, 69.78715111652664405 ) ) ;
#13870=CARTESIAN_POINT ( 'NONE',  ( -7.413536378130524795, -16.17550971119529990, 54.49999999999995026 ) ) ;
#13871=EDGE_CURVE ( 'NONE', #8571, #33331, #41169, .T. ) ;
#13872=FACE_OUTER_BOUND ( 'NONE', #11238, .T. ) ;
#13874=CARTESIAN_POINT ( 'NONE',  ( -16.84865286310842336, -21.83598151670433296, 68.98088545748413480 ) ) ;
#13875=ORIENTED_EDGE ( 'NONE', *, *, #17645, .T. ) ;
#13877=EDGE_CURVE ( 'NONE', #47795, #11148, #17396, .T. ) ;
#13880=CARTESIAN_POINT ( 'NONE',  ( -10.00761947527410634, -15.51609109068450465, 57.75288224187332276 ) ) ;
#13881=ORIENTED_EDGE ( 'NONE', *, *, #11020, .T. ) ;
#13882=( BOUNDED_CURVE ( )  B_SPLINE_CURVE ( 3, ( #8414, #30355, #8187, #38189 ),
 .UNSPECIFIED., .F., .F. ) 
 B_SPLINE_CURVE_WITH_KNOTS ( ( 4, 4 ),
 ( 0.5000000000000000000, 0.9074455897393690629 ),
 .UNSPECIFIED. ) 
 CURVE ( )  GEOMETRIC_REPRESENTATION_ITEM ( )  RATIONAL_B_SPLINE_CURVE ( ( 1.000000000000022871, 0.4567392136813371861, 0.3561768502900161115, 0.6983129098260846268 ) ) 
 REPRESENTATION_ITEM ( '' )  );
#13883=LINE ( 'NONE', #14844, #42031 ) ;
#13885=VERTEX_POINT ( 'NONE', #785 ) ;
#13887=CARTESIAN_POINT ( 'NONE',  ( -13.96006710246513549, -20.89348392225634754, 71.99778020514392551 ) ) ;
#13888=CARTESIAN_POINT ( 'NONE',  ( -13.11945872550529835, -9.225962324091906197, 67.67942785705487552 ) ) ;
#13891=CARTESIAN_POINT ( 'NONE',  ( -12.91576191806997542, -9.388722997169708151, 71.13453240065665284 ) ) ;
#13892=( BOUNDED_SURFACE ( )  B_SPLINE_SURFACE ( 3, 1, ( 
 ( #12014, #27026 ),
 ( #42049, #8321 ),
 ( #23335, #4618 ),
 ( #15926, #20616 ),
 ( #25274, #35846 ),
 ( #24559, #25027 ),
 ( #32179, #28486 ) ),
 .UNSPECIFIED., .T., .F., .F. ) 
 B_SPLINE_SURFACE_WITH_KNOTS ( ( 4, 3, 4 ),
 ( 2, 2 ),
 ( 0.000000000000000000, 0.5000000000000000000, 1.000000000000000000 ),
 ( 0.000000000000000000, 1.000000000000000000 ),
 .UNSPECIFIED. ) 
 GEOMETRIC_REPRESENTATION_ITEM ( )  RATIONAL_B_SPLINE_SURFACE ( (
 ( 1.000000000000000000, 1.000000000000000000),
 ( 0.3333333333333335369, 0.3333333333333330373),
 ( 0.3333333333333335369, 0.3333333333333330373),
 ( 1.000000000000000000, 1.000000000000000000),
 ( 0.3333333333333333703, 0.3333333333333333703),
 ( 0.3333333333333333703, 0.3333333333333333703),
 ( 1.000000000000000000, 1.000000000000000000) ) ) 
 REPRESENTATION_ITEM ( '' )  SURFACE ( )  );
#13894=ORIENTED_EDGE ( 'NONE', *, *, #16079, .F. ) ;
#13895=ORIENTED_EDGE ( 'NONE', *, *, #29866, .F. ) ;
#13899=CARTESIAN_POINT ( 'NONE',  ( -11.32469277870022850, -18.34471304272907588, 58.10714594244493725 ) ) ;
#13902=AXIS2_PLACEMENT_3D ( 'NONE', #21003, #5980, #28638 ) ;
#13903=ORIENTED_EDGE ( 'NONE', *, *, #17197, .F. ) ;
#13904=DIRECTION ( 'NONE',  ( -4.664556984129884891E-06, 8.285185772962303489E-06, -0.9999999999547988239 ) ) ;
#13905=DIRECTION ( 'NONE',  ( 0.3667195576449455152, -0.9303315355510074491, -1.591455084066187253E-08 ) ) ;
#13907=ORIENTED_EDGE ( 'NONE', *, *, #22282, .T. ) ;
#13908=CARTESIAN_POINT ( 'NONE',  ( -16.97946104448713101, -21.84517140583366057, 72.46543221429990922 ) ) ;
#13910=FACE_OUTER_BOUND ( 'NONE', #9256, .T. ) ;
#13911=CARTESIAN_POINT ( 'NONE',  ( -21.41863048803932656, -8.999699081277377388, 73.61600897546567523 ) ) ;
#13912=CARTESIAN_POINT ( 'NONE',  ( -21.57785772703445559, -20.99377414531294406, 72.72435196568677895 ) ) ;
#13914=CARTESIAN_POINT ( 'NONE',  ( -19.30271930833434979, -8.014115225907463724, 60.11092997145157568 ) ) ;
#13915=DIRECTION ( 'NONE',  ( 0.9999889394985580493, 0.004703284017506803583, -7.734398264755851970E-09 ) ) ;
#13917=ORIENTED_EDGE ( 'NONE', *, *, #1030, .T. ) ;
#13918=CARTESIAN_POINT ( 'NONE',  ( -24.83005653327608897, -15.61813750885534979, 73.10280114214759806 ) ) ;
#13920=ORIENTED_EDGE ( 'NONE', *, *, #28577, .F. ) ;
#13921=CARTESIAN_POINT ( 'NONE',  ( -13.60236376389480384, -20.73382277062339085, 61.80174179654961364 ) ) ;
#13924=CARTESIAN_POINT ( 'NONE',  ( -13.19071075504626478, -8.678814667849811926, 60.54611945450858457 ) ) ;
#13925=CARTESIAN_POINT ( 'NONE',  ( -13.82689732469268229, -20.87277619789260186, 68.47097268802275494 ) ) ;
#13926=FACE_OUTER_BOUND ( 'NONE', #8663, .T. ) ;
#13928=DIRECTION ( 'NONE',  ( 3.141253923644155253E-07, -8.288700512985352896E-07, 0.9999999999996072031 ) ) ;
#13930=DIRECTION ( 'NONE',  ( 4.133538118270764137E-06, -2.214839422975871337E-07, 0.9999999999914324089 ) ) ;
#13931=CARTESIAN_POINT ( 'NONE',  ( -11.35974425695043699, -11.20802616635808313, 64.56370858977317084 ) ) ;
#13932=CARTESIAN_POINT ( 'NONE',  ( -24.26595263201846109, -13.32969024507516309, 59.66267925069213618 ) ) ;
#13934=CARTESIAN_POINT ( 'NONE',  ( -10.16587528726038414, -13.12915031972860902, 71.33015799040107652 ) ) ;
#13935=AXIS2_PLACEMENT_3D ( 'NONE', #30373, #3512, #18526 ) ;
#13936=CARTESIAN_POINT ( 'NONE',  ( -19.59334240102641544, -21.51721888655241699, 65.46486226986607448 ) ) ;
#13937=ORIENTED_EDGE ( 'NONE', *, *, #23854, .F. ) ;
#13940=CIRCLE ( 'NONE', #28146, 2.499999999999999556 ) ;
#13941=FACE_OUTER_BOUND ( 'NONE', #25923, .T. ) ;
#13943=CARTESIAN_POINT ( 'NONE',  ( -13.08910764958623574, -9.312959504979252401, 67.39445176332881715 ) ) ;
#13944=CARTESIAN_POINT ( 'NONE',  ( -22.56207008003183745, -19.63703213565221262, 72.92928497383269359 ) ) ;
#13946=ADVANCED_FACE ( 'NONE', ( #15532 ), #26897, .T. ) ;
#13948=ORIENTED_EDGE ( 'NONE', *, *, #23986, .F. ) ;
#13950=EDGE_CURVE ( 'NONE', #39081, #22354, #40341, .T. ) ;
#13953=CARTESIAN_POINT ( 'NONE',  ( -19.85131540638528591, -8.243492900160722670, 73.82982733467895287 ) ) ;
#13958=ORIENTED_EDGE ( 'NONE', *, *, #44753, .T. ) ;
#13963=CARTESIAN_POINT ( 'NONE',  ( -10.01366804335076210, -15.58332129913256381, 61.22444385224647334 ) ) ;
#13964=VERTEX_POINT ( 'NONE', #11616 ) ;
#13966=VECTOR ( 'NONE', #393, 1000.000000000000114 ) ;
#13967=CARTESIAN_POINT ( 'NONE',  ( -13.42824119710918573, -20.62712141855529779, 65.13062048310476371 ) ) ;
#13968=CARTESIAN_POINT ( 'NONE',  ( -20.19231657184298356, -8.325423463105360966, 70.25100341277898508 ) ) ;
#13969=EDGE_CURVE ( 'NONE', #9242, #17387, #18928, .T. ) ;
#13972=CARTESIAN_POINT ( 'NONE',  ( -10.82146677850202465, -17.29089146116874076, 68.18901905820221998 ) ) ;
#13973=ORIENTED_EDGE ( 'NONE', *, *, #24140, .F. ) ;
#13974=CARTESIAN_POINT ( 'NONE',  ( -23.05503254776601096, -18.96763528207466720, 58.99296609845764294 ) ) ;
#13979=ORIENTED_EDGE ( 'NONE', *, *, #47323, .F. ) ;
#13980=CARTESIAN_POINT ( 'NONE',  ( -20.41456109077558168, -8.424717559663436717, 66.78663853121041427 ) ) ;
#13982=EDGE_CURVE ( 'NONE', #45729, #17630, #34014, .T. ) ;
#13985=CARTESIAN_POINT ( 'NONE',  ( -20.19053640067075506, -7.838066347919499854, 53.49999999999994316 ) ) ;
#13986=CARTESIAN_POINT ( 'NONE',  ( -23.89279295945009096, -11.11331726805715725, 69.93564813258274171 ) ) ;
#13987=VERTEX_POINT ( 'NONE', #308 ) ;
#13990=CARTESIAN_POINT ( 'NONE',  ( -12.02825722964846022, -10.34976005852228020, 67.49896853033064303 ) ) ;
#13992=ORIENTED_EDGE ( 'NONE', *, *, #47634, .T. ) ;
#13993=CYLINDRICAL_SURFACE ( 'NONE', #22023, 0.1500000000000060729 ) ;
#13998=CARTESIAN_POINT ( 'NONE',  ( -12.79154865046270473, -8.973695691655201756, 67.49287406301634462 ) ) ;
#13999=CARTESIAN_POINT ( 'NONE',  ( -20.56498907581264390, -8.053615130811071054, 66.97442378999858192 ) ) ;
#14001=AXIS2_PLACEMENT_3D ( 'NONE', #38344, #12026, #12971 ) ;
#14003=ORIENTED_EDGE ( 'NONE', *, *, #38654, .T. ) ;
#14004=FACE_OUTER_BOUND ( 'NONE', #17865, .T. ) ;
#14006=EDGE_CURVE ( 'NONE', #41870, #45990, #2236, .T. ) ;
#14007=CARTESIAN_POINT ( 'NONE',  ( -13.51031400108801428, -20.61338249540413869, 61.53263022144881234 ) ) ;
#14008=( BOUNDED_CURVE ( )  B_SPLINE_CURVE ( 3, ( #1904, #40534, #10516, #25521 ),
 .UNSPECIFIED., .F., .F. ) 
 B_SPLINE_CURVE_WITH_KNOTS ( ( 4, 4 ),
 ( 0.4074455897393691739, 0.5000000000000000000 ),
 .UNSPECIFIED. ) 
 CURVE ( )  GEOMETRIC_REPRESENTATION_ITEM ( )  RATIONAL_B_SPLINE_CURVE ( ( 0.6983129098261000589, 0.7760317562606808828, 0.8765941196519739798, 0.9999999999999630296 ) ) 
 REPRESENTATION_ITEM ( '' )  );
#14010=ADVANCED_FACE ( 'NONE', ( #37953 ), #6988, .T. ) ;
#14011=EDGE_CURVE ( 'NONE', #3943, #445, #15447, .T. ) ;
#14012=VERTEX_POINT ( 'NONE', #9145 ) ;
#14013=CARTESIAN_POINT ( 'NONE',  ( -20.56934712877496807, -8.555617018170707411, 59.95011231546465069 ) ) ;
#14014=CARTESIAN_POINT ( 'NONE',  ( -12.46122051107220230, -19.81685944811288635, 64.88146935704573082 ) ) ;
#14016=CARTESIAN_POINT ( 'NONE',  ( -23.88856641767997857, -11.10584043512839791, 70.01397978569940506 ) ) ;
#14019=( BOUNDED_SURFACE ( )  B_SPLINE_SURFACE ( 3, 1, ( 
 ( #45940, #27220 ),
 ( #42246, #27458 ),
 ( #8506, #23538 ),
 ( #8766, #38536 ),
 ( #32132, #21044 ),
 ( #28193, #35804 ),
 ( #14282, #39754 ) ),
 .UNSPECIFIED., .T., .F., .F. ) 
 B_SPLINE_SURFACE_WITH_KNOTS ( ( 4, 3, 4 ),
 ( 2, 2 ),
 ( 0.000000000000000000, 0.5000000000000000000, 1.000000000000000000 ),
 ( 0.000000000000000000, 1.000000000000000000 ),
 .UNSPECIFIED. ) 
 GEOMETRIC_REPRESENTATION_ITEM ( )  RATIONAL_B_SPLINE_SURFACE ( (
 ( 1.000000000000000000, 1.000000000000000000),
 ( 0.3333333333333335369, 0.3333333333333330373),
 ( 0.3333333333333335369, 0.3333333333333330373),
 ( 1.000000000000000000, 1.000000000000000000),
 ( 0.3333333333333333703, 0.3333333333333333703),
 ( 0.3333333333333333703, 0.3333333333333333703),
 ( 1.000000000000000000, 1.000000000000000000) ) ) 
 REPRESENTATION_ITEM ( '' )  SURFACE ( )  );
#14020=CARTESIAN_POINT ( 'NONE',  ( -24.25719323842812258, -13.28918340244882224, 59.66267871176336968 ) ) ;
#14023=ORIENTED_EDGE ( 'NONE', *, *, #27323, .F. ) ;
#14025=VECTOR ( 'NONE', #24452, 1000.000000000000114 ) ;
#14026=CARTESIAN_POINT ( 'NONE',  ( -17.84029708445064344, -21.79726103445669239, 61.89152536399645044 ) ) ;
#14028=CARTESIAN_POINT ( 'NONE',  ( -23.33225598143976498, -10.27063514773017516, 59.76236756523886129 ) ) ;
#14029=EDGE_LOOP ( 'NONE', ( #25070, #14570 ) ) ;
#14030=FACE_OUTER_BOUND ( 'NONE', #37935, .T. ) ;
#14031=AXIS2_PLACEMENT_3D ( 'NONE', #27423, #4782, #23988 ) ;
#14033=ORIENTED_EDGE ( 'NONE', *, *, #45555, .F. ) ;
#14034=CARTESIAN_POINT ( 'NONE',  ( -24.31883679440356261, -17.63164986302842152, 66.20003142906764992 ) ) ;
#14035=CYLINDRICAL_SURFACE ( 'NONE', #35394, 0.1500000000000034084 ) ;
#14036=CARTESIAN_POINT ( 'NONE',  ( -11.29134393598116937, -11.33126488396075260, 64.16354160640879911 ) ) ;
#14037=ORIENTED_EDGE ( 'NONE', *, *, #25735, .F. ) ;
#14038=CARTESIAN_POINT ( 'NONE',  ( -16.21670493413017766, -7.863214532617857522, 60.49468660818079968 ) ) ;
#14039=DIRECTION ( 'NONE',  ( 2.161108583753623267E-06, 4.147204431722191678E-06, 0.9999999999890650804 ) ) ;
#14040=CARTESIAN_POINT ( 'NONE',  ( -10.52215041504658188, -13.37196039468858011, 74.97817647370040106 ) ) ;
#14041=DIRECTION ( 'NONE',  ( 2.872222170658504970E-06, -2.507089450317157248E-06, -0.9999999999927324801 ) ) ;
#14043=ORIENTED_EDGE ( 'NONE', *, *, #18187, .T. ) ;
#14044=CARTESIAN_POINT ( 'NONE',  ( -12.26099810431060533, -10.00863248521528703, 60.85918089305128831 ) ) ;
#14045=CARTESIAN_POINT ( 'NONE',  ( -9.995623895585607599, -14.24219643007072023, 64.64449787557668969 ) ) ;
#14046=LINE ( 'NONE', #25168, #25872 ) ;
#14047=CARTESIAN_POINT ( 'NONE',  ( -23.74619244455239198, -11.68933966055485207, 63.25218278636740621 ) ) ;
#14048=CARTESIAN_POINT ( 'NONE',  ( -10.81980145280015115, -12.48416413777423806, 60.90926616978132557 ) ) ;
#14049=CARTESIAN_POINT ( 'NONE',  ( -24.22177711603362482, -13.13842781680106420, 62.83264177645653348 ) ) ;
#14050=EDGE_LOOP ( 'NONE', ( #19777, #30275, #23714, #11039, #12923 ) ) ;
#14052=CARTESIAN_POINT ( 'NONE',  ( -21.12380683100872858, -21.27649256055507365, 65.77109308171978341 ) ) ;
#14053=CARTESIAN_POINT ( 'NONE',  ( -10.83536388074712598, -17.31742051234312640, 64.92739380450886699 ) ) ;
#14054=ORIENTED_EDGE ( 'NONE', *, *, #35991, .F. ) ;
#14055=CARTESIAN_POINT ( 'NONE',  ( -19.23866564181064831, -21.62168251543363695, 58.82507384655652771 ) ) ;
#14056=CARTESIAN_POINT ( 'NONE',  ( -23.56138404952065812, -11.33988834032953008, 70.19210750372964469 ) ) ;
#14058=CARTESIAN_POINT ( 'NONE',  ( -13.67448191250337430, -20.77955027102393615, 64.99188703928707866 ) ) ;
#14060=EDGE_CURVE ( 'NONE', #30297, #15772, #32282, .T. ) ;
#14061=CARTESIAN_POINT ( 'NONE',  ( -24.78768057424481341, -16.32668859419483454, 53.76227901944321275 ) ) ;
#14062=CARTESIAN_POINT ( 'NONE',  ( -24.38111619087839799, -15.96880572012975286, 62.47839786477943136 ) ) ;
#14064=CARTESIAN_POINT ( 'NONE',  ( -10.42297871322231551, -14.76125519756164017, 74.86949220091082680 ) ) ;
#14065=CARTESIAN_POINT ( 'NONE',  ( -14.79922817013080483, -7.836842635312091687, 57.03495431467663224 ) ) ;
#14066=ADVANCED_FACE ( 'NONE', ( #47303 ), #17037, .T. ) ;
#14067=EDGE_LOOP ( 'NONE', ( #45732, #45564, #26504, #30846, #28818 ) ) ;
#14068=CARTESIAN_POINT ( 'NONE',  ( -10.74628672884880132, -17.07053172313825939, 61.17215199736627795 ) ) ;
#14069=CARTESIAN_POINT ( 'NONE',  ( -23.91439714532632621, -17.43141235356291574, 65.94357239632037704 ) ) ;
#14070=AXIS2_PLACEMENT_3D ( 'NONE', #23648, #16216, #35429 ) ;
#14073=CARTESIAN_POINT ( 'NONE',  ( -12.68381401182790569, -19.95991009262169413, 68.33657438305763776 ) ) ;
#14074=VECTOR ( 'NONE', #54, 1000.000000000000114 ) ;
#14081=CARTESIAN_POINT ( 'NONE',  ( -17.35252955274262732, -7.359423945522111765, 67.19756513320511715 ) ) ;
#14083=CARTESIAN_POINT ( 'NONE',  ( -11.80131277442636240, -10.54314289786156777, 67.65463988879716339 ) ) ;
#14084=AXIS2_PLACEMENT_3D ( 'NONE', #31286, #12575, #45839 ) ;
#14085=ADVANCED_FACE ( 'NONE', ( #13053 ), #382, .T. ) ;
#14089=CARTESIAN_POINT ( 'NONE',  ( -10.98855013657561841, -11.05570324207465660, 60.83919106357873829 ) ) ;
#14090=CARTESIAN_POINT ( 'NONE',  ( -20.89788161767221197, -20.94431024770144489, 62.39999296070408974 ) ) ;
#14091=ADVANCED_FACE ( 'NONE', ( #40607 ), #32967, .T. ) ;
#14094=CARTESIAN_POINT ( 'NONE',  ( -18.37786432726835883, -21.79469297182707521, 69.10042588711679912 ) ) ;
#14095=EDGE_LOOP ( 'NONE', ( #41961, #19214, #43951, #44655, #39946 ) ) ;
#14096=LINE ( 'NONE', #14816, #41755 ) ;
#14100=CARTESIAN_POINT ( 'NONE',  ( -20.20277394004996196, -7.896613096357342876, 73.86063200510004378 ) ) ;
#14101=CARTESIAN_POINT ( 'NONE',  ( -12.84719963800786502, -9.512789006345032661, 74.31923006385322594 ) ) ;
#14103=CARTESIAN_POINT ( 'NONE',  ( -13.38462506958126319, -20.58719851387657940, 58.04650077714654088 ) ) ;
#14104=FACE_OUTER_BOUND ( 'NONE', #33484, .T. ) ;
#14105=VERTEX_POINT ( 'NONE', #21194 ) ;
#14110=DIRECTION ( 'NONE',  ( 3.597453744745084160E-07, 4.264980248628041219E-06, -0.9999999999908402160 ) ) ;
#14112=VERTEX_POINT ( 'NONE', #47537 ) ;
#14115=CARTESIAN_POINT ( 'NONE',  ( -24.31482301288783532, -13.31912224170856796, 59.66267924674056644 ) ) ;
#14116=EDGE_CURVE ( 'NONE', #9892, #7972, #40621, .T. ) ;
#14118=CARTESIAN_POINT ( 'NONE',  ( -19.82413079548422274, -21.27835043604049403, 47.99999999999994316 ) ) ;
#14119=VERTEX_POINT ( 'NONE', #21907 ) ;
#14120=ORIENTED_EDGE ( 'NONE', *, *, #45025, .T. ) ;
#14121=ORIENTED_EDGE ( 'NONE', *, *, #26891, .T. ) ;
#14122=CARTESIAN_POINT ( 'NONE',  ( -21.32599660273145759, -20.68102258270527471, 72.52446460307699283 ) ) ;
#14123=CARTESIAN_POINT ( 'NONE',  ( -10.99586753834015695, -11.04334891231907534, 60.86381058728009208 ) ) ;
#14125=CARTESIAN_POINT ( 'NONE',  ( -12.68656345882633296, -9.059469911947932275, 70.89279414395181789 ) ) ;
#14127=ORIENTED_EDGE ( 'NONE', *, *, #31002, .T. ) ;
#14130=VECTOR ( 'NONE', #18917, 1000.000000000000000 ) ;
#14132=DIRECTION ( 'NONE',  ( -0.6538427738826437796, -0.7566304428460742804, 5.916677973164435741E-08 ) ) ;
#14133=AXIS2_PLACEMENT_3D ( 'NONE', #30560, #8152, #995 ) ;
#14134=EDGE_CURVE ( 'NONE', #1251, #47122, #34498, .T. ) ;
#14137=EDGE_LOOP ( 'NONE', ( #16472, #38137, #9172, #9120, #11739 ) ) ;
#14138=ADVANCED_FACE ( 'NONE', ( #14004 ), #7145, .T. ) ;
#14139=CARTESIAN_POINT ( 'NONE',  ( -10.79785091779906381, -12.40172372778942034, 57.32857331700826364 ) ) ;
#14140=CARTESIAN_POINT ( 'NONE',  ( -24.80769047312930553, -15.80232199467591947, 69.71802767292497549 ) ) ;
#14141=VECTOR ( 'NONE', #23339, 1000.000000000000227 ) ;
#14142=ADVANCED_FACE ( 'NONE', ( #13772 ), #2474, .T. ) ;
#14143=( BOUNDED_CURVE ( )  B_SPLINE_CURVE ( 3, ( #36603, #14191, #17169, #40092 ),
 .UNSPECIFIED., .F., .F. ) 
 B_SPLINE_CURVE_WITH_KNOTS ( ( 4, 4 ),
 ( 0.9074455897393687298, 1.000000000000000000 ),
 .UNSPECIFIED. ) 
 CURVE ( )  GEOMETRIC_REPRESENTATION_ITEM ( )  RATIONAL_B_SPLINE_CURVE ( ( 0.6983129098261082746, 0.7760317562607114139, 0.8765941196520086187, 1.000000000000000000 ) ) 
 REPRESENTATION_ITEM ( '' )  );
#14145=CARTESIAN_POINT ( 'NONE',  ( -17.00326681110915672, -21.84667578895833628, 72.46543211950746866 ) ) ;
#14147=ORIENTED_EDGE ( 'NONE', *, *, #12314, .F. ) ;
#14148=DIRECTION ( 'NONE',  ( 0.2696806815386222911, -0.9629498065864410261, 2.003044183322984602E-16 ) ) ;
#14149=DIRECTION ( 'NONE',  ( 0.8467008005855422015, -0.3141239757129651311, -0.4294460177601863160 ) ) ;
#14150=LINE ( 'NONE', #40516, #19717 ) ;
#14151=CARTESIAN_POINT ( 'NONE',  ( -17.04413539470109740, -21.84925844046378174, 72.45071136019464575 ) ) ;
#14153=CARTESIAN_POINT ( 'NONE',  ( -12.36756753426621813, -9.896138138887707214, 57.37463480816234096 ) ) ;
#14154=CARTESIAN_POINT ( 'NONE',  ( -22.83563034752066656, -10.36892392777437522, 63.08688399054229734 ) ) ;
#14155=CARTESIAN_POINT ( 'NONE',  ( -10.45859239952313224, -15.89938452881993847, 64.79299464097340433 ) ) ;
#14156=ORIENTED_EDGE ( 'NONE', *, *, #10767, .T. ) ;
#14158=CARTESIAN_POINT ( 'NONE',  ( -21.53550107051403018, -9.078485192726875042, 74.01617645989524874 ) ) ;
#14159=( BOUNDED_CURVE ( )  B_SPLINE_CURVE ( 3, ( #4243, #19254, #540, #23203 ),
 .UNSPECIFIED., .F., .F. ) 
 B_SPLINE_CURVE_WITH_KNOTS ( ( 4, 4 ),
 ( 0.5000000000000000000, 0.9074455897393671755 ),
 .UNSPECIFIED. ) 
 CURVE ( )  GEOMETRIC_REPRESENTATION_ITEM ( )  RATIONAL_B_SPLINE_CURVE ( ( 1.000000000000001776, 0.4567392136813420156, 0.3561768502900327649, 0.6983129098260758560 ) ) 
 REPRESENTATION_ITEM ( '' )  );
#14160=CARTESIAN_POINT ( 'NONE',  ( -12.54253442593986456, -19.82621537833410841, 64.86674886820043184 ) ) ;
#14161=EDGE_LOOP ( 'NONE', ( #27587, #6586, #31323, #4220, #2718 ) ) ;
#14162=CARTESIAN_POINT ( 'NONE',  ( -13.73970650151387751, -20.76112128469266693, 64.98628881673506896 ) ) ;
#14163=VERTEX_POINT ( 'NONE', #18201 ) ;
#14164=CARTESIAN_POINT ( 'NONE',  ( -13.23632661096056928, -8.647559330782417675, 60.54676144413815564 ) ) ;
#14165=CARTESIAN_POINT ( 'NONE',  ( -14.01118748589248320, -10.49619482288619920, 53.49999999999995026 ) ) ;
#14167=CARTESIAN_POINT ( 'NONE',  ( -10.40174263535760524, -17.29725023780839166, 61.34238537770443855 ) ) ;
#14168=ORIENTED_EDGE ( 'NONE', *, *, #8575, .F. ) ;
#14169=CYLINDRICAL_SURFACE ( 'NONE', #13440, 0.1499999999999979128 ) ;
#14170=CARTESIAN_POINT ( 'NONE',  ( -24.23802539630901265, -11.79523892523793371, 59.66890987421792403 ) ) ;
#14171=EDGE_CURVE ( 'NONE', #20165, #30692, #7291, .T. ) ;
#14172=CARTESIAN_POINT ( 'NONE',  ( -23.38272234930034088, -18.48272619114020188, 69.40257884200109118 ) ) ;
#14173=ORIENTED_EDGE ( 'NONE', *, *, #4548, .F. ) ;
#14174=CARTESIAN_POINT ( 'NONE',  ( -11.22559363225283491, -18.94243559922078646, 64.88560521426357752 ) ) ;
#14175=VECTOR ( 'NONE', #17611, 1000.000000000000114 ) ;
#14176=( BOUNDED_SURFACE ( )  B_SPLINE_SURFACE ( 3, 1, ( 
 ( #47252, #25327 ),
 ( #28774, #17442 ),
 ( #47496, #17906 ),
 ( #21398, #17673 ),
 ( #43807, #13496 ),
 ( #36619, #32236 ),
 ( #33171, #5887 ) ),
 .UNSPECIFIED., .T., .F., .F. ) 
 B_SPLINE_SURFACE_WITH_KNOTS ( ( 4, 3, 4 ),
 ( 2, 2 ),
 ( 0.000000000000000000, 0.5000000000000000000, 1.000000000000000000 ),
 ( 0.000000000000000000, 1.000000000000000000 ),
 .UNSPECIFIED. ) 
 GEOMETRIC_REPRESENTATION_ITEM ( )  RATIONAL_B_SPLINE_SURFACE ( (
 ( 1.000000000000000000, 1.000000000000000000),
 ( 0.3333333333333335369, 0.3333333333333330373),
 ( 0.3333333333333335369, 0.3333333333333330373),
 ( 1.000000000000000000, 1.000000000000000000),
 ( 0.3333333333333333703, 0.3333333333333333703),
 ( 0.3333333333333333703, 0.3333333333333333703),
 ( 1.000000000000000000, 1.000000000000000000) ) ) 
 REPRESENTATION_ITEM ( '' )  SURFACE ( )  );
#14177=CARTESIAN_POINT ( 'NONE',  ( -24.76540221579651302, -16.07765826482591365, 66.17829537637275905 ) ) ;
#14178=ORIENTED_EDGE ( 'NONE', *, *, #13758, .F. ) ;
#14179=ORIENTED_EDGE ( 'NONE', *, *, #26539, .T. ) ;
#14180=CARTESIAN_POINT ( 'NONE',  ( -15.06305009558132646, -21.87596932251961590, 65.21941411614068329 ) ) ;
#14181=CARTESIAN_POINT ( 'NONE',  ( -10.02748777283063220, -15.69962750030634524, 61.23777819939896006 ) ) ;
#14184=CARTESIAN_POINT ( 'NONE',  ( -19.45445856626800918, -21.50841060167162055, 61.99503609350492184 ) ) ;
#14185=DIRECTION ( 'NONE',  ( -0.9410372374137780938, -0.3383029970317210644, -1.029646047569396398E-09 ) ) ;
#14186=CARTESIAN_POINT ( 'NONE',  ( -11.15036096168905821, -11.58527761980847970, 64.35701831376418625 ) ) ;
#14187=EDGE_CURVE ( 'NONE', #7578, #3868, #20528, .T. ) ;
#14188=CARTESIAN_POINT ( 'NONE',  ( -14.75426735376592013, -21.76440006487333179, 61.73626185728981142 ) ) ;
#14189=ORIENTED_EDGE ( 'NONE', *, *, #15458, .F. ) ;
#14191=CARTESIAN_POINT ( 'NONE',  ( -22.90827110196059735, -10.37898438100278575, 63.37185973727753208 ) ) ;
#14195=PLANE ( 'NONE',  #42940 ) ;
#14196=CARTESIAN_POINT ( 'NONE',  ( -18.60850724411298529, -7.453946191617336403, 73.94090162317939985 ) ) ;
#14197=EDGE_LOOP ( 'NONE', ( #29501, #5478, #31803, #6914, #27665 ) ) ;
#14198=B_SPLINE_CURVE_WITH_KNOTS ( 'NONE', 3,
 ( #3247, #51, #44161, #30098, #29847, #10410, #33757, #21491, #47820, #6704 ),
 .UNSPECIFIED., .F., .F.,
 ( 4, 2, 2, 2, 4 ),
 ( 0.000000000000000000, 0.2500000000000000000, 0.5000000000000000000, 0.7500000000000000000, 1.000000000000000000 ),
 .UNSPECIFIED. ) ;
#14200=EDGE_LOOP ( 'NONE', ( #4264, #20517, #4712, #8003, #29044 ) ) ;
#14202=AXIS2_PLACEMENT_3D ( 'NONE', #25321, #26046, #11273 ) ;
#14203=CARTESIAN_POINT ( 'NONE',  ( -24.33635500431102017, -15.92417168687779494, 69.64380670067536983 ) ) ;
#14205=EDGE_CURVE ( 'NONE', #30144, #5852, #7396, .T. ) ;
#14206=AXIS2_PLACEMENT_3D ( 'NONE', #45534, #11791, #14960 ) ;
#14207=CARTESIAN_POINT ( 'NONE',  ( -23.19948571119275726, -18.85291137746750323, 65.83861571032234394 ) ) ;
#14208=CARTESIAN_POINT ( 'NONE',  ( -10.02191638112385697, -15.65273889608829982, 61.15293747381159761 ) ) ;
#14210=B_SPLINE_CURVE_WITH_KNOTS ( 'NONE', 1,
 ( #18052, #29397 ),
 .UNSPECIFIED., .F., .F.,
 ( 2, 2 ),
 ( 0.000000000000000000, 1.000000000000000000 ),
 .UNSPECIFIED. ) ;
#14211=CARTESIAN_POINT ( 'NONE',  ( -13.53189383941936264, -21.16172133628754892, 65.02982926591782586 ) ) ;
#14212=CARTESIAN_POINT ( 'NONE',  ( -15.77653169993974558, -7.543659789509001179, 67.33996046129556134 ) ) ;
#14213=AXIS2_PLACEMENT_3D ( 'NONE', #37399, #263, #7896 ) ;
#14214=DIRECTION ( 'NONE',  ( -0.5562740912439653185, -0.8309988781043535777, -7.851267778718615459E-08 ) ) ;
#14216=CARTESIAN_POINT ( 'NONE',  ( -24.11345430931175926, -12.58310556425532312, 73.24225580887585352 ) ) ;
#14217=VERTEX_POINT ( 'NONE', #41111 ) ;
#14218=CYLINDRICAL_SURFACE ( 'NONE', #24410, 0.1500000000000071554 ) ;
#14219=EDGE_CURVE ( 'NONE', #35817, #33222, #20800, .T. ) ;
#14220=VERTEX_POINT ( 'NONE', #11321 ) ;
#14221=CARTESIAN_POINT ( 'NONE',  ( -23.84953956799437691, -11.90778598363859686, 59.48795493759783426 ) ) ;
#14222=CARTESIAN_POINT ( 'NONE',  ( -24.87179831301899924, -14.62392340704838745, 62.91285274408475914 ) ) ;
#14223=VERTEX_POINT ( 'NONE', #29793 ) ;
#14225=EDGE_CURVE ( 'NONE', #19018, #41432, #13862, .T. ) ;
#14226=CARTESIAN_POINT ( 'NONE',  ( -22.39682231837810988, -19.80670998913449665, 69.47417992432380629 ) ) ;
#14227=VECTOR ( 'NONE', #2728, 1000.000000000000114 ) ;
#14228=CARTESIAN_POINT ( 'NONE',  ( -20.24469333105209046, -8.402151907256357077, 70.26716930211884460 ) ) ;
#14229=ORIENTED_EDGE ( 'NONE', *, *, #10924, .F. ) ;
#14231=CARTESIAN_POINT ( 'NONE',  ( -11.10871725088146356, -18.76147163815154784, 61.45427695282393898 ) ) ;
#14234=B_SPLINE_CURVE_WITH_KNOTS ( 'NONE', 3,
 ( #44124, #29321, #32530, #6670, #44355, #21689, #47555, #36444, #35966, #3213 ),
 .UNSPECIFIED., .F., .F.,
 ( 4, 2, 2, 2, 4 ),
 ( 0.1272669073658234118, 0.2522669073463141287, 0.3772669073268049011, 0.5022669073072956181, 0.6272669072877863350 ),
 .UNSPECIFIED. ) ;
#14235=CARTESIAN_POINT ( 'NONE',  ( -13.47975436313424957, -21.12944577273253088, 65.17967206052510676 ) ) ;
#14236=CARTESIAN_POINT ( 'NONE',  ( -10.22687501107677477, -12.88500788934134889, 67.88832345126935763 ) ) ;
#14237=DIRECTION ( 'NONE',  ( 0.8201047403141396019, -0.5722134347551369737, -7.883065731092009224E-08 ) ) ;
#14239=VERTEX_POINT ( 'NONE', #3940 ) ;
#14240=VECTOR ( 'NONE', #9196, 1000.000000000000227 ) ;
#14241=CARTESIAN_POINT ( 'NONE',  ( -12.79111265990729507, -9.490472886863006607, 71.05745174362085947 ) ) ;
#14243=PLANE ( 'NONE',  #35915 ) ;
#14245=CARTESIAN_POINT ( 'NONE',  ( -23.77487038158592014, -11.74745262826995607, 62.96690348473899235 ) ) ;
#14246=CARTESIAN_POINT ( 'NONE',  ( -13.38504989191835826, -9.021193483636507082, 67.52375889928833885 ) ) ;
#14247=CARTESIAN_POINT ( 'NONE',  ( -15.03263910315855512, -8.176888424288378587, 56.86472059657746314 ) ) ;
#14248=CARTESIAN_POINT ( 'NONE',  ( -16.51307038081223766, -22.20334437192797949, 65.41902708460563076 ) ) ;
#14249=EDGE_LOOP ( 'NONE', ( #29559, #24533, #35513, #805, #13973 ) ) ;
#14250=CARTESIAN_POINT ( 'NONE',  ( -21.00642299473589247, -8.276168789376990631, 60.02780591114678543 ) ) ;
#14251=EDGE_CURVE ( 'NONE', #30525, #21614, #20987, .T. ) ;
#14253=CYLINDRICAL_SURFACE ( 'NONE', #13792, 0.1499999999999992173 ) ;
#14254=CARTESIAN_POINT ( 'NONE',  ( -19.74200936563729769, -21.46758226568296024, 68.94954551542706156 ) ) ;
#14255=ORIENTED_EDGE ( 'NONE', *, *, #44739, .F. ) ;
#14257=CARTESIAN_POINT ( 'NONE',  ( -16.95219942996303786, -7.374113640801781777, 74.15292427101722694 ) ) ;
#14259=CARTESIAN_POINT ( 'NONE',  ( -22.52885229756875773, -10.01948407182677592, 70.12064572036962318 ) ) ;
#14260=CARTESIAN_POINT ( 'NONE',  ( -11.41497442304007670, -19.21309820834011362, 71.80190602235010999 ) ) ;
#14261=B_SPLINE_CURVE_WITH_KNOTS ( 'NONE', 3,
 ( #15140, #45221, #11463, #41504, #19839, #8763, #20315, #16606, #38273, #30925 ),
 .UNSPECIFIED., .F., .F.,
 ( 4, 2, 2, 2, 4 ),
 ( 0.000000000000000000, 0.2500000000000000000, 0.5000000000000000000, 0.7500000000000000000, 1.000000000000000000 ),
 .UNSPECIFIED. ) ;
#14263=CARTESIAN_POINT ( 'NONE',  ( -23.94361510234960733, -17.49256946932371548, 65.94916996934229303 ) ) ;
#14264=CARTESIAN_POINT ( 'NONE',  ( -23.82024019063151243, -17.65337816030916684, 59.11264479274999672 ) ) ;
#14265=VERTEX_POINT ( 'NONE', #18948 ) ;
#14268=CARTESIAN_POINT ( 'NONE',  ( -10.43073328261085386, -14.50439875238632403, 67.85800126138448718 ) ) ;
#14269=B_SPLINE_CURVE_WITH_KNOTS ( 'NONE', 3,
 ( #41172, #22715, #40674, #26395, #6955, #14539, #30354, #7212, #37452, #26161 ),
 .UNSPECIFIED., .F., .F.,
 ( 4, 2, 2, 2, 4 ),
 ( 0.1272669073658406202, 0.2522669073463340572, 0.3772669073268274387, 0.5022669073073209312, 0.6272669072878143126 ),
 .UNSPECIFIED. ) ;
#14270=CARTESIAN_POINT ( 'NONE',  ( -23.30016224357493826, -19.38910683590379236, 59.14056577394535452 ) ) ;
#14271=ORIENTED_EDGE ( 'NONE', *, *, #39426, .F. ) ;
#14272=CARTESIAN_POINT ( 'NONE',  ( -14.60783717270099835, -21.70648693424663378, 58.35113322083577003 ) ) ;
#14273=ORIENTED_EDGE ( 'NONE', *, *, #1459, .F. ) ;
#14274=CARTESIAN_POINT ( 'NONE',  ( -10.47425561207849753, -17.49314520081206936, 64.81234810402725088 ) ) ;
#14275=CARTESIAN_POINT ( 'NONE',  ( -19.45183578605709940, -21.56134185002573744, 62.29503624138732221 ) ) ;
#14276=VERTEX_POINT ( 'NONE', #26335 ) ;
#14277=CARTESIAN_POINT ( 'NONE',  ( -24.17003186015574201, -17.97068590651718267, 59.20367199723977336 ) ) ;
#14278=EDGE_CURVE ( 'NONE', #19672, #20573, #33960, .T. ) ;
#14279=ADVANCED_FACE ( 'NONE', ( #3682 ), #7642, .T. ) ;
#14280=CARTESIAN_POINT ( 'NONE',  ( -19.40609653032597492, -21.57490932759623092, 61.99503665003788910 ) ) ;
#14281=DIRECTION ( 'NONE',  ( 3.395770063048969188E-06, 1.105252680118079259E-06, -0.9999999999936236561 ) ) ;
#14282=CARTESIAN_POINT ( 'NONE',  ( -21.79028809537168243, -9.273590339475653366, 63.47681654923867711 ) ) ;
#14283=DIRECTION ( 'NONE',  ( 0.000000000000000000, 0.000000000000000000, 1.000000000000000000 ) ) ;
#14285=EDGE_LOOP ( 'NONE', ( #4327, #11728 ) ) ;
#14286=CARTESIAN_POINT ( 'NONE',  ( -24.87105361238793932, -14.59201401153533340, 62.89013408101026670 ) ) ;
#14287=CARTESIAN_POINT ( 'NONE',  ( -10.78978129946085929, -12.42417050351721919, 57.47857332104950956 ) ) ;
#14290=EDGE_CURVE ( 'NONE', #1066, #48422, #22908, .T. ) ;
#14291=DIRECTION ( 'NONE',  ( -0.2843796944294934015, -0.9587117342539338560, -5.205739956168919862E-08 ) ) ;
#14292=CARTESIAN_POINT ( 'NONE',  ( -16.16379340615718618, -22.15191857530921382, 58.47080845268740035 ) ) ;
#14293=CARTESIAN_POINT ( 'NONE',  ( -24.26335575918792742, -16.30820562957639197, 62.70401880319807475 ) ) ;
#14294=EDGE_LOOP ( 'NONE', ( #30749, #40581, #27372, #16307 ) ) ;
#14296=CARTESIAN_POINT ( 'NONE',  ( -24.02580441457500982, -11.35651424597849690, 66.67860437913579119 ) ) ;
#14297=CARTESIAN_POINT ( 'NONE',  ( -9.975806665192521905, -14.64185444168544947, 71.48929178254144290 ) ) ;
#14299=CARTESIAN_POINT ( 'NONE',  ( -23.81302322525746362, -11.80978145726242978, 66.56647414731462220 ) ) ;
#14303=CARTESIAN_POINT ( 'NONE',  ( -14.60783614669699304, -21.70648650955843806, 58.35113213314874514 ) ) ;
#14304=( BOUNDED_CURVE ( )  B_SPLINE_CURVE ( 3, ( #19168, #15444, #24082, #34173 ),
 .UNSPECIFIED., .F., .F. ) 
 B_SPLINE_CURVE_WITH_KNOTS ( ( 4, 4 ),
 ( 1.570796326794896780, 1.780235837034223945 ),
 .UNSPECIFIED. ) 
 CURVE ( )  GEOMETRIC_REPRESENTATION_ITEM ( )  RATIONAL_B_SPLINE_CURVE ( ( 1.000000000000000000, 0.9963479302455153785, 0.9963479302455153785, 1.000000000000000000 ) ) 
 REPRESENTATION_ITEM ( '' )  );
#14305=CARTESIAN_POINT ( 'NONE',  ( -20.94465790601859467, -8.243431112063134947, 59.95629843672877257 ) ) ;
#14306=CARTESIAN_POINT ( 'NONE',  ( -12.14862823326899743, -9.548716677428323862, 57.19661362441988928 ) ) ;
#14307=CARTESIAN_POINT ( 'NONE',  ( -23.32103368030945489, -19.36207380375006082, 59.03410639999821541 ) ) ;
#14308=CARTESIAN_POINT ( 'NONE',  ( -21.01123981933952223, -20.87838139577334573, 65.73453944496496604 ) ) ;
#14309=ADVANCED_FACE ( 'NONE', ( #45074 ), #37900, .T. ) ;
#14310=ORIENTED_EDGE ( 'NONE', *, *, #44962, .T. ) ;
#14311=CARTESIAN_POINT ( 'NONE',  ( -14.19282086353638661, -8.542981675383003903, 71.01485553001869278 ) ) ;
#14312=LINE ( 'NONE', #26162, #25840 ) ;
#14313=CARTESIAN_POINT ( 'NONE',  ( -16.92014803599858652, -22.24222107688192196, 72.42189142509964483 ) ) ;
#14314=LINE ( 'NONE', #33772, #25596 ) ;
#14316=CARTESIAN_POINT ( 'NONE',  ( -15.03764954898300488, -21.45148416623199594, 58.32185190926050211 ) ) ;
#14317=CARTESIAN_POINT ( 'NONE',  ( -16.09577467286060681, -7.881796084464274266, 67.23187563413577550 ) ) ;
#14318=( BOUNDED_SURFACE ( )  B_SPLINE_SURFACE ( 3, 1, ( 
 ( #1082, #41971 ),
 ( #42211, #19554 ),
 ( #8243, #23503 ),
 ( #23259, #34565 ),
 ( #38504, #4786 ),
 ( #19812, #34811 ),
 ( #16083, #31123 ) ),
 .UNSPECIFIED., .T., .F., .F. ) 
 B_SPLINE_SURFACE_WITH_KNOTS ( ( 4, 3, 4 ),
 ( 2, 2 ),
 ( 0.000000000000000000, 0.5000000000000000000, 1.000000000000000000 ),
 ( 0.000000000000000000, 1.000000000000000000 ),
 .UNSPECIFIED. ) 
 GEOMETRIC_REPRESENTATION_ITEM ( )  RATIONAL_B_SPLINE_SURFACE ( (
 ( 1.000000000000000000, 1.000000000000000000),
 ( 0.3333333333333335369, 0.3333333333333330373),
 ( 0.3333333333333335369, 0.3333333333333330373),
 ( 1.000000000000000000, 1.000000000000000000),
 ( 0.3333333333333333703, 0.3333333333333333703),
 ( 0.3333333333333333703, 0.3333333333333333703),
 ( 1.000000000000000000, 1.000000000000000000) ) ) 
 REPRESENTATION_ITEM ( '' )  SURFACE ( )  );
#14319=ORIENTED_EDGE ( 'NONE', *, *, #2872, .T. ) ;
#14322=VERTEX_POINT ( 'NONE', #45556 ) ;
#14323=CARTESIAN_POINT ( 'NONE',  ( -23.57241774487040331, -19.01643176791860412, 66.02378197632246781 ) ) ;
#14325=CARTESIAN_POINT ( 'NONE',  ( -15.54431827633925778, -7.600127216965169019, 70.78706699909608346 ) ) ;
#14326=ORIENTED_EDGE ( 'NONE', *, *, #15039, .T. ) ;
#14327=CARTESIAN_POINT ( 'NONE',  ( -15.37556480380028745, -25.39340727801265984, 54.49999999999995026 ) ) ;
#14328=ORIENTED_EDGE ( 'NONE', *, *, #40359, .T. ) ;
#14330=CARTESIAN_POINT ( 'NONE',  ( -12.33606046264216083, -19.68942273586096547, 61.40238395048532283 ) ) ;
#14331=ORIENTED_EDGE ( 'NONE', *, *, #18547, .F. ) ;
#14332=CARTESIAN_POINT ( 'NONE',  ( -10.52483499103918874, -17.62059296423454313, 68.35367848399930324 ) ) ;
#14333=CARTESIAN_POINT ( 'NONE',  ( -11.05753694418977773, -11.89913863384178683, 74.85840159189888254 ) ) ;
#14334=CARTESIAN_POINT ( 'NONE',  ( -9.978978019336247840, -14.53486877964845192, 68.01833503670710002 ) ) ;
#14335=ORIENTED_EDGE ( 'NONE', *, *, #14584, .T. ) ;
#14337=ADVANCED_FACE ( 'NONE', ( #11812 ), #3833, .T. ) ;
#14339=CARTESIAN_POINT ( 'NONE',  ( -19.30706890485013005, -22.01740903849647069, 58.64011989901568711 ) ) ;
#14340=CARTESIAN_POINT ( 'NONE',  ( -22.17253171379126897, -20.54993857985014216, 59.02088830234949057 ) ) ;
#14343=CARTESIAN_POINT ( 'NONE',  ( -15.35564863419042858, -21.49796178713217287, 72.11745751386041547 ) ) ;
#14344=CARTESIAN_POINT ( 'NONE',  ( -23.23311957587295495, -18.80921362937865382, 69.70860875969677295 ) ) ;
#14345=EDGE_CURVE ( 'NONE', #20165, #8795, #46987, .T. ) ;
#14347=VERTEX_POINT ( 'NONE', #24105 ) ;
#14349=CARTESIAN_POINT ( 'NONE',  ( -20.78451513435706133, -21.00713107796517320, 62.12943504870421663 ) ) ;
#14350=CARTESIAN_POINT ( 'NONE',  ( -22.78151503426583702, -19.98625364524674097, 72.75905110386234753 ) ) ;
#14351=EDGE_LOOP ( 'NONE', ( #47690, #10525, #46604, #23705, #42663 ) ) ;
#14353=EDGE_CURVE ( 'NONE', #5443, #32972, #27308, .T. ) ;
#14354=CARTESIAN_POINT ( 'NONE',  ( -22.55072583747034543, -9.969711375825740518, 73.48161092416185625 ) ) ;
#14355=CARTESIAN_POINT ( 'NONE',  ( -18.86321414053259105, -7.899510124550229051, 73.98497555292401273 ) ) ;
#14356=EDGE_LOOP ( 'NONE', ( #33731, #28649 ) ) ;
#14357=CARTESIAN_POINT ( 'NONE',  ( -24.38391064099431915, -14.06024038319858960, 73.42271507915008044 ) ) ;
#14359=B_SPLINE_CURVE_WITH_KNOTS ( 'NONE', 3,
 ( #19022, #14081, #29132, #36981, #6967, #3760, #10662, #21743, #11153, #44408 ),
 .UNSPECIFIED., .F., .F.,
 ( 4, 2, 2, 2, 4 ),
 ( 0.6272669072877655738, 0.7522669073072847379, 0.8772669073268037909, 1.002266907346323066, 1.127266907365842119 ),
 .UNSPECIFIED. ) ;
#14361=ADVANCED_FACE ( 'NONE', ( #31733 ), #23981, .T. ) ;
#14362=ORIENTED_EDGE ( 'NONE', *, *, #34209, .F. ) ;
#14365=CARTESIAN_POINT ( 'NONE',  ( -18.82742234287504601, -7.492519652536670627, 70.56406355907934369 ) ) ;
#14366=CARTESIAN_POINT ( 'NONE',  ( -12.35277332135121675, -20.26681466537264242, 68.45162004874669037 ) ) ;
#14367=CARTESIAN_POINT ( 'NONE',  ( -13.12596155740353154, -8.723179898376328012, 60.55294873703923031 ) ) ;
#14369=VERTEX_POINT ( 'NONE', #20654 ) ;
#14373=ORIENTED_EDGE ( 'NONE', *, *, #21809, .F. ) ;
#14374=B_SPLINE_CURVE_WITH_KNOTS ( 'NONE', 3,
 ( #42779, #27507, #19392, #8560, #23585, #38831, #23102, #5351, #46480, #35129 ),
 .UNSPECIFIED., .F., .F.,
 ( 4, 2, 2, 2, 4 ),
 ( 0.6272669072877817831, 0.7522669073072956181, 0.8772669073268095641, 1.002266907346323510, 1.127266907365837234 ),
 .UNSPECIFIED. ) ;
#14377=( BOUNDED_SURFACE ( )  B_SPLINE_SURFACE ( 3, 1, ( 
 ( #2468, #48008 ),
 ( #29294, #33203 ),
 ( #14713, #11072 ),
 ( #21662, #40858 ),
 ( #25839, #29786 ),
 ( #17477, #32506 ),
 ( #2934, #44331 ) ),
 .UNSPECIFIED., .T., .F., .F. ) 
 B_SPLINE_SURFACE_WITH_KNOTS ( ( 4, 3, 4 ),
 ( 2, 2 ),
 ( 0.000000000000000000, 0.5000000000000000000, 1.000000000000000000 ),
 ( 0.000000000000000000, 1.000000000000000000 ),
 .UNSPECIFIED. ) 
 GEOMETRIC_REPRESENTATION_ITEM ( )  RATIONAL_B_SPLINE_SURFACE ( (
 ( 1.000000000000000000, 1.000000000000000000),
 ( 0.3333333333333335369, 0.3333333333333330373),
 ( 0.3333333333333335369, 0.3333333333333330373),
 ( 1.000000000000000000, 1.000000000000000000),
 ( 0.3333333333333333703, 0.3333333333333333703),
 ( 0.3333333333333333703, 0.3333333333333333703),
 ( 1.000000000000000000, 1.000000000000000000) ) ) 
 REPRESENTATION_ITEM ( '' )  SURFACE ( )  );
#14378=CARTESIAN_POINT ( 'NONE',  ( -10.13265761198657167, -13.28029711567731397, 74.87828850252731172 ) ) ;
#14379=EDGE_CURVE ( 'NONE', #19087, #33339, #5743, .T. ) ;
#14380=VERTEX_POINT ( 'NONE', #4915 ) ;
#14384=CARTESIAN_POINT ( 'NONE',  ( -10.11997142774249880, -16.27652841963017138, 71.64088708844454345 ) ) ;
#14385=CARTESIAN_POINT ( 'NONE',  ( -9.989611971821876324, -14.32602191216411569, 64.52657349001064802 ) ) ;
#14386=ADVANCED_FACE ( 'NONE', ( #1695 ), #45695, .T. ) ;
#14389=CARTESIAN_POINT ( 'NONE',  ( -10.62096356601691660, -12.92974252456203743, 60.95420737114066156 ) ) ;
#14390=CARTESIAN_POINT ( 'NONE',  ( -15.31846949587358431, -21.95558135219415163, 72.22388224403276524 ) ) ;
#14391=LINE ( 'NONE', #44729, #42579 ) ;
#14392=EDGE_LOOP ( 'NONE', ( #12985, #47503, #12996, #10050 ) ) ;
#14393=CARTESIAN_POINT ( 'NONE',  ( -10.37424879026167979, -14.74379641705365174, 71.62222930935075738 ) ) ;
#14395=CARTESIAN_POINT ( 'NONE',  ( -21.47456293661849713, -9.038556783377254433, 70.41660404402310292 ) ) ;
#14397=CARTESIAN_POINT ( 'NONE',  ( -19.17604249790256077, -21.63836284480991878, 58.53979515915469278 ) ) ;
#14399=DIRECTION ( 'NONE',  ( -0.9979768094191905359, -0.06357898915123237626, -3.501668460141644652E-17 ) ) ;
#14401=EDGE_CURVE ( 'NONE', #37972, #43339, #43328, .T. ) ;
#14402=CARTESIAN_POINT ( 'NONE',  ( -14.29154966128864857, -8.493214084104669936, 70.73517404774455031 ) ) ;
#14403=EDGE_LOOP ( 'NONE', ( #13865, #5098 ) ) ;
#14404=CARTESIAN_POINT ( 'NONE',  ( -24.15060978519040091, -18.01196315242050261, 59.26024333157867119 ) ) ;
#14406=ORIENTED_EDGE ( 'NONE', *, *, #19430, .T. ) ;
#14407=CARTESIAN_POINT ( 'NONE',  ( -10.96142808812597735, -11.10142881709785101, 64.33537400591416144 ) ) ;
#14408=CARTESIAN_POINT ( 'NONE',  ( -15.55648817577099585, -8.010769314271311003, 74.09457776258329886 ) ) ;
#14409=ORIENTED_EDGE ( 'NONE', *, *, #7580, .F. ) ;
#14411=CARTESIAN_POINT ( 'NONE',  ( -19.61601346313181082, -21.50980264518277707, 65.46486213821819433 ) ) ;
#14412=VERTEX_POINT ( 'NONE', #2886 ) ;
#14415=DIRECTION ( 'NONE',  ( 0.5497669574358331479, -0.8353180786453389128, -7.898837270956392542E-08 ) ) ;
#14417=CARTESIAN_POINT ( 'NONE',  ( -16.92050523043788957, -21.84918965566402704, 65.38131313066115524 ) ) ;
#14418=ADVANCED_FACE ( 'NONE', ( #28998 ), #6835, .T. ) ;
#14419=CARTESIAN_POINT ( 'NONE',  ( -14.84266674508882744, -8.302458032430561019, 60.61996277900374253 ) ) ;
#14421=CARTESIAN_POINT ( 'NONE',  ( -17.83878094755516486, -7.370707184827939074, 60.27399068567451934 ) ) ;
#14422=VERTEX_POINT ( 'NONE', #29247 ) ;
#14423=ORIENTED_EDGE ( 'NONE', *, *, #31751, .T. ) ;
#14425=CARTESIAN_POINT ( 'NONE',  ( -19.91954111600424326, -8.269053586180861615, 74.00631301559766939 ) ) ;
#14426=DIRECTION ( 'NONE',  ( -4.556087730354191539E-06, 5.696494007380787447E-06, -0.9999999999733960587 ) ) ;
#14428=CARTESIAN_POINT ( 'NONE',  ( -18.63018970549565978, -7.457396494496333794, 73.95569010969242640 ) ) ;
#14430=( BOUNDED_CURVE ( )  B_SPLINE_CURVE ( 3, ( #30612, #42167, #45633, #8430 ),
 .UNSPECIFIED., .F., .F. ) 
 B_SPLINE_CURVE_WITH_KNOTS ( ( 4, 4 ),
 ( 0.000000000000000000, 0.4074455897393691739 ),
 .UNSPECIFIED. ) 
 CURVE ( )  GEOMETRIC_REPRESENTATION_ITEM ( )  RATIONAL_B_SPLINE_CURVE ( ( 1.000000000000000000, 0.4567392136813301917, 0.3561768502900296562, 0.6983129098260982826 ) ) 
 REPRESENTATION_ITEM ( '' )  );
#14433=CARTESIAN_POINT ( 'NONE',  ( -24.34625421034940018, -15.85315431188110225, 69.81690982159123848 ) ) ;
#14434=CARTESIAN_POINT ( 'NONE',  ( -19.74200936563729769, -21.46758226568296024, 68.94954551542706156 ) ) ;
#14435=CARTESIAN_POINT ( 'NONE',  ( -10.78905007119639059, -17.04131871017208155, 61.17359741050059796 ) ) ;
#14436=CARTESIAN_POINT ( 'NONE',  ( -11.19252025440407472, -18.89210953133327919, 64.94718283645474344 ) ) ;
#14437=ADVANCED_FACE ( 'NONE', ( #36134 ), #44048, .T. ) ;
#14438=ORIENTED_EDGE ( 'NONE', *, *, #5156, .T. ) ;
#14439=( BOUNDED_SURFACE ( )  B_SPLINE_SURFACE ( 3, 1, ( 
 ( #11196, #41465 ),
 ( #37764, #42201 ),
 ( #30404, #19303 ),
 ( #45420, #11673 ),
 ( #23021, #15841 ),
 ( #3804, #27180 ),
 ( #19545, #34305 ) ),
 .UNSPECIFIED., .T., .F., .F. ) 
 B_SPLINE_SURFACE_WITH_KNOTS ( ( 4, 3, 4 ),
 ( 2, 2 ),
 ( 0.000000000000000000, 0.5000000000000000000, 1.000000000000000000 ),
 ( 0.000000000000000000, 1.000000000000000000 ),
 .UNSPECIFIED. ) 
 GEOMETRIC_REPRESENTATION_ITEM ( )  RATIONAL_B_SPLINE_SURFACE ( (
 ( 1.000000000000000000, 1.000000000000000000),
 ( 0.3333333333333335369, 0.3333333333333330373),
 ( 0.3333333333333335369, 0.3333333333333330373),
 ( 1.000000000000000000, 1.000000000000000000),
 ( 0.3333333333333333703, 0.3333333333333333703),
 ( 0.3333333333333333703, 0.3333333333333333703),
 ( 1.000000000000000000, 1.000000000000000000) ) ) 
 REPRESENTATION_ITEM ( '' )  SURFACE ( )  );
#14440=DIRECTION ( 'NONE',  ( 7.340779720199402358E-07, -8.195271891664201640E-07, 0.9999999999993947064 ) ) ;
#14441=CARTESIAN_POINT ( 'NONE',  ( -21.65477688667505518, -9.232350752012335349, 66.66149992610201025 ) ) ;
#14442=B_SPLINE_CURVE_WITH_KNOTS ( 'NONE', 3,
 ( #23488, #8458, #5251, #34547, #12388, #19796, #585, #26694, #15580, #1069 ),
 .UNSPECIFIED., .F., .F.,
 ( 4, 2, 2, 2, 4 ),
 ( 0.000000000000000000, 0.2500000000000000000, 0.5000000000000000000, 0.7500000000000000000, 1.000000000000000000 ),
 .UNSPECIFIED. ) ;
#14443=ORIENTED_EDGE ( 'NONE', *, *, #10422, .F. ) ;
#14444=CARTESIAN_POINT ( 'NONE',  ( -15.55910223978619200, -7.596364071707596644, 70.80263970476339352 ) ) ;
#14445=CARTESIAN_POINT ( 'NONE',  ( -10.13546849559099883, -16.35223934790467837, 71.60783702123018202 ) ) ;
#14446=ORIENTED_EDGE ( 'NONE', *, *, #23462, .F. ) ;
#14447=EDGE_CURVE ( 'NONE', #34717, #3552, #28992, .T. ) ;
#14448=DIRECTION ( 'NONE',  ( 0.3566357048164924826, -0.9342435303763380050, 8.054691247936225743E-09 ) ) ;
#14449=( BOUNDED_CURVE ( )  B_SPLINE_CURVE ( 3, ( #37498, #26688, #41451, #16062 ),
 .UNSPECIFIED., .F., .F. ) 
 B_SPLINE_CURVE_WITH_KNOTS ( ( 4, 4 ),
 ( 0.4074455897393585713, 0.5000000000000000000 ),
 .UNSPECIFIED. ) 
 CURVE ( )  GEOMETRIC_REPRESENTATION_ITEM ( )  RATIONAL_B_SPLINE_CURVE ( ( 0.6983129098260824064, 0.7760317562606839914, 0.8765941196519885237, 0.9999999999999921174 ) ) 
 REPRESENTATION_ITEM ( '' )  );
#14451=VECTOR ( 'NONE', #33262, 1000.000000000000227 ) ;
#14453=ORIENTED_EDGE ( 'NONE', *, *, #44169, .F. ) ;
#14454=CARTESIAN_POINT ( 'NONE',  ( -23.96969171478034610, -17.42802645644465542, 66.24357243629151526 ) ) ;
#14456=CARTESIAN_POINT ( 'NONE',  ( -22.07805708657739885, -20.69058616546009333, 54.27966884056654351 ) ) ;
#14459=CARTESIAN_POINT ( 'NONE',  ( -23.37999588001404661, -18.58199455739222827, 69.57899840282863124 ) ) ;
#14460=CARTESIAN_POINT ( 'NONE',  ( -11.09242024638942148, -18.73509009507580458, 61.37687196085482810 ) ) ;
#14461=B_SPLINE_CURVE_WITH_KNOTS ( 'NONE', 3,
 ( #23966, #2027, #5245, #35269, #28619, #39214, #16551, #9187, #24205, #20513 ),
 .UNSPECIFIED., .F., .F.,
 ( 4, 2, 2, 2, 4 ),
 ( 0.1272669073658570793, 0.2522669073463328360, 0.3772669073268085649, 0.5022669073072844048, 0.6272669072877601337 ),
 .UNSPECIFIED. ) ;
#14462=B_SPLINE_CURVE_WITH_KNOTS ( 'NONE', 3,
 ( #18255, #44883, #10417, #14064, #29113, #25426, #29357, #47597, #18502, #44388 ),
 .UNSPECIFIED., .F., .F.,
 ( 4, 2, 2, 2, 4 ),
 ( 0.000000000000000000, 0.2500000000000000000, 0.5000000000000000000, 0.7500000000000000000, 1.000000000000000000 ),
 .UNSPECIFIED. ) ;
#14463=ORIENTED_EDGE ( 'NONE', *, *, #2901, .F. ) ;
#14464=CARTESIAN_POINT ( 'NONE',  ( -9.990623027812100432, -14.31192454061599229, 64.57299275950818185 ) ) ;
#14465=EDGE_CURVE ( 'NONE', #14468, #47695, #22096, .T. ) ;
#14468=VERTEX_POINT ( 'NONE', #21852 ) ;
#14469=ORIENTED_EDGE ( 'NONE', *, *, #12879, .T. ) ;
#14470=CARTESIAN_POINT ( 'NONE',  ( -23.39277566991647817, -10.35052415317939278, 59.74170096327360113 ) ) ;
#14471=CARTESIAN_POINT ( 'NONE',  ( -24.69852180232685157, -16.41745880042978101, 59.30827708941524889 ) ) ;
#14475=DIRECTION ( 'NONE',  ( -0.3478314405900310158, -0.9375570856950865561, 0.000000000000000000 ) ) ;
#14478=CARTESIAN_POINT ( 'NONE',  ( -10.66703338591908690, -12.79807911521252883, 64.41836111017862265 ) ) ;
#14482=CARTESIAN_POINT ( 'NONE',  ( -24.87385082706414607, -14.87839859077033822, 59.49946141495512819 ) ) ;
#14483=CARTESIAN_POINT ( 'NONE',  ( -13.57788212914492476, -8.959029760704318335, 60.51120652236025421 ) ) ;
#14484=EDGE_CURVE ( 'NONE', #43727, #24972, #45978, .T. ) ;
#14485=ORIENTED_EDGE ( 'NONE', *, *, #30763, .F. ) ;
#14486=EDGE_CURVE ( 'NONE', #26903, #2787, #14143, .T. ) ;
#14489=ADVANCED_FACE ( 'NONE', ( #10768 ), #34021, .T. ) ;
#14490=CARTESIAN_POINT ( 'NONE',  ( -11.19706266256277694, -11.50303319689152737, 67.63336710488009373 ) ) ;
#14492=DIRECTION ( 'NONE',  ( -0.9930145540378111368, 0.1179919296777755672, 4.526730167978065139E-08 ) ) ;
#14493=CARTESIAN_POINT ( 'NONE',  ( -10.00963232195547903, -14.08228650966967876, 61.01797661620253166 ) ) ;
#14494=CARTESIAN_POINT ( 'NONE',  ( -11.64235247690698571, -18.84330696305777408, 68.51689631558762983 ) ) ;
#14495=ORIENTED_EDGE ( 'NONE', *, *, #34287, .F. ) ;
#14496=CARTESIAN_POINT ( 'NONE',  ( -24.47628618758622210, -12.40716135712818868, 73.34887263294206150 ) ) ;
#14497=CARTESIAN_POINT ( 'NONE',  ( -13.06825169942196752, -9.255684228991221119, 74.46356075877366720 ) ) ;
#14498=ORIENTED_EDGE ( 'NONE', *, *, #45151, .F. ) ;
#14500=CARTESIAN_POINT ( 'NONE',  ( -23.06636451794179976, -10.57604847539621851, 63.37186202593429130 ) ) ;
#14501=CARTESIAN_POINT ( 'NONE',  ( -16.98261445675647963, -21.79527095473675402, 72.46543221550747660 ) ) ;
#14502=ORIENTED_EDGE ( 'NONE', *, *, #17968, .T. ) ;
#14503=ORIENTED_EDGE ( 'NONE', *, *, #24110, .F. ) ;
#14504=CARTESIAN_POINT ( 'NONE',  ( -23.79119299285383349, -10.94096587987842639, 73.46854977554494326 ) ) ;
#14505=CARTESIAN_POINT ( 'NONE',  ( -24.39022378835582927, -14.12080876765324078, 69.87948639740776002 ) ) ;
#14506=ORIENTED_EDGE ( 'NONE', *, *, #34445, .F. ) ;
#14507=CARTESIAN_POINT ( 'NONE',  ( -16.26183769579148475, -7.855670737815882987, 60.50028478907628937 ) ) ;
#14508=CARTESIAN_POINT ( 'NONE',  ( -24.17147434587301191, -12.75550446831573126, 73.65714286828524848 ) ) ;
#14511=CARTESIAN_POINT ( 'NONE',  ( -10.05522069275589736, -15.90572865272950409, 64.60747954325734099 ) ) ;
#14512=CARTESIAN_POINT ( 'NONE',  ( -22.96481576609224717, -19.16891988936071556, 58.89882756593014790 ) ) ;
#14513=DIRECTION ( 'NONE',  ( 0.3996021513128669711, 0.9166886716143756164, 9.834836654444491158E-09 ) ) ;
#14515=CARTESIAN_POINT ( 'NONE',  ( -16.94392004664433671, -22.24372332546570163, 72.36554421717424646 ) ) ;
#14516=CARTESIAN_POINT ( 'NONE',  ( -17.42409385541300892, -14.80920654474439502, 75.49999999999994316 ) ) ;
#14517=CARTESIAN_POINT ( 'NONE',  ( -14.48623784902251899, -7.962796613987291217, 63.96791570607779676 ) ) ;
#14519=FACE_OUTER_BOUND ( 'NONE', #41995, .T. ) ;
#14524=ORIENTED_EDGE ( 'NONE', *, *, #26409, .T. ) ;
#14526=CARTESIAN_POINT ( 'NONE',  ( -18.30727046116018286, -21.75326869042403288, 69.11514702556002021 ) ) ;
#14528=VERTEX_POINT ( 'NONE', #19373 ) ;
#14529=CARTESIAN_POINT ( 'NONE',  ( -17.72612443559818018, -7.765381109175947927, 60.36588690973874094 ) ) ;
#14530=CARTESIAN_POINT ( 'NONE',  ( -14.09390608941906819, -21.02325857983911561, 72.22047898906316732 ) ) ;
#14531=CARTESIAN_POINT ( 'NONE',  ( -13.40146611816620847, -9.019296439419454359, 60.73390453098559050 ) ) ;
#14532=CARTESIAN_POINT ( 'NONE',  ( -20.69509153224808173, -8.115601224564374050, 63.49616927690831858 ) ) ;
#14533=CARTESIAN_POINT ( 'NONE',  ( -12.32278866559117780, -19.67576434477648917, 61.41150688479135766 ) ) ;
#14534=CARTESIAN_POINT ( 'NONE',  ( -24.30164805153987473, -16.37256343635084477, 63.00817566860099106 ) ) ;
#14536=CARTESIAN_POINT ( 'NONE',  ( -11.46592951257400905, -19.28193112475830873, 71.82539333254983660 ) ) ;
#14537=CARTESIAN_POINT ( 'NONE',  ( -16.71067917923000579, -21.77319752884913129, 68.71177304229871652 ) ) ;
#14538=ORIENTED_EDGE ( 'NONE', *, *, #7295, .F. ) ;
#14539=CARTESIAN_POINT ( 'NONE',  ( -24.11691640979936224, -11.53669002245029951, 63.14556576031020541 ) ) ;
#14540=CARTESIAN_POINT ( 'NONE',  ( -10.48085305489969521, -13.91959585118948617, 57.74825035244229809 ) ) ;
#14541=CARTESIAN_POINT ( 'NONE',  ( -24.71633098454773148, -13.28334072004885869, 59.52414474877395634 ) ) ;
#14542=CARTESIAN_POINT ( 'NONE',  ( -24.29424039954640691, -13.46050364628763063, 59.43438299228309774 ) ) ;
#14543=CARTESIAN_POINT ( 'NONE',  ( -24.13185811504778755, -12.61356036044664464, 66.45813649863244166 ) ) ;
#14544=FACE_OUTER_BOUND ( 'NONE', #22056, .T. ) ;
#14545=CARTESIAN_POINT ( 'NONE',  ( -15.93879930885702656, -7.917138641544857691, 67.15479422225767792 ) ) ;
#14546=EDGE_CURVE ( 'NONE', #31797, #7279, #23344, .T. ) ;
#14550=VERTEX_POINT ( 'NONE', #18387 ) ;
#14551=EDGE_CURVE ( 'NONE', #26197, #39806, #39733, .T. ) ;
#14552=ADVANCED_FACE ( 'NONE', ( #48433 ), #27700, .T. ) ;
#14554=CARTESIAN_POINT ( 'NONE',  ( -11.68672781637937419, -10.05669048882576533, 67.68392176937598492 ) ) ;
#14555=B_SPLINE_CURVE_WITH_KNOTS ( 'NONE', 3,
 ( #7992, #45405, #12147, #15332, #30148, #27168, #37751, #42189, #30634, #34055 ),
 .UNSPECIFIED., .F., .F.,
 ( 4, 2, 2, 2, 4 ),
 ( 0.000000000000000000, 0.2500000000000000000, 0.5000000000000000000, 0.7500000000000000000, 1.000000000000000000 ),
 .UNSPECIFIED. ) ;
#14557=CARTESIAN_POINT ( 'NONE',  ( -24.61808062994217394, -12.87247312369571439, 66.42529869958860900 ) ) ;
#14558=CARTESIAN_POINT ( 'NONE',  ( -15.53801481854660871, -7.601731716485351065, 70.74843289815109415 ) ) ;
#14560=CARTESIAN_POINT ( 'NONE',  ( -23.08399920647563519, -9.964749700819742984, 66.73456405495493016 ) ) ;
#14561=CARTESIAN_POINT ( 'NONE',  ( -12.50766613833180152, -19.86205114983803810, 64.86674886870797252 ) ) ;
#14562=( BOUNDED_SURFACE ( )  B_SPLINE_SURFACE ( 3, 1, ( 
 ( #43107, #12582 ),
 ( #12820, #19977 ),
 ( #34979, #13286 ),
 ( #38925, #43606 ),
 ( #35222, #39416 ),
 ( #9864, #1247 ),
 ( #1497, #4967 ) ),
 .UNSPECIFIED., .T., .F., .F. ) 
 B_SPLINE_SURFACE_WITH_KNOTS ( ( 4, 3, 4 ),
 ( 2, 2 ),
 ( 0.000000000000000000, 0.5000000000000000000, 1.000000000000000000 ),
 ( 0.000000000000000000, 1.000000000000000000 ),
 .UNSPECIFIED. ) 
 GEOMETRIC_REPRESENTATION_ITEM ( )  RATIONAL_B_SPLINE_SURFACE ( (
 ( 1.000000000000000000, 1.000000000000000000),
 ( 0.3333333333333335369, 0.3333333333333330373),
 ( 0.3333333333333335369, 0.3333333333333330373),
 ( 1.000000000000000000, 1.000000000000000000),
 ( 0.3333333333333333703, 0.3333333333333333703),
 ( 0.3333333333333333703, 0.3333333333333333703),
 ( 1.000000000000000000, 1.000000000000000000) ) ) 
 REPRESENTATION_ITEM ( '' )  SURFACE ( )  );
#14564=CARTESIAN_POINT ( 'NONE',  ( -13.86248685510225087, -21.35271135026633971, 72.07607701462937655 ) ) ;
#14567=CARTESIAN_POINT ( 'NONE',  ( -10.49754805884589004, -17.55449835891870691, 68.28377192865846723 ) ) ;
#14568=FACE_OUTER_BOUND ( 'NONE', #23630, .T. ) ;
#14570=ORIENTED_EDGE ( 'NONE', *, *, #23834, .T. ) ;
#14572=ADVANCED_FACE ( 'NONE', ( #15413 ), #35880, .T. ) ;
#14573=CARTESIAN_POINT ( 'NONE',  ( -15.65537882804863834, -7.980949930599003039, 67.34826994618644846 ) ) ;
#14574=( BOUNDED_CURVE ( )  B_SPLINE_CURVE ( 3, ( #43601, #43098, #35216, #2464 ),
 .UNSPECIFIED., .F., .F. ) 
 B_SPLINE_CURVE_WITH_KNOTS ( ( 4, 4 ),
 ( 0.9074455897393672865, 1.000000000000000000 ),
 .UNSPECIFIED. ) 
 CURVE ( )  GEOMETRIC_REPRESENTATION_ITEM ( )  RATIONAL_B_SPLINE_CURVE ( ( 0.6983129098260870693, 0.7760317562606930952, 0.8765941196519974055, 1.000000000000000000 ) ) 
 REPRESENTATION_ITEM ( '' )  );
#14575=CARTESIAN_POINT ( 'NONE',  ( -16.06050865347321732, -9.480920197610746669, 53.49899999999994549 ) ) ;
#14576=PLANE ( 'NONE',  #2483 ) ;
#14577=ORIENTED_EDGE ( 'NONE', *, *, #33178, .F. ) ;
#14578=CARTESIAN_POINT ( 'NONE',  ( -10.78978130820344994, -12.42417047965500743, 57.62857332104950814 ) ) ;
#14579=FACE_OUTER_BOUND ( 'NONE', #7780, .T. ) ;
#14583=ORIENTED_EDGE ( 'NONE', *, *, #6824, .T. ) ;
#14584=EDGE_CURVE ( 'NONE', #30119, #5861, #39114, .T. ) ;
#14585=CARTESIAN_POINT ( 'NONE',  ( -16.39155704513022016, -21.78318439201321866, 61.75568132354042206 ) ) ;
#14586=FACE_OUTER_BOUND ( 'NONE', #35089, .T. ) ;
#14587=ORIENTED_EDGE ( 'NONE', *, *, #12174, .F. ) ;
#14592=CARTESIAN_POINT ( 'NONE',  ( -19.83743235192402210, -21.38007574497211039, 69.22777528876429187 ) ) ;
#14593=( BOUNDED_CURVE ( )  B_SPLINE_CURVE ( 3, ( #38525, #7358, #26296, #22356 ),
 .UNSPECIFIED., .F., .F. ) 
 B_SPLINE_CURVE_WITH_KNOTS ( ( 4, 4 ),
 ( 0.4074455897393582937, 0.5000000000000000000 ),
 .UNSPECIFIED. ) 
 CURVE ( )  GEOMETRIC_REPRESENTATION_ITEM ( )  RATIONAL_B_SPLINE_CURVE ( ( 0.6983129098260915102, 0.7760317562606909858, 0.8765941196519919654, 0.9999999999999905631 ) ) 
 REPRESENTATION_ITEM ( '' )  );
#14594=AXIS2_PLACEMENT_3D ( 'NONE', #7227, #33524, #41185 ) ;
#14595=CARTESIAN_POINT ( 'NONE',  ( -10.20995793436087595, -16.92613924295324423, 54.02312124697527906 ) ) ;
#14596=EDGE_LOOP ( 'NONE', ( #40615, #19259 ) ) ;
#14600=CARTESIAN_POINT ( 'NONE',  ( -10.99586753834015695, -11.04334891231907534, 60.86381058728009208 ) ) ;
#14601=CARTESIAN_POINT ( 'NONE',  ( -24.79676515827134153, -15.88070078827938048, 69.65590621464686194 ) ) ;
#14603=LINE ( 'NONE', #25975, #32294 ) ;
#14605=ORIENTED_EDGE ( 'NONE', *, *, #47053, .F. ) ;
#14607=EDGE_CURVE ( 'NONE', #34613, #37103, #5414, .T. ) ;
#14610=EDGE_CURVE ( 'NONE', #40496, #6954, #32116, .T. ) ;
#14616=DIRECTION ( 'NONE',  ( -3.289814948237356682E-07, -7.277561423860909391E-07, 0.9999999999996810329 ) ) ;
#14617=EDGE_CURVE ( 'NONE', #31313, #46311, #41477, .T. ) ;
#14618=CARTESIAN_POINT ( 'NONE',  ( -24.40527833060663454, -14.29480840995819335, 69.95275285367253559 ) ) ;
#14619=ORIENTED_EDGE ( 'NONE', *, *, #18953, .F. ) ;
#14620=FACE_OUTER_BOUND ( 'NONE', #4494, .T. ) ;
#14622=ORIENTED_EDGE ( 'NONE', *, *, #38306, .F. ) ;
#14623=CARTESIAN_POINT ( 'NONE',  ( -22.14851325272248062, -9.572347091288939680, 60.13659902389549927 ) ) ;
#14624=CARTESIAN_POINT ( 'NONE',  ( -18.15846822104387925, -21.77219406509840738, 69.00441818213361955 ) ) ;
#14625=CARTESIAN_POINT ( 'NONE',  ( -24.41081920617251200, -17.39538559163089815, 69.51316173558434741 ) ) ;
#14626=CARTESIAN_POINT ( 'NONE',  ( -10.42288197367123459, -12.26238041423571623, 57.43583165137763302 ) ) ;
#14628=ORIENTED_EDGE ( 'NONE', *, *, #37841, .F. ) ;
#14629=CARTESIAN_POINT ( 'NONE',  ( -19.04074814492602030, -7.997133300950575396, 66.97242149538513445 ) ) ;
#14631=CARTESIAN_POINT ( 'NONE',  ( -13.49145512112739631, -18.65424914341562612, 53.49899999999994549 ) ) ;
#14632=DIRECTION ( 'NONE',  ( 0.5820088206811424580, -0.8131824719270213109, 7.019974882119936121E-08 ) ) ;
#14635=CARTESIAN_POINT ( 'NONE',  ( -17.13721359355439233, -7.364564939118506182, 70.62889357192571538 ) ) ;
#14638=FACE_BOUND ( 'NONE', #25582, .T. ) ;
#14640=CARTESIAN_POINT ( 'NONE',  ( -18.31357888663955080, -21.80286911112441217, 69.11514702303101387 ) ) ;
#14641=CARTESIAN_POINT ( 'NONE',  ( -23.44637151138313058, -19.19494152140299548, 62.50406877911783710 ) ) ;
#14642=CARTESIAN_POINT ( 'NONE',  ( -13.89389072038462025, -21.36980434119256600, 72.11103101793651149 ) ) ;
#14643=FACE_OUTER_BOUND ( 'NONE', #8204, .T. ) ;
#14647=CARTESIAN_POINT ( 'NONE',  ( -10.16748990304072464, -13.12235252378331651, 71.39323974795351546 ) ) ;
#14648=ORIENTED_EDGE ( 'NONE', *, *, #4316, .T. ) ;
#14649=CARTESIAN_POINT ( 'NONE',  ( -16.09337498760136853, -22.13948385882417824, 58.40090183616962349 ) ) ;
#14650=CARTESIAN_POINT ( 'NONE',  ( -13.52494119223468338, -20.62276537180227720, 58.27323320193088563 ) ) ;
#14651=ORIENTED_EDGE ( 'NONE', *, *, #38747, .T. ) ;
#14653=CARTESIAN_POINT ( 'NONE',  ( -15.56683366104601696, -8.060027224340267082, 70.68277797453286837 ) ) ;
#14654=CARTESIAN_POINT ( 'NONE',  ( -22.24952110180534604, -19.88199308653408792, 69.24588173298749894 ) ) ;
#14657=CARTESIAN_POINT ( 'NONE',  ( -10.58706256399181100, -13.30549982004886012, 74.96201107970274791 ) ) ;
#14658=ADVANCED_FACE ( 'NONE', ( #45862 ), #30361, .T. ) ;
#14659=CARTESIAN_POINT ( 'NONE',  ( -24.15187520166839974, -12.87586873588168324, 66.31749134914322497 ) ) ;
#14660=CARTESIAN_POINT ( 'NONE',  ( -17.60291880755090332, -7.361353052781006490, 63.70057029387179881 ) ) ;
#14661=CARTESIAN_POINT ( 'NONE',  ( -14.79254118299126119, -21.77901061722586817, 61.74262151019149059 ) ) ;
#14664=ORIENTED_EDGE ( 'NONE', *, *, #43440, .F. ) ;
#14666=CARTESIAN_POINT ( 'NONE',  ( -17.25805186741143871, -7.753187986760909034, 63.70624286928425306 ) ) ;
#14667=ADVANCED_FACE ( 'NONE', ( #16031 ), #27128, .T. ) ;
#14669=CARTESIAN_POINT ( 'NONE',  ( -21.92639021642452946, -9.447133411642054668, 63.30226860340928852 ) ) ;
#14671=( BOUNDED_CURVE ( )  B_SPLINE_CURVE ( 3, ( #4046, #8709, #19787, #34792 ),
 .UNSPECIFIED., .F., .F. ) 
 B_SPLINE_CURVE_WITH_KNOTS ( ( 4, 4 ),
 ( 0.5000000000000000000, 0.9074455897393621795 ),
 .UNSPECIFIED. ) 
 CURVE ( )  GEOMETRIC_REPRESENTATION_ITEM ( )  RATIONAL_B_SPLINE_CURVE ( ( 1.000000000000031530, 0.4567392136813390180, 0.3561768502900107825, 0.6983129098260809631 ) ) 
 REPRESENTATION_ITEM ( '' )  );
#14673=DIRECTION ( 'NONE',  ( 0.3224496555704362000, 0.8691421305882578441, 0.3749909018349790180 ) ) ;
#14674=ORIENTED_EDGE ( 'NONE', *, *, #3655, .T. ) ;
#14681=ORIENTED_EDGE ( 'NONE', *, *, #16181, .T. ) ;
#14682=CARTESIAN_POINT ( 'NONE',  ( -22.92319755143357085, -10.39759026177046763, 63.37185995336191979 ) ) ;
#14683=LINE ( 'NONE', #29754, #7590 ) ;
#14684=ORIENTED_EDGE ( 'NONE', *, *, #12140, .T. ) ;
#14687=FACE_OUTER_BOUND ( 'NONE', #45372, .T. ) ;
#14688=EDGE_LOOP ( 'NONE', ( #35995, #36485 ) ) ;
#14690=AXIS2_PLACEMENT_3D ( 'NONE', #39898, #3434, #44336 ) ;
#14693=DIRECTION ( 'NONE',  ( 1.404489475409085785E-08, -6.428047479010519175E-07, -0.9999999999997932765 ) ) ;
#14694=CARTESIAN_POINT ( 'NONE',  ( -11.50075484580269070, -18.54176165173950253, 64.97537046917975090 ) ) ;
#14695=ORIENTED_EDGE ( 'NONE', *, *, #36386, .F. ) ;
#14697=CARTESIAN_POINT ( 'NONE',  ( -18.53556552080321751, -22.17591605216722428, 72.40015545304112266 ) ) ;
#14698=ORIENTED_EDGE ( 'NONE', *, *, #25362, .F. ) ;
#14699=CARTESIAN_POINT ( 'NONE',  ( -17.42409385541300892, -14.80920654474439679, 47.99999999999994316 ) ) ;
#14700=AXIS2_PLACEMENT_3D ( 'NONE', #3782, #18793, #41439 ) ;
#14701=CARTESIAN_POINT ( 'NONE',  ( -11.10837990474057158, -18.76092553618217451, 61.39898045628379464 ) ) ;
#14702=CARTESIAN_POINT ( 'NONE',  ( -23.72641715273374530, -11.63183476396761407, 70.03643756225406491 ) ) ;
#14703=EDGE_LOOP ( 'NONE', ( #27756, #6562, #29997, #7440, #39704 ) ) ;
#14704=CARTESIAN_POINT ( 'NONE',  ( -19.89775169278732392, -21.83667719550688346, 69.11295222586642240 ) ) ;
#14706=CARTESIAN_POINT ( 'NONE',  ( -23.29918339618657086, -19.39037464299967439, 58.99915238703562181 ) ) ;
#14708=ORIENTED_EDGE ( 'NONE', *, *, #8917, .F. ) ;
#14710=CARTESIAN_POINT ( 'NONE',  ( -16.87202378910036771, -7.830949141774897981, 74.18691624321796496 ) ) ;
#14711=CARTESIAN_POINT ( 'NONE',  ( -23.46741908093438767, -19.16603997859080266, 62.53902161361033052 ) ) ;
#14713=CARTESIAN_POINT ( 'NONE',  ( -22.79444606840252874, -10.23710104419528122, 62.95697184964878090 ) ) ;
#14714=( BOUNDED_CURVE ( )  B_SPLINE_CURVE ( 3, ( #43380, #12356, #16035, #27376 ),
 .UNSPECIFIED., .F., .F. ) 
 B_SPLINE_CURVE_WITH_KNOTS ( ( 4, 4 ),
 ( 0.9074455897393653991, 1.000000000000000000 ),
 .UNSPECIFIED. ) 
 CURVE ( )  GEOMETRIC_REPRESENTATION_ITEM ( )  RATIONAL_B_SPLINE_CURVE ( ( 0.6983129098260982826, 0.7760317562607027542, 0.8765941196520032896, 1.000000000000000000 ) ) 
 REPRESENTATION_ITEM ( '' )  );
#14716=FACE_OUTER_BOUND ( 'NONE', #45713, .T. ) ;
#14717=CARTESIAN_POINT ( 'NONE',  ( -24.03783269458455862, -17.25936868619852760, 65.82868649746481537 ) ) ;
#14719=ORIENTED_EDGE ( 'NONE', *, *, #31494, .T. ) ;
#14720=B_SPLINE_CURVE_WITH_KNOTS ( 'NONE', 3,
 ( #44683, #11188, #29903, #26203, #26693, #18549, #7751, #10938, #41214, #7503 ),
 .UNSPECIFIED., .F., .F.,
 ( 4, 2, 2, 2, 4 ),
 ( 0.1272669073658150574, 0.2522669073463055245, 0.3772669073267960194, 0.5022669073072865142, 0.6272669072877770091 ),
 .UNSPECIFIED. ) ;
#14722=CARTESIAN_POINT ( 'NONE',  ( -18.26818317795011737, -21.80864274563727889, 68.82074505211160442 ) ) ;
#14724=( BOUNDED_CURVE ( )  B_SPLINE_CURVE ( 3, ( #36006, #33026, #47363, #29596 ),
 .UNSPECIFIED., .F., .F. ) 
 B_SPLINE_CURVE_WITH_KNOTS ( ( 4, 4 ),
 ( 4.712388980384690562, 4.921828490624009511 ),
 .UNSPECIFIED. ) 
 CURVE ( )  GEOMETRIC_REPRESENTATION_ITEM ( )  RATIONAL_B_SPLINE_CURVE ( ( 1.000000000000000000, 0.9963479302455156006, 0.9963479302455156006, 1.000000000000000000 ) ) 
 REPRESENTATION_ITEM ( '' )  );
#14726=ORIENTED_EDGE ( 'NONE', *, *, #1209, .T. ) ;
#14728=VERTEX_POINT ( 'NONE', #48295 ) ;
#14729=CARTESIAN_POINT ( 'NONE',  ( -17.03007621496013968, -7.369466030635982712, 74.12164781354181287 ) ) ;
#14731=EDGE_CURVE ( 'NONE', #33555, #28685, #12302, .T. ) ;
#14732=CARTESIAN_POINT ( 'NONE',  ( -13.35181980949104741, -21.04778605225073207, 61.70920450351935216 ) ) ;
#14733=CARTESIAN_POINT ( 'NONE',  ( -10.18401502636761968, -13.05277926903019470, 71.32333192088977114 ) ) ;
#14735=EDGE_CURVE ( 'NONE', #17705, #46048, #25536, .T. ) ;
#14736=EDGE_LOOP ( 'NONE', ( #18470, #20370, #5418, #41506, #30709 ) ) ;
#14737=B_SPLINE_CURVE_WITH_KNOTS ( 'NONE', 3,
 ( #6376, #2190, #32244, #28545, #24850, #2437, #32478, #21870, #14444, #11776 ),
 .UNSPECIFIED., .F., .F.,
 ( 4, 2, 2, 2, 4 ),
 ( 0.1272669073659020711, 0.2522669073463749134, 0.3772669073268477558, 0.5022669073073343649, 0.6272669072878209739 ),
 .UNSPECIFIED. ) ;
#14742=CARTESIAN_POINT ( 'NONE',  ( -22.14090652532222236, -20.04928072148792495, 62.51967078134249078 ) ) ;
#14743=EDGE_CURVE ( 'NONE', #40402, #596, #35009, .T. ) ;
#14744=CARTESIAN_POINT ( 'NONE',  ( -24.17271849214968071, -12.95015691860989371, 66.60246741689840633 ) ) ;
#14745=DIRECTION ( 'NONE',  ( 0.6408936281290996684, 0.7676297007174210929, 4.260501105223829223E-08 ) ) ;
#14746=ORIENTED_EDGE ( 'NONE', *, *, #5457, .F. ) ;
#14747=CARTESIAN_POINT ( 'NONE',  ( -17.54761319933287211, -7.808689222983000278, 67.13112577798570157 ) ) ;
#14749=CARTESIAN_POINT ( 'NONE',  ( -19.50997552649656086, -21.96132259753523996, 62.25149580216906742 ) ) ;
#14750=DIRECTION ( 'NONE',  ( -0.8356905716187448263, 0.5492005722024784209, 7.728900804118606451E-08 ) ) ;
#14752=CARTESIAN_POINT ( 'NONE',  ( -13.29676203468008033, -8.606078807347360637, 57.08312357396523140 ) ) ;
#14753=LINE ( 'NONE', #41141, #5361 ) ;
#14756=CARTESIAN_POINT ( 'NONE',  ( -14.32608993321936453, -8.532007372683787949, 67.48648493512258995 ) ) ;
#14757=AXIS2_PLACEMENT_3D ( 'NONE', #18306, #33317, #33562 ) ;
#14758=EDGE_CURVE ( 'NONE', #46590, #43248, #10719, .T. ) ;
#14759=CARTESIAN_POINT ( 'NONE',  ( -24.26499744607890818, -17.75976858747020160, 62.65856309191605789 ) ) ;
#14760=PLANE ( 'NONE',  #48106 ) ;
#14761=CARTESIAN_POINT ( 'NONE',  ( -16.63294949632448905, -21.81482455919772789, 65.52004579927108807 ) ) ;
#14764=EDGE_CURVE ( 'NONE', #35214, #22721, #3904, .T. ) ;
#14766=CARTESIAN_POINT ( 'NONE',  ( -14.41428173599358331, -7.994163662063686893, 63.97474278339937115 ) ) ;
#14769=DIRECTION ( 'NONE',  ( -0.4780674886490096087, 0.8783231047267435754, 5.292596395488305015E-08 ) ) ;
#14770=VERTEX_POINT ( 'NONE', #17760 ) ;
#14773=CARTESIAN_POINT ( 'NONE',  ( -14.98927377128279126, -8.246306944878790901, 56.84999999999994458 ) ) ;
#14774=EDGE_LOOP ( 'NONE', ( #24661, #280 ) ) ;
#14775=DIRECTION ( 'NONE',  ( -0.6323592902076723421, -0.7746752403995151859, 4.984538757074985308E-08 ) ) ;
#14776=CARTESIAN_POINT ( 'NONE',  ( -24.05059673655033947, -17.06518960458298650, 73.18336032079744768 ) ) ;
#14777=CARTESIAN_POINT ( 'NONE',  ( -11.32868395029271724, -18.25189577030657517, 57.82331260959011843 ) ) ;
#14778=VECTOR ( 'NONE', #33604, 1000.000000000000000 ) ;
#14779=CARTESIAN_POINT ( 'NONE',  ( -14.45498764112879186, -8.410827627250604621, 71.02957685130120069 ) ) ;
#14780=CARTESIAN_POINT ( 'NONE',  ( -20.19053640067075506, -7.838066347919499854, 47.99999999999994316 ) ) ;
#14781=EDGE_CURVE ( 'NONE', #6686, #9124, #47819, .T. ) ;
#14782=CARTESIAN_POINT ( 'NONE',  ( -18.11889201384288128, -21.82488578508536747, 65.34532159284481168 ) ) ;
#14784=CARTESIAN_POINT ( 'NONE',  ( -11.46606301615817713, -19.28211147136272174, 71.84719208600056106 ) ) ;
#14785=DIRECTION ( 'NONE',  ( -5.731567514496413899E-31, -1.020425574103664789E-16, -1.000000000000000000 ) ) ;
#14787=CARTESIAN_POINT ( 'NONE',  ( -13.21312298333807611, -8.663458122980285836, 60.58950274328479679 ) ) ;
#14788=CARTESIAN_POINT ( 'NONE',  ( -21.50272164136802999, -9.054240346128722194, 66.66149779378484652 ) ) ;
#14789=CARTESIAN_POINT ( 'NONE',  ( -12.07145959968993409, -19.99109779731879399, 61.49704379391130260 ) ) ;
#14790=CYLINDRICAL_SURFACE ( 'NONE', #44488, 0.1500000000000054068 ) ;
#14792=CARTESIAN_POINT ( 'NONE',  ( -14.53767063111817137, -21.24453063237525541, 58.58106478802027084 ) ) ;
#14793=CARTESIAN_POINT ( 'NONE',  ( -23.35641471936834535, -10.99444570894131168, 73.24704464419542660 ) ) ;
#14794=ORIENTED_EDGE ( 'NONE', *, *, #47350, .T. ) ;
#14795=VERTEX_POINT ( 'NONE', #29105 ) ;
#14798=CARTESIAN_POINT ( 'NONE',  ( -22.92319839529956838, -10.39759132684999265, 63.22185995336808162 ) ) ;
#14805=CARTESIAN_POINT ( 'NONE',  ( -24.61605457543312525, -12.86511826566283290, 66.41751344402152313 ) ) ;
#14806=CARTESIAN_POINT ( 'NONE',  ( -15.61361955732275497, -7.582487114453736687, 70.71715703711943490 ) ) ;
#14808=EDGE_CURVE ( 'NONE', #43944, #28462, #19211, .T. ) ;
#14809=CARTESIAN_POINT ( 'NONE',  ( -15.95707209241614422, -7.504986913482371236, 63.85506412386598640 ) ) ;
#14811=CARTESIAN_POINT ( 'NONE',  ( -22.05923648098858791, -20.05472392750071720, 62.23439162613904330 ) ) ;
#14812=VERTEX_POINT ( 'NONE', #35917 ) ;
#14813=CARTESIAN_POINT ( 'NONE',  ( -13.11946129443726861, -9.225960368241006293, 67.37942785707224402 ) ) ;
#14816=CARTESIAN_POINT ( 'NONE',  ( -18.34560609025200861, -9.386954687716539070, 53.49899999999994549 ) ) ;
#14818=CARTESIAN_POINT ( 'NONE',  ( -23.29871437377730814, -10.22635856038569990, 59.71548043103533843 ) ) ;
#14820=CARTESIAN_POINT ( 'NONE',  ( -20.03282965983824226, -21.84088468745754597, 47.99999999999994316 ) ) ;
#14821=CARTESIAN_POINT ( 'NONE',  ( -23.52949419687348964, -11.28347464189849525, 70.17738639980606763 ) ) ;
#14822=EDGE_CURVE ( 'NONE', #19035, #9708, #37762, .T. ) ;
#14824=CARTESIAN_POINT ( 'NONE',  ( -21.39310587431502242, -21.11392247816499435, 69.20450181858771543 ) ) ;
#14825=VERTEX_POINT ( 'NONE', #2197 ) ;
#14826=CARTESIAN_POINT ( 'NONE',  ( -11.88016137193916677, -19.16921147633432199, 71.57197012879584008 ) ) ;
#14827=DIRECTION ( 'NONE',  ( -0.5022914217388751990, 0.8646984027090225400, 6.766381827299041184E-08 ) ) ;
#14829=ADVANCED_FACE ( 'NONE', ( #29275 ), #28552, .T. ) ;
#14832=EDGE_CURVE ( 'NONE', #24815, #5348, #17331, .T. ) ;
#14835=ORIENTED_EDGE ( 'NONE', *, *, #45969, .F. ) ;
#14837=CARTESIAN_POINT ( 'NONE',  ( -16.22958052549516950, -7.455513305798441515, 60.45674424308347739 ) ) ;
#14839=ORIENTED_EDGE ( 'NONE', *, *, #32782, .F. ) ;
#14840=CARTESIAN_POINT ( 'NONE',  ( -22.53429319464571279, -9.952421322533329118, 73.48161091678163359 ) ) ;
#14842=ORIENTED_EDGE ( 'NONE', *, *, #34978, .T. ) ;
#14843=B_SPLINE_CURVE_WITH_KNOTS ( 'NONE', 3,
 ( #1773, #46353, #27866, #42665, #1274, #46103, #35493, #20238, #12363, #27384 ),
 .UNSPECIFIED., .F., .F.,
 ( 4, 2, 2, 2, 4 ),
 ( 0.000000000000000000, 0.2500000000000000000, 0.5000000000000000000, 0.7500000000000000000, 1.000000000000000000 ),
 .UNSPECIFIED. ) ;
#14844=CARTESIAN_POINT ( 'NONE',  ( -23.56138519289638822, -11.33989039198723070, 69.89210750373884196 ) ) ;
#14846=AXIS2_PLACEMENT_3D ( 'NONE', #19232, #34233, #15508 ) ;
#14847=CARTESIAN_POINT ( 'NONE',  ( -14.58623519113625200, -21.69754534531507772, 58.26594266842833036 ) ) ;
#14849=VERTEX_POINT ( 'NONE', #21163 ) ;
#14852=CARTESIAN_POINT ( 'NONE',  ( -11.47236213698566054, -10.32806074475630886, 74.55389686390628867 ) ) ;
#14855=CARTESIAN_POINT ( 'NONE',  ( -21.15825550006504940, -20.79330918033647535, 72.61626714470398269 ) ) ;
#14856=EDGE_LOOP ( 'NONE', ( #29972, #27815 ) ) ;
#14859=EDGE_CURVE ( 'NONE', #34680, #16467, #40931, .T. ) ;
#14861=CARTESIAN_POINT ( 'NONE',  ( -10.84048750645423098, -17.18764830010450595, 61.44277775138327513 ) ) ;
#14862=( BOUNDED_CURVE ( )  B_SPLINE_CURVE ( 3, ( #44632, #15050, #11376, #18506 ),
 .UNSPECIFIED., .F., .F. ) 
 B_SPLINE_CURVE_WITH_KNOTS ( ( 4, 4 ),
 ( 0.9074455897393705062, 1.000000000000000000 ),
 .UNSPECIFIED. ) 
 CURVE ( )  GEOMETRIC_REPRESENTATION_ITEM ( )  RATIONAL_B_SPLINE_CURVE ( ( 0.6983129098261057210, 0.7760317562607091935, 0.8765941196520072864, 1.000000000000000000 ) ) 
 REPRESENTATION_ITEM ( '' )  );
#14863=B_SPLINE_CURVE_WITH_KNOTS ( 'NONE', 1,
 ( #26696, #25960 ),
 .UNSPECIFIED., .F., .F.,
 ( 2, 2 ),
 ( 0.000000000000000000, 1.000000000000000000 ),
 .UNSPECIFIED. ) ;
#14865=VERTEX_POINT ( 'NONE', #36397 ) ;
#14866=CARTESIAN_POINT ( 'NONE',  ( -15.53265176333180619, -21.60105060138385369, 72.33103357390284316 ) ) ;
#14869=FACE_OUTER_BOUND ( 'NONE', #22913, .T. ) ;
#14871=( BOUNDED_CURVE ( )  B_SPLINE_CURVE ( 3, ( #26232, #15616, #15131, #30188 ),
 .UNSPECIFIED., .F., .F. ) 
 B_SPLINE_CURVE_WITH_KNOTS ( ( 4, 4 ),
 ( 0.5000000000000000000, 0.9074455897393693959 ),
 .UNSPECIFIED. ) 
 CURVE ( )  GEOMETRIC_REPRESENTATION_ITEM ( )  RATIONAL_B_SPLINE_CURVE ( ( 1.000000000000009992, 0.4567392136813236414, 0.3561768502900199418, 0.6983129098261101619 ) ) 
 REPRESENTATION_ITEM ( '' )  );
#14872=CARTESIAN_POINT ( 'NONE',  ( -23.00382247466728103, -19.03821840904449303, 62.42577227956508068 ) ) ;
#14873=( BOUNDED_CURVE ( )  B_SPLINE_CURVE ( 3, ( #32342, #20282, #35285, #31610 ),
 .UNSPECIFIED., .F., .F. ) 
 B_SPLINE_CURVE_WITH_KNOTS ( ( 4, 4 ),
 ( 0.9074455897393675086, 1.000000000000000000 ),
 .UNSPECIFIED. ) 
 CURVE ( )  GEOMETRIC_REPRESENTATION_ITEM ( )  RATIONAL_B_SPLINE_CURVE ( ( 0.6983129098261082746, 0.7760317562607114139, 0.8765941196520086187, 1.000000000000000000 ) ) 
 REPRESENTATION_ITEM ( '' )  );
#14876=FACE_OUTER_BOUND ( 'NONE', #23659, .T. ) ;
#14877=CYLINDRICAL_SURFACE ( 'NONE', #13164, 0.1500000000000028255 ) ;
#14878=CARTESIAN_POINT ( 'NONE',  ( -18.52415950777489684, -7.896185818571675341, 74.14064402152244782 ) ) ;
#14879=CARTESIAN_POINT ( 'NONE',  ( -21.53861794036900079, -21.02004141303368101, 72.63951040967180006 ) ) ;
#14880=B_SPLINE_CURVE_WITH_KNOTS ( 'NONE', 3,
 ( #19829, #4551, #8987, #19575, #15866, #38524, #16346, #31138, #16831, #46415 ),
 .UNSPECIFIED., .F., .F.,
 ( 4, 2, 2, 2, 4 ),
 ( 0.000000000000000000, 0.2500000000000000000, 0.5000000000000000000, 0.7500000000000000000, 1.000000000000000000 ),
 .UNSPECIFIED. ) ;
#14882=CARTESIAN_POINT ( 'NONE',  ( -10.42477179210370686, -17.36325313327283482, 61.27087820301521504 ) ) ;
#14883=AXIS2_PLACEMENT_3D ( 'NONE', #25118, #47033, #6158 ) ;
#14884=CARTESIAN_POINT ( 'NONE',  ( -24.21474372977315070, -11.74455924407879337, 59.64382217289720955 ) ) ;
#14885=CARTESIAN_POINT ( 'NONE',  ( -13.18904211892902367, -11.30002761096173280, 54.07175714974879099 ) ) ;
#14886=DIRECTION ( 'NONE',  ( 9.352133743349324758E-06, 6.779811746737758835E-06, 0.9999999999332858103 ) ) ;
#14887=ORIENTED_EDGE ( 'NONE', *, *, #25495, .T. ) ;
#14888=CARTESIAN_POINT ( 'NONE',  ( -10.54823608622644038, -17.67727527167151536, 68.20383655110275356 ) ) ;
#14889=CARTESIAN_POINT ( 'NONE',  ( -18.46649413407774887, -22.18667672369172550, 72.47166315949273496 ) ) ;
#14890=CARTESIAN_POINT ( 'NONE',  ( -18.66311988809301425, -7.868636481342422329, 70.65595886192740238 ) ) ;
#14891=( BOUNDED_SURFACE ( )  B_SPLINE_SURFACE ( 3, 1, ( 
 ( #9197, #39224 ),
 ( #13102, #36700 ),
 ( #25898, #44159 ),
 ( #29845, #40911 ),
 ( #14299, #10408 ),
 ( #33018, #48538 ),
 ( #25417, #29589 ) ),
 .UNSPECIFIED., .T., .F., .F. ) 
 B_SPLINE_SURFACE_WITH_KNOTS ( ( 4, 3, 4 ),
 ( 2, 2 ),
 ( 0.000000000000000000, 0.5000000000000000000, 1.000000000000000000 ),
 ( 0.000000000000000000, 1.000000000000000000 ),
 .UNSPECIFIED. ) 
 GEOMETRIC_REPRESENTATION_ITEM ( )  RATIONAL_B_SPLINE_SURFACE ( (
 ( 1.000000000000000000, 1.000000000000000000),
 ( 0.3333333333333335369, 0.3333333333333330373),
 ( 0.3333333333333335369, 0.3333333333333330373),
 ( 1.000000000000000000, 1.000000000000000000),
 ( 0.3333333333333333703, 0.3333333333333333703),
 ( 0.3333333333333333703, 0.3333333333333333703),
 ( 1.000000000000000000, 1.000000000000000000) ) ) 
 REPRESENTATION_ITEM ( '' )  SURFACE ( )  );
#14892=FACE_BOUND ( 'NONE', #13153, .T. ) ;
#14896=DIRECTION ( 'NONE',  ( -0.9729319276368276759, -0.2310918955413239773, 6.827553174175007530E-08 ) ) ;
#14897=CARTESIAN_POINT ( 'NONE',  ( -10.53619943228106948, -16.06595316453636713, 71.55823587554787935 ) ) ;
#14898=CARTESIAN_POINT ( 'NONE',  ( -24.41706613368967282, -14.49561630978402071, 62.90399773248653048 ) ) ;
#14900=ORIENTED_EDGE ( 'NONE', *, *, #28654, .T. ) ;
#14901=CARTESIAN_POINT ( 'NONE',  ( -10.44202778021669609, -14.30845378979165794, 64.68803863533310050 ) ) ;
#14902=EDGE_LOOP ( 'NONE', ( #43587, #20091, #20202, #19544, #11265 ) ) ;
#14903=FACE_OUTER_BOUND ( 'NONE', #47600, .T. ) ;
#14906=B_SPLINE_CURVE_WITH_KNOTS ( 'NONE', 1,
 ( #11105, #30563 ),
 .UNSPECIFIED., .F., .F.,
 ( 2, 2 ),
 ( 0.000000000000000000, 1.000000000000000000 ),
 .UNSPECIFIED. ) ;
#14908=CARTESIAN_POINT ( 'NONE',  ( -12.70616753690738143, -9.559812705026583757, 71.00492334522255078 ) ) ;
#14910=EDGE_CURVE ( 'NONE', #31125, #1137, #24261, .T. ) ;
#14912=ORIENTED_EDGE ( 'NONE', *, *, #15456, .F. ) ;
#14915=CARTESIAN_POINT ( 'NONE',  ( -15.53265176333180619, -21.60105060138385369, 72.33103357390284316 ) ) ;
#14917=CARTESIAN_POINT ( 'NONE',  ( -22.31677908589231762, -19.81551989533932101, 69.47417984703402283 ) ) ;
#14919=CARTESIAN_POINT ( 'NONE',  ( -12.56171917241870695, -20.45376946399996854, 71.99148991968543498 ) ) ;
#14920=DIRECTION ( 'NONE',  ( -5.731567514496413899E-31, -1.020425574103664789E-16, -1.000000000000000000 ) ) ;
#14921=CARTESIAN_POINT ( 'NONE',  ( -24.22725865585316285, -12.95987763975231388, 66.30246766143382331 ) ) ;
#14924=EDGE_LOOP ( 'NONE', ( #28318, #31214, #41611, #23702, #38977 ) ) ;
#14926=CARTESIAN_POINT ( 'NONE',  ( -16.30010877417799264, -7.443724743308521852, 60.38683862147721726 ) ) ;
#14927=EDGE_CURVE ( 'NONE', #2344, #40137, #19201, .T. ) ;
#14928=CARTESIAN_POINT ( 'NONE',  ( -13.92949766901237041, -8.229479445867253773, 74.33921261090144128 ) ) ;
#14929=CARTESIAN_POINT ( 'NONE',  ( -14.93209738089114857, -21.40413054883831734, 61.93600443765902241 ) ) ;
#14930=AXIS2_PLACEMENT_3D ( 'NONE', #16569, #42932, #46140 ) ;
#14935=CARTESIAN_POINT ( 'NONE',  ( -10.61946413101933295, -12.96527513164080148, 67.73832368323806463 ) ) ;
#14936=FACE_OUTER_BOUND ( 'NONE', #28589, .T. ) ;
#14938=CARTESIAN_POINT ( 'NONE',  ( -10.39215600595210454, -14.30487551902977650, 64.38803863383273551 ) ) ;
#14940=CARTESIAN_POINT ( 'NONE',  ( -22.51786048828498465, -9.935131201570847281, 73.78161090940139388 ) ) ;
#14941=B_SPLINE_CURVE_WITH_KNOTS ( 'NONE', 3,
 ( #32463, #11271, #26284, #48435, #14669, #6601, #40558, #18145, #11022, #40328 ),
 .UNSPECIFIED., .F., .F.,
 ( 4, 2, 2, 2, 4 ),
 ( 0.000000000000000000, 0.2500000000000000000, 0.5000000000000000000, 0.7500000000000000000, 1.000000000000000000 ),
 .UNSPECIFIED. ) ;
#14942=CARTESIAN_POINT ( 'NONE',  ( -10.47274630608271373, -15.98537029978553825, 67.98327651004974825 ) ) ;
#14943=FACE_OUTER_BOUND ( 'NONE', #21851, .T. ) ;
#14946=CARTESIAN_POINT ( 'NONE',  ( -10.40245588357037043, -14.17414831712846990, 61.20349182037644198 ) ) ;
#14947=CARTESIAN_POINT ( 'NONE',  ( -10.45859239952313224, -15.89938452881993847, 64.79299464097340433 ) ) ;
#14949=VERTEX_POINT ( 'NONE', #47269 ) ;
#14950=CARTESIAN_POINT ( 'NONE',  ( -20.72713954719890239, -8.131453259470875494, 63.46121511881940336 ) ) ;
#14952=ORIENTED_EDGE ( 'NONE', *, *, #25894, .T. ) ;
#14953=CARTESIAN_POINT ( 'NONE',  ( -24.47401588439614528, -14.84236418521736312, 59.54300237059217693 ) ) ;
#14954=CARTESIAN_POINT ( 'NONE',  ( -11.53125380103513109, -18.58817033051094825, 64.76323772856727601 ) ) ;
#14957=LINE ( 'NONE', #41326, #48619 ) ;
#14958=CARTESIAN_POINT ( 'NONE',  ( -23.34288396506439867, -19.33377296368179543, 59.06906041190286771 ) ) ;
#14959=ORIENTED_EDGE ( 'NONE', *, *, #17663, .T. ) ;
#14960=DIRECTION ( 'NONE',  ( -3.811252426750347363E-06, -6.838859004669815670E-06, -0.9999999999693520714 ) ) ;
#14961=AXIS2_PLACEMENT_3D ( 'NONE', #27247, #15908, #41542 ) ;
#14962=CARTESIAN_POINT ( 'NONE',  ( -10.90274299180159012, -17.35673364766031668, 68.32551725290736044 ) ) ;
#14964=CARTESIAN_POINT ( 'NONE',  ( -12.10369346210734243, -9.594120923840563364, 57.27430859790474926 ) ) ;
#14965=ADVANCED_FACE ( 'NONE', ( #24623 ), #45047, .T. ) ;
#14966=CARTESIAN_POINT ( 'NONE',  ( -21.80081500731019872, -8.780166552249799139, 70.27099206861544189 ) ) ;
#14969=EDGE_LOOP ( 'NONE', ( #457, #40292 ) ) ;
#14971=ADVANCED_FACE ( 'NONE', ( #45527 ), #41084, .T. ) ;
#14972=CARTESIAN_POINT ( 'NONE',  ( -23.35559249269254423, -10.30144050037046810, 59.80192198407322479 ) ) ;
#14974=LINE ( 'NONE', #37381, #2882 ) ;
#14976=( BOUNDED_CURVE ( )  B_SPLINE_CURVE ( 3, ( #8464, #37761, #41716, #16313 ),
 .UNSPECIFIED., .F., .F. ) 
 B_SPLINE_CURVE_WITH_KNOTS ( ( 4, 4 ),
 ( 4.712388980384690562, 4.921828490624009511 ),
 .UNSPECIFIED. ) 
 CURVE ( )  GEOMETRIC_REPRESENTATION_ITEM ( )  RATIONAL_B_SPLINE_CURVE ( ( 1.000000000000000000, 0.9963479302455156006, 0.9963479302455156006, 1.000000000000000000 ) ) 
 REPRESENTATION_ITEM ( '' )  );
#14979=CARTESIAN_POINT ( 'NONE',  ( -10.40218298486903592, -14.14017159955334435, 57.44824790076416576 ) ) ;
#14980=CARTESIAN_POINT ( 'NONE',  ( -12.40319033546273531, -19.76959921888892424, 68.48090162751329046 ) ) ;
#14981=CARTESIAN_POINT ( 'NONE',  ( -17.36767326789754406, -7.755820026086070129, 63.75877036558070898 ) ) ;
#14982=CARTESIAN_POINT ( 'NONE',  ( -13.54822921233619226, -20.69819393533649077, 61.51646323540209949 ) ) ;
#14985=B_SPLINE_CURVE_WITH_KNOTS ( 'NONE', 3,
 ( #12054, #38135, #22910, #45801, #30781, #731, #15724, #3, #11560, #4667 ),
 .UNSPECIFIED., .F., .F.,
 ( 4, 2, 2, 2, 4 ),
 ( 0.6272669072877804508, 0.7522669073072891788, 0.8772669073267977957, 1.002266907346306635, 1.127266907365815252 ),
 .UNSPECIFIED. ) ;
#14987=DIRECTION ( 'NONE',  ( 3.549360974554993999E-17, -6.371834667797928663E-18, -1.000000000000000000 ) ) ;
#14988=DIRECTION ( 'NONE',  ( -0.6538427738826437796, -0.7566304428460742804, 5.916677973164435741E-08 ) ) ;
#14989=AXIS2_PLACEMENT_3D ( 'NONE', #8553, #46220, #39312 ) ;
#14990=ORIENTED_EDGE ( 'NONE', *, *, #35650, .T. ) ;
#14991=ORIENTED_EDGE ( 'NONE', *, *, #32466, .T. ) ;
#14993=CARTESIAN_POINT ( 'NONE',  ( -10.64823551202976937, -13.04561788836951308, 71.39755745898455075 ) ) ;
#14994=CARTESIAN_POINT ( 'NONE',  ( -21.79028809537168243, -9.273590339475653366, 63.47681654923867711 ) ) ;
#14995=CARTESIAN_POINT ( 'NONE',  ( -10.45859239952313224, -15.89938452881993847, 64.79299464097340433 ) ) ;
#14998=B_SPLINE_CURVE_WITH_KNOTS ( 'NONE', 3,
 ( #46872, #47604, #9455, #17050, #32096, #31616, #36012, #39237, #2292, #9703 ),
 .UNSPECIFIED., .F., .F.,
 ( 4, 2, 2, 2, 4 ),
 ( 0.000000000000000000, 0.2500000000000000000, 0.5000000000000000000, 0.7500000000000000000, 1.000000000000000000 ),
 .UNSPECIFIED. ) ;
#14999=CARTESIAN_POINT ( 'NONE',  ( -24.47111443619382243, -12.39179416916012855, 73.41942463439355038 ) ) ;
#15000=CARTESIAN_POINT ( 'NONE',  ( -12.79725882921341373, -20.12850138265567068, 72.10653676770067477 ) ) ;
#15002=ORIENTED_EDGE ( 'NONE', *, *, #33942, .F. ) ;
#15005=CARTESIAN_POINT ( 'NONE',  ( -23.04367560227575140, -10.55211830211007218, 59.60203429193362012 ) ) ;
#15007=VERTEX_POINT ( 'NONE', #15203 ) ;
#15009=ORIENTED_EDGE ( 'NONE', *, *, #6688, .T. ) ;
#15010=CARTESIAN_POINT ( 'NONE',  ( -19.62622408449249178, -21.50961356628077326, 61.88014844347227950 ) ) ;
#15011=CARTESIAN_POINT ( 'NONE',  ( -11.14114413899577904, -10.80566798617789459, 57.32407932063995304 ) ) ;
#15012=ORIENTED_EDGE ( 'NONE', *, *, #19348, .T. ) ;
#15017=CARTESIAN_POINT ( 'NONE',  ( -10.35611353805053980, -12.45393147150008772, 61.05499485166044593 ) ) ;
#15018=( BOUNDED_CURVE ( )  B_SPLINE_CURVE ( 3, ( #35458, #21432, #9135, #43358 ),
 .UNSPECIFIED., .F., .F. ) 
 B_SPLINE_CURVE_WITH_KNOTS ( ( 4, 4 ),
 ( 0.000000000000000000, 0.4074455897393596260 ),
 .UNSPECIFIED. ) 
 CURVE ( )  GEOMETRIC_REPRESENTATION_ITEM ( )  RATIONAL_B_SPLINE_CURVE ( ( 1.000000000000000000, 0.4567392136813386294, 0.3561768502900327649, 0.6983129098260822953 ) ) 
 REPRESENTATION_ITEM ( '' )  );
#15019=CARTESIAN_POINT ( 'NONE',  ( -24.26499744607890818, -17.75976858747020160, 62.65856309191605789 ) ) ;
#15024=CARTESIAN_POINT ( 'NONE',  ( -19.09647057632575340, -21.60781438815542188, 58.75337332744499719 ) ) ;
#15025=CARTESIAN_POINT ( 'NONE',  ( -10.40687472791218049, -14.09964931664121579, 64.80292589203708076 ) ) ;
#15026=CARTESIAN_POINT ( 'NONE',  ( -23.34481426128875370, -18.63642081788812987, 69.29371984264746231 ) ) ;
#15028=CARTESIAN_POINT ( 'NONE',  ( -16.04563226305852908, -7.895241551553309201, 63.97010999323463665 ) ) ;
#15031=EDGE_CURVE ( 'NONE', #5311, #31006, #33931, .T. ) ;
#15032=CARTESIAN_POINT ( 'NONE',  ( -24.05923365589681140, -11.41972516488058176, 66.60869825954527812 ) ) ;
#15033=CARTESIAN_POINT ( 'NONE',  ( -10.50893933415051507, -13.43540278197273885, 74.96345540680638919 ) ) ;
#15034=ORIENTED_EDGE ( 'NONE', *, *, #29131, .F. ) ;
#15035=CARTESIAN_POINT ( 'NONE',  ( -17.79084007069931417, -7.768752218527305686, 60.38060768310333515 ) ) ;
#15037=CARTESIAN_POINT ( 'NONE',  ( -18.19389434033494268, -22.21941471489327569, 65.53027570717884487 ) ) ;
#15038=CARTESIAN_POINT ( 'NONE',  ( -12.47631366984485268, -9.857336861045936871, 57.38935527210361442 ) ) ;
#15039=EDGE_CURVE ( 'NONE', #8569, #35964, #30336, .T. ) ;
#15040=CARTESIAN_POINT ( 'NONE',  ( -10.45988366621089405, -15.51674690159928005, 57.58295249508964275 ) ) ;
#15042=CARTESIAN_POINT ( 'NONE',  ( -24.30048588269890431, -16.36411231998812710, 59.12332431758469653 ) ) ;
#15043=( BOUNDED_SURFACE ( )  B_SPLINE_SURFACE ( 3, 1, ( 
 ( #29308, #25605 ),
 ( #36917, #40870 ),
 ( #3442, #27074 ),
 ( #23880, #38142 ),
 ( #31497, #15975 ),
 ( #4926, #39117 ),
 ( #46282, #34938 ) ),
 .UNSPECIFIED., .T., .F., .F. ) 
 B_SPLINE_SURFACE_WITH_KNOTS ( ( 4, 3, 4 ),
 ( 2, 2 ),
 ( 0.000000000000000000, 0.5000000000000000000, 1.000000000000000000 ),
 ( 0.000000000000000000, 1.000000000000000000 ),
 .UNSPECIFIED. ) 
 GEOMETRIC_REPRESENTATION_ITEM ( )  RATIONAL_B_SPLINE_SURFACE ( (
 ( 1.000000000000000000, 1.000000000000000000),
 ( 0.3333333333333335369, 0.3333333333333330373),
 ( 0.3333333333333335369, 0.3333333333333330373),
 ( 1.000000000000000000, 1.000000000000000000),
 ( 0.3333333333333333703, 0.3333333333333333703),
 ( 0.3333333333333333703, 0.3333333333333333703),
 ( 1.000000000000000000, 1.000000000000000000) ) ) 
 REPRESENTATION_ITEM ( '' )  SURFACE ( )  );
#15044=CARTESIAN_POINT ( 'NONE',  ( -13.98060997152859741, -8.714678138767887106, 74.42628082040340587 ) ) ;
#15048=VERTEX_POINT ( 'NONE', #460 ) ;
#15050=CARTESIAN_POINT ( 'NONE',  ( -20.35133084405233816, -8.395599718752041696, 67.08104079005559583 ) ) ;
#15052=CARTESIAN_POINT ( 'NONE',  ( -15.65211700886707469, -8.035536993839519582, 74.19058801755400623 ) ) ;
#15055=EDGE_CURVE ( 'NONE', #43598, #9477, #34451, .T. ) ;
#15056=CARTESIAN_POINT ( 'NONE',  ( -11.83525646650322827, -10.59418119787233259, 74.43885130403194239 ) ) ;
#15057=CARTESIAN_POINT ( 'NONE',  ( -18.19389323530821301, -22.21941482433020809, 65.53027461949925225 ) ) ;
#15062=ORIENTED_EDGE ( 'NONE', *, *, #89, .T. ) ;
#15065=DIRECTION ( 'NONE',  ( -0.9789991564299000970, -0.2038642972899922245, 4.410747590293501912E-08 ) ) ;
#15067=CARTESIAN_POINT ( 'NONE',  ( -17.84575570470781258, -7.371070506658266908, 60.33706685437874739 ) ) ;
#15069=CARTESIAN_POINT ( 'NONE',  ( -13.59269417415731063, -21.19935819725622039, 65.09973481642835225 ) ) ;
#15071=CARTESIAN_POINT ( 'NONE',  ( -21.84079957929829874, -9.314189696129256291, 63.19153755727188582 ) ) ;
#15072=ORIENTED_EDGE ( 'NONE', *, *, #39126, .T. ) ;
#15074=ADVANCED_FACE ( 'NONE', ( #30012 ), #12599, .T. ) ;
#15075=CARTESIAN_POINT ( 'NONE',  ( -12.26463566984678621, -20.18368350662160182, 65.02708282775662951 ) ) ;
#15078=DIRECTION ( 'NONE',  ( -0.7489133456531320565, -0.6626679415081376812, 6.686399169904807862E-09 ) ) ;
#15079=CARTESIAN_POINT ( 'NONE',  ( -24.03361690119365335, -12.50376453790854647, 73.52760217071977422 ) ) ;
#15081=CARTESIAN_POINT ( 'NONE',  ( -19.78614017500849087, -21.39864787494504839, 68.93482476778672208 ) ) ;
#15082=B_SPLINE_CURVE_WITH_KNOTS ( 'NONE', 3,
 ( #42110, #38651, #8629, #42611, #23892, #26857, #4938, #45582, #34948, #991 ),
 .UNSPECIFIED., .F., .F.,
 ( 4, 2, 2, 2, 4 ),
 ( 0.000000000000000000, 0.2500000000000000000, 0.5000000000000000000, 0.7500000000000000000, 1.000000000000000000 ),
 .UNSPECIFIED. ) ;
#15083=DIRECTION ( 'NONE',  ( 0.9710973231077277834, -0.2386838684389877285, 7.431671637556432894E-08 ) ) ;
#15084=B_SPLINE_CURVE_WITH_KNOTS ( 'NONE', 3,
 ( #12968, #38599, #23345, #1407, #1660, #30981, #27760, #23840, #20380, #35138 ),
 .UNSPECIFIED., .F., .F.,
 ( 4, 2, 2, 2, 4 ),
 ( 0.6272669072877694596, 0.7522669073072851820, 0.8772669073268009043, 1.002266907346316627, 1.127266907365832349 ),
 .UNSPECIFIED. ) ;
#15085=CARTESIAN_POINT ( 'NONE',  ( -24.71334354870178274, -13.26952572216105075, 59.47772645308575790 ) ) ;
#15088=CARTESIAN_POINT ( 'NONE',  ( -24.37445139888341927, -16.03700657411734198, 59.27899288712937675 ) ) ;
#15090=EDGE_CURVE ( 'NONE', #33946, #7654, #39052, .T. ) ;
#15092=CARTESIAN_POINT ( 'NONE',  ( -18.44528782684011858, -21.78515541812411982, 72.29983070759432451 ) ) ;
#15093=CARTESIAN_POINT ( 'NONE',  ( -16.14646913593085742, -7.469405111292049426, 60.36061804874157843 ) ) ;
#15096=VERTEX_POINT ( 'NONE', #37119 ) ;
#15097=AXIS2_PLACEMENT_3D ( 'NONE', #39305, #2357, #42767 ) ;
#15098=CARTESIAN_POINT ( 'NONE',  ( -16.30010877417799264, -7.443724743308521852, 60.38683862147721726 ) ) ;
#15100=ORIENTED_EDGE ( 'NONE', *, *, #13877, .T. ) ;
#15101=CARTESIAN_POINT ( 'NONE',  ( -22.37985709289073455, -19.82347726015160205, 69.17417989525732480 ) ) ;
#15102=CARTESIAN_POINT ( 'NONE',  ( -22.49805064719525305, -9.986866608920609067, 73.48161091687566682 ) ) ;
#15103=DIRECTION ( 'NONE',  ( -0.9375570856950864451, 0.3478314405900309603, -3.549360974553817487E-17 ) ) ;
#15104=VERTEX_POINT ( 'NONE', #31700 ) ;
#15105=DIRECTION ( 'NONE',  ( 3.964551030465574775E-06, 2.747358549199493871E-07, -0.9999999999921034277 ) ) ;
#15106=EDGE_CURVE ( 'NONE', #4399, #956, #43288, .T. ) ;
#15108=B_SPLINE_CURVE_WITH_KNOTS ( 'NONE', 1,
 ( #46894, #31386 ),
 .UNSPECIFIED., .F., .F.,
 ( 2, 2 ),
 ( 0.000000000000000000, 1.000000000000000000 ),
 .UNSPECIFIED. ) ;
#15111=EDGE_CURVE ( 'NONE', #6268, #36141, #44398, .T. ) ;
#15113=CARTESIAN_POINT ( 'NONE',  ( -18.77307807160576303, -7.482301894102196371, 70.56342156955103917 ) ) ;
#15115=CARTESIAN_POINT ( 'NONE',  ( -13.62948724496060215, -8.926948417807865965, 57.26967755883410405 ) ) ;
#15119=B_SPLINE_CURVE_WITH_KNOTS ( 'NONE', 3,
 ( #40928, #24773, #43245, #14541, #9262, #40677, #5581, #7214, #29606, #44395 ),
 .UNSPECIFIED., .F., .F.,
 ( 4, 2, 2, 2, 4 ),
 ( 0.1272669073658040384, 0.2522669073462902034, 0.3772669073267763129, 0.5022669073072624224, 0.6272669072877485874 ),
 .UNSPECIFIED. ) ;
#15121=CARTESIAN_POINT ( 'NONE',  ( -16.19814190158817269, -21.75179548504963023, 58.43585572027992470 ) ) ;
#15124=EDGE_CURVE ( 'NONE', #46532, #12430, #6301, .T. ) ;
#15125=EDGE_CURVE ( 'NONE', #21906, #19358, #12023, .T. ) ;
#15127=CARTESIAN_POINT ( 'NONE',  ( -17.85728874018076340, -21.84618329174708151, 61.89007996730683203 ) ) ;
#15128=CARTESIAN_POINT ( 'NONE',  ( -18.83482760403246203, -7.952772484924772733, 67.18606370727887622 ) ) ;
#15129=CARTESIAN_POINT ( 'NONE',  ( -23.79305894267454491, -17.83234277001198365, 59.00378422961142633 ) ) ;
#15130=EDGE_LOOP ( 'NONE', ( #24092, #26357, #1617, #10322, #48047 ) ) ;
#15131=CARTESIAN_POINT ( 'NONE',  ( -12.20851000913748585, -19.55815686523975927, 61.69678616734186960 ) ) ;
#15132=VERTEX_POINT ( 'NONE', #43021 ) ;
#15133=CARTESIAN_POINT ( 'NONE',  ( -13.01482893870565682, -8.804038099563683772, 63.95300575187839343 ) ) ;
#15134=CARTESIAN_POINT ( 'NONE',  ( -24.83243314287557268, -14.02236757053316651, 73.32282709813433996 ) ) ;
#15136=FACE_OUTER_BOUND ( 'NONE', #25575, .T. ) ;
#15137=EDGE_LOOP ( 'NONE', ( #11099, #20509, #11537, #15807, #43294 ) ) ;
#15138=CARTESIAN_POINT ( 'NONE',  ( -18.05557233295238362, -22.23314744338585669, 61.98880637900742130 ) ) ;
#15140=CARTESIAN_POINT ( 'NONE',  ( -20.17268378225416825, -8.371407738384645469, 70.25100341248858626 ) ) ;
#15141=CARTESIAN_POINT ( 'NONE',  ( -24.31482341358216104, -13.31912415075585088, 59.51267924675325816 ) ) ;
#15142=EDGE_LOOP ( 'NONE', ( #26842, #25135, #4833, #21879, #33828 ) ) ;
#15143=CARTESIAN_POINT ( 'NONE',  ( -23.00441930688031889, -19.11762475274336737, 59.03410642058399560 ) ) ;
#15144=CYLINDRICAL_SURFACE ( 'NONE', #39187, 0.1499999999999954148 ) ;
#15145=CARTESIAN_POINT ( 'NONE',  ( -24.20371252810814866, -12.87440185077122834, 66.58774614429587757 ) ) ;
#15146=FACE_BOUND ( 'NONE', #46050, .T. ) ;
#15147=ORIENTED_EDGE ( 'NONE', *, *, #32228, .F. ) ;
#15150=EDGE_CURVE ( 'NONE', #2446, #13964, #15084, .T. ) ;
#15152=CARTESIAN_POINT ( 'NONE',  ( -13.08322001584757643, -9.253902105542977097, 67.67382971635112199 ) ) ;
#15153=CARTESIAN_POINT ( 'NONE',  ( -21.19428927390184114, -8.848463597801222491, 73.48639860482715847 ) ) ;
#15154=ORIENTED_EDGE ( 'NONE', *, *, #35430, .F. ) ;
#15157=CARTESIAN_POINT ( 'NONE',  ( -12.74071866071660075, -9.015263582886822391, 70.96429948631303830 ) ) ;
#15158=CARTESIAN_POINT ( 'NONE',  ( -17.15134141312287852, -7.364115244199362920, 70.67531166753866501 ) ) ;
#15161=CARTESIAN_POINT ( 'NONE',  ( -10.96962198434375146, -17.51872840680399790, 68.09721950251682188 ) ) ;
#15162=EDGE_CURVE ( 'NONE', #5861, #7442, #10413, .T. ) ;
#15163=ORIENTED_EDGE ( 'NONE', *, *, #22639, .F. ) ;
#15165=VERTEX_POINT ( 'NONE', #5120 ) ;
#15166=DIRECTION ( 'NONE',  ( -0.2737502900231349456, -0.9618007999124592589, 5.400150802763565238E-08 ) ) ;
#15167=CARTESIAN_POINT ( 'NONE',  ( -13.32832405134409548, -21.03232224849095289, 61.66646320379408053 ) ) ;
#15168=CARTESIAN_POINT ( 'NONE',  ( -12.84615363328625826, -20.17103110633857455, 72.09181604382622766 ) ) ;
#15169=CARTESIAN_POINT ( 'NONE',  ( -10.03795483766491969, -13.83545689752550345, 57.64163354902277803 ) ) ;
#15170=( BOUNDED_CURVE ( )  B_SPLINE_CURVE ( 3, ( #8968, #4527, #5516, #20039 ),
 .UNSPECIFIED., .F., .F. ) 
 B_SPLINE_CURVE_WITH_KNOTS ( ( 4, 4 ),
 ( 0.000000000000000000, 0.4074455897393726156 ),
 .UNSPECIFIED. ) 
 CURVE ( )  GEOMETRIC_REPRESENTATION_ITEM ( )  RATIONAL_B_SPLINE_CURVE ( ( 1.000000000000000000, 0.4567392136813217540, 0.3561768502900264921, 0.6983129098261142698 ) ) 
 REPRESENTATION_ITEM ( '' )  );
#15171=CARTESIAN_POINT ( 'NONE',  ( -10.37818533259200748, -17.22973363664382873, 61.27247698181179913 ) ) ;
#15173=CARTESIAN_POINT ( 'NONE',  ( -17.42409385541300892, -14.80920654474439502, 75.49999999999994316 ) ) ;
#15175=ORIENTED_EDGE ( 'NONE', *, *, #34889, .F. ) ;
#15176=CARTESIAN_POINT ( 'NONE',  ( -10.37394849890712401, -14.76283852923608286, 71.61310637325181006 ) ) ;
#15177=CARTESIAN_POINT ( 'NONE',  ( -13.92301192392296727, -8.232980258883593194, 74.37767385738736436 ) ) ;
#15178=DIRECTION ( 'NONE',  ( -0.9243256318339804212, 0.3816046728418208134, -8.614662759602032238E-09 ) ) ;
#15179=DIRECTION ( 'NONE',  ( -0.9926276493613469531, -0.06323820549165627691, 0.1033986416233890343 ) ) ;
#15182=( BOUNDED_CURVE ( )  B_SPLINE_CURVE ( 3, ( #23496, #35042, #45421, #1308 ),
 .UNSPECIFIED., .F., .F. ) 
 B_SPLINE_CURVE_WITH_KNOTS ( ( 4, 4 ),
 ( 0.9074455897393683967, 1.000000000000000000 ),
 .UNSPECIFIED. ) 
 CURVE ( )  GEOMETRIC_REPRESENTATION_ITEM ( )  RATIONAL_B_SPLINE_CURVE ( ( 0.6983129098260925094, 0.7760317562606977582, 0.8765941196520002920, 1.000000000000000000 ) ) 
 REPRESENTATION_ITEM ( '' )  );
#15183=EDGE_CURVE ( 'NONE', #22634, #47594, #672, .T. ) ;
#15186=ADVANCED_FACE ( 'NONE', ( #34662 ), #12031, .T. ) ;
#15187=CARTESIAN_POINT ( 'NONE',  ( -17.01596769717176372, -7.370308014455987156, 74.07522855441366971 ) ) ;
#15188=CARTESIAN_POINT ( 'NONE',  ( -12.31380156693488992, -10.02538874655004442, 60.85918086676540639 ) ) ;
#15189=AXIS2_PLACEMENT_3D ( 'NONE', #21589, #24135, #40300 ) ;
#15190=DIRECTION ( 'NONE',  ( 1.078386539787844256E-05, -7.293043934967424929E-06, 0.9999999999152597852 ) ) ;
#15192=CARTESIAN_POINT ( 'NONE',  ( -14.22441497990486958, -8.081217732231424478, 67.44470516081543110 ) ) ;
#15193=( BOUNDED_CURVE ( )  B_SPLINE_CURVE ( 3, ( #35974, #16537, #9419, #46609 ),
 .UNSPECIFIED., .F., .F. ) 
 B_SPLINE_CURVE_WITH_KNOTS ( ( 4, 4 ),
 ( 0.000000000000000000, 0.4074455897393700621 ),
 .UNSPECIFIED. ) 
 CURVE ( )  GEOMETRIC_REPRESENTATION_ITEM ( )  RATIONAL_B_SPLINE_CURVE ( ( 1.000000000000000000, 0.4567392136813238634, 0.3561768502900273248, 0.6983129098261103840 ) ) 
 REPRESENTATION_ITEM ( '' )  );
#15195=CARTESIAN_POINT ( 'NONE',  ( -10.90856645720024254, -17.50971350489534828, 64.51250748301919202 ) ) ;
#15196=ORIENTED_EDGE ( 'NONE', *, *, #17958, .T. ) ;
#15197=LINE ( 'NONE', #45275, #39904 ) ;
#15199=CARTESIAN_POINT ( 'NONE',  ( -10.51729421260818498, -16.22293138110306998, 71.44750383217574097 ) ) ;
#15200=ORIENTED_EDGE ( 'NONE', *, *, #37527, .T. ) ;
#15201=CARTESIAN_POINT ( 'NONE',  ( -24.68464418333330102, -16.47883131643914467, 59.31670754753076835 ) ) ;
#15202=VERTEX_POINT ( 'NONE', #14162 ) ;
#15203=CARTESIAN_POINT ( 'NONE',  ( -10.03904597514415009, -13.82694077737217242, 57.56329639008353638 ) ) ;
#15204=CARTESIAN_POINT ( 'NONE',  ( -24.75425692978680559, -16.14426119111164937, 62.70673273743753384 ) ) ;
#15205=ORIENTED_EDGE ( 'NONE', *, *, #23115, .F. ) ;
#15206=CARTESIAN_POINT ( 'NONE',  ( -22.26378936042422296, -19.94069658942875733, 62.23439075274148280 ) ) ;
#15207=CARTESIAN_POINT ( 'NONE',  ( -24.38143469521110518, -15.58083332675401067, 73.00303748421107741 ) ) ;
#15208=EDGE_CURVE ( 'NONE', #27480, #4575, #2547, .T. ) ;
#15209=CARTESIAN_POINT ( 'NONE',  ( -20.31063670516350328, -8.430306149294633400, 70.36173336096577202 ) ) ;
#15211=CARTESIAN_POINT ( 'NONE',  ( -21.42981021932851249, -20.54985930702059349, 72.75119662013757704 ) ) ;
#15213=DIRECTION ( 'NONE',  ( 0.9048399035850771543, 0.4257519804770706906, 1.330923649722295736E-08 ) ) ;
#15214=VERTEX_POINT ( 'NONE', #32430 ) ;
#15215=CARTESIAN_POINT ( 'NONE',  ( -19.24512995744831656, -8.048560962921746054, 63.62016385155983045 ) ) ;
#15216=CARTESIAN_POINT ( 'NONE',  ( -21.75074122386538988, -8.744327870424561056, 70.33121307893182461 ) ) ;
#15217=EDGE_CURVE ( 'NONE', #47695, #11292, #10454, .T. ) ;
#15219=ORIENTED_EDGE ( 'NONE', *, *, #26061, .F. ) ;
#15221=CARTESIAN_POINT ( 'NONE',  ( -10.48241187047983658, -15.71137557247682892, 61.32323669680387468 ) ) ;
#15222=CARTESIAN_POINT ( 'NONE',  ( -24.02518650215770890, -17.29497017970488315, 72.97516058001660610 ) ) ;
#15223=CARTESIAN_POINT ( 'NONE',  ( -22.92560359444879836, -19.23055950467793096, 62.49839992038752712 ) ) ;
#15224=CARTESIAN_POINT ( 'NONE',  ( -24.87556905619337755, -15.80954572138182712, 54.02312124697527906 ) ) ;
#15227=CARTESIAN_POINT ( 'NONE',  ( -11.64339224431418529, -10.10844562305556771, 71.15548443915361077 ) ) ;
#15228=DIRECTION ( 'NONE',  ( -0.03181436478788690625, -0.9994937949748078365, -6.982004198809110323E-09 ) ) ;
#15229=CARTESIAN_POINT ( 'NONE',  ( -12.12844827754892485, -10.15526124722410195, 64.32914323983619909 ) ) ;
#15230=ORIENTED_EDGE ( 'NONE', *, *, #23618, .T. ) ;
#15231=CARTESIAN_POINT ( 'NONE',  ( -27.79065715166790795, -17.71243352067323329, 54.61912878955446615 ) ) ;
#15235=EDGE_LOOP ( 'NONE', ( #6733, #35095 ) ) ;
#15236=ADVANCED_FACE ( 'NONE', ( #17628 ), #2136, .T. ) ;
#15239=CARTESIAN_POINT ( 'NONE',  ( -13.29208520756706235, -21.00847154833298802, 61.63929462826596506 ) ) ;
#15240=DIRECTION ( 'NONE',  ( -0.09077643883959131410, 0.9958712959773468043, 4.338678762321648664E-08 ) ) ;
#15241=EDGE_LOOP ( 'NONE', ( #14054, #23903 ) ) ;
#15242=CARTESIAN_POINT ( 'NONE',  ( -11.46028008028683942, -18.56947564720590194, 61.56238700194530367 ) ) ;
#15244=ADVANCED_FACE ( 'NONE', ( #44017 ), #27417, .T. ) ;
#15245=EDGE_CURVE ( 'NONE', #15772, #39638, #983, .T. ) ;
#15246=DIRECTION ( 'NONE',  ( 0.6827297667453423591, 0.7306709694519485376, 5.176517822219623819E-09 ) ) ;
#15247=ORIENTED_EDGE ( 'NONE', *, *, #4493, .F. ) ;
#15249=CARTESIAN_POINT ( 'NONE',  ( -22.48964968825576705, -9.905448439006629968, 73.76689030015370463 ) ) ;
#15250=CARTESIAN_POINT ( 'NONE',  ( -11.42587710518540334, -11.10406226247761019, 57.49431069621225276 ) ) ;
#15251=ADVANCED_FACE ( 'NONE', ( #9786 ), #39809, .T. ) ;
#15252=CARTESIAN_POINT ( 'NONE',  ( -10.42462062184586635, -14.89508117765250361, 75.09778901762284420 ) ) ;
#15253=VERTEX_POINT ( 'NONE', #14397 ) ;
#15254=CARTESIAN_POINT ( 'NONE',  ( -17.39761456938454742, -7.809256627251312644, 67.32039592144390383 ) ) ;
#15255=ORIENTED_EDGE ( 'NONE', *, *, #33934, .T. ) ;
#15256=B_SPLINE_CURVE_WITH_KNOTS ( 'NONE', 3,
 ( #44813, #29291, #14470, #29529, #17703, #40597, #25356, #14972, #7631, #40372 ),
 .UNSPECIFIED., .F., .F.,
 ( 4, 2, 2, 2, 4 ),
 ( 0.1272669073658270755, 0.2522669073488479907, 0.3772669073318688504, 0.5022669073148897656, 0.6272669072979106808 ),
 .UNSPECIFIED. ) ;
#15258=CARTESIAN_POINT ( 'NONE',  ( -11.49500183448703083, -10.99442376238782337, 57.22375354680192316 ) ) ;
#15259=EDGE_LOOP ( 'NONE', ( #13736, #40887, #34731, #23681, #7485 ) ) ;
#15260=CARTESIAN_POINT ( 'NONE',  ( -11.55897615675186785, -7.397247749063358135, 53.49999999999995026 ) ) ;
#15261=EDGE_CURVE ( 'NONE', #12832, #38958, #3102, .T. ) ;
#15263=LINE ( 'NONE', #22942, #35423 ) ;
#15265=CARTESIAN_POINT ( 'NONE',  ( -12.08107559391734220, -20.00099389537635020, 61.54678633777153607 ) ) ;
#15266=CARTESIAN_POINT ( 'NONE',  ( -22.27817919856018136, -9.157513542003881568, 59.83675792137641736 ) ) ;
#15268=ORIENTED_EDGE ( 'NONE', *, *, #5816, .F. ) ;
#15271=CARTESIAN_POINT ( 'NONE',  ( -22.36648328953754827, -20.38374146207719662, 62.33415536511054711 ) ) ;
#15272=DIRECTION ( 'NONE',  ( -5.731567514496413899E-31, -1.020425574103664789E-16, -1.000000000000000000 ) ) ;
#15273=CARTESIAN_POINT ( 'NONE',  ( -23.76950082168947986, -18.71306838267522821, 72.94181022443689244 ) ) ;
#15274=ORIENTED_EDGE ( 'NONE', *, *, #35855, .T. ) ;
#15275=ORIENTED_EDGE ( 'NONE', *, *, #27467, .T. ) ;
#15276=CARTESIAN_POINT ( 'NONE',  ( -23.81302322525746362, -11.80978145726242978, 66.56647414731462220 ) ) ;
#15277=CARTESIAN_POINT ( 'NONE',  ( -11.89178903705324863, -10.43929771899554737, 71.26893105542536944 ) ) ;
#15278=ORIENTED_EDGE ( 'NONE', *, *, #33153, .T. ) ;
#15279=CARTESIAN_POINT ( 'NONE',  ( -24.11881394502254849, -17.01995806294775448, 73.16863963025599560 ) ) ;
#15280=CARTESIAN_POINT ( 'NONE',  ( -16.38254737672540884, -22.18621074043892349, 61.91601456499802225 ) ) ;
#15281=CARTESIAN_POINT ( 'NONE',  ( -12.54283200749232918, -9.790123543357045932, 57.16105715312289703 ) ) ;
#15283=CARTESIAN_POINT ( 'NONE',  ( -18.15014757327930539, -21.82545121811569189, 61.87535875776518424 ) ) ;
#15284=CARTESIAN_POINT ( 'NONE',  ( -19.58369474063720261, -21.93945548790455291, 62.11690869439961205 ) ) ;
#15289=CARTESIAN_POINT ( 'NONE',  ( -24.86610167639389246, -14.46236660854407674, 66.29797298380238146 ) ) ;
#15290=CARTESIAN_POINT ( 'NONE',  ( -11.57079330372311787, -10.20035596359355878, 71.16881880436550034 ) ) ;
#15292=CARTESIAN_POINT ( 'NONE',  ( -24.25486363958986757, -13.06355980472538469, 63.11792038370487035 ) ) ;
#15294=CARTESIAN_POINT ( 'NONE',  ( -23.56879427660422266, -11.34691063241640130, 73.77682139093690239 ) ) ;
#15295=EDGE_LOOP ( 'NONE', ( #27275, #26854, #40771, #10255, #8753 ) ) ;
#15296=ORIENTED_EDGE ( 'NONE', *, *, #26943, .F. ) ;
#15298=ORIENTED_EDGE ( 'NONE', *, *, #2607, .T. ) ;
#15299=ADVANCED_FACE ( 'NONE', ( #4105, #22818, #18861, #18598, #3591, #23057, #44989, #7312, #11236, #41510, #33362, #33610, #26747, #29954, #19104, #48652, #37810, #44489, #14638, #26249, #40777, #25756, #34111, #10991, #41263, #15384, #48406, #41766, #44737, #30448, #33128, #14892, #33869, #7550, #37551, #18110, #45227, #26012, #3856, #7059, #22072, #45462, #170, #37069, #22312, #37304, #15146, #30206, #11471, #48166, #26494, #8052, #7803, #402, #29457, #10739, #4822, #38539, #9246, #31156, #27225, #27463, #45943, #34350, #31401, #42004, #9005, #12686, #19341, #23543, #34845, #1114, #35334, #20076, #1604, #19845, #42496, #8277, #16112 ), #884, .T. ) ;
#15302=CARTESIAN_POINT ( 'NONE',  ( -13.35550429318260512, -8.568184490765622385, 57.15463139269148485 ) ) ;
#15303=CARTESIAN_POINT ( 'NONE',  ( -16.98831825750070479, -22.24652902502744922, 72.20897298418123000 ) ) ;
#15304=EDGE_LOOP ( 'NONE', ( #24283, #1508, #29867, #28393, #40789 ) ) ;
#15305=EDGE_CURVE ( 'NONE', #10765, #9098, #47978, .T. ) ;
#15307=CARTESIAN_POINT ( 'NONE',  ( -14.81535805098777736, -7.777528402031247623, 47.99999999999994316 ) ) ;
#15308=EDGE_CURVE ( 'NONE', #3400, #4198, #36787, .T. ) ;
#15309=ORIENTED_EDGE ( 'NONE', *, *, #29970, .T. ) ;
#15310=( BOUNDED_SURFACE ( )  B_SPLINE_SURFACE ( 3, 1, ( 
 ( #21382, #43786 ),
 ( #10762, #33154 ),
 ( #21848, #40086 ),
 ( #36370, #36843 ),
 ( #48430, #2650 ),
 ( #48190, #7085 ),
 ( #3130, #32686 ) ),
 .UNSPECIFIED., .T., .F., .F. ) 
 B_SPLINE_SURFACE_WITH_KNOTS ( ( 4, 3, 4 ),
 ( 2, 2 ),
 ( 0.000000000000000000, 0.5000000000000000000, 1.000000000000000000 ),
 ( 0.000000000000000000, 1.000000000000000000 ),
 .UNSPECIFIED. ) 
 GEOMETRIC_REPRESENTATION_ITEM ( )  RATIONAL_B_SPLINE_SURFACE ( (
 ( 1.000000000000000000, 1.000000000000000000),
 ( 0.3333333333333335369, 0.3333333333333330373),
 ( 0.3333333333333335369, 0.3333333333333330373),
 ( 1.000000000000000000, 1.000000000000000000),
 ( 0.3333333333333333703, 0.3333333333333333703),
 ( 0.3333333333333333703, 0.3333333333333333703),
 ( 1.000000000000000000, 1.000000000000000000) ) ) 
 REPRESENTATION_ITEM ( '' )  SURFACE ( )  );
#15312=CARTESIAN_POINT ( 'NONE',  ( -23.95744587143639492, -17.32345433839075710, 69.42956382067292509 ) ) ;
#15313=AXIS2_PLACEMENT_3D ( 'NONE', #38808, #35101, #42025 ) ;
#15315=ADVANCED_FACE ( 'NONE', ( #23786 ), #27707, .T. ) ;
#15317=CARTESIAN_POINT ( 'NONE',  ( -11.07356115161467436, -11.86355474871830573, 74.57456719742380358 ) ) ;
#15319=ORIENTED_EDGE ( 'NONE', *, *, #14401, .T. ) ;
#15320=CARTESIAN_POINT ( 'NONE',  ( -10.92333774552318104, -11.17005719542045483, 64.34220356397069907 ) ) ;
#15322=DIRECTION ( 'NONE',  ( -0.9811758422909350186, -0.1931164583992469319, -7.863147538403236401E-08 ) ) ;
#15324=CARTESIAN_POINT ( 'NONE',  ( -18.37786432726835883, -21.79469297182707521, 69.10042588711679912 ) ) ;
#15325=CARTESIAN_POINT ( 'NONE',  ( -24.49584582974870628, -12.46528025919705485, 73.49871492906470394 ) ) ;
#15326=ORIENTED_EDGE ( 'NONE', *, *, #42888, .T. ) ;
#15327=CARTESIAN_POINT ( 'NONE',  ( -24.71393967724174345, -16.34927462137609311, 59.23677039840046632 ) ) ;
#15328=CYLINDRICAL_SURFACE ( 'NONE', #23500, 0.1499999999999953315 ) ;
#15330=( BOUNDED_CURVE ( )  B_SPLINE_CURVE ( 3, ( #158, #37798, #23284, #38037 ),
 .UNSPECIFIED., .F., .F. ) 
 B_SPLINE_CURVE_WITH_KNOTS ( ( 4, 4 ),
 ( 1.570796326794896780, 1.780235837034217505 ),
 .UNSPECIFIED. ) 
 CURVE ( )  GEOMETRIC_REPRESENTATION_ITEM ( )  RATIONAL_B_SPLINE_CURVE ( ( 1.000000000000000000, 0.9963479302455154896, 0.9963479302455154896, 1.000000000000000000 ) ) 
 REPRESENTATION_ITEM ( '' )  );
#15331=CARTESIAN_POINT ( 'NONE',  ( -23.73810165963432084, -18.76483127932742789, 69.40716580542252245 ) ) ;
#15332=CARTESIAN_POINT ( 'NONE',  ( -20.93445280450092127, -20.86546091266223968, 62.18759423706340073 ) ) ;
#15335=ORIENTED_EDGE ( 'NONE', *, *, #24615, .T. ) ;
#15336=CARTESIAN_POINT ( 'NONE',  ( -24.31944129331298399, -13.32629719641017729, 63.24753052856355140 ) ) ;
#15337=CARTESIAN_POINT ( 'NONE',  ( -14.29947512317492730, -8.480563224953527879, 63.94546151666516209 ) ) ;
#15338=ORIENTED_EDGE ( 'NONE', *, *, #48321, .T. ) ;
#15341=CARTESIAN_POINT ( 'NONE',  ( -10.72017361938626934, -12.61779402817458973, 57.21368711609748203 ) ) ;
#15342=B_SPLINE_CURVE_WITH_KNOTS ( 'NONE', 3,
 ( #47359, #43908, #39225, #38980, #5255, #46629, #20275, #35279, #28632, #1554 ),
 .UNSPECIFIED., .F., .F.,
 ( 4, 2, 2, 2, 4 ),
 ( 0.1272669073658351802, 0.2522669073463199574, 0.3772669073268047901, 0.5022669073072896229, 0.6272669072877743446 ),
 .UNSPECIFIED. ) ;
#15343=VERTEX_POINT ( 'NONE', #42738 ) ;
#15344=CARTESIAN_POINT ( 'NONE',  ( -10.37497030826117417, -14.69804335084345581, 71.32782692816427073 ) ) ;
#15349=CARTESIAN_POINT ( 'NONE',  ( -23.80338573481879294, -11.80731802715296119, 59.76763678108634537 ) ) ;
#15352=CARTESIAN_POINT ( 'NONE',  ( -15.48396703021662546, -7.615489166865526904, 70.72334449499163611 ) ) ;
#15353=CARTESIAN_POINT ( 'NONE',  ( -21.29196722032537537, -20.70380199363842877, 72.53918572867779346 ) ) ;
#15354=ORIENTED_EDGE ( 'NONE', *, *, #14743, .T. ) ;
#15355=EDGE_LOOP ( 'NONE', ( #9598, #25280 ) ) ;
#15358=CARTESIAN_POINT ( 'NONE',  ( -20.00308622248979162, -8.244632374337111713, 70.13611736960565679 ) ) ;
#15361=CARTESIAN_POINT ( 'NONE',  ( -10.23569597183452728, -12.85201410577908732, 67.99478283741052564 ) ) ;
#15363=CARTESIAN_POINT ( 'NONE',  ( -18.28326045751188289, -21.81039776412065834, 72.58511189374844719 ) ) ;
#15365=EDGE_LOOP ( 'NONE', ( #24927, #16096, #35126, #19587, #17772 ) ) ;
#15366=CARTESIAN_POINT ( 'NONE',  ( -22.99430652176234702, -19.05128528775244234, 62.54334036401282049 ) ) ;
#15368=EDGE_CURVE ( 'NONE', #4639, #12198, #29282, .T. ) ;
#15370=CARTESIAN_POINT ( 'NONE',  ( -15.70730708645226237, -24.91091750872855215, 53.49999999999995026 ) ) ;
#15371=CARTESIAN_POINT ( 'NONE',  ( -24.41897151118743636, -17.37347349776957017, 69.59835227440868266 ) ) ;
#15372=CARTESIAN_POINT ( 'NONE',  ( -10.42546210075913748, -12.25520342886974845, 57.44361899967025664 ) ) ;
#15373=ORIENTED_EDGE ( 'NONE', *, *, #46653, .F. ) ;
#15375=LINE ( 'NONE', #34104, #13966 ) ;
#15376=EDGE_CURVE ( 'NONE', #2848, #13213, #32453, .T. ) ;
#15377=CARTESIAN_POINT ( 'NONE',  ( -19.36122378369438835, -7.615284416629393149, 60.09946467050916397 ) ) ;
#15378=CARTESIAN_POINT ( 'NONE',  ( -23.99312268326606201, -11.29471679256767125, 66.60709928216182618 ) ) ;
#15380=DIRECTION ( 'NONE',  ( -5.215802026392426595E-06, 6.671378403414619972E-06, 0.9999999999641440152 ) ) ;
#15381=CYLINDRICAL_SURFACE ( 'NONE', #36019, 0.1500000000000066835 ) ;
#15382=FACE_OUTER_BOUND ( 'NONE', #14969, .T. ) ;
#15384=FACE_BOUND ( 'NONE', #16372, .T. ) ;
#15386=ORIENTED_EDGE ( 'NONE', *, *, #18933, .F. ) ;
#15387=DIRECTION ( 'NONE',  ( 2.842893050599252319E-07, -1.090087279701840163E-07, 0.9999999999999535927 ) ) ;
#15388=CARTESIAN_POINT ( 'NONE',  ( -14.60689764421331738, -8.346551857622415582, 63.78978840692987262 ) ) ;
#15389=CARTESIAN_POINT ( 'NONE',  ( -16.00544582274271477, -7.903112417841744453, 63.95538887075813506 ) ) ;
#15390=ORIENTED_EDGE ( 'NONE', *, *, #37535, .F. ) ;
#15391=CARTESIAN_POINT ( 'NONE',  ( -10.44483711275296933, -14.26928301035353819, 64.38803882970550774 ) ) ;
#15392=VERTEX_POINT ( 'NONE', #46432 ) ;
#15393=CARTESIAN_POINT ( 'NONE',  ( -12.27038830856583296, -10.07030047048361077, 64.25744141247331243 ) ) ;
#15398=ADVANCED_FACE ( 'NONE', ( #8509 ), #4336, .T. ) ;
#15401=ADVANCED_FACE ( 'NONE', ( #32135 ), #30599, .T. ) ;
#15403=ORIENTED_EDGE ( 'NONE', *, *, #39745, .T. ) ;
#15404=CARTESIAN_POINT ( 'NONE',  ( -20.25191534917340874, -8.350868906188830820, 70.26572394742477456 ) ) ;
#15405=CARTESIAN_POINT ( 'NONE',  ( -22.80983080810246832, -13.62945529097500419, 53.69233794759167466 ) ) ;
#15406=CARTESIAN_POINT ( 'NONE',  ( -12.56171917241870695, -20.45376946399996854, 71.99148991968543498 ) ) ;
#15407=CARTESIAN_POINT ( 'NONE',  ( -20.60788153932096023, -8.518722016582884748, 63.32593600985608617 ) ) ;
#15409=CARTESIAN_POINT ( 'NONE',  ( -12.69763806180496601, -20.04058448603118592, 68.62185382311069759 ) ) ;
#15410=CARTESIAN_POINT ( 'NONE',  ( -12.50776634899986384, -20.40684016789016297, 71.92158251742569064 ) ) ;
#15411=ORIENTED_EDGE ( 'NONE', *, *, #19637, .T. ) ;
#15413=FACE_OUTER_BOUND ( 'NONE', #31091, .T. ) ;
#15414=B_SPLINE_CURVE_WITH_KNOTS ( 'NONE', 3,
 ( #22989, #33791, #44656, #7723, #18528, #88, #19031, #26670, #37975, #26184 ),
 .UNSPECIFIED., .F., .F.,
 ( 4, 2, 2, 2, 4 ),
 ( 0.1272669073658270200, 0.2522669073463124079, 0.3772669073267977957, 0.5022669073072831836, 0.6272669072877685714 ),
 .UNSPECIFIED. ) ;
#15416=CARTESIAN_POINT ( 'NONE',  ( -10.50673370502780557, -15.88996622876637588, 68.04938193442052352 ) ) ;
#15417=CARTESIAN_POINT ( 'NONE',  ( -23.52687218415512760, -18.35477548540580273, 69.44938804596051796 ) ) ;
#15420=AXIS2_PLACEMENT_3D ( 'NONE', #6430, #32981, #36920 ) ;
#15421=AXIS2_PLACEMENT_3D ( 'NONE', #8314, #34641, #4866 ) ;
#15422=EDGE_LOOP ( 'NONE', ( #9169, #31107, #44228, #11254, #38803 ) ) ;
#15423=CARTESIAN_POINT ( 'NONE',  ( -11.71918404020638427, -18.95175453447548009, 71.70158022526054253 ) ) ;
#15425=FACE_OUTER_BOUND ( 'NONE', #5584, .T. ) ;
#15428=ADVANCED_FACE ( 'NONE', ( #20808 ), #6024, .F. ) ;
#15430=CARTESIAN_POINT ( 'NONE',  ( -13.01616685277437568, -9.306763517318225709, 70.86397465682092900 ) ) ;
#15431=ADVANCED_FACE ( 'NONE', ( #21047 ), #43223, .T. ) ;
#15432=ORIENTED_EDGE ( 'NONE', *, *, #6809, .F. ) ;
#15433=LINE ( 'NONE', #37358, #12380 ) ;
#15435=CARTESIAN_POINT ( 'NONE',  ( -23.98503169607928953, -17.39005800936845603, 66.22885190747201989 ) ) ;
#15436=ORIENTED_EDGE ( 'NONE', *, *, #2845, .F. ) ;
#15437=CARTESIAN_POINT ( 'NONE',  ( -12.25434508901797770, -20.17367074759813406, 65.05170324716399932 ) ) ;
#15440=CARTESIAN_POINT ( 'NONE',  ( -14.93181132608235195, -7.787654600965993268, 57.03655263075181381 ) ) ;
#15442=CARTESIAN_POINT ( 'NONE',  ( -13.06813783877040969, -9.265530354883374287, 67.66470656304637998 ) ) ;
#15443=CARTESIAN_POINT ( 'NONE',  ( -23.84087125894599168, -12.00869244310661266, 59.71065521759481953 ) ) ;
#15444=CARTESIAN_POINT ( 'NONE',  ( -10.57487349103886132, -17.90974545538605867, 53.76227901944324117 ) ) ;
#15445=ORIENTED_EDGE ( 'NONE', *, *, #4853, .T. ) ;
#15446=DIRECTION ( 'NONE',  ( -2.872222159185455981E-06, 2.507089443456002334E-06, 0.9999999999927324801 ) ) ;
#15447=( BOUNDED_CURVE ( )  B_SPLINE_CURVE ( 3, ( #39657, #35468, #35699, #27845 ),
 .UNSPECIFIED., .F., .F. ) 
 B_SPLINE_CURVE_WITH_KNOTS ( ( 4, 4 ),
 ( 0.5000000000000000000, 0.9074455897393628456 ),
 .UNSPECIFIED. ) 
 CURVE ( )  GEOMETRIC_REPRESENTATION_ITEM ( )  RATIONAL_B_SPLINE_CURVE ( ( 0.9999999999999765743, 0.4567392136813410164, 0.3561768502900499178, 0.6983129098260780765 ) ) 
 REPRESENTATION_ITEM ( '' )  );
#15448=CARTESIAN_POINT ( 'NONE',  ( -22.25907719862886935, -19.87120158787481117, 65.98956406266549379 ) ) ;
#15451=CARTESIAN_POINT ( 'NONE',  ( -23.83043768205027035, -11.86620487761972420, 59.63235732590894855 ) ) ;
#15452=ADVANCED_FACE ( 'NONE', ( #32612 ), #1851, .F. ) ;
#15455=CARTESIAN_POINT ( 'NONE',  ( -21.73229268148169879, -8.731123941674052702, 70.17486588183628271 ) ) ;
#15456=EDGE_CURVE ( 'NONE', #41019, #32914, #47834, .T. ) ;
#15457=EDGE_CURVE ( 'NONE', #36238, #38209, #9157, .T. ) ;
#15458=EDGE_CURVE ( 'NONE', #25120, #20357, #35600, .T. ) ;
#15461=CARTESIAN_POINT ( 'NONE',  ( -24.85185494555865660, -14.23383234075676640, 69.75301023497073061 ) ) ;
#15462=CARTESIAN_POINT ( 'NONE',  ( -24.02419424914158341, -17.29788473263632298, 73.18336065054975847 ) ) ;
#15463=CARTESIAN_POINT ( 'NONE',  ( -23.16117746674104438, -18.90708040007733359, 62.63934749780565880 ) ) ;
#15466=CARTESIAN_POINT ( 'NONE',  ( -12.45759248923961060, -19.74223015388843194, 61.68213320638649577 ) ) ;
#15467=CARTESIAN_POINT ( 'NONE',  ( -12.14795427363658575, -9.549397679475163159, 57.28273822603964049 ) ) ;
#15469=( BOUNDED_SURFACE ( )  B_SPLINE_SURFACE ( 3, 1, ( 
 ( #40604, #6889 ),
 ( #32739, #21902 ),
 ( #36905, #2701 ),
 ( #47299, #35945 ),
 ( #13533, #39653 ),
 ( #5924, #36185 ),
 ( #6410, #2471 ) ),
 .UNSPECIFIED., .T., .F., .F. ) 
 B_SPLINE_SURFACE_WITH_KNOTS ( ( 4, 3, 4 ),
 ( 2, 2 ),
 ( 0.000000000000000000, 0.5000000000000000000, 1.000000000000000000 ),
 ( 0.000000000000000000, 1.000000000000000000 ),
 .UNSPECIFIED. ) 
 GEOMETRIC_REPRESENTATION_ITEM ( )  RATIONAL_B_SPLINE_SURFACE ( (
 ( 1.000000000000000000, 1.000000000000000000),
 ( 0.3333333333333335369, 0.3333333333333330373),
 ( 0.3333333333333335369, 0.3333333333333330373),
 ( 1.000000000000000000, 1.000000000000000000),
 ( 0.3333333333333333703, 0.3333333333333333703),
 ( 0.3333333333333333703, 0.3333333333333333703),
 ( 1.000000000000000000, 1.000000000000000000) ) ) 
 REPRESENTATION_ITEM ( '' )  SURFACE ( )  );
#15470=FACE_OUTER_BOUND ( 'NONE', #12050, .T. ) ;
#15471=ORIENTED_EDGE ( 'NONE', *, *, #35779, .T. ) ;
#15472=B_SPLINE_CURVE_WITH_KNOTS ( 'NONE', 1,
 ( #48253, #39910 ),
 .UNSPECIFIED., .F., .F.,
 ( 2, 2 ),
 ( 0.000000000000000000, 1.000000000000000000 ),
 .UNSPECIFIED. ) ;
#15473=DIRECTION ( 'NONE',  ( 1.149299188226319421E-05, -1.849289876324834950E-06, 0.9999999999322456423 ) ) ;
#15474=CARTESIAN_POINT ( 'NONE',  ( -21.85546194014773391, -9.390365834825972868, 59.94844577305733679 ) ) ;
#15475=EDGE_LOOP ( 'NONE', ( #15963, #36303, #33127, #23703, #20995 ) ) ;
#15476=( BOUNDED_CURVE ( )  B_SPLINE_CURVE ( 3, ( #5559, #40001, #43219, #13635 ),
 .UNSPECIFIED., .F., .F. ) 
 B_SPLINE_CURVE_WITH_KNOTS ( ( 4, 4 ),
 ( 0.5000000000000000000, 0.9074455897393666204 ),
 .UNSPECIFIED. ) 
 CURVE ( )  GEOMETRIC_REPRESENTATION_ITEM ( )  RATIONAL_B_SPLINE_CURVE ( ( 0.9999999999999905631, 0.4567392136813254178, 0.3561768502900344302, 0.6983129098261073864 ) ) 
 REPRESENTATION_ITEM ( '' )  );
#15478=EDGE_CURVE ( 'NONE', #43051, #45493, #21472, .T. ) ;
#15479=CARTESIAN_POINT ( 'NONE',  ( -16.20683463515880973, -21.70255690700738782, 58.28585572422844052 ) ) ;
#15481=CARTESIAN_POINT ( 'NONE',  ( -22.06477193427564387, -8.981018767459000074, 63.23507824025425350 ) ) ;
#15482=CARTESIAN_POINT ( 'NONE',  ( -10.18577798186947625, -13.04535695669732220, 71.33111718294915704 ) ) ;
#15487=CARTESIAN_POINT ( 'NONE',  ( -13.46273918380367185, -8.972896482542827457, 64.20946814027203686 ) ) ;
#15488=ORIENTED_EDGE ( 'NONE', *, *, #7580, .T. ) ;
#15489=EDGE_CURVE ( 'NONE', #23907, #21434, #29161, .T. ) ;
#15490=AXIS2_PLACEMENT_3D ( 'NONE', #36032, #25451, #13620 ) ;
#15491=CARTESIAN_POINT ( 'NONE',  ( -20.19231683483797113, -8.325423577284544407, 70.55100341277886855 ) ) ;
#15492=B_SPLINE_CURVE_WITH_KNOTS ( 'NONE', 1,
 ( #22812, #3847 ),
 .UNSPECIFIED., .F., .F.,
 ( 2, 2 ),
 ( 0.000000000000000000, 1.000000000000000000 ),
 .UNSPECIFIED. ) ;
#15496=ORIENTED_EDGE ( 'NONE', *, *, #28302, .T. ) ;
#15497=CARTESIAN_POINT ( 'NONE',  ( -18.50932193227059486, -21.77517953109191140, 72.58510940649487964 ) ) ;
#15498=FACE_OUTER_BOUND ( 'NONE', #14703, .T. ) ;
#15499=ORIENTED_EDGE ( 'NONE', *, *, #40586, .T. ) ;
#15500=CARTESIAN_POINT ( 'NONE',  ( -13.41424841794075462, -8.530288970272771110, 57.22613703607469660 ) ) ;
#15501=CARTESIAN_POINT ( 'NONE',  ( -13.88293259567353743, -20.90532631576516565, 68.45625136994867432 ) ) ;
#15503=CARTESIAN_POINT ( 'NONE',  ( -17.72419722990865054, -21.80277058550420577, 58.40553378253839156 ) ) ;
#15504=CARTESIAN_POINT ( 'NONE',  ( -18.78584198798900928, -7.883846953673406155, 63.58656136513857149 ) ) ;
#15505=CARTESIAN_POINT ( 'NONE',  ( -22.40225758545279788, -19.80633875317364456, 65.91241718764763391 ) ) ;
#15506=ORIENTED_EDGE ( 'NONE', *, *, #8917, .T. ) ;
#15507=CARTESIAN_POINT ( 'NONE',  ( -15.26018413780878724, -21.51894302366104483, 68.57592926692872481 ) ) ;
#15508=DIRECTION ( 'NONE',  ( -0.3478314405900309603, -0.9375570856950864451, 0.000000000000000000 ) ) ;
#15509=DIRECTION ( 'NONE',  ( 5.854827030937197869E-31, 1.020425574103664912E-16, 1.000000000000000000 ) ) ;
#15511=DIRECTION ( 'NONE',  ( 3.549360974554993999E-17, -6.371834667797928663E-18, -1.000000000000000000 ) ) ;
#15512=EDGE_CURVE ( 'NONE', #5832, #32391, #4141, .T. ) ;
#15513=EDGE_CURVE ( 'NONE', #34444, #14112, #17612, .T. ) ;
#15518=CARTESIAN_POINT ( 'NONE',  ( -10.34868689528060060, -12.47656361335272734, 60.99864767591832049 ) ) ;
#15519=EDGE_LOOP ( 'NONE', ( #22686, #45541, #19870, #16047, #6446 ) ) ;
#15520=CARTESIAN_POINT ( 'NONE',  ( -12.81525634688827786, -20.14415600020443264, 72.10653672084445986 ) ) ;
#15521=CARTESIAN_POINT ( 'NONE',  ( -15.19548991633585011, -21.91815178685365595, 68.76088227238139439 ) ) ;
#15522=CARTESIAN_POINT ( 'NONE',  ( -10.26942273409980722, -12.73178763592770579, 64.40689592259661822 ) ) ;
#15523=CARTESIAN_POINT ( 'NONE',  ( -10.46600813091865412, -15.57464811048514619, 57.79466158264115450 ) ) ;
#15524=B_SPLINE_CURVE_WITH_KNOTS ( 'NONE', 3,
 ( #44507, #28522, #6827, #7081, #36839, #3126, #22094, #3370, #10043, #13710 ),
 .UNSPECIFIED., .F., .F.,
 ( 4, 2, 2, 2, 4 ),
 ( 0.6272669072878274132, 0.7522669073073278145, 0.8772669073268283269, 1.002266907346328839, 1.127266907365829240 ),
 .UNSPECIFIED. ) ;
#15525=CARTESIAN_POINT ( 'NONE',  ( -14.36817892824948650, -8.455618309860652104, 67.54503025475185041 ) ) ;
#15526=CARTESIAN_POINT ( 'NONE',  ( -19.59054600911842670, -21.93742321824504415, 62.13357111270039468 ) ) ;
#15527=AXIS2_PLACEMENT_3D ( 'NONE', #4250, #15543, #27617 ) ;
#15530=EDGE_CURVE ( 'NONE', #28527, #7211, #34303, .T. ) ;
#15531=EDGE_CURVE ( 'NONE', #32823, #17138, #25822, .T. ) ;
#15532=FACE_OUTER_BOUND ( 'NONE', #25507, .T. ) ;
#15534=ADVANCED_FACE ( 'NONE', ( #7745 ), #37750, .T. ) ;
#15537=CARTESIAN_POINT ( 'NONE',  ( -13.79232177786185432, -20.79486811282113123, 68.52795486457198137 ) ) ;
#15538=CARTESIAN_POINT ( 'NONE',  ( -19.92776479198160189, -21.39998277484045275, 72.41950795000725805 ) ) ;
#15539=FACE_OUTER_BOUND ( 'NONE', #9847, .T. ) ;
#15543=DIRECTION ( 'NONE',  ( 0.7107718805962432995, 0.7034225854731135374, 7.722840060723789693E-09 ) ) ;
#15544=VERTEX_POINT ( 'NONE', #15092 ) ;
#15545=EDGE_CURVE ( 'NONE', #29624, #8171, #48491, .T. ) ;
#15547=CARTESIAN_POINT ( 'NONE',  ( -10.38863864971416184, -14.24588297309210816, 57.60391932725825370 ) ) ;
#15548=CARTESIAN_POINT ( 'NONE',  ( -11.26665320750704602, -11.47952451810412455, 64.43416648033296212 ) ) ;
#15549=CARTESIAN_POINT ( 'NONE',  ( -10.40888601095206312, -14.10966482229656194, 61.21821293885882653 ) ) ;
#15550=ORIENTED_EDGE ( 'NONE', *, *, #3491, .F. ) ;
#15551=CARTESIAN_POINT ( 'NONE',  ( -16.01976337179375776, -7.492708285372152943, 63.77736896427055058 ) ) ;
#15552=AXIS2_PLACEMENT_3D ( 'NONE', #996, #33982, #11838 ) ;
#15553=CARTESIAN_POINT ( 'NONE',  ( -18.55557756536243375, -7.850556297346193979, 73.84064430960019365 ) ) ;
#15555=ORIENTED_EDGE ( 'NONE', *, *, #4313, .T. ) ;
#15556=CARTESIAN_POINT ( 'NONE',  ( -24.45577199812615632, -12.20047074031916168, 53.49999999999994316 ) ) ;
#15560=CARTESIAN_POINT ( 'NONE',  ( -23.24415167771102020, -18.79314401478295338, 62.23918030722157368 ) ) ;
#15561=CARTESIAN_POINT ( 'NONE',  ( -22.17715676677442715, -20.54607711729781983, 58.87168751005452805 ) ) ;
#15562=CARTESIAN_POINT ( 'NONE',  ( -24.04524516174978643, -12.53718734719852002, 73.24225551612813945 ) ) ;
#15563=ORIENTED_EDGE ( 'NONE', *, *, #873, .F. ) ;
#15564=DIRECTION ( 'NONE',  ( -2.584300828889512628E-08, -1.497441464807615962E-06, 0.9999999999988784527 ) ) ;
#15565=CARTESIAN_POINT ( 'NONE',  ( -11.67943375510494874, -18.89645239624664796, 68.50217487844219022 ) ) ;
#15568=CARTESIAN_POINT ( 'NONE',  ( -14.54969778468464270, -21.68242161614711705, 58.35956174891157389 ) ) ;
#15569=CARTESIAN_POINT ( 'NONE',  ( -24.17147434587301191, -12.75550446831573126, 73.65714286828524848 ) ) ;
#15570=ORIENTED_EDGE ( 'NONE', *, *, #20444, .T. ) ;
#15571=FACE_OUTER_BOUND ( 'NONE', #29875, .T. ) ;
#15575=CARTESIAN_POINT ( 'NONE',  ( -22.58588533274201282, -20.18224782263116523, 69.36073240021890740 ) ) ;
#15578=EDGE_LOOP ( 'NONE', ( #14179, #16781, #29208, #39346 ) ) ;
#15580=CARTESIAN_POINT ( 'NONE',  ( -24.26085839341466155, -16.31265863350449408, 59.42332382718851136 ) ) ;
#15581=ORIENTED_EDGE ( 'NONE', *, *, #9280, .F. ) ;
#15582=DIRECTION ( 'NONE',  ( -0.03181436478788691319, -0.9994937949748079475, -6.982004198809111150E-09 ) ) ;
#15585=CARTESIAN_POINT ( 'NONE',  ( -14.60831034098102066, -21.21965606200325993, 58.27690872140736644 ) ) ;
#15586=B_SPLINE_CURVE_WITH_KNOTS ( 'NONE', 1,
 ( #27992, #9057 ),
 .UNSPECIFIED., .F., .F.,
 ( 2, 2 ),
 ( 0.000000000000000000, 1.000000000000000000 ),
 .UNSPECIFIED. ) ;
#15587=VERTEX_POINT ( 'NONE', #7499 ) ;
#15588=CARTESIAN_POINT ( 'NONE',  ( -25.31403878743076774, -21.34684298153750603, 53.49999999999995026 ) ) ;
#15589=CARTESIAN_POINT ( 'NONE',  ( -16.79871736827016449, -7.783984993247369921, 73.84529564069914898 ) ) ;
#15590=EDGE_CURVE ( 'NONE', #1214, #12470, #37457, .T. ) ;
#15591=CARTESIAN_POINT ( 'NONE',  ( -10.66160605790631344, -13.00123564105898666, 68.03832347539896830 ) ) ;
#15594=ADVANCED_FACE ( 'NONE', ( #45172 ), #22668, .T. ) ;
#15596=EDGE_CURVE ( 'NONE', #1510, #14770, #8869, .T. ) ;
#15599=CARTESIAN_POINT ( 'NONE',  ( -24.80132792067086811, -15.84796731252138180, 69.73318694624859404 ) ) ;
#15600=CARTESIAN_POINT ( 'NONE',  ( -14.02608879878888182, -8.179082098857648475, 70.86811127254848941 ) ) ;
#15601=CARTESIAN_POINT ( 'NONE',  ( -23.08260857892799578, -18.93003297495478776, 62.35406880915004280 ) ) ;
#15605=EDGE_LOOP ( 'NONE', ( #46800, #33448 ) ) ;
#15607=CARTESIAN_POINT ( 'NONE',  ( -24.40329140489778936, -15.80613695201593671, 69.53307515782529435 ) ) ;
#15610=CARTESIAN_POINT ( 'NONE',  ( -16.19792114999740562, -7.866354181730329742, 60.48556343814865954 ) ) ;
#15611=( BOUNDED_SURFACE ( )  B_SPLINE_SURFACE ( 3, 1, ( 
 ( #24577, #47458 ),
 ( #28738, #47211 ),
 ( #39574, #13455 ),
 ( #31705, #46732 ),
 ( #9792, #5850 ),
 ( #21110, #35862 ),
 ( #17402, #10021 ) ),
 .UNSPECIFIED., .T., .F., .F. ) 
 B_SPLINE_SURFACE_WITH_KNOTS ( ( 4, 3, 4 ),
 ( 2, 2 ),
 ( 0.000000000000000000, 0.5000000000000000000, 1.000000000000000000 ),
 ( 0.000000000000000000, 1.000000000000000000 ),
 .UNSPECIFIED. ) 
 GEOMETRIC_REPRESENTATION_ITEM ( )  RATIONAL_B_SPLINE_SURFACE ( (
 ( 1.000000000000000000, 1.000000000000000000),
 ( 0.3333333333333335369, 0.3333333333333330373),
 ( 0.3333333333333335369, 0.3333333333333330373),
 ( 1.000000000000000000, 1.000000000000000000),
 ( 0.3333333333333333703, 0.3333333333333333703),
 ( 0.3333333333333333703, 0.3333333333333333703),
 ( 1.000000000000000000, 1.000000000000000000) ) ) 
 REPRESENTATION_ITEM ( '' )  SURFACE ( )  );
#15612=CARTESIAN_POINT ( 'NONE',  ( -17.77920954038207668, -22.25082405446125122, 58.59048702730397196 ) ) ;
#15613=CARTESIAN_POINT ( 'NONE',  ( -11.01408789448753822, -11.01258660117674104, 60.82885777859402054 ) ) ;
#15614=CARTESIAN_POINT ( 'NONE',  ( -13.54822921233619226, -20.69819393533649077, 61.51646323540209949 ) ) ;
#15615=VERTEX_POINT ( 'NONE', #23007 ) ;
#15616=CARTESIAN_POINT ( 'NONE',  ( -12.21065591164131092, -19.56036527704336692, 61.48858610352198184 ) ) ;
#15617=B_SPLINE_CURVE_WITH_KNOTS ( 'NONE', 3,
 ( #37507, #48603, #10467, #25963, #29170, #40982, #48123, #22026, #7265, #18554 ),
 .UNSPECIFIED., .F., .F.,
 ( 4, 2, 2, 2, 4 ),
 ( 0.1272669073658323213, 0.2522669073442346255, 0.3772669073226370129, 0.5022669073010392893, 0.6272669072794416767 ),
 .UNSPECIFIED. ) ;
#15618=( BOUNDED_SURFACE ( )  B_SPLINE_SURFACE ( 3, 1, ( 
 ( #26649, #48311 ),
 ( #14543, #3261 ),
 ( #41664, #7216 ),
 ( #29861, #37214 ),
 ( #33773, #26166 ),
 ( #18510, #7955 ),
 ( #3749, #7706 ) ),
 .UNSPECIFIED., .T., .F., .F. ) 
 B_SPLINE_SURFACE_WITH_KNOTS ( ( 4, 3, 4 ),
 ( 2, 2 ),
 ( 0.000000000000000000, 0.5000000000000000000, 1.000000000000000000 ),
 ( 0.000000000000000000, 1.000000000000000000 ),
 .UNSPECIFIED. ) 
 GEOMETRIC_REPRESENTATION_ITEM ( )  RATIONAL_B_SPLINE_SURFACE ( (
 ( 1.000000000000000000, 1.000000000000000000),
 ( 0.3333333333333335369, 0.3333333333333330373),
 ( 0.3333333333333335369, 0.3333333333333330373),
 ( 1.000000000000000000, 1.000000000000000000),
 ( 0.3333333333333333703, 0.3333333333333333703),
 ( 0.3333333333333333703, 0.3333333333333333703),
 ( 1.000000000000000000, 1.000000000000000000) ) ) 
 REPRESENTATION_ITEM ( '' )  SURFACE ( )  );
#15620=CARTESIAN_POINT ( 'NONE',  ( -12.52591642561268515, -9.195683996340104471, 74.50418400381258266 ) ) ;
#15621=CARTESIAN_POINT ( 'NONE',  ( -15.07292840516123000, -21.45564092615730090, 65.10596683003562646 ) ) ;
#15622=CARTESIAN_POINT ( 'NONE',  ( -24.42389991426342988, -17.36022673893785750, 69.55193308739468705 ) ) ;
#15623=CARTESIAN_POINT ( 'NONE',  ( -20.75354924259569245, -21.52967727414722887, 47.99999999999994316 ) ) ;
#15624=VERTEX_POINT ( 'NONE', #8947 ) ;
#15627=CARTESIAN_POINT ( 'NONE',  ( -19.85909577874797449, -21.37257635846961890, 72.46322212860958700 ) ) ;
#15629=ADVANCED_FACE ( 'NONE', ( #46370 ), #4763, .T. ) ;
#15631=CARTESIAN_POINT ( 'NONE',  ( -19.36518065869528726, -8.031383756764064685, 59.97565108339750850 ) ) ;
#15633=DIRECTION ( 'NONE',  ( -9.632611953450936153E-07, 3.816342149705755051E-07, 0.9999999999994632072 ) ) ;
#15635=AXIS2_PLACEMENT_3D ( 'NONE', #11139, #29360, #41409 ) ;
#15639=VERTEX_POINT ( 'NONE', #8222 ) ;
#15640=CARTESIAN_POINT ( 'NONE',  ( -24.74075724160099554, -16.21284971877490122, 62.77824058731629009 ) ) ;
#15643=CARTESIAN_POINT ( 'NONE',  ( -15.95707318215220205, -7.504986700048139170, 63.85506303619484214 ) ) ;
#15645=CARTESIAN_POINT ( 'NONE',  ( -10.58454466348024425, -16.55148359085594478, 71.60317204484042009 ) ) ;
#15647=ORIENTED_EDGE ( 'NONE', *, *, #18095, .T. ) ;
#15648=B_SPLINE_CURVE_WITH_KNOTS ( 'NONE', 1,
 ( #9110, #503 ),
 .UNSPECIFIED., .F., .F.,
 ( 2, 2 ),
 ( 0.000000000000000000, 1.000000000000000000 ),
 .UNSPECIFIED. ) ;
#15649=CARTESIAN_POINT ( 'NONE',  ( -20.53534356219854118, -19.36092059621579509, 53.88362224778186516 ) ) ;
#15650=CARTESIAN_POINT ( 'NONE',  ( -16.76012850172728719, -22.22957059519031020, 68.79537020757767607 ) ) ;
#15653=ORIENTED_EDGE ( 'NONE', *, *, #18291, .F. ) ;
#15654=EDGE_LOOP ( 'NONE', ( #22186, #4338 ) ) ;
#15655=VERTEX_POINT ( 'NONE', #38725 ) ;
#15658=CARTESIAN_POINT ( 'NONE',  ( -16.55451525393793233, -12.46531383050667863, 75.49999999999994316 ) ) ;
#15661=CARTESIAN_POINT ( 'NONE',  ( -24.15197288150306321, -12.87620330113281497, 66.58781343342795367 ) ) ;
#15662=CARTESIAN_POINT ( 'NONE',  ( -11.82099675438171005, -9.899106633794131582, 64.21409753874590365 ) ) ;
#15664=ORIENTED_EDGE ( 'NONE', *, *, #21495, .T. ) ;
#15666=EDGE_CURVE ( 'NONE', #21656, #19435, #42532, .T. ) ;
#15667=CARTESIAN_POINT ( 'NONE',  ( -24.43827367352892210, -15.52193379869737377, 73.28831629023289906 ) ) ;
#15668=DIRECTION ( 'NONE',  ( 0.3124635249310679930, 0.8422251632096489082, -0.4393441931380591692 ) ) ;
#15670=FACE_OUTER_BOUND ( 'NONE', #28595, .T. ) ;
#15671=DIRECTION ( 'NONE',  ( -0.5497669574358330369, 0.8353180786453389128, 7.898837271846008747E-08 ) ) ;
#15673=EDGE_CURVE ( 'NONE', #44868, #5874, #23482, .T. ) ;
#15675=EDGE_CURVE ( 'NONE', #38891, #12034, #47550, .T. ) ;
#15678=ORIENTED_EDGE ( 'NONE', *, *, #35148, .T. ) ;
#15680=CARTESIAN_POINT ( 'NONE',  ( -15.37172156182068328, -21.50163546728593289, 68.59095364069538903 ) ) ;
#15681=CARTESIAN_POINT ( 'NONE',  ( -10.02107422201081732, -13.96720754792729480, 57.56169656168945181 ) ) ;
#15682=VERTEX_POINT ( 'NONE', #34538 ) ;
#15684=CARTESIAN_POINT ( 'NONE',  ( -12.36756753426621813, -9.896138138887707214, 57.37463480816234096 ) ) ;
#15685=ORIENTED_EDGE ( 'NONE', *, *, #3819, .F. ) ;
#15686=CARTESIAN_POINT ( 'NONE',  ( -10.44902896174112428, -15.40082452545022562, 57.56792826000953056 ) ) ;
#15687=EDGE_CURVE ( 'NONE', #445, #41870, #39354, .T. ) ;
#15689=CARTESIAN_POINT ( 'NONE',  ( -12.36892846946874336, -20.28168252396862670, 68.43683184314359380 ) ) ;
#15690=EDGE_LOOP ( 'NONE', ( #2337, #42465 ) ) ;
#15691=DIRECTION ( 'NONE',  ( 2.191687980765842865E-06, -1.258878960415826265E-05, -0.9999999999183594168 ) ) ;
#15693=CARTESIAN_POINT ( 'NONE',  ( -10.57990114081760957, -13.11695186304741334, 71.22300718686659593 ) ) ;
#15694=CARTESIAN_POINT ( 'NONE',  ( -14.73368791995220839, -7.861157911666011522, 56.96344736924808672 ) ) ;
#15696=CARTESIAN_POINT ( 'NONE',  ( -10.83536383905390998, -17.31742040078651357, 64.62739380450889826 ) ) ;
#15697=DIRECTION ( 'NONE',  ( -0.9979768094191902028, -0.06357898915123888495, 6.487762650558939457E-18 ) ) ;
#15702=CARTESIAN_POINT ( 'NONE',  ( -16.30881325926348424, -7.898512564620374654, 60.50028524973911459 ) ) ;
#15703=CARTESIAN_POINT ( 'NONE',  ( -11.95563469220200581, -9.749529029264454749, 60.73635005636825923 ) ) ;
#15704=VERTEX_POINT ( 'NONE', #1290 ) ;
#15706=CARTESIAN_POINT ( 'NONE',  ( -12.36756753426621813, -9.896138138887707214, 57.37463480816234096 ) ) ;
#15708=DIRECTION ( 'NONE',  ( 0.3163880819683246859, 0.8528035521334704772, -0.4154812667942318627 ) ) ;
#15709=EDGE_LOOP ( 'NONE', ( #9949, #19828, #6053, #46026, #31143 ) ) ;
#15711=DIRECTION ( 'NONE',  ( 1.069388062422745569E-05, -2.778940570413862605E-06, -0.9999999999389592720 ) ) ;
#15712=CARTESIAN_POINT ( 'NONE',  ( -24.07704370891654122, -17.14264987453632827, 72.89808101046213551 ) ) ;
#15716=CARTESIAN_POINT ( 'NONE',  ( -20.13271805750754595, -8.299978134201072777, 70.53628287813307907 ) ) ;
#15717=CARTESIAN_POINT ( 'NONE',  ( -12.60227155074094441, -19.95281705956671559, 68.35129494334645983 ) ) ;
#15719=CARTESIAN_POINT ( 'NONE',  ( -9.974309423965010524, -14.87247496791766821, 74.90504757659225277 ) ) ;
#15720=EDGE_LOOP ( 'NONE', ( #17273, #2673 ) ) ;
#15722=CARTESIAN_POINT ( 'NONE',  ( -22.94192455449829993, -9.803488759991966006, 70.05532601532212311 ) ) ;
#15723=ADVANCED_FACE ( 'NONE', ( #579 ), #45889, .T. ) ;
#15724=CARTESIAN_POINT ( 'NONE',  ( -10.03292950473385403, -13.87467889623203554, 57.54801398733246742 ) ) ;
#15726=CARTESIAN_POINT ( 'NONE',  ( -24.38152189803567538, -12.22801735019761793, 54.27143602781901421 ) ) ;
#15728=VERTEX_POINT ( 'NONE', #27167 ) ;
#15730=DIRECTION ( 'NONE',  ( 0.9466432954593471116, 0.3222832157619555660, 8.771047036255756069E-09 ) ) ;
#15732=CARTESIAN_POINT ( 'NONE',  ( -15.39389095703113952, -21.97733419268598709, 72.23070866474378704 ) ) ;
#15733=CARTESIAN_POINT ( 'NONE',  ( -10.16748990304072464, -13.12235252378331651, 71.39323974795351546 ) ) ;
#15736=ORIENTED_EDGE ( 'NONE', *, *, #45298, .F. ) ;
#15738=ADVANCED_FACE ( 'NONE', ( #12381 ), #46122, .T. ) ;
#15739=CARTESIAN_POINT ( 'NONE',  ( -23.55638888376047646, -11.43265673080018097, 69.90827408357159811 ) ) ;
#15740=CARTESIAN_POINT ( 'NONE',  ( -23.08261055559088248, -18.93003034027461950, 62.65406880913197796 ) ) ;
#15741=EDGE_CURVE ( 'NONE', #11741, #41372, #9186, .T. ) ;
#15742=ADVANCED_FACE ( 'NONE', ( #28387, #9677 ), #17275, .T. ) ;
#15743=ORIENTED_EDGE ( 'NONE', *, *, #46058, .T. ) ;
#15746=( BOUNDED_CURVE ( )  B_SPLINE_CURVE ( 3, ( #40025, #32850, #39534, #46923 ),
 .UNSPECIFIED., .F., .F. ) 
 B_SPLINE_CURVE_WITH_KNOTS ( ( 4, 4 ),
 ( 0.000000000000000000, 0.4074455897393662873 ),
 .UNSPECIFIED. ) 
 CURVE ( )  GEOMETRIC_REPRESENTATION_ITEM ( )  RATIONAL_B_SPLINE_CURVE ( ( 1.000000000000000000, 0.4567392136813360759, 0.3561768502900318212, 0.6983129098260872913 ) ) 
 REPRESENTATION_ITEM ( '' )  );
#15747=VERTEX_POINT ( 'NONE', #35515 ) ;
#15748=CARTESIAN_POINT ( 'NONE',  ( -11.53247046633659245, -18.68106308600668441, 64.74707076449911369 ) ) ;
#15751=CARTESIAN_POINT ( 'NONE',  ( -11.42587710518540334, -11.10406226247761019, 57.49431069621225276 ) ) ;
#15752=ORIENTED_EDGE ( 'NONE', *, *, #17013, .F. ) ;
#15753=DIRECTION ( 'NONE',  ( 7.484513349675954647E-07, -7.898531916559714080E-07, -0.9999999999994080291 ) ) ;
#15754=CARTESIAN_POINT ( 'NONE',  ( -12.79725838692604434, -20.12850099319811292, 71.80653676770127447 ) ) ;
#15756=CARTESIAN_POINT ( 'NONE',  ( -24.47110706704248528, -14.59897147552597474, 63.00736729327273622 ) ) ;
#15759=EDGE_LOOP ( 'NONE', ( #654, #12577, #30085, #20652, #44126 ) ) ;
#15760=( BOUNDED_CURVE ( )  B_SPLINE_CURVE ( 3, ( #19425, #14981, #45071, #41851 ),
 .UNSPECIFIED., .F., .F. ) 
 B_SPLINE_CURVE_WITH_KNOTS ( ( 4, 4 ),
 ( 0.000000000000000000, 0.4074455897393688408 ),
 .UNSPECIFIED. ) 
 CURVE ( )  GEOMETRIC_REPRESENTATION_ITEM ( )  RATIONAL_B_SPLINE_CURVE ( ( 1.000000000000000000, 0.4567392136813259174, 0.3561768502900280464, 0.6983129098261063872 ) ) 
 REPRESENTATION_ITEM ( '' )  );
#15761=CARTESIAN_POINT ( 'NONE',  ( -10.44202778021669609, -14.30845378979165794, 64.68803863533310050 ) ) ;
#15763=DIRECTION ( 'NONE',  ( 0.8083598999316399247, 0.5886886037477750966, 6.671815825018553389E-08 ) ) ;
#15765=CARTESIAN_POINT ( 'NONE',  ( -12.90354087724769272, -8.887350501024684490, 67.49447389996370816 ) ) ;
#15766=EDGE_CURVE ( 'NONE', #35214, #22721, #8566, .T. ) ;
#15767=ORIENTED_EDGE ( 'NONE', *, *, #7866, .T. ) ;
#15770=CARTESIAN_POINT ( 'NONE',  ( -21.94242186726961208, -9.397052521110282441, 60.00699132926281010 ) ) ;
#15771=CARTESIAN_POINT ( 'NONE',  ( -24.33947722655236845, -16.19878214197559529, 66.15505208431230244 ) ) ;
#15772=VERTEX_POINT ( 'NONE', #47345 ) ;
#15773=CARTESIAN_POINT ( 'NONE',  ( -10.43298842381219238, -15.77843866184169208, 57.72359922229868801 ) ) ;
#15774=CARTESIAN_POINT ( 'NONE',  ( -15.12888584993918428, -21.89692032561032775, 68.83238837976321634 ) ) ;
#15777=CARTESIAN_POINT ( 'NONE',  ( -12.05128958966154329, -19.97034025487388931, 61.57491367064827159 ) ) ;
#15778=CARTESIAN_POINT ( 'NONE',  ( -19.50843993236927432, -21.96177808838975665, 62.11008241541560437 ) ) ;
#15779=VECTOR ( 'NONE', #33404, 1000.000000000000114 ) ;
#15780=CARTESIAN_POINT ( 'NONE',  ( -14.03172754404545053, -8.686077560366827655, 74.48489347840799724 ) ) ;
#15781=( BOUNDED_SURFACE ( )  B_SPLINE_SURFACE ( 3, 1, ( 
 ( #37529, #18840 ),
 ( #25736, #18575 ),
 ( #48631, #45205 ),
 ( #38763, #35062 ),
 ( #4800, #16343 ),
 ( #15863, #45693 ),
 ( #5044, #16095 ) ),
 .UNSPECIFIED., .T., .F., .F. ) 
 B_SPLINE_SURFACE_WITH_KNOTS ( ( 4, 3, 4 ),
 ( 2, 2 ),
 ( 0.000000000000000000, 0.5000000000000000000, 1.000000000000000000 ),
 ( 0.000000000000000000, 1.000000000000000000 ),
 .UNSPECIFIED. ) 
 GEOMETRIC_REPRESENTATION_ITEM ( )  RATIONAL_B_SPLINE_SURFACE ( (
 ( 1.000000000000000000, 1.000000000000000000),
 ( 0.3333333333333335369, 0.3333333333333330373),
 ( 0.3333333333333335369, 0.3333333333333330373),
 ( 1.000000000000000000, 1.000000000000000000),
 ( 0.3333333333333333703, 0.3333333333333333703),
 ( 0.3333333333333333703, 0.3333333333333333703),
 ( 1.000000000000000000, 1.000000000000000000) ) ) 
 REPRESENTATION_ITEM ( '' )  SURFACE ( )  );
#15785=CARTESIAN_POINT ( 'NONE',  ( -24.00901317767523935, -17.32824147414624960, 69.42811846502259243 ) ) ;
#15788=CARTESIAN_POINT ( 'NONE',  ( -14.89095676091066345, -21.33490639913799924, 61.93600435359637402 ) ) ;
#15790=VERTEX_POINT ( 'NONE', #13573 ) ;
#15791=CARTESIAN_POINT ( 'NONE',  ( -19.67573413203048460, -21.49838315979392789, 72.54911470401957274 ) ) ;
#15792=ORIENTED_EDGE ( 'NONE', *, *, #35991, .T. ) ;
#15793=CARTESIAN_POINT ( 'NONE',  ( -19.14088062437382831, -4.707495580760234333, 53.49999999999995026 ) ) ;
#15794=AXIS2_PLACEMENT_3D ( 'NONE', #41316, #2500, #45277 ) ;
#15795=CARTESIAN_POINT ( 'NONE',  ( -10.45740709548926262, -13.70915569549963031, 57.86313879094461754 ) ) ;
#15796=ORIENTED_EDGE ( 'NONE', *, *, #10452, .T. ) ;
#15797=CARTESIAN_POINT ( 'NONE',  ( -10.82471902208573766, -11.35211385731556710, 67.81202917830380272 ) ) ;
#15799=LINE ( 'NONE', #11391, #26100 ) ;
#15800=EDGE_CURVE ( 'NONE', #37303, #4227, #25260, .T. ) ;
#15803=ORIENTED_EDGE ( 'NONE', *, *, #24140, .T. ) ;
#15804=AXIS2_PLACEMENT_3D ( 'NONE', #16179, #38608, #15945 ) ;
#15805=CARTESIAN_POINT ( 'NONE',  ( -20.94465790601859467, -8.243431112063134947, 59.95629843672877257 ) ) ;
#15807=ORIENTED_EDGE ( 'NONE', *, *, #27015, .F. ) ;
#15810=CARTESIAN_POINT ( 'NONE',  ( -12.24819225201853001, -20.16768402423936024, 64.97336598306215194 ) ) ;
#15812=ADVANCED_FACE ( 'NONE', ( #27886 ), #31870, .T. ) ;
#15813=ADVANCED_FACE ( 'NONE', ( #32547 ), #28132, .T. ) ;
#15814=CARTESIAN_POINT ( 'NONE',  ( -23.46647660864419294, -19.16733412182131246, 62.39760931945144051 ) ) ;
#15815=CARTESIAN_POINT ( 'NONE',  ( -16.57921203443829583, -21.81142124131518756, 69.11049422539112186 ) ) ;
#15817=ORIENTED_EDGE ( 'NONE', *, *, #42149, .T. ) ;
#15818=CARTESIAN_POINT ( 'NONE',  ( -23.22746095445554815, -10.13763477365454868, 63.17162361582423813 ) ) ;
#15819=CARTESIAN_POINT ( 'NONE',  ( -17.72419709140651278, -21.80277058947482516, 58.70553378253836030 ) ) ;
#15824=CARTESIAN_POINT ( 'NONE',  ( -20.21425406316526363, -8.334789581166827332, 70.25100338998272775 ) ) ;
#15826=DIRECTION ( 'NONE',  ( -0.6973657521612035559, 0.7167154300785205656, -1.015100525525034718E-08 ) ) ;
#15827=CARTESIAN_POINT ( 'NONE',  ( -10.95381465013825206, -17.48043978162002077, 68.39721944380028162 ) ) ;
#15829=EDGE_CURVE ( 'NONE', #4057, #47942, #5086, .T. ) ;
#15832=CARTESIAN_POINT ( 'NONE',  ( -16.58751243259469277, -21.80939447449397051, 65.37564390318223673 ) ) ;
#15833=CARTESIAN_POINT ( 'NONE',  ( -10.47425561207849753, -17.49314520081206936, 64.81234810402725088 ) ) ;
#15835=B_SPLINE_CURVE_WITH_KNOTS ( 'NONE', 3,
 ( #32026, #34748, #27115, #16018, #8409, #28082, #31062, #5205, #24160, #39165 ),
 .UNSPECIFIED., .F., .F.,
 ( 4, 2, 2, 2, 4 ),
 ( 0.000000000000000000, 0.2500000000000000000, 0.5000000000000000000, 0.7500000000000000000, 1.000000000000000000 ),
 .UNSPECIFIED. ) ;
#15837=CARTESIAN_POINT ( 'NONE',  ( -23.88415222675040184, -17.63235122089636775, 62.47360984996718258 ) ) ;
#15838=CARTESIAN_POINT ( 'NONE',  ( -12.78427029111582236, -20.05066579198349075, 68.56330852931057507 ) ) ;
#15840=ORIENTED_EDGE ( 'NONE', *, *, #44706, .F. ) ;
#15841=CARTESIAN_POINT ( 'NONE',  ( -18.25923033419348940, -22.21300364388852344, 69.00170051292239748 ) ) ;
#15842=CARTESIAN_POINT ( 'NONE',  ( -10.41921500249975807, -15.63170790598816140, 64.92260423241262401 ) ) ;
#15844=CARTESIAN_POINT ( 'NONE',  ( -14.56205194875994735, -21.68753530842563748, 58.26643629975792038 ) ) ;
#15845=ORIENTED_EDGE ( 'NONE', *, *, #9691, .F. ) ;
#15848=CARTESIAN_POINT ( 'NONE',  ( -23.80338573481879294, -11.80731802715296119, 59.76763678108634537 ) ) ;
#15849=DIRECTION ( 'NONE',  ( 0.4182840851231336421, -0.9083162577718748576, 8.112345261759808545E-09 ) ) ;
#15851=CARTESIAN_POINT ( 'NONE',  ( -23.10700766261894046, -18.89652940832406358, 62.65406835416833786 ) ) ;
#15853=ORIENTED_EDGE ( 'NONE', *, *, #19543, .F. ) ;
#15855=CARTESIAN_POINT ( 'NONE',  ( -21.24554616535955631, -21.20453920045676810, 65.76949338751086316 ) ) ;
#15856=CARTESIAN_POINT ( 'NONE',  ( -23.37964394754908781, -11.13058451656118386, 73.37695695401920659 ) ) ;
#15858=CARTESIAN_POINT ( 'NONE',  ( -20.31413516131974717, -8.378470924821744603, 67.06632013881642251 ) ) ;
#15859=AXIS2_PLACEMENT_3D ( 'NONE', #43477, #24990, #5133 ) ;
#15862=CARTESIAN_POINT ( 'NONE',  ( -20.47364684392118050, -8.506973744139683546, 66.85274300213296783 ) ) ;
#15863=CARTESIAN_POINT ( 'NONE',  ( -14.25645962476006368, -8.507545769726087670, 74.61443249008125633 ) ) ;
#15864=CARTESIAN_POINT ( 'NONE',  ( -11.50273595086851763, -11.07590776185467263, 57.20903212540526539 ) ) ;
#15866=CARTESIAN_POINT ( 'NONE',  ( -21.19335628676919470, -20.70964401715573189, 72.63519632848037588 ) ) ;
#15870=ADVANCED_FACE ( 'NONE', ( #44147 ), #33007, .T. ) ;
#15874=CARTESIAN_POINT ( 'NONE',  ( -9.534148923395315833, -8.271570107951246698, 53.49999999999995026 ) ) ;
#15875=EDGE_CURVE ( 'NONE', #47624, #38508, #11640, .T. ) ;
#15877=VERTEX_POINT ( 'NONE', #40651 ) ;
#15878=CARTESIAN_POINT ( 'NONE',  ( -10.83008762082782006, -12.29245259246931354, 60.94286399630310314 ) ) ;
#15879=EDGE_CURVE ( 'NONE', #37877, #2353, #11118, .T. ) ;
#15881=CARTESIAN_POINT ( 'NONE',  ( -20.93791933404421002, -8.239859431045912785, 59.94851102954661570 ) ) ;
#15882=VERTEX_POINT ( 'NONE', #29093 ) ;
#15884=CARTESIAN_POINT ( 'NONE',  ( -24.05845721068777010, -12.57644527891515551, 73.54225570276561541 ) ) ;
#15885=CARTESIAN_POINT ( 'NONE',  ( -10.41531639268335496, -14.04517892474411589, 60.93293405735092705 ) ) ;
#15886=DIRECTION ( 'NONE',  ( -5.731567514496413899E-31, -1.020425574103664789E-16, -1.000000000000000000 ) ) ;
#15887=CARTESIAN_POINT ( 'NONE',  ( -24.35389707626741185, -16.10709931453380861, 62.87856533165624029 ) ) ;
#15889=EDGE_CURVE ( 'NONE', #19236, #46816, #13245, .T. ) ;
#15890=DIRECTION ( 'NONE',  ( 0.9048399035850771543, 0.4257519804770706906, 1.330923649722295736E-08 ) ) ;
#15892=PLANE ( 'NONE',  #31535 ) ;
#15894=CARTESIAN_POINT ( 'NONE',  ( -11.19247825287758857, -11.62036905852712110, 67.91864580735541779 ) ) ;
#15895=CARTESIAN_POINT ( 'NONE',  ( -11.05034076241727625, -11.79557573020262318, 71.37388789199357575 ) ) ;
#15896=EDGE_LOOP ( 'NONE', ( #9647, #25368 ) ) ;
#15897=DIRECTION ( 'NONE',  ( 0.9848822020395751053, -0.1732254256905498280, -7.367703375118635757E-08 ) ) ;
#15898=FACE_BOUND ( 'NONE', #9767, .T. ) ;
#15899=VERTEX_POINT ( 'NONE', #3470 ) ;
#15900=EDGE_LOOP ( 'NONE', ( #3240, #19577, #8313, #44205, #21133 ) ) ;
#15901=ORIENTED_EDGE ( 'NONE', *, *, #28820, .F. ) ;
#15902=CARTESIAN_POINT ( 'NONE',  ( -10.43098718212803000, -15.70539730037032911, 61.32316937334011442 ) ) ;
#15904=CARTESIAN_POINT ( 'NONE',  ( -16.65185932245351808, -21.81708442718849383, 65.51092266128213737 ) ) ;
#15905=( BOUNDED_SURFACE ( )  B_SPLINE_SURFACE ( 3, 1, ( 
 ( #41204, #48108 ),
 ( #37743, #3784 ),
 ( #18794, #33801 ),
 ( #21764, #15085 ),
 ( #36750, #41440 ),
 ( #7738, #48341 ),
 ( #22752, #3039 ) ),
 .UNSPECIFIED., .T., .F., .F. ) 
 B_SPLINE_SURFACE_WITH_KNOTS ( ( 4, 3, 4 ),
 ( 2, 2 ),
 ( 0.000000000000000000, 0.5000000000000000000, 1.000000000000000000 ),
 ( 0.000000000000000000, 1.000000000000000000 ),
 .UNSPECIFIED. ) 
 GEOMETRIC_REPRESENTATION_ITEM ( )  RATIONAL_B_SPLINE_SURFACE ( (
 ( 1.000000000000000000, 1.000000000000000000),
 ( 0.3333333333333335369, 0.3333333333333330373),
 ( 0.3333333333333335369, 0.3333333333333330373),
 ( 1.000000000000000000, 1.000000000000000000),
 ( 0.3333333333333333703, 0.3333333333333333703),
 ( 0.3333333333333333703, 0.3333333333333333703),
 ( 1.000000000000000000, 1.000000000000000000) ) ) 
 REPRESENTATION_ITEM ( '' )  SURFACE ( )  );
#15906=CARTESIAN_POINT ( 'NONE',  ( -21.27305602007818663, -8.962297277456373834, 73.88663334704315844 ) ) ;
#15907=CARTESIAN_POINT ( 'NONE',  ( -11.83648969670631068, -9.881597305254256725, 64.12890704636625117 ) ) ;
#15908=DIRECTION ( 'NONE',  ( -0.9918916210775228226, -0.1270866320121812332, 6.503929234589264523E-08 ) ) ;
#15909=VERTEX_POINT ( 'NONE', #41150 ) ;
#15910=ORIENTED_EDGE ( 'NONE', *, *, #26350, .T. ) ;
#15912=CARTESIAN_POINT ( 'NONE',  ( -13.73367451952834095, -20.81619193053765926, 65.28628851148928902 ) ) ;
#15913=DIRECTION ( 'NONE',  ( 8.329294198805576557E-07, -2.487164606213012505E-06, 0.9999999999965599740 ) ) ;
#15914=DIRECTION ( 'NONE',  ( 0.3478314405900309603, 0.9375570856950864451, -9.567072274253696421E-17 ) ) ;
#15916=ADVANCED_FACE ( 'NONE', ( #3234 ), #33245, .T. ) ;
#15918=( BOUNDED_CURVE ( )  B_SPLINE_CURVE ( 3, ( #22649, #2942, #4, #29303 ),
 .UNSPECIFIED., .F., .F. ) 
 B_SPLINE_CURVE_WITH_KNOTS ( ( 4, 4 ),
 ( 1.570796326794896558, 1.780235837034217727 ),
 .UNSPECIFIED. ) 
 CURVE ( )  GEOMETRIC_REPRESENTATION_ITEM ( )  RATIONAL_B_SPLINE_CURVE ( ( 1.000000000000000000, 0.9963479302455154896, 0.9963479302455154896, 1.000000000000000000 ) ) 
 REPRESENTATION_ITEM ( '' )  );
#15921=ADVANCED_FACE ( 'NONE', ( #47807 ), #1368, .T. ) ;
#15922=CARTESIAN_POINT ( 'NONE',  ( -10.51729497052147977, -16.22293520194095606, 71.74750383215044280 ) ) ;
#15923=CARTESIAN_POINT ( 'NONE',  ( -10.04821600842096174, -15.85811274820897410, 64.62276192103250594 ) ) ;
#15926=CARTESIAN_POINT ( 'NONE',  ( -11.60526899143904345, -18.79015832504765271, 68.23161775275829655 ) ) ;
#15927=CARTESIAN_POINT ( 'NONE',  ( -12.15286730501820678, -9.544433317881530598, 57.34581436681493471 ) ) ;
#15929=VERTEX_POINT ( 'NONE', #3724 ) ;
#15930=CARTESIAN_POINT ( 'NONE',  ( -12.24833890097646005, -19.59612930767528738, 58.22682369889817267 ) ) ;
#15932=CARTESIAN_POINT ( 'NONE',  ( -17.36175868705992897, -7.359389033274929659, 67.06393689457253515 ) ) ;
#15933=CARTESIAN_POINT ( 'NONE',  ( -11.46875891826176819, -18.48806303968299858, 61.27710833525312495 ) ) ;
#15934=ORIENTED_EDGE ( 'NONE', *, *, #42800, .T. ) ;
#15935=CARTESIAN_POINT ( 'NONE',  ( -10.38847021856859421, -14.31440148336201545, 60.80332504197532728 ) ) ;
#15936=ORIENTED_EDGE ( 'NONE', *, *, #23779, .T. ) ;
#15937=CARTESIAN_POINT ( 'NONE',  ( -9.975463547418753407, -14.66361225716259575, 71.43508524632446210 ) ) ;
#15939=EDGE_CURVE ( 'NONE', #6635, #28650, #7431, .T. ) ;
#15940=EDGE_LOOP ( 'NONE', ( #25746, #25959, #10701, #8973, #15390 ) ) ;
#15941=CARTESIAN_POINT ( 'NONE',  ( -16.22845603143158755, -22.16339683637704638, 61.94223519165076652 ) ) ;
#15942=CARTESIAN_POINT ( 'NONE',  ( -17.98657259272421172, -21.83703102787368167, 62.16063850355641307 ) ) ;
#15943=CARTESIAN_POINT ( 'NONE',  ( -14.21750986585362320, -8.084461106059640301, 67.43691998704751711 ) ) ;
#15944=VERTEX_POINT ( 'NONE', #45110 ) ;
#15945=DIRECTION ( 'NONE',  ( -1.077913161506870186E-05, 7.121115479698836302E-06, 0.9999999999165498643 ) ) ;
#15946=EDGE_CURVE ( 'NONE', #44664, #35872, #22691, .T. ) ;
#15949=CYLINDRICAL_SURFACE ( 'NONE', #2291, 0.1499999999999948874 ) ;
#15952=CARTESIAN_POINT ( 'NONE',  ( -21.84598475011588903, -8.812495317756813051, 70.31787921227815730 ) ) ;
#15959=CARTESIAN_POINT ( 'NONE',  ( -24.82767328945774210, -13.97813652794827988, 73.16625576376715401 ) ) ;
#15960=CARTESIAN_POINT ( 'NONE',  ( -12.69763806180496601, -20.04058448603118592, 68.62185382311069759 ) ) ;
#15961=CARTESIAN_POINT ( 'NONE',  ( -10.72530867274958410, -17.00760959713300835, 57.97288447305809456 ) ) ;
#15962=CARTESIAN_POINT ( 'NONE',  ( -10.56317305444034105, -16.44707251114675728, 71.44750086157920066 ) ) ;
#15963=ORIENTED_EDGE ( 'NONE', *, *, #21918, .F. ) ;
#15964=ORIENTED_EDGE ( 'NONE', *, *, #39882, .T. ) ;
#15965=CARTESIAN_POINT ( 'NONE',  ( -11.32522400900782067, -11.27219014254736074, 60.96413645226084554 ) ) ;
#15967=CARTESIAN_POINT ( 'NONE',  ( -14.60783614669699304, -21.70648650955843806, 58.35113213314874514 ) ) ;
#15968=CARTESIAN_POINT ( 'NONE',  ( -10.93232766038821424, -17.55941949638709687, 68.38249893951126523 ) ) ;
#15969=CARTESIAN_POINT ( 'NONE',  ( -18.66311988809301425, -7.868636481342422329, 70.65595886192740238 ) ) ;
#15970=ADVANCED_FACE ( 'NONE', ( #21949 ), #41939, .T. ) ;
#15971=VERTEX_POINT ( 'NONE', #12979 ) ;
#15972=B_SPLINE_CURVE_WITH_KNOTS ( 'NONE', 1,
 ( #41269, #30213 ),
 .UNSPECIFIED., .F., .F.,
 ( 2, 2 ),
 ( 0.000000000000000000, 1.000000000000000000 ),
 .UNSPECIFIED. ) ;
#15974=CYLINDRICAL_SURFACE ( 'NONE', #22539, 0.1500000000000065448 ) ;
#15975=CARTESIAN_POINT ( 'NONE',  ( -24.86969121598721344, -14.53217971827670496, 66.36947994509128534 ) ) ;
#15977=CARTESIAN_POINT ( 'NONE',  ( -24.03161744405940325, -17.27608056677072312, 73.29824685711943744 ) ) ;
#15979=CARTESIAN_POINT ( 'NONE',  ( -13.10126076353387603, -9.301845420481674509, 70.92095663008969098 ) ) ;
#15980=CARTESIAN_POINT ( 'NONE',  ( -24.80769047312930553, -15.80232199467591947, 69.71802767292497549 ) ) ;
#15981=EDGE_LOOP ( 'NONE', ( #38939, #16903 ) ) ;
#15982=EDGE_CURVE ( 'NONE', #39713, #21906, #5373, .T. ) ;
#15983=CARTESIAN_POINT ( 'NONE',  ( -20.00946575929301474, -8.250368826910309039, 74.02096600124984604 ) ) ;
#15986=B_SPLINE_CURVE_WITH_KNOTS ( 'NONE', 3,
 ( #16712, #46292, #23891, #42109, #34458, #9109, #746, #8373, #23397, #38393 ),
 .UNSPECIFIED., .F., .F.,
 ( 4, 2, 2, 2, 4 ),
 ( 0.000000000000000000, 0.2500000000000000000, 0.5000000000000000000, 0.7500000000000000000, 1.000000000000000000 ),
 .UNSPECIFIED. ) ;
#15987=CARTESIAN_POINT ( 'NONE',  ( -23.66133310609451712, -18.88359296917171903, 69.40876596050124192 ) ) ;
#15988=ORIENTED_EDGE ( 'NONE', *, *, #16553, .T. ) ;
#15989=FACE_OUTER_BOUND ( 'NONE', #39228, .T. ) ;
#15991=CARTESIAN_POINT ( 'NONE',  ( -19.26584314952366128, -21.56270023830151317, 58.82507339201525554 ) ) ;
#15992=VERTEX_POINT ( 'NONE', #20390 ) ;
#15994=CARTESIAN_POINT ( 'NONE',  ( -10.28660183209414569, -12.67406856256811309, 64.46847312737159541 ) ) ;
#15997=FACE_OUTER_BOUND ( 'NONE', #9340, .T. ) ;
#15999=CARTESIAN_POINT ( 'NONE',  ( -19.17403394478084522, -7.567564808342563509, 63.47443287871421091 ) ) ;
#16000=CARTESIAN_POINT ( 'NONE',  ( -13.39423282786765590, -8.543200923198597252, 57.16978962524147789 ) ) ;
#16001=ORIENTED_EDGE ( 'NONE', *, *, #10035, .F. ) ;
#16002=LINE ( 'NONE', #519, #3493 ) ;
#16003=CARTESIAN_POINT ( 'NONE',  ( -13.18342752238402582, -20.93459749068556874, 58.09004124675303160 ) ) ;
#16006=PLANE ( 'NONE',  #16030 ) ;
#16008=ORIENTED_EDGE ( 'NONE', *, *, #8083, .F. ) ;
#16009=CARTESIAN_POINT ( 'NONE',  ( -18.63018860987378389, -7.457396320151260305, 73.95569119842126327 ) ) ;
#16010=DIRECTION ( 'NONE',  ( 5.104528489711356381E-07, 5.317498756133547718E-07, 0.9999999999997283284 ) ) ;
#16012=CARTESIAN_POINT ( 'NONE',  ( -22.28468842640968006, -19.91619389767071269, 65.98949666203347419 ) ) ;
#16015=CARTESIAN_POINT ( 'NONE',  ( -10.48067351556794158, -16.03044098841782628, 68.27767830705533925 ) ) ;
#16016=EDGE_CURVE ( 'NONE', #20234, #48679, #46736, .T. ) ;
#16017=CARTESIAN_POINT ( 'NONE',  ( -21.60438134605806226, -20.97601912272344293, 72.70163284247159652 ) ) ;
#16018=CARTESIAN_POINT ( 'NONE',  ( -15.82706446313400939, -7.992505727924407388, 70.68160198162291863 ) ) ;
#16019=CARTESIAN_POINT ( 'NONE',  ( -14.09914643654217947, -8.649277595337252933, 74.49954655170296292 ) ) ;
#16020=EDGE_CURVE ( 'NONE', #14239, #37402, #2105, .T. ) ;
#16021=ORIENTED_EDGE ( 'NONE', *, *, #29551, .F. ) ;
#16026=CARTESIAN_POINT ( 'NONE',  ( -17.59211730330735435, -7.811223398082945302, 63.85057029380297422 ) ) ;
#16028=ORIENTED_EDGE ( 'NONE', *, *, #11107, .F. ) ;
#16029=EDGE_LOOP ( 'NONE', ( #48018, #21146, #25549, #20060, #44973 ) ) ;
#16030=AXIS2_PLACEMENT_3D ( 'NONE', #2460, #14237, #21429 ) ;
#16031=FACE_OUTER_BOUND ( 'NONE', #23754, .T. ) ;
#16033=CARTESIAN_POINT ( 'NONE',  ( -11.34829033918305718, -18.40080557649748272, 64.89140246238697785 ) ) ;
#16035=CARTESIAN_POINT ( 'NONE',  ( -18.48682678124872680, -7.839616045628057250, 74.13504580984984216 ) ) ;
#16036=( BOUNDED_SURFACE ( )  B_SPLINE_SURFACE ( 3, 1, ( 
 ( #36593, #24819 ),
 ( #17653, #32906 ),
 ( #39588, #25062 ),
 ( #17417, #44036 ),
 ( #29236, #48184 ),
 ( #21377, #13472 ),
 ( #2157, #43298 ) ),
 .UNSPECIFIED., .T., .F., .F. ) 
 B_SPLINE_SURFACE_WITH_KNOTS ( ( 4, 3, 4 ),
 ( 2, 2 ),
 ( 0.000000000000000000, 0.5000000000000000000, 1.000000000000000000 ),
 ( 0.000000000000000000, 1.000000000000000000 ),
 .UNSPECIFIED. ) 
 GEOMETRIC_REPRESENTATION_ITEM ( )  RATIONAL_B_SPLINE_SURFACE ( (
 ( 1.000000000000000000, 1.000000000000000000),
 ( 0.3333333333333335369, 0.3333333333333330373),
 ( 0.3333333333333335369, 0.3333333333333330373),
 ( 1.000000000000000000, 1.000000000000000000),
 ( 0.3333333333333333703, 0.3333333333333333703),
 ( 0.3333333333333333703, 0.3333333333333333703),
 ( 1.000000000000000000, 1.000000000000000000) ) ) 
 REPRESENTATION_ITEM ( '' )  SURFACE ( )  );
#16037=EDGE_LOOP ( 'NONE', ( #9648, #21640, #48640, #45482, #26104 ) ) ;
#16039=CARTESIAN_POINT ( 'NONE',  ( -11.23900738907041941, -11.53116396801028287, 64.37555317960440959 ) ) ;
#16042=CYLINDRICAL_SURFACE ( 'NONE', #44629, 0.1499999999999977185 ) ;
#16043=VERTEX_POINT ( 'NONE', #1907 ) ;
#16044=CARTESIAN_POINT ( 'NONE',  ( -19.60932529797995727, -21.51514414075818493, 69.34971148877966129 ) ) ;
#16045=( BOUNDED_CURVE ( )  B_SPLINE_CURVE ( 3, ( #32384, #10687, #13638, #21541 ),
 .UNSPECIFIED., .F., .F. ) 
 B_SPLINE_CURVE_WITH_KNOTS ( ( 4, 4 ),
 ( 0.9074455897393624015, 1.000000000000000000 ),
 .UNSPECIFIED. ) 
 CURVE ( )  GEOMETRIC_REPRESENTATION_ITEM ( )  RATIONAL_B_SPLINE_CURVE ( ( 0.6983129098260905110, 0.7760317562606959818, 0.8765941196519991818, 1.000000000000000000 ) ) 
 REPRESENTATION_ITEM ( '' )  );
#16046=CARTESIAN_POINT ( 'NONE',  ( -13.53974279883776255, -21.16658004109286040, 65.16345737345569944 ) ) ;
#16047=ORIENTED_EDGE ( 'NONE', *, *, #29658, .F. ) ;
#16048=CARTESIAN_POINT ( 'NONE',  ( -11.14521337614216101, -10.79921377940424954, 57.33186350582411706 ) ) ;
#16050=ADVANCED_FACE ( 'NONE', ( #8583 ), #31948, .T. ) ;
#16051=CARTESIAN_POINT ( 'NONE',  ( -17.22979626510402085, -7.361617988748135666, 70.66848571475107121 ) ) ;
#16052=ORIENTED_EDGE ( 'NONE', *, *, #8939, .T. ) ;
#16053=CARTESIAN_POINT ( 'NONE',  ( -19.71243449262119896, -21.42506837973052214, 68.95099091562512683 ) ) ;
#16054=CARTESIAN_POINT ( 'NONE',  ( -17.76560209638259025, -21.80099384504234550, 58.70553380167749680 ) ) ;
#16055=CARTESIAN_POINT ( 'NONE',  ( -11.59533477946176738, -10.16928643397592325, 71.07618957754787914 ) ) ;
#16056=CARTESIAN_POINT ( 'NONE',  ( -21.24416713127566325, -21.20535426119284139, 65.62808000370414163 ) ) ;
#16059=( BOUNDED_SURFACE ( )  B_SPLINE_SURFACE ( 3, 1, ( 
 ( #44952, #11205 ),
 ( #19068, #15352 ),
 ( #11432, #45430 ),
 ( #11683, #26710 ),
 ( #41725, #46642 ),
 ( #1814, #1083 ),
 ( #1568, #31619 ) ),
 .UNSPECIFIED., .T., .F., .F. ) 
 B_SPLINE_SURFACE_WITH_KNOTS ( ( 4, 3, 4 ),
 ( 2, 2 ),
 ( 0.000000000000000000, 0.5000000000000000000, 1.000000000000000000 ),
 ( 0.000000000000000000, 1.000000000000000000 ),
 .UNSPECIFIED. ) 
 GEOMETRIC_REPRESENTATION_ITEM ( )  RATIONAL_B_SPLINE_SURFACE ( (
 ( 1.000000000000000000, 1.000000000000000000),
 ( 0.3333333333333335369, 0.3333333333333330373),
 ( 0.3333333333333335369, 0.3333333333333330373),
 ( 1.000000000000000000, 1.000000000000000000),
 ( 0.3333333333333333703, 0.3333333333333333703),
 ( 0.3333333333333333703, 0.3333333333333333703),
 ( 1.000000000000000000, 1.000000000000000000) ) ) 
 REPRESENTATION_ITEM ( '' )  SURFACE ( )  );
#16060=CARTESIAN_POINT ( 'NONE',  ( -19.85891393954322837, -21.37210614461000446, 47.99999999999994316 ) ) ;
#16061=DIRECTION ( 'NONE',  ( 0.9774082387306984865, -0.2113602016968848807, 7.903122840289808494E-08 ) ) ;
#16062=CARTESIAN_POINT ( 'NONE',  ( -11.10681587527927938, -11.67891925637714401, 71.10332952723315714 ) ) ;
#16064=AXIS2_PLACEMENT_3D ( 'NONE', #47281, #20928, #28564 ) ;
#16066=CARTESIAN_POINT ( 'NONE',  ( -21.66247382830096768, -9.170857770714572865, 63.19153610464900339 ) ) ;
#16067=CARTESIAN_POINT ( 'NONE',  ( -11.02793337088870729, -10.98921060197374722, 60.87224103154665045 ) ) ;
#16068=EDGE_LOOP ( 'NONE', ( #37, #1050, #28071, #46616, #45351 ) ) ;
#16070=CARTESIAN_POINT ( 'NONE',  ( -10.78171168112265832, -12.44661727924501449, 57.62857332509076969 ) ) ;
#16071=CARTESIAN_POINT ( 'NONE',  ( -23.26235167723834962, -10.18112620132981228, 63.19469118497043780 ) ) ;
#16072=CARTESIAN_POINT ( 'NONE',  ( -20.51885330616224579, -21.64595032723701706, 54.15157107980257933 ) ) ;
#16074=CARTESIAN_POINT ( 'NONE',  ( -24.40552668661833735, -14.29970115358017502, 66.37395989550236663 ) ) ;
#16075=EDGE_CURVE ( 'NONE', #5574, #32131, #19738, .T. ) ;
#16077=CARTESIAN_POINT ( 'NONE',  ( -24.02981955162125516, -11.36410642080215894, 66.60027269894509061 ) ) ;
#16078=ADVANCED_FACE ( 'NONE', ( #46249 ), #19937, .T. ) ;
#16079=EDGE_CURVE ( 'NONE', #23975, #6043, #38472, .T. ) ;
#16080=ORIENTED_EDGE ( 'NONE', *, *, #2685, .F. ) ;
#16081=CARTESIAN_POINT ( 'NONE',  ( -17.53499440593470737, -7.752105970505813737, 70.63468544436783247 ) ) ;
#16082=CARTESIAN_POINT ( 'NONE',  ( -24.17899325218984785, -11.66673737571591296, 59.66731058339561855 ) ) ;
#16083=CARTESIAN_POINT ( 'NONE',  ( -10.40245588357037043, -14.17414831712846990, 61.20349182037644198 ) ) ;
#16084=CARTESIAN_POINT ( 'NONE',  ( -21.75000248771700129, -8.743799152774244021, 70.23108901470999399 ) ) ;
#16085=DIRECTION ( 'NONE',  ( 2.526377665399295826E-06, 1.273612633031948423E-05, -0.9999999999157042074 ) ) ;
#16086=ORIENTED_EDGE ( 'NONE', *, *, #32853, .T. ) ;
#16087=ORIENTED_EDGE ( 'NONE', *, *, #3325, .F. ) ;
#16090=DIRECTION ( 'NONE',  ( 0.7915359335728472390, 0.6111226275167354061, 5.146443701300905010E-08 ) ) ;
#16091=VECTOR ( 'NONE', #5367, 1000.000000000000114 ) ;
#16092=CARTESIAN_POINT ( 'NONE',  ( -10.81484411697162962, -17.11524594140972155, 61.15743118925659161 ) ) ;
#16095=CARTESIAN_POINT ( 'NONE',  ( -13.85393748347032528, -8.270264590973253505, 74.38449983516251507 ) ) ;
#16096=ORIENTED_EDGE ( 'NONE', *, *, #31645, .T. ) ;
#16098=CARTESIAN_POINT ( 'NONE',  ( -10.38888248908913958, -14.35051868308065437, 64.68244075910853041 ) ) ;
#16099=ORIENTED_EDGE ( 'NONE', *, *, #14486, .F. ) ;
#16100=CARTESIAN_POINT ( 'NONE',  ( -13.36402663293916682, -21.05582000094733530, 61.63833528390372152 ) ) ;
#16101=EDGE_LOOP ( 'NONE', ( #18168, #36620, #14495, #17187, #16291 ) ) ;
#16102=LINE ( 'NONE', #15623, #12810 ) ;
#16103=EDGE_CURVE ( 'NONE', #16763, #25179, #26848, .T. ) ;
#16104=CARTESIAN_POINT ( 'NONE',  ( -21.92407967000237790, -20.23628646485057914, 58.76442916245459003 ) ) ;
#16105=EDGE_CURVE ( 'NONE', #37668, #40518, #42228, .T. ) ;
#16106=CARTESIAN_POINT ( 'NONE',  ( -15.13863373983067717, -21.47863424849249014, 65.40036913793611006 ) ) ;
#16107=CARTESIAN_POINT ( 'NONE',  ( -22.48114103837971101, -19.64927616005747879, 72.64400547034465205 ) ) ;
#16108=EDGE_LOOP ( 'NONE', ( #13318, #32866, #40552, #35273, #2531 ) ) ;
#16109=CARTESIAN_POINT ( 'NONE',  ( -18.71262049920375503, -21.74350751539899562, 72.17022092985547488 ) ) ;
#16110=CARTESIAN_POINT ( 'NONE',  ( -17.77063367917941861, -22.25119205618777585, 58.51215086126244103 ) ) ;
#16111=CARTESIAN_POINT ( 'NONE',  ( -10.88583436550758776, -11.23762803245173103, 64.30915376540053785 ) ) ;
#16112=FACE_BOUND ( 'NONE', #10605, .T. ) ;
#16114=B_SPLINE_CURVE_WITH_KNOTS ( 'NONE', 1,
 ( #13368, #17552 ),
 .UNSPECIFIED., .F., .F.,
 ( 2, 2 ),
 ( 0.000000000000000000, 1.000000000000000000 ),
 .UNSPECIFIED. ) ;
#16115=CARTESIAN_POINT ( 'NONE',  ( -22.83929682888979329, -10.29453308790037980, 66.55654356380499337 ) ) ;
#16116=CYLINDRICAL_SURFACE ( 'NONE', #35787, 0.1499999999999985234 ) ;
#16117=B_SPLINE_CURVE_WITH_KNOTS ( 'NONE', 3,
 ( #8349, #11547, #1185, #19675, #7875, #7632, #12040, #22637, #37633, #26573 ),
 .UNSPECIFIED., .F., .F.,
 ( 4, 2, 2, 2, 4 ),
 ( 0.6272669072878104268, 0.7522669073073157131, 0.8772669073268208884, 1.002266907346326175, 1.127266907365831461 ),
 .UNSPECIFIED. ) ;
#16119=ORIENTED_EDGE ( 'NONE', *, *, #22985, .T. ) ;
#16120=CARTESIAN_POINT ( 'NONE',  ( -12.08002915394404120, -10.28786663478488350, 67.79896886176341297 ) ) ;
#16122=CARTESIAN_POINT ( 'NONE',  ( -20.08713612207380450, -21.76716563359125800, 72.56625224360259097 ) ) ;
#16124=B_SPLINE_CURVE_WITH_KNOTS ( 'NONE', 3,
 ( #29592, #3737, #41163, #52, #6946, #11609, #3990, #7693, #44623, #21962 ),
 .UNSPECIFIED., .F., .F.,
 ( 4, 2, 2, 2, 4 ),
 ( 0.000000000000000000, 0.2500000000000000000, 0.5000000000000000000, 0.7500000000000000000, 1.000000000000000000 ),
 .UNSPECIFIED. ) ;
#16126=CYLINDRICAL_SURFACE ( 'NONE', #1204, 0.1499999999999994671 ) ;
#16127=AXIS2_PLACEMENT_3D ( 'NONE', #17769, #32797, #3253 ) ;
#16128=FACE_BOUND ( 'NONE', #37477, .T. ) ;
#16131=ADVANCED_FACE ( 'NONE', ( #5854 ), #9872, .T. ) ;
#16133=VERTEX_POINT ( 'NONE', #21115 ) ;
#16134=CARTESIAN_POINT ( 'NONE',  ( -18.25645571269274825, -21.81792545032241293, 62.03103110229211836 ) ) ;
#16135=CARTESIAN_POINT ( 'NONE',  ( -13.14999064602648637, -9.265557826385967033, 67.37942786034257381 ) ) ;
#16136=CARTESIAN_POINT ( 'NONE',  ( -24.44055745662519641, -14.11932379769929113, 73.13743607903229815 ) ) ;
#16138=CARTESIAN_POINT ( 'NONE',  ( -12.65491863400508876, -19.93331718326324165, 68.33657436096362403 ) ) ;
#16139=CARTESIAN_POINT ( 'NONE',  ( -10.75331649400429868, -16.93069871048427544, 57.68760548944693056 ) ) ;
#16140=ORIENTED_EDGE ( 'NONE', *, *, #436, .T. ) ;
#16142=EDGE_CURVE ( 'NONE', #9880, #5480, #13851, .T. ) ;
#16145=EDGE_CURVE ( 'NONE', #10344, #43128, #20218, .T. ) ;
#16146=CARTESIAN_POINT ( 'NONE',  ( -21.29196722032537537, -20.70380199363843232, 72.53918572867779346 ) ) ;
#16147=CARTESIAN_POINT ( 'NONE',  ( -10.52311507911083055, -15.98310348350391230, 68.27767878681093805 ) ) ;
#16149=ADVANCED_FACE ( 'NONE', ( #14903 ), #34359, .T. ) ;
#16150=ORIENTED_EDGE ( 'NONE', *, *, #24281, .T. ) ;
#16153=DIRECTION ( 'NONE',  ( -0.5881408891789769999, -0.8087584895849666555, 7.565907428972491290E-08 ) ) ;
#16154=ADVANCED_FACE ( 'NONE', ( #41041 ), #26757, .T. ) ;
#16155=CARTESIAN_POINT ( 'NONE',  ( -12.41310947992116098, -19.76871611099698001, 61.68206578716802113 ) ) ;
#16156=CARTESIAN_POINT ( 'NONE',  ( -17.42409385541300892, -14.80920654474439679, 47.99999999999994316 ) ) ;
#16158=FACE_OUTER_BOUND ( 'NONE', #33277, .T. ) ;
#16159=LINE ( 'NONE', #38830, #2358 ) ;
#16160=CARTESIAN_POINT ( 'NONE',  ( -10.71605034603323148, -17.00400043661996108, 64.77172137060364321 ) ) ;
#16163=ORIENTED_EDGE ( 'NONE', *, *, #2829, .F. ) ;
#16164=CARTESIAN_POINT ( 'NONE',  ( -10.45256735519816615, -15.43993469624229853, 57.56792809193251514 ) ) ;
#16165=CARTESIAN_POINT ( 'NONE',  ( -23.85748962928175132, -11.92509172808648543, 59.49707787073156595 ) ) ;
#16166=CARTESIAN_POINT ( 'NONE',  ( -12.40538999107997498, -20.31523868419091272, 68.52152871938794476 ) ) ;
#16169=ORIENTED_EDGE ( 'NONE', *, *, #19039, .T. ) ;
#16170=CARTESIAN_POINT ( 'NONE',  ( -15.06305009558132646, -21.87596932251961590, 65.21941411614068329 ) ) ;
#16172=B_SPLINE_CURVE_WITH_KNOTS ( 'NONE', 1,
 ( #25533, #3124 ),
 .UNSPECIFIED., .F., .F.,
 ( 2, 2 ),
 ( 0.000000000000000000, 1.000000000000000000 ),
 .UNSPECIFIED. ) ;
#16174=CARTESIAN_POINT ( 'NONE',  ( -22.19081608276703221, -20.53467296680696563, 58.96454102209866477 ) ) ;
#16176=CARTESIAN_POINT ( 'NONE',  ( -24.25372049150513831, -13.26839097538318946, 63.06094141181949198 ) ) ;
#16177=CARTESIAN_POINT ( 'NONE',  ( -10.43073325114686511, -14.50439929630985603, 68.15800126138398696 ) ) ;
#16178=VERTEX_POINT ( 'NONE', #30217 ) ;
#16179=CARTESIAN_POINT ( 'NONE',  ( -21.34582024633207098, -20.66775256773563285, 72.67446429491059234 ) ) ;
#16180=DIRECTION ( 'NONE',  ( -0.8604039311673230550, -0.5096126717731922495, 7.110477544621476444E-08 ) ) ;
#16181=EDGE_CURVE ( 'NONE', #22557, #39502, #32629, .T. ) ;
#16182=CARTESIAN_POINT ( 'NONE',  ( -23.58525830889974984, -18.99772868593042219, 65.86743475655129032 ) ) ;
#16183=( BOUNDED_CURVE ( )  B_SPLINE_CURVE ( 3, ( #28190, #20571, #32377, #47630 ),
 .UNSPECIFIED., .F., .F. ) 
 B_SPLINE_CURVE_WITH_KNOTS ( ( 4, 4 ),
 ( 0.9074455897393697290, 1.000000000000000000 ),
 .UNSPECIFIED. ) 
 CURVE ( )  GEOMETRIC_REPRESENTATION_ITEM ( )  RATIONAL_B_SPLINE_CURVE ( ( 0.6983129098260940637, 0.7760317562606990904, 0.8765941196520010692, 1.000000000000000000 ) ) 
 REPRESENTATION_ITEM ( '' )  );
#16184=CARTESIAN_POINT ( 'NONE',  ( -22.27817919856018136, -9.157513542003881568, 59.83675792137641736 ) ) ;
#16185=ORIENTED_EDGE ( 'NONE', *, *, #33872, .T. ) ;
#16186=CARTESIAN_POINT ( 'NONE',  ( -15.68463861365884249, -7.564349260043091938, 67.25351876580783994 ) ) ;
#16189=ORIENTED_EDGE ( 'NONE', *, *, #34171, .T. ) ;
#16190=ORIENTED_EDGE ( 'NONE', *, *, #20467, .F. ) ;
#16192=CARTESIAN_POINT ( 'NONE',  ( -23.83833621072449560, -17.61232891644574394, 62.47360984984814536 ) ) ;
#16197=( BOUNDED_CURVE ( )  B_SPLINE_CURVE ( 3, ( #14055, #37195, #29104, #36956 ),
 .UNSPECIFIED., .F., .F. ) 
 B_SPLINE_CURVE_WITH_KNOTS ( ( 4, 4 ),
 ( 0.9074455897393632897, 1.000000000000000000 ),
 .UNSPECIFIED. ) 
 CURVE ( )  GEOMETRIC_REPRESENTATION_ITEM ( )  RATIONAL_B_SPLINE_CURVE ( ( 0.6983129098260867362, 0.7760317562606927622, 0.8765941196519971834, 1.000000000000000000 ) ) 
 REPRESENTATION_ITEM ( '' )  );
#16198=CARTESIAN_POINT ( 'NONE',  ( -12.36756753426621813, -9.896138138887707214, 57.37463480816234096 ) ) ;
#16200=ORIENTED_EDGE ( 'NONE', *, *, #30101, .F. ) ;
#16201=EDGE_LOOP ( 'NONE', ( #30559, #19071, #11646, #22029, #26713 ) ) ;
#16202=CARTESIAN_POINT ( 'NONE',  ( -10.99586753834015695, -11.04334891231907534, 60.86381058728009208 ) ) ;
#16204=EDGE_CURVE ( 'NONE', #6133, #24855, #7070, .T. ) ;
#16206=CARTESIAN_POINT ( 'NONE',  ( -22.88264614489240856, -10.34704276773305764, 63.35713876973677827 ) ) ;
#16207=EDGE_CURVE ( 'NONE', #21537, #12524, #30307, .T. ) ;
#16208=ORIENTED_EDGE ( 'NONE', *, *, #16858, .T. ) ;
#16209=CARTESIAN_POINT ( 'NONE',  ( -14.13242279744181573, -8.574497162196568212, 74.21426705364891063 ) ) ;
#16210=CARTESIAN_POINT ( 'NONE',  ( -10.78031428196279329, -11.32923628920978310, 53.49999999999994316 ) ) ;
#16211=CARTESIAN_POINT ( 'NONE',  ( -17.17171767447154096, -7.760110763219655539, 67.22859634205599377 ) ) ;
#16212=CARTESIAN_POINT ( 'NONE',  ( -15.83638662446498380, -7.530183628806756957, 67.30153828690920648 ) ) ;
#16213=EDGE_CURVE ( 'NONE', #19324, #20830, #33710, .T. ) ;
#16216=DIRECTION ( 'NONE',  ( -5.731567514496413899E-31, -1.020425574103664789E-16, -1.000000000000000000 ) ) ;
#16218=ORIENTED_EDGE ( 'NONE', *, *, #45271, .F. ) ;
#16219=CARTESIAN_POINT ( 'NONE',  ( -22.63560516303400050, -20.13310814558360917, 69.28922553891734992 ) ) ;
#16220=PLANE ( 'NONE',  #10802 ) ;
#16222=CARTESIAN_POINT ( 'NONE',  ( -23.69601271365505823, -18.82994329453045168, 69.48646111030700467 ) ) ;
#16223=AXIS2_PLACEMENT_3D ( 'NONE', #11070, #33439, #3931 ) ;
#16225=ORIENTED_EDGE ( 'NONE', *, *, #30544, .T. ) ;
#16226=DIRECTION ( 'NONE',  ( 1.206829990107966821E-05, 1.995688255855010801E-06, 0.9999999999251867333 ) ) ;
#16228=ORIENTED_EDGE ( 'NONE', *, *, #4722, .T. ) ;
#16229=CARTESIAN_POINT ( 'NONE',  ( -24.23700366861210753, -17.82382531738836562, 62.73006892227505915 ) ) ;
#16230=CARTESIAN_POINT ( 'NONE',  ( -10.37462440636232053, -14.89569459299594278, 75.09778901493891112 ) ) ;
#16232=CARTESIAN_POINT ( 'NONE',  ( -12.01398263875733718, -10.36526583719368233, 71.04063403505170982 ) ) ;
#16234=EDGE_CURVE ( 'NONE', #40830, #47966, #4117, .T. ) ;
#16236=CARTESIAN_POINT ( 'NONE',  ( -14.66844689667836299, -21.73163918518723037, 61.82255689998408599 ) ) ;
#16237=ORIENTED_EDGE ( 'NONE', *, *, #5260, .T. ) ;
#16238=CARTESIAN_POINT ( 'NONE',  ( -12.27729925481933471, -9.991218852276039897, 60.55918086709623083 ) ) ;
#16239=CARTESIAN_POINT ( 'NONE',  ( -11.97212546196701943, -10.32690635925306211, 74.58318462221375000 ) ) ;
#16242=CARTESIAN_POINT ( 'NONE',  ( -12.20424117383341311, -20.12491952255346206, 65.12320790045656338 ) ) ;
#16243=ORIENTED_EDGE ( 'NONE', *, *, #2089, .F. ) ;
#16244=ORIENTED_EDGE ( 'NONE', *, *, #27858, .T. ) ;
#16245=FACE_OUTER_BOUND ( 'NONE', #10592, .T. ) ;
#16246=CARTESIAN_POINT ( 'NONE',  ( -10.33669513760112224, -12.51310759931308070, 60.99127726887360978 ) ) ;
#16247=EDGE_LOOP ( 'NONE', ( #7069, #47814, #41802, #48290, #27109 ) ) ;
#16248=CARTESIAN_POINT ( 'NONE',  ( -24.35072239393756632, -15.82005629120157231, 66.17210830061728188 ) ) ;
#16249=CARTESIAN_POINT ( 'NONE',  ( -15.77564557227241160, -7.543859306641682139, 67.23983639585463834 ) ) ;
#16250=CARTESIAN_POINT ( 'NONE',  ( -10.27590366065288485, -12.71001274655382041, 64.37497800382601554 ) ) ;
#16254=FACE_OUTER_BOUND ( 'NONE', #46797, .T. ) ;
#16258=ADVANCED_FACE ( 'NONE', ( #45730 ), #22321, .F. ) ;
#16259=CARTESIAN_POINT ( 'NONE',  ( -23.25757715627672795, -10.17517474196413474, 63.18690702823881367 ) ) ;
#16260=CARTESIAN_POINT ( 'NONE',  ( -13.84034316733854730, -20.82276307383959946, 68.47241820953060198 ) ) ;
#16261=CARTESIAN_POINT ( 'NONE',  ( -17.42127804818254688, -7.759166751185505362, 67.02039588450487884 ) ) ;
#16264=VECTOR ( 'NONE', #35947, 1000.000000000000227 ) ;
#16265=ORIENTED_EDGE ( 'NONE', *, *, #4037, .T. ) ;
#16267=CARTESIAN_POINT ( 'NONE',  ( -19.79646526366146375, -21.45124607735644062, 72.81967355032548994 ) ) ;
#16268=EDGE_CURVE ( 'NONE', #26197, #39806, #27311, .T. ) ;
#16271=B_SPLINE_CURVE_WITH_KNOTS ( 'NONE', 3,
 ( #5778, #13375, #17317, #6003, #9474, #17065, #10439, #43692, #21026, #24963 ),
 .UNSPECIFIED., .F., .F.,
 ( 4, 2, 2, 2, 4 ),
 ( 0.000000000000000000, 0.2500000000000000000, 0.5000000000000000000, 0.7500000000000000000, 1.000000000000000000 ),
 .UNSPECIFIED. ) ;
#16272=CARTESIAN_POINT ( 'NONE',  ( -10.96069643151774109, -18.51437482595545347, 57.92219192461608657 ) ) ;
#16273=( BOUNDED_CURVE ( )  B_SPLINE_CURVE ( 3, ( #18261, #7213, #14788, #29856 ),
 .UNSPECIFIED., .F., .F. ) 
 B_SPLINE_CURVE_WITH_KNOTS ( ( 4, 4 ),
 ( 0.000000000000000000, 0.4074455897393664539 ),
 .UNSPECIFIED. ) 
 CURVE ( )  GEOMETRIC_REPRESENTATION_ITEM ( )  RATIONAL_B_SPLINE_CURVE ( ( 1.000000000000000000, 0.4567392136813308579, 0.3561768502900298783, 0.6983129098260970613 ) ) 
 REPRESENTATION_ITEM ( '' )  );
#16274=EDGE_CURVE ( 'NONE', #29274, #42743, #18474, .T. ) ;
#16276=VERTEX_POINT ( 'NONE', #5568 ) ;
#16277=CARTESIAN_POINT ( 'NONE',  ( -17.42409385541300892, -14.80920654474439679, 56.49999999999994316 ) ) ;
#16278=DIRECTION ( 'NONE',  ( 0.8839923186919885767, -0.4675014229855998793, 2.842058574697910297E-08 ) ) ;
#16279=ORIENTED_EDGE ( 'NONE', *, *, #12621, .T. ) ;
#16280=CARTESIAN_POINT ( 'NONE',  ( -17.72634068467203505, -21.85272461955047874, 58.70553378267869959 ) ) ;
#16281=CARTESIAN_POINT ( 'NONE',  ( -10.47141000957850743, -13.99617255615227940, 57.46327426011240647 ) ) ;
#16283=CARTESIAN_POINT ( 'NONE',  ( -10.82281966776723792, -12.48006615504498207, 57.32857332801585670 ) ) ;
#16284=EDGE_CURVE ( 'NONE', #44255, #30207, #8778, .T. ) ;
#16285=LINE ( 'NONE', #9171, #32210 ) ;
#16286=EDGE_CURVE ( 'NONE', #445, #12446, #11982, .T. ) ;
#16287=ORIENTED_EDGE ( 'NONE', *, *, #24122, .T. ) ;
#16288=DIRECTION ( 'NONE',  ( 0.9939059412784551073, 0.1102314832132140626, 5.576311685107536405E-08 ) ) ;
#16289=CARTESIAN_POINT ( 'NONE',  ( -22.23205057465639456, -20.50024631022522925, 58.94159781348408700 ) ) ;
#16291=ORIENTED_EDGE ( 'NONE', *, *, #30824, .F. ) ;
#16295=CARTESIAN_POINT ( 'NONE',  ( -16.20999063017906749, -7.914000527602912172, 63.89841002104740397 ) ) ;
#16296=CARTESIAN_POINT ( 'NONE',  ( -21.12380683100872858, -21.27649256055507365, 65.77109308171978341 ) ) ;
#16297=CARTESIAN_POINT ( 'NONE',  ( -10.97703272106552319, -11.95613849865247680, 74.85280472847954059 ) ) ;
#16298=CARTESIAN_POINT ( 'NONE',  ( -14.78754745127378634, -8.270772244812135909, 60.61996282000563241 ) ) ;
#16302=CARTESIAN_POINT ( 'NONE',  ( -10.35661267713556022, -12.45241038966069347, 60.91358145539074798 ) ) ;
#16303=CARTESIAN_POINT ( 'NONE',  ( -19.92499704562962037, -21.82691083785356057, 69.03508226000913339 ) ) ;
#16305=EDGE_LOOP ( 'NONE', ( #11579, #36179, #38347, #46550, #40039 ) ) ;
#16307=ORIENTED_EDGE ( 'NONE', *, *, #47467, .T. ) ;
#16308=CARTESIAN_POINT ( 'NONE',  ( -14.11063322135152909, -21.03236308526469855, 72.21135587486895702 ) ) ;
#16310=CARTESIAN_POINT ( 'NONE',  ( -16.15533939627269078, -22.15042573278388005, 58.39247240179898313 ) ) ;
#16312=CARTESIAN_POINT ( 'NONE',  ( -24.46714309859813241, -14.49289777169556714, 66.18852495040353290 ) ) ;
#16313=CARTESIAN_POINT ( 'NONE',  ( -18.78767905735283605, -20.13749289187802916, 54.07175714974878389 ) ) ;
#16314=ORIENTED_EDGE ( 'NONE', *, *, #37527, .F. ) ;
#16315=ADVANCED_FACE ( 'NONE', ( #30940 ), #32165, .T. ) ;
#16317=CARTESIAN_POINT ( 'NONE',  ( -14.28913879486226435, -8.050816564744696535, 67.37479651646088996 ) ) ;
#16318=CARTESIAN_POINT ( 'NONE',  ( -14.54881252626503851, -21.68205518681590149, 58.27343714710344358 ) ) ;
#16319=ORIENTED_EDGE ( 'NONE', *, *, #6496, .T. ) ;
#16320=CARTESIAN_POINT ( 'NONE',  ( -18.46801905451614445, -7.836623195388688679, 74.12592262855558545 ) ) ;
#16323=( BOUNDED_CURVE ( )  B_SPLINE_CURVE ( 3, ( #32020, #44328, #17706, #40375 ),
 .UNSPECIFIED., .F., .F. ) 
 B_SPLINE_CURVE_WITH_KNOTS ( ( 4, 4 ),
 ( 0.9074455897393643999, 1.000000000000000000 ),
 .UNSPECIFIED. ) 
 CURVE ( )  GEOMETRIC_REPRESENTATION_ITEM ( )  RATIONAL_B_SPLINE_CURVE ( ( 0.6983129098260918433, 0.7760317562606970920, 0.8765941196519998480, 1.000000000000000000 ) ) 
 REPRESENTATION_ITEM ( '' )  );
#16324=CARTESIAN_POINT ( 'NONE',  ( -21.72530822383671634, -8.726125037250696437, 70.25319750298596944 ) ) ;
#16325=B_SPLINE_CURVE_WITH_KNOTS ( 'NONE', 1,
 ( #18965, #33971 ),
 .UNSPECIFIED., .F., .F.,
 ( 2, 2 ),
 ( 0.000000000000000000, 1.000000000000000000 ),
 .UNSPECIFIED. ) ;
#16327=ORIENTED_EDGE ( 'NONE', *, *, #35573, .F. ) ;
#16328=ORIENTED_EDGE ( 'NONE', *, *, #38164, .T. ) ;
#16330=EDGE_CURVE ( 'NONE', #46532, #34511, #36872, .T. ) ;
#16331=B_SPLINE_CURVE_WITH_KNOTS ( 'NONE', 3,
 ( #1520, #12606, #42664, #8927, #16529, #31566, #35723, #40168, #35965, #27865 ),
 .UNSPECIFIED., .F., .F.,
 ( 4, 2, 2, 2, 4 ),
 ( 0.6272669072782128818, 0.7522669073001225781, 0.8772669073220322744, 1.002266907343941860, 1.127266907365851667 ),
 .UNSPECIFIED. ) ;
#16332=CARTESIAN_POINT ( 'NONE',  ( -18.78767905735283605, -20.13749289187802916, 53.49899999999994549 ) ) ;
#16334=VECTOR ( 'NONE', #18045, 999.9999999999998863 ) ;
#16335=CARTESIAN_POINT ( 'NONE',  ( -15.29626560849200878, -8.084834557582363246, 73.96496852212565898 ) ) ;
#16336=( BOUNDED_SURFACE ( )  B_SPLINE_SURFACE ( 3, 1, ( 
 ( #35034, #31113 ),
 ( #3869, #44752 ),
 ( #835, #4774 ),
 ( #27661, #41045 ),
 ( #42693, #11251 ),
 ( #1302, #33887 ),
 ( #19798, #3609 ) ),
 .UNSPECIFIED., .T., .F., .F. ) 
 B_SPLINE_SURFACE_WITH_KNOTS ( ( 4, 3, 4 ),
 ( 2, 2 ),
 ( 0.000000000000000000, 0.5000000000000000000, 1.000000000000000000 ),
 ( 0.000000000000000000, 1.000000000000000000 ),
 .UNSPECIFIED. ) 
 GEOMETRIC_REPRESENTATION_ITEM ( )  RATIONAL_B_SPLINE_SURFACE ( (
 ( 1.000000000000000000, 1.000000000000000000),
 ( 0.3333333333333335369, 0.3333333333333330373),
 ( 0.3333333333333335369, 0.3333333333333330373),
 ( 1.000000000000000000, 1.000000000000000000),
 ( 0.3333333333333333703, 0.3333333333333333703),
 ( 0.3333333333333333703, 0.3333333333333333703),
 ( 1.000000000000000000, 1.000000000000000000) ) ) 
 REPRESENTATION_ITEM ( '' )  SURFACE ( )  );
#16337=AXIS2_PLACEMENT_3D ( 'NONE', #4511, #23733, #41947 ) ;
#16338=AXIS2_PLACEMENT_3D ( 'NONE', #22428, #3462, #18471 ) ;
#16340=CARTESIAN_POINT ( 'NONE',  ( -24.31537953241868522, -17.64020703937282519, 66.06640318968284475 ) ) ;
#16342=B_SPLINE_CURVE_WITH_KNOTS ( 'NONE', 1,
 ( #20097, #12462 ),
 .UNSPECIFIED., .F., .F.,
 ( 2, 2 ),
 ( 0.000000000000000000, 1.000000000000000000 ),
 .UNSPECIFIED. ) ;
#16343=CARTESIAN_POINT ( 'NONE',  ( -13.97837889017616320, -8.203094814523453238, 74.38609903144701718 ) ) ;
#16344=CARTESIAN_POINT ( 'NONE',  ( -24.00901317767524290, -17.32824147414624960, 69.42811846502259243 ) ) ;
#16345=EDGE_LOOP ( 'NONE', ( #3404, #32388 ) ) ;
#16346=CARTESIAN_POINT ( 'NONE',  ( -21.20679145237652108, -20.70065047275357273, 72.75276402661107511 ) ) ;
#16348=VECTOR ( 'NONE', #5349, 1000.000000000000114 ) ;
#16350=ADVANCED_FACE ( 'NONE', ( #46678 ), #42980, .T. ) ;
#16351=( BOUNDED_CURVE ( )  B_SPLINE_CURVE ( 3, ( #22760, #37752, #19051, #31103 ),
 .UNSPECIFIED., .F., .F. ) 
 B_SPLINE_CURVE_WITH_KNOTS ( ( 4, 4 ),
 ( 0.000000000000000000, 0.4074455897393624015 ),
 .UNSPECIFIED. ) 
 CURVE ( )  GEOMETRIC_REPRESENTATION_ITEM ( )  RATIONAL_B_SPLINE_CURVE ( ( 1.000000000000000000, 0.4567392136813347436, 0.3561768502900313216, 0.6983129098260898449 ) ) 
 REPRESENTATION_ITEM ( '' )  );
#16352=B_SPLINE_CURVE_WITH_KNOTS ( 'NONE', 3,
 ( #27169, #3793, #12148, #41707, #4765, #19790, #33811, #7993, #109, #23009 ),
 .UNSPECIFIED., .F., .F.,
 ( 4, 2, 2, 2, 4 ),
 ( 0.000000000000000000, 0.2500000000000000000, 0.5000000000000000000, 0.7500000000000000000, 1.000000000000000000 ),
 .UNSPECIFIED. ) ;
#16355=CARTESIAN_POINT ( 'NONE',  ( -9.974039711714500100, -14.85049230159630618, 74.93745556479784398 ) ) ;
#16356=EDGE_CURVE ( 'NONE', #25757, #46361, #8475, .T. ) ;
#16359=FACE_OUTER_BOUND ( 'NONE', #48026, .T. ) ;
#16360=CARTESIAN_POINT ( 'NONE',  ( -16.97946044980448121, -21.84517136462328324, 72.31543221430108304 ) ) ;
#16361=CARTESIAN_POINT ( 'NONE',  ( -10.35423477582964225, -12.45965686662758110, 60.90579408580234855 ) ) ;
#16362=CARTESIAN_POINT ( 'NONE',  ( -11.53247254227971652, -18.68106628708273931, 65.04707076447483871 ) ) ;
#16363=ORIENTED_EDGE ( 'NONE', *, *, #30362, .T. ) ;
#16364=CARTESIAN_POINT ( 'NONE',  ( -18.84068548446033731, -21.72355622379298978, 72.44077832767429470 ) ) ;
#16366=CARTESIAN_POINT ( 'NONE',  ( -23.48344415125163565, -18.41350569598871090, 73.04896097104848707 ) ) ;
#16369=CARTESIAN_POINT ( 'NONE',  ( -14.22253886256124389, -8.524026329579788452, 67.46795094879617238 ) ) ;
#16372=EDGE_LOOP ( 'NONE', ( #6384, #40578 ) ) ;
#16373=DIRECTION ( 'NONE',  ( 0.9999889394985580493, 0.004703284017506803583, -7.734398264755851970E-09 ) ) ;
#16374=ORIENTED_EDGE ( 'NONE', *, *, #10445, .F. ) ;
#16376=CARTESIAN_POINT ( 'NONE',  ( -11.37338168604670408, -19.15691247995520996, 71.87341272242258583 ) ) ;
#16377=CARTESIAN_POINT ( 'NONE',  ( -11.99468485875942925, -10.30643380866937697, 64.23734308384325686 ) ) ;
#16378=EDGE_LOOP ( 'NONE', ( #22366, #28883, #3320, #46148, #23890 ) ) ;
#16382=CARTESIAN_POINT ( 'NONE',  ( -20.37299750454370439, -8.405577324698720432, 66.78104082189589974 ) ) ;
#16383=VERTEX_POINT ( 'NONE', #24993 ) ;
#16384=EDGE_CURVE ( 'NONE', #24660, #8287, #28426, .T. ) ;
#16386=ORIENTED_EDGE ( 'NONE', *, *, #17312, .T. ) ;
#16387=FACE_OUTER_BOUND ( 'NONE', #33611, .T. ) ;
#16388=AXIS2_PLACEMENT_3D ( 'NONE', #3095, #22306, #18103 ) ;
#16390=CARTESIAN_POINT ( 'NONE',  ( -14.54749350918766204, -8.372447261038935551, 64.07506791522041567 ) ) ;
#16391=CARTESIAN_POINT ( 'NONE',  ( -21.36284794767689377, -21.13297080501056513, 69.16954792666395235 ) ) ;
#16392=CARTESIAN_POINT ( 'NONE',  ( -13.40431825323822146, -9.078389689080667679, 60.72484859302592497 ) ) ;
#16394=ORIENTED_EDGE ( 'NONE', *, *, #41055, .T. ) ;
#16395=B_SPLINE_CURVE_WITH_KNOTS ( 'NONE', 1,
 ( #45037, #19576 ),
 .UNSPECIFIED., .F., .F.,
 ( 2, 2 ),
 ( 0.000000000000000000, 1.000000000000000000 ),
 .UNSPECIFIED. ) ;
#16397=CARTESIAN_POINT ( 'NONE',  ( -22.52619951119469022, -19.67884242972143483, 69.05929390617204433 ) ) ;
#16398=CARTESIAN_POINT ( 'NONE',  ( -24.87417962317557496, -14.80849170857717567, 59.42795673386487465 ) ) ;
#16402=CARTESIAN_POINT ( 'NONE',  ( -14.77786946956392278, -21.77340987454994092, 61.83589227476007721 ) ) ;
#16403=CARTESIAN_POINT ( 'NONE',  ( -12.15470796376391682, -20.07677110164151557, 61.51023378490003068 ) ) ;
#16404=AXIS2_PLACEMENT_3D ( 'NONE', #11180, #3788, #3042 ) ;
#16405=CARTESIAN_POINT ( 'NONE',  ( -12.48641670427285355, -19.77161270282481098, 65.15058277296205347 ) ) ;
#16410=CARTESIAN_POINT ( 'NONE',  ( -22.89702288877819214, -9.753446293288515534, 73.66816357947271854 ) ) ;
#16413=ADVANCED_FACE ( 'NONE', ( #10466 ), #28204, .T. ) ;
#16414=CARTESIAN_POINT ( 'NONE',  ( -12.20316607747752613, -9.493609027659992705, 57.27590782196710251 ) ) ;
#16415=VERTEX_POINT ( 'NONE', #6031 ) ;
#16417=CARTESIAN_POINT ( 'NONE',  ( -22.91699352949043700, -19.14904340809635741, 59.16794112173154474 ) ) ;
#16420=CARTESIAN_POINT ( 'NONE',  ( -10.01424894596331505, -14.03598936870067782, 61.17467227907766869 ) ) ;
#16421=ORIENTED_EDGE ( 'NONE', *, *, #5511, .T. ) ;
#16422=CARTESIAN_POINT ( 'NONE',  ( -18.72681101482837818, -7.880611649715417499, 70.37068030201731972 ) ) ;
#16423=EDGE_CURVE ( 'NONE', #42703, #45668, #37226, .T. ) ;
#16425=CARTESIAN_POINT ( 'NONE',  ( -14.62647943160224528, -7.904425104641775945, 60.41972663192098025 ) ) ;
#16426=VERTEX_POINT ( 'NONE', #29169 ) ;
#16428=CARTESIAN_POINT ( 'NONE',  ( -10.67632725396948956, -12.73975884439864359, 57.48424594490033002 ) ) ;
#16429=DIRECTION ( 'NONE',  ( -0.9729319276368275649, -0.2310918955413239495, 6.827553174175006206E-08 ) ) ;
#16431=ORIENTED_EDGE ( 'NONE', *, *, #46385, .F. ) ;
#16432=CYLINDRICAL_SURFACE ( 'NONE', #15804, 0.1499999999999971079 ) ;
#16434=CARTESIAN_POINT ( 'NONE',  ( -10.08080428754885105, -16.06609343925254763, 68.23413777636764621 ) ) ;
#16437=CARTESIAN_POINT ( 'NONE',  ( -15.56465948913147557, -7.543361525925789124, 47.99999999999994316 ) ) ;
#16439=ORIENTED_EDGE ( 'NONE', *, *, #37788, .T. ) ;
#16441=CARTESIAN_POINT ( 'NONE',  ( -23.89460186926044472, -11.99007647016461320, 63.09651074612323640 ) ) ;
#16442=CARTESIAN_POINT ( 'NONE',  ( -12.95699726224880699, -8.846094125884357950, 64.02291131566488502 ) ) ;
#16444=CARTESIAN_POINT ( 'NONE',  ( -21.33159362617910659, -4.962723823544877177, 53.49999999999995026 ) ) ;
#16447=CARTESIAN_POINT ( 'NONE',  ( -23.80941655268207668, -18.64734661885979961, 72.80722282987319716 ) ) ;
#16449=AXIS2_PLACEMENT_3D ( 'NONE', #14236, #21179, #40593 ) ;
#16451=CARTESIAN_POINT ( 'NONE',  ( -10.82867469351122836, -11.34449526142513598, 67.73369307302053244 ) ) ;
#16454=B_SPLINE_CURVE_WITH_KNOTS ( 'NONE', 3,
 ( #37836, #38070, #14659, #19365, #26275, #34373, #661, #15661, #42026, #30716 ),
 .UNSPECIFIED., .F., .F.,
 ( 4, 2, 2, 2, 4 ),
 ( 0.000000000000000000, 0.2500000000000000000, 0.5000000000000000000, 0.7500000000000000000, 1.000000000000000000 ),
 .UNSPECIFIED. ) ;
#16455=CARTESIAN_POINT ( 'NONE',  ( -10.99586753834015695, -11.04334891231907534, 60.86381058728009208 ) ) ;
#16456=CARTESIAN_POINT ( 'NONE',  ( -22.01346526549441407, -20.09489739794641849, 58.99116211847115920 ) ) ;
#16457=CARTESIAN_POINT ( 'NONE',  ( -22.45398798615017455, -19.67764645536353996, 72.94400540998888971 ) ) ;
#16458=DIRECTION ( 'NONE',  ( 2.723496474639940985E-06, 1.584719855340916648E-07, 0.9999999999962787545 ) ) ;
#16461=CARTESIAN_POINT ( 'NONE',  ( -22.06352460594304787, -8.980016202103444201, 63.37649054182217867 ) ) ;
#16462=( BOUNDED_CURVE ( )  B_SPLINE_CURVE ( 3, ( #19357, #41046, #34364, #45244 ),
 .UNSPECIFIED., .F., .F. ) 
 B_SPLINE_CURVE_WITH_KNOTS ( ( 4, 4 ),
 ( 0.4074455897393636783, 0.5000000000000000000 ),
 .UNSPECIFIED. ) 
 CURVE ( )  GEOMETRIC_REPRESENTATION_ITEM ( )  RATIONAL_B_SPLINE_CURVE ( ( 0.6983129098260917322, 0.7760317562606919850, 0.8765941196519932976, 0.9999999999999918954 ) ) 
 REPRESENTATION_ITEM ( '' )  );
#16466=EDGE_CURVE ( 'NONE', #22481, #2842, #11747, .T. ) ;
#16467=VERTEX_POINT ( 'NONE', #40262 ) ;
#16469=CARTESIAN_POINT ( 'NONE',  ( -22.68646480449111635, -20.08284195570847430, 69.35913425646373298 ) ) ;
#16470=CARTESIAN_POINT ( 'NONE',  ( -13.85393748347032528, -8.270264590973253505, 74.38449983516251507 ) ) ;
#16471=( BOUNDED_CURVE ( )  B_SPLINE_CURVE ( 3, ( #34176, #22626, #34414, #45056 ),
 .UNSPECIFIED., .F., .F. ) 
 B_SPLINE_CURVE_WITH_KNOTS ( ( 4, 4 ),
 ( 0.5000000000000000000, 0.9074455897393638448 ),
 .UNSPECIFIED. ) 
 CURVE ( )  GEOMETRIC_REPRESENTATION_ITEM ( )  RATIONAL_B_SPLINE_CURVE ( ( 0.9999999999999754641, 0.4567392136813280268, 0.3561768502900458655, 0.6983129098261023904 ) ) 
 REPRESENTATION_ITEM ( '' )  );
#16472=ORIENTED_EDGE ( 'NONE', *, *, #27278, .F. ) ;
#16473=( BOUNDED_CURVE ( )  B_SPLINE_CURVE ( 3, ( #4424, #34454, #24119, #35184 ),
 .UNSPECIFIED., .F., .F. ) 
 B_SPLINE_CURVE_WITH_KNOTS ( ( 4, 4 ),
 ( 0.9074455897393645110, 1.000000000000000000 ),
 .UNSPECIFIED. ) 
 CURVE ( )  GEOMETRIC_REPRESENTATION_ITEM ( )  RATIONAL_B_SPLINE_CURVE ( ( 0.6983129098260982826, 0.7760317562607027542, 0.8765941196520032896, 1.000000000000000000 ) ) 
 REPRESENTATION_ITEM ( '' )  );
#16474=CARTESIAN_POINT ( 'NONE',  ( -10.49080411414803926, -13.84192971499166269, 57.46441715484542812 ) ) ;
#16475=VECTOR ( 'NONE', #28265, 999.9999999999998863 ) ;
#16479=B_SPLINE_CURVE_WITH_KNOTS ( 'NONE', 1,
 ( #31338, #42186 ),
 .UNSPECIFIED., .F., .F.,
 ( 2, 2 ),
 ( 0.000000000000000000, 1.000000000000000000 ),
 .UNSPECIFIED. ) ;
#16480=CARTESIAN_POINT ( 'NONE',  ( -18.67529344402863956, -22.15414776727839907, 72.39855560065855400 ) ) ;
#16481=ORIENTED_EDGE ( 'NONE', *, *, #41189, .F. ) ;
#16482=CARTESIAN_POINT ( 'NONE',  ( -14.27319502748954783, -8.558459675072437989, 70.72957628730870283 ) ) ;
#16483=CARTESIAN_POINT ( 'NONE',  ( -13.04244981547684823, -8.783951787904593189, 64.05946526178860267 ) ) ;
#16484=EDGE_CURVE ( 'NONE', #33892, #16133, #21524, .T. ) ;
#16487=CARTESIAN_POINT ( 'NONE',  ( -11.93102662126159785, -10.47028825497329585, 70.96893105764984000 ) ) ;
#16489=EDGE_CURVE ( 'NONE', #17121, #10137, #48396, .T. ) ;
#16490=CARTESIAN_POINT ( 'NONE',  ( -24.10114582721934084, -12.70328895263707913, 73.47055430460139291 ) ) ;
#16491=CARTESIAN_POINT ( 'NONE',  ( -14.80056043599933524, -21.78207186541723317, 61.82095768364339960 ) ) ;
#16492=EDGE_LOOP ( 'NONE', ( #32620, #12773 ) ) ;
#16493=CARTESIAN_POINT ( 'NONE',  ( -16.13712438557350737, -7.928469192395482423, 60.27316438348749017 ) ) ;
#16494=( BOUNDED_CURVE ( )  B_SPLINE_CURVE ( 3, ( #20982, #18729, #25884, #36943 ),
 .UNSPECIFIED., .F., .F. ) 
 B_SPLINE_CURVE_WITH_KNOTS ( ( 4, 4 ),
 ( 4.712388980384690562, 4.921828490624010399 ),
 .UNSPECIFIED. ) 
 CURVE ( )  GEOMETRIC_REPRESENTATION_ITEM ( )  RATIONAL_B_SPLINE_CURVE ( ( 1.000000000000000000, 0.9963479302455154896, 0.9963479302455154896, 1.000000000000000000 ) ) 
 REPRESENTATION_ITEM ( '' )  );
#16495=FACE_OUTER_BOUND ( 'NONE', #17849, .T. ) ;
#16497=FACE_OUTER_BOUND ( 'NONE', #4175, .T. ) ;
#16500=ORIENTED_EDGE ( 'NONE', *, *, #24197, .T. ) ;
#16501=DIRECTION ( 'NONE',  ( 0.4433615477241707459, -0.8963428685495451465, 2.661652803430218851E-08 ) ) ;
#16502=CARTESIAN_POINT ( 'NONE',  ( -21.48252188606478086, -21.05763224395268196, 69.16794793541382091 ) ) ;
#16504=B_SPLINE_CURVE_WITH_KNOTS ( 'NONE', 3,
 ( #5824, #47181, #24055, #43499, #6048, #43255, #20836, #28702, #25015, #39051 ),
 .UNSPECIFIED., .F., .F.,
 ( 4, 2, 2, 2, 4 ),
 ( 0.000000000000000000, 0.2500000000000000000, 0.5000000000000000000, 0.7500000000000000000, 1.000000000000000000 ),
 .UNSPECIFIED. ) ;
#16505=CARTESIAN_POINT ( 'NONE',  ( -16.07630405233268434, -7.886179812623181462, 67.55496168274575552 ) ) ;
#16506=CARTESIAN_POINT ( 'NONE',  ( -21.81985589881223930, -9.292801929985119003, 59.92991148151821079 ) ) ;
#16507=CARTESIAN_POINT ( 'NONE',  ( -10.29385348138020539, -12.64970417265235803, 64.38340698725603772 ) ) ;
#16508=CARTESIAN_POINT ( 'NONE',  ( -13.07753640729841571, -8.758436312614517050, 64.03229666249436036 ) ) ;
#16510=CARTESIAN_POINT ( 'NONE',  ( -12.22244147144377280, -10.12480163234519281, 60.63206217599131520 ) ) ;
#16512=CARTESIAN_POINT ( 'NONE',  ( -22.73618463404748624, -20.03370227938794912, 69.28762739622011679 ) ) ;
#16513=FACE_OUTER_BOUND ( 'NONE', #18247, .T. ) ;
#16514=CARTESIAN_POINT ( 'NONE',  ( -10.45859239952313224, -15.89938452881993847, 64.79299464097340433 ) ) ;
#16517=LINE ( 'NONE', #31551, #160 ) ;
#16518=VERTEX_POINT ( 'NONE', #33561 ) ;
#16519=ORIENTED_EDGE ( 'NONE', *, *, #7099, .F. ) ;
#16520=ORIENTED_EDGE ( 'NONE', *, *, #43911, .F. ) ;
#16521=CARTESIAN_POINT ( 'NONE',  ( -17.56877512014188625, -7.360533253644350182, 63.59411120999686062 ) ) ;
#16522=DIRECTION ( 'NONE',  ( -5.731567514496413899E-31, -1.020425574103664789E-16, -1.000000000000000000 ) ) ;
#16524=EDGE_CURVE ( 'NONE', #10223, #36492, #43532, .T. ) ;
#16525=ORIENTED_EDGE ( 'NONE', *, *, #9153, .F. ) ;
#16526=CARTESIAN_POINT ( 'NONE',  ( -21.89953879547803695, -8.853196296446007807, 66.70504049802050872 ) ) ;
#16527=CARTESIAN_POINT ( 'NONE',  ( -10.37795889460693033, -14.56696403379599225, 68.14328054657653411 ) ) ;
#16528=ORIENTED_EDGE ( 'NONE', *, *, #27553, .T. ) ;
#16529=CARTESIAN_POINT ( 'NONE',  ( -10.63768371389235767, -17.88312332652141023, 71.68905463271586598 ) ) ;
#16530=CARTESIAN_POINT ( 'NONE',  ( -19.30861700655685098, -22.01699669475148724, 58.78153328179137560 ) ) ;
#16533=CARTESIAN_POINT ( 'NONE',  ( -10.13784000599894597, -13.25541019000276499, 74.79322239981686948 ) ) ;
#16536=CARTESIAN_POINT ( 'NONE',  ( -22.47873160378920687, -20.28232442305464645, 65.82704820931039080 ) ) ;
#16537=CARTESIAN_POINT ( 'NONE',  ( -21.03862266567373851, -20.86632007393060917, 62.32291251243861296 ) ) ;
#16539=CARTESIAN_POINT ( 'NONE',  ( -24.23941684483994408, -17.81830337043964718, 62.58086817458297446 ) ) ;
#16541=EDGE_CURVE ( 'NONE', #7654, #31760, #43813, .T. ) ;
#16542=CARTESIAN_POINT ( 'NONE',  ( -19.11145557798581152, -7.964112677450091660, 63.73089235102099792 ) ) ;
#16544=CARTESIAN_POINT ( 'NONE',  ( -14.72744631621160494, -8.295007313424175521, 60.60524229057013201 ) ) ;
#16545=CARTESIAN_POINT ( 'NONE',  ( -22.23733836534369601, -19.96043719841513564, 65.85421731380807842 ) ) ;
#16546=CARTESIAN_POINT ( 'NONE',  ( -20.57444639489040483, -21.06071912686655168, 58.92858597573613366 ) ) ;
#16550=CARTESIAN_POINT ( 'NONE',  ( -16.58751243259469277, -21.80939447449397051, 65.37564390318223673 ) ) ;
#16551=CARTESIAN_POINT ( 'NONE',  ( -24.86479638606408571, -14.43697995806947176, 66.38303926562055324 ) ) ;
#16552=CARTESIAN_POINT ( 'NONE',  ( -16.39155882215229099, -21.78318466615559146, 61.90568132352964881 ) ) ;
#16553=EDGE_CURVE ( 'NONE', #36936, #16629, #30006, .T. ) ;
#16556=ORIENTED_EDGE ( 'NONE', *, *, #40359, .F. ) ;
#16557=CARTESIAN_POINT ( 'NONE',  ( -13.99679447977218061, -20.97040113148658591, 71.94079819673058296 ) ) ;
#16559=EDGE_LOOP ( 'NONE', ( #32147, #46280, #10871, #32288, #48414 ) ) ;
#16560=CARTESIAN_POINT ( 'NONE',  ( -23.36391615787244191, -18.61340847718015823, 66.03209153377542862 ) ) ;
#16561=CARTESIAN_POINT ( 'NONE',  ( -14.47983125967835960, -7.965589368325148634, 63.90483512601500848 ) ) ;
#16563=CARTESIAN_POINT ( 'NONE',  ( -12.74083618280373642, -20.01189185905951007, 68.35159915988243995 ) ) ;
#16565=EDGE_CURVE ( 'NONE', #48128, #44170, #19638, .T. ) ;
#16566=ORIENTED_EDGE ( 'NONE', *, *, #42600, .F. ) ;
#16567=FACE_OUTER_BOUND ( 'NONE', #32219, .T. ) ;
#16568=CARTESIAN_POINT ( 'NONE',  ( -13.65684165595416921, -8.849801312179289781, 56.98439896120441261 ) ) ;
#16569=CARTESIAN_POINT ( 'NONE',  ( -10.51729459156483237, -16.22293329152201480, 71.59750383216309899 ) ) ;
#16570=ORIENTED_EDGE ( 'NONE', *, *, #40792, .T. ) ;
#16572=FACE_OUTER_BOUND ( 'NONE', #21363, .T. ) ;
#16573=( BOUNDED_CURVE ( )  B_SPLINE_CURVE ( 3, ( #4387, #14454, #29513, #18415 ),
 .UNSPECIFIED., .F., .F. ) 
 B_SPLINE_CURVE_WITH_KNOTS ( ( 4, 4 ),
 ( 0.9074455897393657322, 1.000000000000000000 ),
 .UNSPECIFIED. ) 
 CURVE ( )  GEOMETRIC_REPRESENTATION_ITEM ( )  RATIONAL_B_SPLINE_CURVE ( ( 0.6983129098260912881, 0.7760317562606967590, 0.8765941196519996259, 1.000000000000000000 ) ) 
 REPRESENTATION_ITEM ( '' )  );
#16574=CARTESIAN_POINT ( 'NONE',  ( -13.22164718542227035, -8.657617455897696601, 60.63961484927665424 ) ) ;
#16575=CARTESIAN_POINT ( 'NONE',  ( -17.96636798352247055, -9.322503134287590143, 53.69233794759168887 ) ) ;
#16576=PLANE ( 'NONE',  #26773 ) ;
#16577=CARTESIAN_POINT ( 'NONE',  ( -23.08261055559088248, -18.93003034027461950, 62.65406880913197796 ) ) ;
#16582=CARTESIAN_POINT ( 'NONE',  ( -22.97166404482257107, -9.836574275791852173, 70.21189719861501999 ) ) ;
#16587=B_SPLINE_CURVE_WITH_KNOTS ( 'NONE', 3,
 ( #8217, #41699, #7985, #4272, #38221, #38473, #16295, #34788, #4505, #20253 ),
 .UNSPECIFIED., .F., .F.,
 ( 4, 2, 2, 2, 4 ),
 ( 0.000000000000000000, 0.2500000000000000000, 0.5000000000000000000, 0.7500000000000000000, 1.000000000000000000 ),
 .UNSPECIFIED. ) ;
#16590=ORIENTED_EDGE ( 'NONE', *, *, #38911, .F. ) ;
#16591=DIRECTION ( 'NONE',  ( -0.4408917724886824430, -0.07492959997082740409, 0.8944271909999157444 ) ) ;
#16592=B_SPLINE_CURVE_WITH_KNOTS ( 'NONE', 1,
 ( #47243, #21391 ),
 .UNSPECIFIED., .F., .F.,
 ( 2, 2 ),
 ( 0.000000000000000000, 1.000000000000000000 ),
 .UNSPECIFIED. ) ;
#16593=CARTESIAN_POINT ( 'NONE',  ( -18.19389323530821301, -22.21941482433020809, 65.53027461949925225 ) ) ;
#16595=CARTESIAN_POINT ( 'NONE',  ( -24.14992870231961319, -18.01341063617936911, 59.11883102335588802 ) ) ;
#16602=CARTESIAN_POINT ( 'NONE',  ( -17.77920954038207668, -22.25082405446125122, 58.59048702730397196 ) ) ;
#16604=EDGE_CURVE ( 'NONE', #46504, #7981, #22265, .T. ) ;
#16606=CARTESIAN_POINT ( 'NONE',  ( -20.10190376251898670, -8.341580098330338089, 70.53635029990871885 ) ) ;
#16607=CARTESIAN_POINT ( 'NONE',  ( -24.70870331492811900, -13.24806755967459537, 59.46293686089323671 ) ) ;
#16609=CARTESIAN_POINT ( 'NONE',  ( -18.46649413407774887, -22.18667672369172550, 72.47166315949273496 ) ) ;
#16610=CARTESIAN_POINT ( 'NONE',  ( -22.24652905638778577, -19.95594847178128362, 62.11950460074248781 ) ) ;
#16611=CARTESIAN_POINT ( 'NONE',  ( -23.10667289873031649, -18.98809891091294233, 66.12389717179522108 ) ) ;
#16612=CARTESIAN_POINT ( 'NONE',  ( -10.00761947527410634, -15.51609109068450465, 57.75288224187332276 ) ) ;
#16613=EDGE_CURVE ( 'NONE', #34949, #28014, #20239, .T. ) ;
#16614=CARTESIAN_POINT ( 'NONE',  ( -22.09029313690021112, -20.02728107436852767, 62.53439146813792604 ) ) ;
#16615=FACE_OUTER_BOUND ( 'NONE', #33978, .T. ) ;
#16617=CARTESIAN_POINT ( 'NONE',  ( -24.50530043060364349, -7.885727737951715888, 53.49999999999995026 ) ) ;
#16618=ORIENTED_EDGE ( 'NONE', *, *, #5457, .T. ) ;
#16619=CARTESIAN_POINT ( 'NONE',  ( -15.47038549838128674, -21.58309193914155344, 72.19575460769013375 ) ) ;
#16620=EDGE_CURVE ( 'NONE', #10403, #20439, #40820, .T. ) ;
#16621=ORIENTED_EDGE ( 'NONE', *, *, #14290, .F. ) ;
#16622=CARTESIAN_POINT ( 'NONE',  ( -11.41497442304007670, -19.21309820834011362, 71.80190602235010999 ) ) ;
#16623=CARTESIAN_POINT ( 'NONE',  ( -20.81921389985186721, -21.44071754855728784, 58.75979745677555854 ) ) ;
#16624=( BOUNDED_SURFACE ( )  B_SPLINE_SURFACE ( 3, 1, ( 
 ( #44156, #3985 ),
 ( #22702, #40908 ),
 ( #10873, #25414 ),
 ( #21957, #22205 ),
 ( #36953, #48535 ),
 ( #18245, #17999 ),
 ( #48058, #33254 ) ),
 .UNSPECIFIED., .T., .F., .F. ) 
 B_SPLINE_SURFACE_WITH_KNOTS ( ( 4, 3, 4 ),
 ( 2, 2 ),
 ( 0.000000000000000000, 0.5000000000000000000, 1.000000000000000000 ),
 ( 0.000000000000000000, 1.000000000000000000 ),
 .UNSPECIFIED. ) 
 GEOMETRIC_REPRESENTATION_ITEM ( )  RATIONAL_B_SPLINE_SURFACE ( (
 ( 1.000000000000000000, 1.000000000000000000),
 ( 0.3333333333333335369, 0.3333333333333330373),
 ( 0.3333333333333335369, 0.3333333333333330373),
 ( 1.000000000000000000, 1.000000000000000000),
 ( 0.3333333333333333703, 0.3333333333333333703),
 ( 0.3333333333333333703, 0.3333333333333333703),
 ( 1.000000000000000000, 1.000000000000000000) ) ) 
 REPRESENTATION_ITEM ( '' )  SURFACE ( )  );
#16625=ORIENTED_EDGE ( 'NONE', *, *, #10435, .F. ) ;
#16626=LINE ( 'NONE', #36060, #44458 ) ;
#16627=FACE_BOUND ( 'NONE', #36276, .T. ) ;
#16629=VERTEX_POINT ( 'NONE', #27414 ) ;
#16632=VECTOR ( 'NONE', #32109, 1000.000000000000114 ) ;
#16635=EDGE_CURVE ( 'NONE', #23522, #44556, #6418, .T. ) ;
#16636=CARTESIAN_POINT ( 'NONE',  ( -11.97490362423377164, -10.33561459433851404, 67.78424783647008667 ) ) ;
#16637=( BOUNDED_SURFACE ( )  B_SPLINE_SURFACE ( 3, 1, ( 
 ( #10269, #1224 ),
 ( #31040, #42364 ),
 ( #46054, #25284 ),
 ( #27335, #8637 ),
 ( #27580, #23660 ),
 ( #34956, #16229 ),
 ( #31271, #12558 ) ),
 .UNSPECIFIED., .T., .F., .F. ) 
 B_SPLINE_SURFACE_WITH_KNOTS ( ( 4, 3, 4 ),
 ( 2, 2 ),
 ( 0.000000000000000000, 0.5000000000000000000, 1.000000000000000000 ),
 ( 0.000000000000000000, 1.000000000000000000 ),
 .UNSPECIFIED. ) 
 GEOMETRIC_REPRESENTATION_ITEM ( )  RATIONAL_B_SPLINE_SURFACE ( (
 ( 1.000000000000000000, 1.000000000000000000),
 ( 0.3333333333333335369, 0.3333333333333330373),
 ( 0.3333333333333335369, 0.3333333333333330373),
 ( 1.000000000000000000, 1.000000000000000000),
 ( 0.3333333333333333703, 0.3333333333333333703),
 ( 0.3333333333333333703, 0.3333333333333333703),
 ( 1.000000000000000000, 1.000000000000000000) ) ) 
 REPRESENTATION_ITEM ( '' )  SURFACE ( )  );
#16638=EDGE_CURVE ( 'NONE', #32429, #15048, #6113, .T. ) ;
#16643=AXIS2_PLACEMENT_3D ( 'NONE', #14824, #18795, #25462 ) ;
#16646=CYLINDRICAL_SURFACE ( 'NONE', #43353, 0.1500000000000063227 ) ;
#16648=ORIENTED_EDGE ( 'NONE', *, *, #39002, .T. ) ;
#16650=CARTESIAN_POINT ( 'NONE',  ( -23.00381842360518547, -10.58230771189866104, 59.90203429537245228 ) ) ;
#16651=CARTESIAN_POINT ( 'NONE',  ( -17.42409385541300892, -14.80920654474439324, 53.49899999999994549 ) ) ;
#16652=VECTOR ( 'NONE', #35230, 1000.000000000000114 ) ;
#16653=CARTESIAN_POINT ( 'NONE',  ( -24.48565114283276500, -17.18359061586099301, 73.07610194155731165 ) ) ;
#16654=B_SPLINE_CURVE_WITH_KNOTS ( 'NONE', 3,
 ( #5192, #8648, #42379, #46794, #42860, #35211, #1483, #23671, #38672, #20695 ),
 .UNSPECIFIED., .F., .F.,
 ( 4, 2, 2, 2, 4 ),
 ( 0.6272669072782514066, 0.7522669073001546636, 0.8772669073220578095, 1.002266907343960956, 1.127266907365864324 ),
 .UNSPECIFIED. ) ;
#16656=CARTESIAN_POINT ( 'NONE',  ( -17.33262245845742910, -7.759502110702281463, 67.30567542699309058 ) ) ;
#16657=CARTESIAN_POINT ( 'NONE',  ( -10.98115068093432356, -12.07269720428386961, 74.74943597065113465 ) ) ;
#16658=FACE_OUTER_BOUND ( 'NONE', #15475, .T. ) ;
#16659=EDGE_LOOP ( 'NONE', ( #38553, #42660, #24733, #25175, #26859 ) ) ;
#16660=CARTESIAN_POINT ( 'NONE',  ( -10.57990114081760957, -13.11695186304740979, 71.22300718686658172 ) ) ;
#16661=CARTESIAN_POINT ( 'NONE',  ( -17.33262245845742910, -7.759502110702281463, 67.30567542699309058 ) ) ;
#16662=CARTESIAN_POINT ( 'NONE',  ( -11.42760935163198965, -18.42145026959589060, 61.29327518568021560 ) ) ;
#16663=VERTEX_POINT ( 'NONE', #31604 ) ;
#16664=CARTESIAN_POINT ( 'NONE',  ( -10.41531639268335496, -14.04517892474411589, 60.93293405735092705 ) ) ;
#16665=EDGE_LOOP ( 'NONE', ( #36508, #13031 ) ) ;
#16667=CARTESIAN_POINT ( 'NONE',  ( -14.59772110827021763, -7.916021557401901276, 60.49713200689404857 ) ) ;
#16671=CARTESIAN_POINT ( 'NONE',  ( -10.40127108354264429, -12.32249413655887871, 57.51352655450988749 ) ) ;
#16673=EDGE_LOOP ( 'NONE', ( #2080, #16150, #869, #36424, #25478 ) ) ;
#16674=CARTESIAN_POINT ( 'NONE',  ( -10.76763519559319882, -17.13171766695033327, 61.15743118826002700 ) ) ;
#16676=CARTESIAN_POINT ( 'NONE',  ( -23.88415217903648724, -17.63235132829416685, 62.77360984996716553 ) ) ;
#16678=CARTESIAN_POINT ( 'NONE',  ( -10.39215600595210631, -14.30487551902977827, 64.38803863383273551 ) ) ;
#16682=CARTESIAN_POINT ( 'NONE',  ( -14.11063322135152909, -21.03236308526469855, 72.21135587486895702 ) ) ;
#16686=CARTESIAN_POINT ( 'NONE',  ( -18.72681101482837818, -7.880611649715417499, 70.37068030201731972 ) ) ;
#16688=CARTESIAN_POINT ( 'NONE',  ( -10.40127070788197017, -12.32249518151173895, 57.51352764219546998 ) ) ;
#16690=CARTESIAN_POINT ( 'NONE',  ( -23.34288328645119037, -19.33377384263253873, 59.06905932422779415 ) ) ;
#16691=ORIENTED_EDGE ( 'NONE', *, *, #1216, .F. ) ;
#16692=ORIENTED_EDGE ( 'NONE', *, *, #26456, .T. ) ;
#16693=CARTESIAN_POINT ( 'NONE',  ( -23.03538909537400770, -9.907469116741831172, 70.19833813022523827 ) ) ;
#16694=EDGE_CURVE ( 'NONE', #2787, #34596, #40068, .T. ) ;
#16698=CARTESIAN_POINT ( 'NONE',  ( -19.29727288544221864, -21.61407024248036635, 65.60919142207177401 ) ) ;
#16701=B_SPLINE_CURVE_WITH_KNOTS ( 'NONE', 3,
 ( #22172, #17720, #47774, #10595, #14013, #6425, #10365, #25604, #21449, #40616 ),
 .UNSPECIFIED., .F., .F.,
 ( 4, 2, 2, 2, 4 ),
 ( 0.000000000000000000, 0.2500000000000000000, 0.5000000000000000000, 0.7500000000000000000, 1.000000000000000000 ),
 .UNSPECIFIED. ) ;
#16702=ORIENTED_EDGE ( 'NONE', *, *, #47095, .F. ) ;
#16703=CARTESIAN_POINT ( 'NONE',  ( -22.93812568863854295, -10.41619827269718890, 63.07186016945863827 ) ) ;
#16705=CARTESIAN_POINT ( 'NONE',  ( -22.10219206297270489, -9.524287713326932803, 63.33586711951718229 ) ) ;
#16706=CARTESIAN_POINT ( 'NONE',  ( -11.05958060454627656, -18.68192940480324182, 61.41677500004188062 ) ) ;
#16707=VERTEX_POINT ( 'NONE', #5023 ) ;
#16708=CARTESIAN_POINT ( 'NONE',  ( -22.53655473247544805, -20.22829521909097394, 65.88917159596024931 ) ) ;
#16709=CARTESIAN_POINT ( 'NONE',  ( -24.39763799706551950, -15.84669482609578317, 69.54779622430707775 ) ) ;
#16710=ADVANCED_FACE ( 'NONE', ( #1072 ), #13589, .T. ) ;
#16711=CARTESIAN_POINT ( 'NONE',  ( -10.12326218194131044, -13.32541594658350448, 74.86312942357149325 ) ) ;
#16712=CARTESIAN_POINT ( 'NONE',  ( -12.83007281553047108, -20.09077549419061626, 71.80653676829817300 ) ) ;
#16713=CARTESIAN_POINT ( 'NONE',  ( -24.24305685102723018, -16.39138408180526696, 59.42332478927817618 ) ) ;
#16715=CARTESIAN_POINT ( 'NONE',  ( -20.30329177529516116, -7.937872566059631652, 70.41133733428102914 ) ) ;
#16716=ORIENTED_EDGE ( 'NONE', *, *, #26663, .F. ) ;
#16717=CARTESIAN_POINT ( 'NONE',  ( -19.24869282864567310, -7.585968669060765279, 63.60902014247216130 ) ) ;
#16718=CARTESIAN_POINT ( 'NONE',  ( -11.93102524044397938, -10.47028995287008257, 71.26893105764186487 ) ) ;
#16719=EDGE_LOOP ( 'NONE', ( #44324, #143 ) ) ;
#16720=CARTESIAN_POINT ( 'NONE',  ( -18.25923033419348940, -22.21300364388852344, 69.00170051292239748 ) ) ;
#16722=VERTEX_POINT ( 'NONE', #25183 ) ;
#16723=CARTESIAN_POINT ( 'NONE',  ( -17.93803645886973541, -7.826487636815978810, 60.19133818497105182 ) ) ;
#16724=CARTESIAN_POINT ( 'NONE',  ( -14.86477050248655551, -7.812526586475418533, 57.10645908473438226 ) ) ;
#16726=VERTEX_POINT ( 'NONE', #28865 ) ;
#16727=DIRECTION ( 'NONE',  ( -0.7300417127692488961, -0.6834025882427879894, -6.612978995310452690E-09 ) ) ;
#16729=LINE ( 'NONE', #43352, #22733 ) ;
#16730=B_SPLINE_CURVE_WITH_KNOTS ( 'NONE', 3,
 ( #34754, #8188, #27368, #23204, #26401, #22717, #34990, #19983, #31306, #16026 ),
 .UNSPECIFIED., .F., .F.,
 ( 4, 2, 2, 2, 4 ),
 ( 0.000000000000000000, 0.2500000000000000000, 0.5000000000000000000, 0.7500000000000000000, 1.000000000000000000 ),
 .UNSPECIFIED. ) ;
#16731=DIRECTION ( 'NONE',  ( 0.2573866790907599622, 0.9663084897829604669, 6.714855467380901661E-08 ) ) ;
#16732=VECTOR ( 'NONE', #23456, 1000.000000000000227 ) ;
#16733=ORIENTED_EDGE ( 'NONE', *, *, #9103, .T. ) ;
#16734=ORIENTED_EDGE ( 'NONE', *, *, #38791, .F. ) ;
#16735=CYLINDRICAL_SURFACE ( 'NONE', #14883, 0.1500000000000045464 ) ;
#16736=CYLINDRICAL_SURFACE ( 'NONE', #36755, 0.1500000000000002165 ) ;
#16737=VERTEX_POINT ( 'NONE', #32085 ) ;
#16738=CARTESIAN_POINT ( 'NONE',  ( -15.75283698213507755, -7.548994588147243334, 67.32502552484606895 ) ) ;
#16741=CARTESIAN_POINT ( 'NONE',  ( -13.07136655094769750, -8.762923122256669473, 64.02451139116674028 ) ) ;
#16743=DIRECTION ( 'NONE',  ( 0.2573866790907599622, 0.9663084897829604669, 6.714855467380901661E-08 ) ) ;
#16744=EDGE_LOOP ( 'NONE', ( #27875, #27550 ) ) ;
#16746=EDGE_CURVE ( 'NONE', #32101, #35582, #36581, .T. ) ;
#16747=CARTESIAN_POINT ( 'NONE',  ( -18.91168463870544869, -7.914867951563272719, 63.31600393140114136 ) ) ;
#16750=CARTESIAN_POINT ( 'NONE',  ( -13.46392434612064015, -20.58285101795483030, 61.58816697997369261 ) ) ;
#16751=( BOUNDED_CURVE ( )  B_SPLINE_CURVE ( 3, ( #38749, #45909, #46142, #46871 ),
 .UNSPECIFIED., .F., .F. ) 
 B_SPLINE_CURVE_WITH_KNOTS ( ( 4, 4 ),
 ( 0.4074455897393658432, 0.5000000000000000000 ),
 .UNSPECIFIED. ) 
 CURVE ( )  GEOMETRIC_REPRESENTATION_ITEM ( )  RATIONAL_B_SPLINE_CURVE ( ( 0.6983129098260896228, 0.7760317562606886543, 0.8765941196519900780, 0.9999999999999894529 ) ) 
 REPRESENTATION_ITEM ( '' )  );
#16752=ORIENTED_EDGE ( 'NONE', *, *, #31105, .F. ) ;
#16759=ADVANCED_FACE ( 'NONE', ( #13104 ), #23701, .T. ) ;
#16760=CARTESIAN_POINT ( 'NONE',  ( -21.77717176493317552, -9.327196854410527038, 63.49153729606454988 ) ) ;
#16761=ADVANCED_FACE ( 'NONE', ( #21249 ), #2039, .T. ) ;
#16762=( BOUNDED_CURVE ( )  B_SPLINE_CURVE ( 3, ( #12432, #16104, #46175, #35323 ),
 .UNSPECIFIED., .F., .F. ) 
 B_SPLINE_CURVE_WITH_KNOTS ( ( 4, 4 ),
 ( 0.4074455897393719495, 0.5000000000000000000 ),
 .UNSPECIFIED. ) 
 CURVE ( )  GEOMETRIC_REPRESENTATION_ITEM ( )  RATIONAL_B_SPLINE_CURVE ( ( 0.6983129098261073864, 0.7760317562607119690, 0.8765941196520098400, 1.000000000000002220 ) ) 
 REPRESENTATION_ITEM ( '' )  );
#16763=VERTEX_POINT ( 'NONE', #13345 ) ;
#16764=( BOUNDED_CURVE ( )  B_SPLINE_CURVE ( 3, ( #22927, #7663, #33467, #48267 ),
 .UNSPECIFIED., .F., .F. ) 
 B_SPLINE_CURVE_WITH_KNOTS ( ( 4, 4 ),
 ( 0.5000000000000000000, 0.9074455897393621795 ),
 .UNSPECIFIED. ) 
 CURVE ( )  GEOMETRIC_REPRESENTATION_ITEM ( )  RATIONAL_B_SPLINE_CURVE ( ( 0.9999999999999985567, 0.4567392136813397396, 0.3561768502900340971, 0.6983129098260800749 ) ) 
 REPRESENTATION_ITEM ( '' )  );
#16765=CARTESIAN_POINT ( 'NONE',  ( -21.95395705827280963, -8.894478678276469097, 66.91795930326043162 ) ) ;
#16766=CARTESIAN_POINT ( 'NONE',  ( -10.00747521095153303, -15.51449648374953050, 57.61146884931378054 ) ) ;
#16767=EDGE_CURVE ( 'NONE', #24011, #1356, #33412, .T. ) ;
#16769=EDGE_LOOP ( 'NONE', ( #41693, #26030, #36175, #3975, #23226 ) ) ;
#16771=CARTESIAN_POINT ( 'NONE',  ( -23.08280660609100110, -10.60377317445056811, 59.61675562601556067 ) ) ;
#16773=CARTESIAN_POINT ( 'NONE',  ( -16.78411710364782650, -21.83009890335197767, 68.99560651669348488 ) ) ;
#16776=( BOUNDED_CURVE ( )  B_SPLINE_CURVE ( 3, ( #42559, #4630, #42060, #12255 ),
 .UNSPECIFIED., .F., .F. ) 
 B_SPLINE_CURVE_WITH_KNOTS ( ( 4, 4 ),
 ( 0.4074455897393595705, 0.5000000000000000000 ),
 .UNSPECIFIED. ) 
 CURVE ( )  GEOMETRIC_REPRESENTATION_ITEM ( )  RATIONAL_B_SPLINE_CURVE ( ( 0.6983129098260714152, 0.7760317562606651176, 0.8765941196519704270, 0.9999999999999770184 ) ) 
 REPRESENTATION_ITEM ( '' )  );
#16778=CARTESIAN_POINT ( 'NONE',  ( -16.39815193125092208, -7.826197509823805909, 63.81444203941759952 ) ) ;
#16779=CARTESIAN_POINT ( 'NONE',  ( -23.30963478160716562, -18.69084381296369557, 69.30844128244088154 ) ) ;
#16781=ORIENTED_EDGE ( 'NONE', *, *, #43383, .T. ) ;
#16784=CARTESIAN_POINT ( 'NONE',  ( -22.22496508270376481, -20.50616197626463233, 58.80796965402809917 ) ) ;
#16785=CARTESIAN_POINT ( 'NONE',  ( -19.28939690137687535, -8.062307696266060475, 59.96092997387292201 ) ) ;
#16787=CARTESIAN_POINT ( 'NONE',  ( -10.39404051354841485, -17.27517550453656625, 61.25719493627910595 ) ) ;
#16789=CARTESIAN_POINT ( 'NONE',  ( -24.40914445986810577, -13.82741747260119958, 73.12271364670142759 ) ) ;
#16791=CARTESIAN_POINT ( 'NONE',  ( -17.42409385541300892, -14.80920654474439679, 56.49999999999994316 ) ) ;
#16792=CARTESIAN_POINT ( 'NONE',  ( -15.20917060265737675, -21.92251279605420322, 68.73626286540100239 ) ) ;
#16793=B_SPLINE_CURVE_WITH_KNOTS ( 'NONE', 1,
 ( #29531, #25836 ),
 .UNSPECIFIED., .F., .F.,
 ( 2, 2 ),
 ( 0.000000000000000000, 1.000000000000000000 ),
 .UNSPECIFIED. ) ;
#16796=VERTEX_POINT ( 'NONE', #2529 ) ;
#16797=CARTESIAN_POINT ( 'NONE',  ( -24.46809763383182101, -15.25302497427750303, 73.15870697135122214 ) ) ;
#16798=ORIENTED_EDGE ( 'NONE', *, *, #31717, .T. ) ;
#16799=CARTESIAN_POINT ( 'NONE',  ( -10.37599212182869124, -14.63324797960940771, 71.34254748307667171 ) ) ;
#16800=CARTESIAN_POINT ( 'NONE',  ( -16.78865592400587659, -21.78030535593112305, 68.99560651886281448 ) ) ;
#16801=CARTESIAN_POINT ( 'NONE',  ( -14.55629311593335373, -8.423554203384631123, 63.80481326471479520 ) ) ;
#16802=CARTESIAN_POINT ( 'NONE',  ( -19.51114651407244338, -7.656733154341000436, 60.14748342315007790 ) ) ;
#16803=FACE_OUTER_BOUND ( 'NONE', #12212, .T. ) ;
#16804=ADVANCED_FACE ( 'NONE', ( #20998 ), #48542, .T. ) ;
#16805=ORIENTED_EDGE ( 'NONE', *, *, #33351, .T. ) ;
#16807=CARTESIAN_POINT ( 'NONE',  ( -17.33887285826562774, -7.751749031259347333, 74.10451155337131013 ) ) ;
#16808=CARTESIAN_POINT ( 'NONE',  ( -12.00862336911722927, -9.692924116444773475, 60.81563991731260188 ) ) ;
#16809=ADVANCED_FACE ( 'NONE', ( #33022 ), #3484, .T. ) ;
#16815=CARTESIAN_POINT ( 'NONE',  ( -16.39156059917436181, -21.78318494029796781, 62.05568132351888266 ) ) ;
#16816=ORIENTED_EDGE ( 'NONE', *, *, #42418, .F. ) ;
#16817=EDGE_LOOP ( 'NONE', ( #17816, #14498, #18071, #25573, #31370 ) ) ;
#16819=CARTESIAN_POINT ( 'NONE',  ( -13.30711168077662521, -9.147894172712071281, 64.20946529582356277 ) ) ;
#16820=EDGE_CURVE ( 'NONE', #24042, #15944, #41656, .T. ) ;
#16821=EDGE_CURVE ( 'NONE', #30534, #44919, #18328, .T. ) ;
#16822=CARTESIAN_POINT ( 'NONE',  ( -24.60655895611017741, -12.83064783748087301, 66.45246738850991619 ) ) ;
#16823=EDGE_CURVE ( 'NONE', #16518, #31075, #16124, .T. ) ;
#16824=CARTESIAN_POINT ( 'NONE',  ( -10.78978130820344994, -12.42417047965500743, 57.62857332104950814 ) ) ;
#16825=CARTESIAN_POINT ( 'NONE',  ( -24.34502428176253019, -17.56683243011407924, 66.12852677468319484 ) ) ;
#16828=CARTESIAN_POINT ( 'NONE',  ( -24.36966136476852540, -17.50601128794927774, 69.59995046513768102 ) ) ;
#16829=EDGE_CURVE ( 'NONE', #20668, #23498, #30812, .T. ) ;
#16831=CARTESIAN_POINT ( 'NONE',  ( -21.28537490900993134, -20.64804638814173288, 72.82446480614137840 ) ) ;
#16832=CARTESIAN_POINT ( 'NONE',  ( -12.96069338448818087, -9.414713290161156323, 74.42996161600342475 ) ) ;
#16834=EDGE_LOOP ( 'NONE', ( #21556, #1098, #18072, #43368 ) ) ;
#16835=CARTESIAN_POINT ( 'NONE',  ( -11.39216336840796373, -18.45920852072106300, 61.29182966166492719 ) ) ;
#16836=CARTESIAN_POINT ( 'NONE',  ( -12.24245772170515956, -19.51581775654790718, 58.22682380653618139 ) ) ;
#16838=CARTESIAN_POINT ( 'NONE',  ( -17.63792724537347212, -22.25688666393347859, 58.59208636575791473 ) ) ;
#16840=AXIS2_PLACEMENT_3D ( 'NONE', #11355, #8165, #30332 ) ;
#16841=CARTESIAN_POINT ( 'NONE',  ( -10.00889297783421128, -15.53016721190119753, 57.70646298183843470 ) ) ;
#16843=DIRECTION ( 'NONE',  ( -0.8858372764600287441, -0.4639960340712824260, 4.734734194490170989E-17 ) ) ;
#16844=EDGE_LOOP ( 'NONE', ( #20543, #45537, #37870, #44540 ) ) ;
#16845=B_SPLINE_CURVE_WITH_KNOTS ( 'NONE', 3,
 ( #12697, #42747, #39035, #42016, #648, #26758, #41777, #30941, #45952, #8062 ),
 .UNSPECIFIED., .F., .F.,
 ( 4, 2, 2, 2, 4 ),
 ( 0.000000000000000000, 0.2500000000000000000, 0.5000000000000000000, 0.7500000000000000000, 1.000000000000000000 ),
 .UNSPECIFIED. ) ;
#16846=CARTESIAN_POINT ( 'NONE',  ( -10.31252162633752079, -12.58677457285831913, 60.91198276946202128 ) ) ;
#16849=CARTESIAN_POINT ( 'NONE',  ( -11.86614749421525339, -19.77135288044581429, 58.11337654531251218 ) ) ;
#16851=CARTESIAN_POINT ( 'NONE',  ( -17.29025345054776963, -7.359659516233258536, 67.13384346071842401 ) ) ;
#16852=CARTESIAN_POINT ( 'NONE',  ( -10.50893933415051507, -13.43540278197273885, 74.96345540680638919 ) ) ;
#16854=DIRECTION ( 'NONE',  ( -0.2075053346947394739, 0.3961584734335801827, 0.8944271909999157444 ) ) ;
#16855=( BOUNDED_CURVE ( )  B_SPLINE_CURVE ( 3, ( #48642, #44246, #163, #19097 ),
 .UNSPECIFIED., .F., .F. ) 
 B_SPLINE_CURVE_WITH_KNOTS ( ( 4, 4 ),
 ( 0.9074455897393670645, 1.000000000000000000 ),
 .UNSPECIFIED. ) 
 CURVE ( )  GEOMETRIC_REPRESENTATION_ITEM ( )  RATIONAL_B_SPLINE_CURVE ( ( 0.6983129098260884016, 0.7760317562606942055, 0.8765941196519980716, 1.000000000000000000 ) ) 
 REPRESENTATION_ITEM ( '' )  );
#16856=CARTESIAN_POINT ( 'NONE',  ( -18.50932031946840439, -21.77517977232111690, 72.43510940650374152 ) ) ;
#16858=EDGE_CURVE ( 'NONE', #21561, #20725, #22599, .T. ) ;
#16862=ORIENTED_EDGE ( 'NONE', *, *, #8009, .T. ) ;
#16864=CARTESIAN_POINT ( 'NONE',  ( -19.04853579327176760, -7.948602568230340282, 63.71617106789811658 ) ) ;
#16865=CARTESIAN_POINT ( 'NONE',  ( -23.91439695282944200, -17.43141281116713515, 66.24357239631997629 ) ) ;
#16866=CARTESIAN_POINT ( 'NONE',  ( -22.66727051383977809, -10.09628829486277546, 70.31178520457007153 ) ) ;
#16867=CARTESIAN_POINT ( 'NONE',  ( -22.48430581236326731, -20.27711595259535571, 65.81926302645771898 ) ) ;
#16868=CARTESIAN_POINT ( 'NONE',  ( -16.36080021583335409, -22.18299097935824093, 61.94842262253246901 ) ) ;
#16870=ORIENTED_EDGE ( 'NONE', *, *, #7685, .F. ) ;
#16874=CARTESIAN_POINT ( 'NONE',  ( -21.17484060445739757, -20.78220707328100403, 72.93935319279944451 ) ) ;
#16875=CARTESIAN_POINT ( 'NONE',  ( -20.70759918696101920, -21.04805149802216846, 58.93915383139984954 ) ) ;
#16877=EDGE_CURVE ( 'NONE', #40684, #32966, #28703, .T. ) ;
#16879=EDGE_LOOP ( 'NONE', ( #7364, #37036, #1396, #42993, #16327 ) ) ;
#16880=EDGE_CURVE ( 'NONE', #27231, #45924, #26708, .T. ) ;
#16881=CARTESIAN_POINT ( 'NONE',  ( -14.72055112114360753, -21.75152931705752479, 61.79746922803622766 ) ) ;
#16883=CARTESIAN_POINT ( 'NONE',  ( -12.54253407177667512, -19.82621502378690082, 65.16674886820000268 ) ) ;
#16884=EDGE_CURVE ( 'NONE', #23498, #16178, #6727, .T. ) ;
#16886=CARTESIAN_POINT ( 'NONE',  ( -10.81230840161673967, -17.25685697075765646, 64.64211442681141762 ) ) ;
#16887=CARTESIAN_POINT ( 'NONE',  ( -10.40174226954351866, -17.29724918936392442, 61.34238429002267878 ) ) ;
#16888=CARTESIAN_POINT ( 'NONE',  ( -16.35448746628295424, -21.72700549332279607, 58.39471472850929956 ) ) ;
#16889=CARTESIAN_POINT ( 'NONE',  ( -14.40132536252195194, -7.999811592943899541, 63.92832360672956327 ) ) ;
#16890=ORIENTED_EDGE ( 'NONE', *, *, #14764, .T. ) ;
#16892=( BOUNDED_SURFACE ( )  B_SPLINE_SURFACE ( 3, 1, ( 
 ( #24817, #9319 ),
 ( #32447, #39348 ),
 ( #12764, #47224 ),
 ( #28268, #20148 ),
 ( #16441, #32208 ),
 ( #35404, #20643 ),
 ( #5636, #13218 ) ),
 .UNSPECIFIED., .T., .F., .F. ) 
 B_SPLINE_SURFACE_WITH_KNOTS ( ( 4, 3, 4 ),
 ( 2, 2 ),
 ( 0.000000000000000000, 0.5000000000000000000, 1.000000000000000000 ),
 ( 0.000000000000000000, 1.000000000000000000 ),
 .UNSPECIFIED. ) 
 GEOMETRIC_REPRESENTATION_ITEM ( )  RATIONAL_B_SPLINE_SURFACE ( (
 ( 1.000000000000000000, 1.000000000000000000),
 ( 0.3333333333333335369, 0.3333333333333330373),
 ( 0.3333333333333335369, 0.3333333333333330373),
 ( 1.000000000000000000, 1.000000000000000000),
 ( 0.3333333333333333703, 0.3333333333333333703),
 ( 0.3333333333333333703, 0.3333333333333333703),
 ( 1.000000000000000000, 1.000000000000000000) ) ) 
 REPRESENTATION_ITEM ( '' )  SURFACE ( )  );
#16894=CARTESIAN_POINT ( 'NONE',  ( -22.85827772906650424, -10.39656997657325910, 63.07185958088085442 ) ) ;
#16895=CARTESIAN_POINT ( 'NONE',  ( -18.03604899883812607, -21.78284559735032033, 65.62915604077223009 ) ) ;
#16896=EDGE_LOOP ( 'NONE', ( #13920, #25271, #2326, #17951, #40905 ) ) ;
#16898=EDGE_CURVE ( 'NONE', #26785, #7468, #3250, .T. ) ;
#16899=ORIENTED_EDGE ( 'NONE', *, *, #37152, .F. ) ;
#16901=CARTESIAN_POINT ( 'NONE',  ( -14.92957465851463006, -21.82926012297162899, 65.22101360901100975 ) ) ;
#16902=CARTESIAN_POINT ( 'NONE',  ( -16.32142960126235209, -21.72225670208395343, 62.03951630124149119 ) ) ;
#16903=ORIENTED_EDGE ( 'NONE', *, *, #17450, .T. ) ;
#16905=CARTESIAN_POINT ( 'NONE',  ( -10.60402983012795808, -16.62626367578652520, 57.83193508283319773 ) ) ;
#16906=CARTESIAN_POINT ( 'NONE',  ( -21.79520159808653190, -20.27875113210311753, 58.87516014074775228 ) ) ;
#16907=AXIS2_PLACEMENT_3D ( 'NONE', #24765, #39766, #27955 ) ;
#16908=CARTESIAN_POINT ( 'NONE',  ( -13.18494979104506015, -8.682762004662409439, 60.48304321394137162 ) ) ;
#16909=PLANE ( 'NONE',  #32930 ) ;
#16910=ORIENTED_EDGE ( 'NONE', *, *, #38312, .T. ) ;
#16912=ADVANCED_FACE ( 'NONE', ( #16572 ), #31361, .T. ) ;
#16914=CARTESIAN_POINT ( 'NONE',  ( -10.09291371782238045, -16.13494220690481384, 68.16263107114907882 ) ) ;
#16915=EDGE_LOOP ( 'NONE', ( #9437, #48384 ) ) ;
#16916=CARTESIAN_POINT ( 'NONE',  ( -11.42622260759249464, -18.51434353338492400, 61.57710833179551457 ) ) ;
#16917=( BOUNDED_SURFACE ( )  B_SPLINE_SURFACE ( 3, 1, ( 
 ( #40002, #39517 ),
 ( #2576, #24519 ),
 ( #12919, #32610 ),
 ( #13867, #13636 ),
 ( #36293, #5304 ),
 ( #24266, #20320 ),
 ( #31888, #43709 ) ),
 .UNSPECIFIED., .T., .F., .F. ) 
 B_SPLINE_SURFACE_WITH_KNOTS ( ( 4, 3, 4 ),
 ( 2, 2 ),
 ( 0.000000000000000000, 0.5000000000000000000, 1.000000000000000000 ),
 ( 0.000000000000000000, 1.000000000000000000 ),
 .UNSPECIFIED. ) 
 GEOMETRIC_REPRESENTATION_ITEM ( )  RATIONAL_B_SPLINE_SURFACE ( (
 ( 1.000000000000000000, 1.000000000000000000),
 ( 0.3333333333333335369, 0.3333333333333330373),
 ( 0.3333333333333335369, 0.3333333333333330373),
 ( 1.000000000000000000, 1.000000000000000000),
 ( 0.3333333333333333703, 0.3333333333333333703),
 ( 0.3333333333333333703, 0.3333333333333333703),
 ( 1.000000000000000000, 1.000000000000000000) ) ) 
 REPRESENTATION_ITEM ( '' )  SURFACE ( )  );
#16918=CARTESIAN_POINT ( 'NONE',  ( -11.06712688165958269, -18.69414528815109477, 61.39215548186584215 ) ) ;
#16919=ORIENTED_EDGE ( 'NONE', *, *, #41499, .F. ) ;
#16920=ORIENTED_EDGE ( 'NONE', *, *, #4670, .T. ) ;
#16922=DIRECTION ( 'NONE',  ( -0.9345716196833626643, 0.3557750520798445559, 2.412542607589989711E-09 ) ) ;
#16923=CARTESIAN_POINT ( 'NONE',  ( -10.37462438995674319, -14.89569194323783030, 74.79778901495059529 ) ) ;
#16925=CARTESIAN_POINT ( 'NONE',  ( -11.53247254227971474, -18.68106628708273931, 65.04707076447483871 ) ) ;
#16926=CARTESIAN_POINT ( 'NONE',  ( -22.98865756656685022, -9.855479763439479512, 70.12683098403445570 ) ) ;
#16927=CARTESIAN_POINT ( 'NONE',  ( -10.82793724842355765, -11.34591556451386651, 67.87510537416113721 ) ) ;
#16928=EDGE_LOOP ( 'NONE', ( #44196, #30386, #45079, #1327, #31088 ) ) ;
#16929=VERTEX_POINT ( 'NONE', #42208 ) ;
#16930=CARTESIAN_POINT ( 'NONE',  ( -12.34220853212439550, -20.25709170942694115, 68.47624048511032413 ) ) ;
#16932=CARTESIAN_POINT ( 'NONE',  ( -20.66696756681432490, -21.06910030335248152, 58.64475164910062688 ) ) ;
#16936=EDGE_CURVE ( 'NONE', #34178, #7173, #15170, .T. ) ;
#16937=CARTESIAN_POINT ( 'NONE',  ( -14.92764441971231726, -21.34891144748960201, 61.93600440564248544 ) ) ;
#16938=CARTESIAN_POINT ( 'NONE',  ( -24.02655296236175175, -11.35792967378293916, 66.53719098615387395 ) ) ;
#16939=EDGE_CURVE ( 'NONE', #2617, #3562, #4847, .T. ) ;
#16940=CARTESIAN_POINT ( 'NONE',  ( -14.95356710262008626, -21.83765618392649444, 65.30607879145217964 ) ) ;
#16941=CARTESIAN_POINT ( 'NONE',  ( -24.46557908765160860, -17.24254831546467415, 73.13981945087590475 ) ) ;
#16942=VERTEX_POINT ( 'NONE', #5269 ) ;
#16943=CARTESIAN_POINT ( 'NONE',  ( -10.13939525383658236, -13.24794156168132275, 74.80100763153892274 ) ) ;
#16944=CARTESIAN_POINT ( 'NONE',  ( -23.00382044653182945, -10.58231046269237829, 59.60203429539187425 ) ) ;
#16948=CARTESIAN_POINT ( 'NONE',  ( -23.47974657088402850, -11.29780683472819724, 70.17745371881790106 ) ) ;
#16950=CARTESIAN_POINT ( 'NONE',  ( -20.30349787717712573, -7.937960560238677132, 70.38953857791403834 ) ) ;
#16952=ORIENTED_EDGE ( 'NONE', *, *, #9089, .T. ) ;
#16953=CARTESIAN_POINT ( 'NONE',  ( -11.28948497894591263, -19.03661189358662043, 68.33972770741397085 ) ) ;
#16954=CARTESIAN_POINT ( 'NONE',  ( -21.56016804333223646, -8.612711131324969571, 73.64482796973915413 ) ) ;
#16955=EDGE_LOOP ( 'NONE', ( #30996, #23494 ) ) ;
#16956=EDGE_CURVE ( 'NONE', #2636, #24853, #16751, .T. ) ;
#16957=EDGE_CURVE ( 'NONE', #20590, #1538, #13666, .T. ) ;
#16959=CARTESIAN_POINT ( 'NONE',  ( -14.54749350918766204, -8.372447261038935551, 64.07506791522041567 ) ) ;
#16961=VERTEX_POINT ( 'NONE', #16320 ) ;
#16962=DIRECTION ( 'NONE',  ( 9.588441152175118139E-09, 2.115493544230230216E-07, 0.9999999999999775735 ) ) ;
#16963=CARTESIAN_POINT ( 'NONE',  ( -19.94917705995926482, -8.226604131702123013, 74.00624557436877637 ) ) ;
#16964=CARTESIAN_POINT ( 'NONE',  ( -10.93142192406588720, -17.42570591193873497, 64.85412782098468654 ) ) ;
#16965=ORIENTED_EDGE ( 'NONE', *, *, #45905, .F. ) ;
#16966=CARTESIAN_POINT ( 'NONE',  ( -16.19404102203350249, -7.918066801900436325, 60.21530862784245386 ) ) ;
#16967=CARTESIAN_POINT ( 'NONE',  ( -11.57126885336172073, -10.86466612894600381, 74.59451641100736197 ) ) ;
#16971=ORIENTED_EDGE ( 'NONE', *, *, #43012, .T. ) ;
#16972=ORIENTED_EDGE ( 'NONE', *, *, #14781, .F. ) ;
#16974=FACE_OUTER_BOUND ( 'NONE', #37745, .T. ) ;
#16975=CARTESIAN_POINT ( 'NONE',  ( -21.99178464560338497, -9.439038884874848989, 59.87171213140518944 ) ) ;
#16977=CARTESIAN_POINT ( 'NONE',  ( -10.42592298192601241, -14.97187847733016142, 75.08313515325615128 ) ) ;
#16979=CARTESIAN_POINT ( 'NONE',  ( -11.31272926253210542, -18.32407376160489676, 57.80714615569726078 ) ) ;
#16981=CARTESIAN_POINT ( 'NONE',  ( -16.38321341446914658, -21.78497919871296062, 65.64053219190310529 ) ) ;
#16982=EDGE_CURVE ( 'NONE', #44055, #33140, #47263, .T. ) ;
#16984=CARTESIAN_POINT ( 'NONE',  ( -22.79444606840252874, -10.23710104419528122, 62.95697184964878090 ) ) ;
#16985=CARTESIAN_POINT ( 'NONE',  ( -24.87417209744295477, -14.81009202510037959, 59.28654333241698993 ) ) ;
#16986=CARTESIAN_POINT ( 'NONE',  ( -10.79220851498797096, -11.41472892741485623, 67.79581491584505670 ) ) ;
#16987=EDGE_LOOP ( 'NONE', ( #37519, #43735 ) ) ;
#16990=CARTESIAN_POINT ( 'NONE',  ( -10.88210961209655636, -12.31514285474667503, 57.40027529950947383 ) ) ;
#16992=ADVANCED_FACE ( 'NONE', ( #8730 ), #21792, .T. ) ;
#16993=DIRECTION ( 'NONE',  ( -0.3478314405900341799, -0.9375570856950852239, 0.000000000000000000 ) ) ;
#16997=B_SPLINE_CURVE_WITH_KNOTS ( 'NONE', 3,
 ( #38746, #38243, #5264, #5028, #23497, #23753, #42206, #27421, #35043, #8239 ),
 .UNSPECIFIED., .F., .F.,
 ( 4, 2, 2, 2, 4 ),
 ( 0.6272669072978649396, 0.7522669073148475771, 0.8772669073318302146, 1.002266907348812852, 1.127266907365795490 ),
 .UNSPECIFIED. ) ;
#16999=ORIENTED_EDGE ( 'NONE', *, *, #786, .T. ) ;
#17000=CARTESIAN_POINT ( 'NONE',  ( -11.27120819164457899, -11.36022928427317957, 67.71044750680073321 ) ) ;
#17002=EDGE_LOOP ( 'NONE', ( #4577, #7727 ) ) ;
#17003=CARTESIAN_POINT ( 'NONE',  ( -15.84614975837744133, -7.989249925961589227, 67.14007226002782147 ) ) ;
#17005=CARTESIAN_POINT ( 'NONE',  ( -23.67245686711442687, -11.53637809225759625, 69.98390920472554910 ) ) ;
#17006=ORIENTED_EDGE ( 'NONE', *, *, #4444, .T. ) ;
#17009=CARTESIAN_POINT ( 'NONE',  ( -18.18338144371267617, -21.81849904615365432, 65.63060065626805795 ) ) ;
#17010=EDGE_LOOP ( 'NONE', ( #9079, #18466 ) ) ;
#17013=EDGE_CURVE ( 'NONE', #43190, #45590, #5132, .T. ) ;
#17016=CARTESIAN_POINT ( 'NONE',  ( -20.01838156832885574, -21.36851401455050237, 68.93482423123572289 ) ) ;
#17019=EDGE_LOOP ( 'NONE', ( #47698, #12812 ) ) ;
#17021=CARTESIAN_POINT ( 'NONE',  ( -24.65023647254185590, -12.99629722456026393, 63.01759562046499497 ) ) ;
#17022=CARTESIAN_POINT ( 'NONE',  ( -16.22363853529886057, -7.456506500845998531, 60.30754342289255732 ) ) ;
#17023=ADVANCED_FACE ( 'NONE', ( #10173 ), #17543, .F. ) ;
#17025=CARTESIAN_POINT ( 'NONE',  ( -23.35262004249965528, -18.62986191134476499, 65.70900547832829375 ) ) ;
#17026=CARTESIAN_POINT ( 'NONE',  ( -10.98557796499954087, -17.68114198556070704, 71.86718193507100239 ) ) ;
#17029=EDGE_CURVE ( 'NONE', #33357, #26197, #39720, .T. ) ;
#17030=CARTESIAN_POINT ( 'NONE',  ( -13.49145512112739631, -18.65424914341562612, 54.07175714974879099 ) ) ;
#17031=CARTESIAN_POINT ( 'NONE',  ( -24.36252951794159571, -13.53973495479416478, 59.45448211580517750 ) ) ;
#17032=ORIENTED_EDGE ( 'NONE', *, *, #11881, .T. ) ;
#17034=CARTESIAN_POINT ( 'NONE',  ( -10.13258914451759019, -16.33817228489381179, 71.63245656337019796 ) ) ;
#17035=CARTESIAN_POINT ( 'NONE',  ( -14.50327952430959044, -8.447626442811719372, 64.01652269559008346 ) ) ;
#17037=( BOUNDED_SURFACE ( )  B_SPLINE_SURFACE ( 3, 1, ( 
 ( #27607, #34985 ),
 ( #20708, #16512 ),
 ( #23926, #46809 ),
 ( #46332, #4972 ),
 ( #2226, #12826 ),
 ( #31302, #38929 ),
 ( #39420, #47048 ) ),
 .UNSPECIFIED., .T., .F., .F. ) 
 B_SPLINE_SURFACE_WITH_KNOTS ( ( 4, 3, 4 ),
 ( 2, 2 ),
 ( 0.000000000000000000, 0.5000000000000000000, 1.000000000000000000 ),
 ( 0.000000000000000000, 1.000000000000000000 ),
 .UNSPECIFIED. ) 
 GEOMETRIC_REPRESENTATION_ITEM ( )  RATIONAL_B_SPLINE_SURFACE ( (
 ( 1.000000000000000000, 1.000000000000000000),
 ( 0.3333333333333335369, 0.3333333333333330373),
 ( 0.3333333333333335369, 0.3333333333333330373),
 ( 1.000000000000000000, 1.000000000000000000),
 ( 0.3333333333333333703, 0.3333333333333333703),
 ( 0.3333333333333333703, 0.3333333333333333703),
 ( 1.000000000000000000, 1.000000000000000000) ) ) 
 REPRESENTATION_ITEM ( '' )  SURFACE ( )  );
#17038=EDGE_LOOP ( 'NONE', ( #40934, #13365, #9749, #46187, #47748 ) ) ;
#17040=VECTOR ( 'NONE', #43873, 1000.000000000000227 ) ;
#17041=CARTESIAN_POINT ( 'NONE',  ( -20.86206331040166262, -20.96415858629787721, 62.41471384001169298 ) ) ;
#17042=AXIS2_PLACEMENT_3D ( 'NONE', #22798, #30429, #38027 ) ;
#17043=CARTESIAN_POINT ( 'NONE',  ( -12.58002213166789041, -9.148928514680237711, 74.43427606957253317 ) ) ;
#17044=EDGE_CURVE ( 'NONE', #2461, #5461, #11442, .T. ) ;
#17046=CARTESIAN_POINT ( 'NONE',  ( -21.57946453887431204, -8.565578233975859490, 53.49999999999994316 ) ) ;
#17047=SURFACE_SIDE_STYLE ('',( #31179 ) ) ;
#17048=B_SPLINE_CURVE_WITH_KNOTS ( 'NONE', 3,
 ( #48359, #14592, #43971, #2587 ),
 .UNSPECIFIED., .F., .F.,
 ( 4, 4 ),
 ( 0.8266992229644638535, 1.000000000000000000 ),
 .UNSPECIFIED. ) ;
#17050=CARTESIAN_POINT ( 'NONE',  ( -13.41535341985785301, -9.069179271060303194, 63.98116896315330848 ) ) ;
#17051=CARTESIAN_POINT ( 'NONE',  ( -20.86114118487399338, -21.41899753141851548, 58.84463944793498058 ) ) ;
#17053=( BOUNDED_CURVE ( )  B_SPLINE_CURVE ( 3, ( #18293, #10455, #33545, #44204 ),
 .UNSPECIFIED., .F., .F. ) 
 B_SPLINE_CURVE_WITH_KNOTS ( ( 4, 4 ),
 ( 0.000000000000000000, 0.4074455897393645665 ),
 .UNSPECIFIED. ) 
 CURVE ( )  GEOMETRIC_REPRESENTATION_ITEM ( )  RATIONAL_B_SPLINE_CURVE ( ( 1.000000000000000000, 0.4567392136813290260, 0.3561768502900292122, 0.6983129098261006140 ) ) 
 REPRESENTATION_ITEM ( '' )  );
#17054=CARTESIAN_POINT ( 'NONE',  ( -10.72615791900921423, -12.77470505732934747, 64.56836133915385290 ) ) ;
#17055=( BOUNDED_SURFACE ( )  B_SPLINE_SURFACE ( 3, 1, ( 
 ( #23083, #910 ),
 ( #35103, #42272 ),
 ( #9029, #8536 ),
 ( #4849, #38561 ),
 ( #19868, #1134 ),
 ( #31182, #1370 ),
 ( #27485, #42520 ) ),
 .UNSPECIFIED., .T., .F., .F. ) 
 B_SPLINE_SURFACE_WITH_KNOTS ( ( 4, 3, 4 ),
 ( 2, 2 ),
 ( 0.000000000000000000, 0.5000000000000000000, 1.000000000000000000 ),
 ( 0.000000000000000000, 1.000000000000000000 ),
 .UNSPECIFIED. ) 
 GEOMETRIC_REPRESENTATION_ITEM ( )  RATIONAL_B_SPLINE_SURFACE ( (
 ( 1.000000000000000000, 1.000000000000000000),
 ( 0.3333333333333335369, 0.3333333333333330373),
 ( 0.3333333333333335369, 0.3333333333333330373),
 ( 1.000000000000000000, 1.000000000000000000),
 ( 0.3333333333333333703, 0.3333333333333333703),
 ( 0.3333333333333333703, 0.3333333333333333703),
 ( 1.000000000000000000, 1.000000000000000000) ) ) 
 REPRESENTATION_ITEM ( '' )  SURFACE ( )  );
#17056=VERTEX_POINT ( 'NONE', #14068 ) ;
#17057=ORIENTED_EDGE ( 'NONE', *, *, #25160, .F. ) ;
#17059=LINE ( 'NONE', #24956, #9938 ) ;
#17060=CARTESIAN_POINT ( 'NONE',  ( -14.07986447567954436, -8.151974645673341513, 70.92968827753317385 ) ) ;
#17061=( BOUNDED_SURFACE ( )  B_SPLINE_SURFACE ( 3, 1, ( 
 ( #48448, #45038 ),
 ( #33922, #215 ),
 ( #15195, #41564 ),
 ( #8814, #34649 ),
 ( #16160, #4873 ),
 ( #42292, #19641 ),
 ( #42544, #30736 ) ),
 .UNSPECIFIED., .T., .F., .F. ) 
 B_SPLINE_SURFACE_WITH_KNOTS ( ( 4, 3, 4 ),
 ( 2, 2 ),
 ( 0.000000000000000000, 0.5000000000000000000, 1.000000000000000000 ),
 ( 0.000000000000000000, 1.000000000000000000 ),
 .UNSPECIFIED. ) 
 GEOMETRIC_REPRESENTATION_ITEM ( )  RATIONAL_B_SPLINE_SURFACE ( (
 ( 1.000000000000000000, 1.000000000000000000),
 ( 0.3333333333333335369, 0.3333333333333330373),
 ( 0.3333333333333335369, 0.3333333333333330373),
 ( 1.000000000000000000, 1.000000000000000000),
 ( 0.3333333333333333703, 0.3333333333333333703),
 ( 0.3333333333333333703, 0.3333333333333333703),
 ( 1.000000000000000000, 1.000000000000000000) ) ) 
 REPRESENTATION_ITEM ( '' )  SURFACE ( )  );
#17062=CARTESIAN_POINT ( 'NONE',  ( -22.95693723218890980, -10.52102731622098375, 59.61705815066174097 ) ) ;
#17064=EDGE_LOOP ( 'NONE', ( #22260, #40446, #38793, #28463, #31079 ) ) ;
#17065=CARTESIAN_POINT ( 'NONE',  ( -21.11440761173729186, -20.75744868006576027, 65.77557061749909906 ) ) ;
#17067=EDGE_LOOP ( 'NONE', ( #13158, #28009 ) ) ;
#17069=CARTESIAN_POINT ( 'NONE',  ( -11.98246295270348405, -15.60836430055780433, 54.07175714974878389 ) ) ;
#17072=CARTESIAN_POINT ( 'NONE',  ( -24.11881394502254849, -17.01995806294775448, 73.16863963025599560 ) ) ;
#17073=DIRECTION ( 'NONE',  ( 5.625773296287788022E-06, 7.100530152274343103E-06, 0.9999999999589664901 ) ) ;
#17074=ORIENTED_EDGE ( 'NONE', *, *, #28511, .F. ) ;
#17076=EDGE_CURVE ( 'NONE', #5475, #34665, #36611, .T. ) ;
#17077=DIRECTION ( 'NONE',  ( -0.06306825763707681054, 0.9980092158285027715, 2.415158932891090531E-08 ) ) ;
#17079=DIRECTION ( 'NONE',  ( 1.027096116490394736E-05, 2.598167872976484874E-06, 0.9999999999438784481 ) ) ;
#17080=CARTESIAN_POINT ( 'NONE',  ( -11.03124120290388532, -17.66077365132053956, 71.86718193465377169 ) ) ;
#17082=CARTESIAN_POINT ( 'NONE',  ( -14.31269513454703102, -8.538704322430856308, 67.45078350274380341 ) ) ;
#17083=CARTESIAN_POINT ( 'NONE',  ( -22.38400238879419391, -20.36826089713532895, 62.41934470639706944 ) ) ;
#17084=CARTESIAN_POINT ( 'NONE',  ( -11.06818430912604256, -11.75871762752125349, 71.38860862825016795 ) ) ;
#17085=DIRECTION ( 'NONE',  ( 0.7670373483544791204, 0.6416024518573233415, -2.496223344567303931E-08 ) ) ;
#17087=B_SPLINE_CURVE_WITH_KNOTS ( 'NONE', 3,
 ( #37934, #45107, #26369, #19721, #37685, #1003, #16000, #22945, #41384, #11848 ),
 .UNSPECIFIED., .F., .F.,
 ( 4, 2, 2, 2, 4 ),
 ( 0.1272669073658400374, 0.2522669073463247313, 0.3772669073268094531, 0.5022669073072940638, 0.6272669072877787855 ),
 .UNSPECIFIED. ) ;
#17088=CARTESIAN_POINT ( 'NONE',  ( -19.94917705995926482, -8.226604131702123013, 74.00624557436877637 ) ) ;
#17089=CARTESIAN_POINT ( 'NONE',  ( -17.33262245845742910, -7.759502110702281463, 67.30567542699309058 ) ) ;
#17090=ADVANCED_FACE ( 'NONE', ( #43920 ), #2542, .T. ) ;
#17091=CARTESIAN_POINT ( 'NONE',  ( -16.16063142123006813, -7.467037929575190525, 60.38523757159160965 ) ) ;
#17092=DIRECTION ( 'NONE',  ( -0.4683180279402421875, 0.8835599723313412035, -4.589753180866139968E-08 ) ) ;
#17093=VERTEX_POINT ( 'NONE', #40441 ) ;
#17094=CARTESIAN_POINT ( 'NONE',  ( -24.34764189302621062, -17.56035350371566750, 66.06544510718885022 ) ) ;
#17097=CARTESIAN_POINT ( 'NONE',  ( -9.999882549351870153, -15.43057416212389832, 57.70759442341619661 ) ) ;
#17100=VERTEX_POINT ( 'NONE', #17046 ) ;
#17103=CARTESIAN_POINT ( 'NONE',  ( -19.11145865927416310, -7.964113456900453691, 63.43089235103783352 ) ) ;
#17106=DIRECTION ( 'NONE',  ( 6.816999858124113439E-06, 9.113320815582587851E-06, 0.9999999999352379154 ) ) ;
#17108=CARTESIAN_POINT ( 'NONE',  ( -23.47355814803600893, -18.42978312378849637, 73.05808415355102170 ) ) ;
#17111=ORIENTED_EDGE ( 'NONE', *, *, #23270, .F. ) ;
#17113=CARTESIAN_POINT ( 'NONE',  ( -21.00520398765801744, -21.34214743040633167, 62.37117330845665464 ) ) ;
#17114=CARTESIAN_POINT ( 'NONE',  ( -14.37682202087475680, -19.38786730597467667, 53.49999999999995026 ) ) ;
#17117=ORIENTED_EDGE ( 'NONE', *, *, #25568, .F. ) ;
#17118=CARTESIAN_POINT ( 'NONE',  ( -24.35706328060247827, -15.77560928887050373, 69.53307488759497801 ) ) ;
#17119=CARTESIAN_POINT ( 'NONE',  ( -24.81734138798520561, -15.73308575106217511, 69.64652101300646336 ) ) ;
#17121=VERTEX_POINT ( 'NONE', #43431 ) ;
#17125=ORIENTED_EDGE ( 'NONE', *, *, #10775, .T. ) ;
#17127=DIRECTION ( 'NONE',  ( 3.549360974554993999E-17, -6.371834667797928663E-18, -1.000000000000000000 ) ) ;
#17131=VERTEX_POINT ( 'NONE', #28643 ) ;
#17132=CARTESIAN_POINT ( 'NONE',  ( -20.64396844604977233, -21.02470390210128670, 58.64475165022597025 ) ) ;
#17135=ORIENTED_EDGE ( 'NONE', *, *, #6617, .T. ) ;
#17138=VERTEX_POINT ( 'NONE', #43675 ) ;
#17139=CARTESIAN_POINT ( 'NONE',  ( -20.89788161767221197, -20.94431024770144489, 62.39999296070408974 ) ) ;
#17140=DIRECTION ( 'NONE',  ( -0.9375570856950864451, 0.3478314405900309603, -3.549360974553816870E-17 ) ) ;
#17141=CARTESIAN_POINT ( 'NONE',  ( -24.22092292145011072, -12.93687797069018153, 66.60246741374322710 ) ) ;
#17143=CARTESIAN_POINT ( 'NONE',  ( -21.17741856139999612, -21.24480563955526691, 65.70737070468148033 ) ) ;
#17145=CARTESIAN_POINT ( 'NONE',  ( -21.95938932932862642, -9.477124872050278981, 60.02171213236835712 ) ) ;
#17150=ORIENTED_EDGE ( 'NONE', *, *, #1008, .T. ) ;
#17151=CARTESIAN_POINT ( 'NONE',  ( -10.16422381746084014, -13.13610325312378713, 71.34682038963120476 ) ) ;
#17152=ADVANCED_FACE ( 'NONE', ( #2765 ), #17773, .T. ) ;
#17153=FACE_OUTER_BOUND ( 'NONE', #23525, .T. ) ;
#17154=ORIENTED_EDGE ( 'NONE', *, *, #38869, .F. ) ;
#17156=CARTESIAN_POINT ( 'NONE',  ( -14.07539681412750809, -8.605278097683306981, 74.49954655214880006 ) ) ;
#17158=CARTESIAN_POINT ( 'NONE',  ( -11.46044050272623416, -11.04924139602722200, 57.20903212151936401 ) ) ;
#17160=LINE ( 'NONE', #20152, #10102 ) ;
#17161=CARTESIAN_POINT ( 'NONE',  ( -19.38219705895271261, -7.621082839763254846, 60.15367139372862937 ) ) ;
#17162=EDGE_CURVE ( 'NONE', #14223, #24550, #14269, .T. ) ;
#17163=CARTESIAN_POINT ( 'NONE',  ( -23.27571566865760033, -18.75553318983527262, 72.90801392080540211 ) ) ;
#17164=FACE_OUTER_BOUND ( 'NONE', #15365, .T. ) ;
#17165=ADVANCED_FACE ( 'NONE', ( #25910 ), #19010, .T. ) ;
#17167=EDGE_LOOP ( 'NONE', ( #4746, #46928, #13331, #33627, #17074 ) ) ;
#17168=ORIENTED_EDGE ( 'NONE', *, *, #23614, .T. ) ;
#17169=CARTESIAN_POINT ( 'NONE',  ( -22.89456339367424675, -10.36189766663814638, 63.36626189060206826 ) ) ;
#17171=CARTESIAN_POINT ( 'NONE',  ( -23.64864599473625262, -11.60591425853287539, 66.43831147808981541 ) ) ;
#17175=CARTESIAN_POINT ( 'NONE',  ( -20.82063550681992226, -21.43998110257799539, 58.90121085131534784 ) ) ;
#17179=ORIENTED_EDGE ( 'NONE', *, *, #46106, .F. ) ;
#17180=CARTESIAN_POINT ( 'NONE',  ( -20.81696448553514855, -20.93198605141084201, 62.41471400679856885 ) ) ;
#17183=CARTESIAN_POINT ( 'NONE',  ( -18.20148605613024628, -22.21866286466902451, 65.52249049189786945 ) ) ;
#17185=( BOUNDED_SURFACE ( )  B_SPLINE_SURFACE ( 3, 1, ( 
 ( #25918, #22719 ),
 ( #26650, #10896 ),
 ( #14793, #7466 ),
 ( #19016, #40933 ),
 ( #22467, #29610 ),
 ( #15294, #11875 ),
 ( #23207, #4247 ) ),
 .UNSPECIFIED., .T., .F., .F. ) 
 B_SPLINE_SURFACE_WITH_KNOTS ( ( 4, 3, 4 ),
 ( 2, 2 ),
 ( 0.000000000000000000, 0.5000000000000000000, 1.000000000000000000 ),
 ( 0.000000000000000000, 1.000000000000000000 ),
 .UNSPECIFIED. ) 
 GEOMETRIC_REPRESENTATION_ITEM ( )  RATIONAL_B_SPLINE_SURFACE ( (
 ( 1.000000000000000000, 1.000000000000000000),
 ( 0.3333333333333335369, 0.3333333333333330373),
 ( 0.3333333333333335369, 0.3333333333333330373),
 ( 1.000000000000000000, 1.000000000000000000),
 ( 0.3333333333333333703, 0.3333333333333333703),
 ( 0.3333333333333333703, 0.3333333333333333703),
 ( 1.000000000000000000, 1.000000000000000000) ) ) 
 REPRESENTATION_ITEM ( '' )  SURFACE ( )  );
#17187=ORIENTED_EDGE ( 'NONE', *, *, #37401, .T. ) ;
#17188=CARTESIAN_POINT ( 'NONE',  ( -24.40217295060720204, -14.25566147773195524, 69.95275273531336779 ) ) ;
#17189=FACE_OUTER_BOUND ( 'NONE', #6788, .T. ) ;
#17191=B_SPLINE_CURVE_WITH_KNOTS ( 'NONE', 1,
 ( #18318, #8015 ),
 .UNSPECIFIED., .F., .F.,
 ( 2, 2 ),
 ( 0.000000000000000000, 1.000000000000000000 ),
 .UNSPECIFIED. ) ;
#17192=CARTESIAN_POINT ( 'NONE',  ( -10.45378225047720200, -13.70027870591744446, 74.83384660681542755 ) ) ;
#17193=CARTESIAN_POINT ( 'NONE',  ( -15.51435322605840739, -21.59577299045269427, 72.34015665073278001 ) ) ;
#17194=CARTESIAN_POINT ( 'NONE',  ( -23.49746296483011321, -11.32841565874639222, 70.19210718165021490 ) ) ;
#17195=FACE_OUTER_BOUND ( 'NONE', #22180, .T. ) ;
#17197=EDGE_CURVE ( 'NONE', #11545, #4554, #20771, .T. ) ;
#17199=( BOUNDED_CURVE ( )  B_SPLINE_CURVE ( 3, ( #45182, #19057, #41713, #7754 ),
 .UNSPECIFIED., .F., .F. ) 
 B_SPLINE_CURVE_WITH_KNOTS ( ( 4, 4 ),
 ( 0.000000000000000000, 0.4074455897393635673 ),
 .UNSPECIFIED. ) 
 CURVE ( )  GEOMETRIC_REPRESENTATION_ITEM ( )  RATIONAL_B_SPLINE_CURVE ( ( 1.000000000000000000, 0.4567392136813370196, 0.3561768502900321542, 0.6983129098260854040 ) ) 
 REPRESENTATION_ITEM ( '' )  );
#17200=ORIENTED_EDGE ( 'NONE', *, *, #20219, .F. ) ;
#17201=DIRECTION ( 'NONE',  ( 1.261798975490001659E-05, -2.391811517362266964E-06, 0.9999999999175328558 ) ) ;
#17202=CARTESIAN_POINT ( 'NONE',  ( -19.25563148410905612, -7.587679091002938137, 63.59235773869015418 ) ) ;
#17207=ORIENTED_EDGE ( 'NONE', *, *, #26850, .F. ) ;
#17208=CARTESIAN_POINT ( 'NONE',  ( -15.60243201887541709, -21.62804181911354817, 68.73160055118694345 ) ) ;
#17209=CARTESIAN_POINT ( 'NONE',  ( -20.72574062298286535, -8.580111251864035893, 59.84125250080548142 ) ) ;
#17211=ORIENTED_EDGE ( 'NONE', *, *, #9696, .F. ) ;
#17212=CARTESIAN_POINT ( 'NONE',  ( -23.85493189207092257, -17.57435386044600278, 62.77360986608242399 ) ) ;
#17213=AXIS2_PLACEMENT_3D ( 'NONE', #28854, #36948, #36468 ) ;
#17216=B_SPLINE_CURVE_WITH_KNOTS ( 'NONE', 1,
 ( #33525, #30608 ),
 .UNSPECIFIED., .F., .F.,
 ( 2, 2 ),
 ( 0.000000000000000000, 1.000000000000000000 ),
 .UNSPECIFIED. ) ;
#17217=EDGE_CURVE ( 'NONE', #43000, #23813, #44888, .T. ) ;
#17218=CARTESIAN_POINT ( 'NONE',  ( -11.96893353090061929, -10.42262660427394039, 67.72570221455328010 ) ) ;
#17220=ORIENTED_EDGE ( 'NONE', *, *, #32645, .T. ) ;
#17221=ORIENTED_EDGE ( 'NONE', *, *, #42356, .T. ) ;
#17222=EDGE_CURVE ( 'NONE', #27479, #5194, #8298, .T. ) ;
#17223=DIRECTION ( 'NONE',  ( 3.913797943140854342E-06, 1.965591624649253694E-06, 0.9999999999904093384 ) ) ;
#17224=CARTESIAN_POINT ( 'NONE',  ( -18.78767905735283605, -20.13749289187802916, 53.49999999999995026 ) ) ;
#17225=ORIENTED_EDGE ( 'NONE', *, *, #28979, .F. ) ;
#17226=CARTESIAN_POINT ( 'NONE',  ( -17.65334680565586112, -7.812901805943546663, 60.15348847797940124 ) ) ;
#17229=EDGE_CURVE ( 'NONE', #36010, #41418, #14862, .T. ) ;
#17231=CARTESIAN_POINT ( 'NONE',  ( -24.41470909780205290, -15.75055545595021478, 66.06324634287898334 ) ) ;
#17232=CARTESIAN_POINT ( 'NONE',  ( -24.30048669258562200, -16.36410883687464946, 59.42332431756337741 ) ) ;
#17233=CARTESIAN_POINT ( 'NONE',  ( -12.34063872187652855, -9.996720073711612642, 60.85918082403506446 ) ) ;
#17237=CARTESIAN_POINT ( 'NONE',  ( -24.72694767484942702, -16.28301260341204326, 62.70833288210281609 ) ) ;
#17238=CARTESIAN_POINT ( 'NONE',  ( -10.78910781157109433, -11.42070086764308812, 67.77897960319765502 ) ) ;
#17239=ADVANCED_FACE ( 'NONE', ( #3257 ), #18260, .T. ) ;
#17241=VERTEX_POINT ( 'NONE', #15289 ) ;
#17242=ORIENTED_EDGE ( 'NONE', *, *, #29490, .F. ) ;
#17245=CARTESIAN_POINT ( 'NONE',  ( -22.63008543824757979, -10.12971389395683097, 70.01178520543939499 ) ) ;
#17247=CARTESIAN_POINT ( 'NONE',  ( -23.90351025910924321, -11.13227635073321764, 69.99187118439921562 ) ) ;
#17248=B_SPLINE_CURVE_WITH_KNOTS ( 'NONE', 3,
 ( #36810, #25749, #33355, #15377, #48398, #10731, #30443, #44481, #45456, #40769 ),
 .UNSPECIFIED., .F., .F.,
 ( 4, 2, 2, 2, 4 ),
 ( 0.6272669072877892216, 0.7522669073072935086, 0.8772669073267977957, 1.002266907346302194, 1.127266907365806370 ),
 .UNSPECIFIED. ) ;
#17249=VERTEX_POINT ( 'NONE', #32550 ) ;
#17250=VECTOR ( 'NONE', #45787, 1000.000000000000114 ) ;
#17251=CARTESIAN_POINT ( 'NONE',  ( -16.22269243185835919, -7.456664632783214230, 60.39366801213454750 ) ) ;
#17252=B_SPLINE_CURVE_WITH_KNOTS ( 'NONE', 3,
 ( #4308, #34321, #31129, #46153, #8976, #1573, #16582, #19315, #45684, #12410 ),
 .UNSPECIFIED., .F., .F.,
 ( 4, 2, 2, 2, 4 ),
 ( 0.1272669073658274641, 0.2522669073463270628, 0.3772669073268266615, 0.5022669073073262602, 0.6272669072878258589 ),
 .UNSPECIFIED. ) ;
#17254=ORIENTED_EDGE ( 'NONE', *, *, #38038, .F. ) ;
#17255=CARTESIAN_POINT ( 'NONE',  ( -20.31649657898477912, -7.943510300654241796, 70.43595776394847974 ) ) ;
#17256=CARTESIAN_POINT ( 'NONE',  ( -17.91840021365262814, -21.79173196354552644, 62.17535923606572368 ) ) ;
#17257=EDGE_LOOP ( 'NONE', ( #5699, #28299, #8019, #2621, #11957 ) ) ;
#17258=CARTESIAN_POINT ( 'NONE',  ( -15.81136650494192963, -7.997455857626498243, 67.15509653266745715 ) ) ;
#17259=ORIENTED_EDGE ( 'NONE', *, *, #5099, .T. ) ;
#17260=CYLINDRICAL_SURFACE ( 'NONE', #11009, 0.1500000000000072387 ) ;
#17261=ORIENTED_EDGE ( 'NONE', *, *, #47663, .T. ) ;
#17262=CARTESIAN_POINT ( 'NONE',  ( -11.90387715906214439, -19.81242515194113807, 58.08828870480375173 ) ) ;
#17263=CARTESIAN_POINT ( 'NONE',  ( -23.33186513658400685, -18.65645323816980294, 69.29372015302412535 ) ) ;
#17264=DIRECTION ( 'NONE',  ( 0.2843796944294933460, 0.9587117342539337450, 5.205739956168972140E-08 ) ) ;
#17266=CARTESIAN_POINT ( 'NONE',  ( -13.41013012084913036, -9.008953577314683159, 56.96967469688792818 ) ) ;
#17267=EDGE_CURVE ( 'NONE', #8655, #40234, #12564, .T. ) ;
#17268=CARTESIAN_POINT ( 'NONE',  ( -16.97946104448713101, -21.84517140583366057, 72.46543221429990922 ) ) ;
#17271=CARTESIAN_POINT ( 'NONE',  ( -23.62594491300536959, -11.45603751788689451, 66.70742424642772050 ) ) ;
#17272=CARTESIAN_POINT ( 'NONE',  ( -19.21526828202639336, -8.042187119094190706, 60.24627617707014338 ) ) ;
#17273=ORIENTED_EDGE ( 'NONE', *, *, #201, .F. ) ;
#17274=CARTESIAN_POINT ( 'NONE',  ( -17.45711534482409988, -7.809224652626227225, 63.62345145953160142 ) ) ;
#17275=PLANE ( 'NONE',  #4584 ) ;
#17276=DIRECTION ( 'NONE',  ( 9.941263206242173230E-06, 7.040377906907692017E-06, -0.9999999999258021299 ) ) ;
#17277=CARTESIAN_POINT ( 'NONE',  ( -13.49409790474204840, -20.66256726344224504, 61.53118467422925164 ) ) ;
#17278=EDGE_CURVE ( 'NONE', #20100, #6805, #46964, .T. ) ;
#17279=LINE ( 'NONE', #28135, #28349 ) ;
#17282=ADVANCED_FACE ( 'NONE', ( #21481 ), #46690, .T. ) ;
#17284=LINE ( 'NONE', #43902, #48698 ) ;
#17285=CARTESIAN_POINT ( 'NONE',  ( -10.48067321144888808, -16.03043919553437036, 68.12767830706636119 ) ) ;
#17286=EDGE_LOOP ( 'NONE', ( #11751, #9748, #20008, #33191, #21072 ) ) ;
#17287=CARTESIAN_POINT ( 'NONE',  ( -9.974456290884534226, -14.72748455880875795, 71.51278017970571454 ) ) ;
#17290=CARTESIAN_POINT ( 'NONE',  ( -11.92202137443377907, -10.38855435516889081, 64.18481546414660954 ) ) ;
#17291=CARTESIAN_POINT ( 'NONE',  ( -16.98991614605047218, -22.24663000551990777, 72.35038637723081933 ) ) ;
#17292=ORIENTED_EDGE ( 'NONE', *, *, #32254, .T. ) ;
#17293=CARTESIAN_POINT ( 'NONE',  ( -24.28579947082789303, -13.18942387424446316, 62.84736316175410309 ) ) ;
#17295=CARTESIAN_POINT ( 'NONE',  ( -20.85039448910245241, -8.638677133180788559, 63.45554403117525055 ) ) ;
#17296=ORIENTED_EDGE ( 'NONE', *, *, #44647, .T. ) ;
#17298=CARTESIAN_POINT ( 'NONE',  ( -15.68502974777997494, -7.977065180327442384, 70.90989839958919561 ) ) ;
#17299=VECTOR ( 'NONE', #1077, 1000.000000000000000 ) ;
#17300=CARTESIAN_POINT ( 'NONE',  ( -13.25427695047628873, -8.635260007732634691, 60.60096827762414051 ) ) ;
#17301=CARTESIAN_POINT ( 'NONE',  ( -24.59706363142188934, -12.79617847886399140, 66.48742024426742603 ) ) ;
#17302=CARTESIAN_POINT ( 'NONE',  ( -20.83700022493356130, -19.12221826660257307, 53.49999999999995026 ) ) ;
#17303=CARTESIAN_POINT ( 'NONE',  ( -11.57411280416560651, -10.96269712432890131, 57.28073583805487345 ) ) ;
#17305=ORIENTED_EDGE ( 'NONE', *, *, #14379, .T. ) ;
#17308=ADVANCED_FACE ( 'NONE', ( #10400 ), #39942, .T. ) ;
#17309=EDGE_CURVE ( 'NONE', #39506, #46704, #3237, .T. ) ;
#17310=CARTESIAN_POINT ( 'NONE',  ( -10.37541943412130863, -14.96049300415475614, 75.08306784598362071 ) ) ;
#17311=CARTESIAN_POINT ( 'NONE',  ( -19.04042132780597996, -7.536568533962904048, 67.01576502235467103 ) ) ;
#17312=EDGE_CURVE ( 'NONE', #1731, #15392, #43721, .T. ) ;
#17313=ADVANCED_FACE ( 'NONE', ( #17751 ), #33010, .F. ) ;
#17314=CARTESIAN_POINT ( 'NONE',  ( -20.18941624216641273, -7.891347737435665977, 73.83601159825586535 ) ) ;
#17315=CARTESIAN_POINT ( 'NONE',  ( -10.40888626530166405, -14.10966241957602563, 60.91821293886854249 ) ) ;
#17317=CARTESIAN_POINT ( 'NONE',  ( -21.05203622307093170, -20.79576407825920725, 65.59956342937501006 ) ) ;
#17321=VECTOR ( 'NONE', #19874, 1000.000000000000227 ) ;
#17322=CARTESIAN_POINT ( 'NONE',  ( -19.30271816048872324, -8.014114901043837946, 60.26092997144682784 ) ) ;
#17324=DIRECTION ( 'NONE',  ( 0.09077643883959131410, -0.9958712959773466933, -4.338678766818132329E-08 ) ) ;
#17325=CARTESIAN_POINT ( 'NONE',  ( -12.16754809903432211, -19.43427161745671228, 58.03755408627969103 ) ) ;
#17326=EDGE_LOOP ( 'NONE', ( #4838, #25831 ) ) ;
#17329=CARTESIAN_POINT ( 'NONE',  ( -12.32278866559117780, -19.67576434477648917, 61.41150688479135766 ) ) ;
#17331=( BOUNDED_CURVE ( )  B_SPLINE_CURVE ( 3, ( #17685, #2908, #2443, #9840 ),
 .UNSPECIFIED., .F., .F. ) 
 B_SPLINE_CURVE_WITH_KNOTS ( ( 4, 4 ),
 ( 0.4074455897393622905, 0.5000000000000000000 ),
 .UNSPECIFIED. ) 
 CURVE ( )  GEOMETRIC_REPRESENTATION_ITEM ( )  RATIONAL_B_SPLINE_CURVE ( ( 0.6983129098260907330, 0.7760317562607114139, 0.8765941196520190548, 1.000000000000024203 ) ) 
 REPRESENTATION_ITEM ( '' )  );
#17333=CARTESIAN_POINT ( 'NONE',  ( -11.08737491380029461, -17.78356865475915427, 71.64006328234201249 ) ) ;
#17334=ORIENTED_EDGE ( 'NONE', *, *, #4473, .T. ) ;
#17335=DIRECTION ( 'NONE',  ( 0.8547111024021492032, 0.5191039697695417621, 7.472447835916433805E-08 ) ) ;
#17337=CARTESIAN_POINT ( 'NONE',  ( -15.40900924028612451, -21.51335189680180804, 72.06192110245186200 ) ) ;
#17338=CARTESIAN_POINT ( 'NONE',  ( -11.91343944425293522, -19.82283459374304968, 58.04187056893558605 ) ) ;
#17340=DIRECTION ( 'NONE',  ( -0.4501286257827957216, -0.8929637284072022840, 1.500157795982635434E-08 ) ) ;
#17341=EDGE_CURVE ( 'NONE', #260, #15899, #7266, .T. ) ;
#17342=VECTOR ( 'NONE', #33292, 1000.000000000000000 ) ;
#17343=DIRECTION ( 'NONE',  ( -0.6105870317843965500, -0.7919491628991826015, 6.540688078712152548E-08 ) ) ;
#17344=CARTESIAN_POINT ( 'NONE',  ( -23.42597896001542424, -18.52301023162717897, 65.97956265853692059 ) ) ;
#17345=EDGE_LOOP ( 'NONE', ( #43035, #2056, #20872, #46228, #11528 ) ) ;
#17346=CARTESIAN_POINT ( 'NONE',  ( -13.84149883539359749, -8.276978603410436008, 74.33808174404438773 ) ) ;
#17350=( BOUNDED_CURVE ( )  B_SPLINE_CURVE ( 3, ( #4974, #34989, #8910, #46085 ),
 .UNSPECIFIED., .F., .F. ) 
 B_SPLINE_CURVE_WITH_KNOTS ( ( 4, 4 ),
 ( 0.000000000000000000, 0.4074455897393651771 ),
 .UNSPECIFIED. ) 
 CURVE ( )  GEOMETRIC_REPRESENTATION_ITEM ( )  RATIONAL_B_SPLINE_CURVE ( ( 1.000000000000000000, 0.4567392136813375192, 0.3561768502900323208, 0.6983129098260844048 ) ) 
 REPRESENTATION_ITEM ( '' )  );
#17352=CIRCLE ( 'NONE', #14202, 2.499999999999999556 ) ;
#17353=ORIENTED_EDGE ( 'NONE', *, *, #34557, .F. ) ;
#17354=ORIENTED_EDGE ( 'NONE', *, *, #10058, .F. ) ;
#17355=VERTEX_POINT ( 'NONE', #34735 ) ;
#17356=AXIS2_PLACEMENT_3D ( 'NONE', #19338, #34347, #15633 ) ;
#17357=CARTESIAN_POINT ( 'NONE',  ( -16.13432406759100601, -21.74052631579560568, 58.30057715624173653 ) ) ;
#17358=CARTESIAN_POINT ( 'NONE',  ( -23.15062936622491563, -18.83573383206660168, 66.10772932244093170 ) ) ;
#17359=CYLINDRICAL_SURFACE ( 'NONE', #43258, 0.1499999999999988565 ) ;
#17362=( BOUNDED_CURVE ( )  B_SPLINE_CURVE ( 3, ( #9898, #42672, #39925, #17009 ),
 .UNSPECIFIED., .F., .F. ) 
 B_SPLINE_CURVE_WITH_KNOTS ( ( 4, 4 ),
 ( 0.9074455897393701731, 1.000000000000000000 ),
 .UNSPECIFIED. ) 
 CURVE ( )  GEOMETRIC_REPRESENTATION_ITEM ( )  RATIONAL_B_SPLINE_CURVE ( ( 0.6983129098261113832, 0.7760317562607140784, 0.8765941196520102840, 1.000000000000000000 ) ) 
 REPRESENTATION_ITEM ( '' )  );
#17366=ADVANCED_FACE ( 'NONE', ( #7434 ), #34481, .T. ) ;
#17367=CARTESIAN_POINT ( 'NONE',  ( -11.47236213698566054, -10.32806074475630886, 74.55389686390628867 ) ) ;
#17371=B_SPLINE_CURVE_WITH_KNOTS ( 'NONE', 3,
 ( #29915, #37513, #11203, #3809, #30169, #4528, #42210, #19308, #26951, #38011 ),
 .UNSPECIFIED., .F., .F.,
 ( 4, 2, 2, 2, 4 ),
 ( 0.6272669072978946936, 0.7522669073148660068, 0.8772669073318372090, 1.002266907348808411, 1.127266907365779725 ),
 .UNSPECIFIED. ) ;
#17372=EDGE_CURVE ( 'NONE', #47972, #41967, #41392, .T. ) ;
#17373=ADVANCED_FACE ( 'NONE', ( #522 ), #19725, .T. ) ;
#17374=ORIENTED_EDGE ( 'NONE', *, *, #48321, .F. ) ;
#17375=CARTESIAN_POINT ( 'NONE',  ( -18.12273401612753077, -22.22646211661374593, 65.46036745194116691 ) ) ;
#17377=CARTESIAN_POINT ( 'NONE',  ( -24.87384330133638599, -14.87999890626018384, 59.35804801245023299 ) ) ;
#17379=ORIENTED_EDGE ( 'NONE', *, *, #13481, .T. ) ;
#17382=CARTESIAN_POINT ( 'NONE',  ( -22.49805064719525305, -9.986866608920609067, 73.48161091687566682 ) ) ;
#17384=CARTESIAN_POINT ( 'NONE',  ( -18.90223155190902915, -7.506551502853892721, 67.01416387246997886 ) ) ;
#17386=AXIS2_PLACEMENT_3D ( 'NONE', #42796, #20139, #39087 ) ;
#17387=VERTEX_POINT ( 'NONE', #1009 ) ;
#17390=FACE_OUTER_BOUND ( 'NONE', #10172, .T. ) ;
#17391=ORIENTED_EDGE ( 'NONE', *, *, #45151, .T. ) ;
#17392=CARTESIAN_POINT ( 'NONE',  ( -24.83419172831454347, -15.58085240086919576, 73.14157211650798729 ) ) ;
#17393=AXIS2_PLACEMENT_3D ( 'NONE', #21341, #47917, #29203 ) ;
#17394=CARTESIAN_POINT ( 'NONE',  ( -24.85911909788007179, -14.32540520456757172, 69.83930567627945152 ) ) ;
#17395=EDGE_LOOP ( 'NONE', ( #29145, #27853 ) ) ;
#17396=B_SPLINE_CURVE_WITH_KNOTS ( 'NONE', 3,
 ( #17594, #32627, #2102, #6039, #19008, #59, #11869, #27119, #22714, #42396 ),
 .UNSPECIFIED., .F., .F.,
 ( 4, 2, 2, 2, 4 ),
 ( 0.6272669072877625762, 0.7522669073072669743, 0.8772669073267712614, 1.002266907346275548, 1.127266907365779947 ),
 .UNSPECIFIED. ) ;
#17400=DIRECTION ( 'NONE',  ( -0.3478314405900308492, -0.9375570856950864451, 0.000000000000000000 ) ) ;
#17401=CARTESIAN_POINT ( 'NONE',  ( -24.66730449611544529, -13.06573935865489844, 62.94768786448354092 ) ) ;
#17402=CARTESIAN_POINT ( 'NONE',  ( -16.93941734680483080, -7.775588144984237005, 74.24546186738449194 ) ) ;
#17403=CARTESIAN_POINT ( 'NONE',  ( -24.03160975973305824, -17.26750547207224784, 69.56339792588553905 ) ) ;
#17404=ORIENTED_EDGE ( 'NONE', *, *, #27758, .T. ) ;
#17405=CARTESIAN_POINT ( 'NONE',  ( -21.98930295831539894, -9.502568441585983905, 59.72171225693869445 ) ) ;
#17407=CARTESIAN_POINT ( 'NONE',  ( -19.04042241193164386, -7.536568769452434147, 67.01576393362593365 ) ) ;
#17408=CARTESIAN_POINT ( 'NONE',  ( -24.35021929840575439, -16.12578517662164401, 62.88768852640185258 ) ) ;
#17409=EDGE_LOOP ( 'NONE', ( #13323, #20879, #39319, #45434, #22424 ) ) ;
#17410=CARTESIAN_POINT ( 'NONE',  ( -10.60570718526854961, -17.81143598018131158, 71.68222757358374508 ) ) ;
#17414=ORIENTED_EDGE ( 'NONE', *, *, #13758, .T. ) ;
#17417=CARTESIAN_POINT ( 'NONE',  ( -13.33151401730585306, -20.55006798877650454, 58.06122216312902395 ) ) ;
#17421=ADVANCED_FACE ( 'NONE', ( #44865 ), #30090, .F. ) ;
#17422=CARTESIAN_POINT ( 'NONE',  ( -21.25790634982353211, -21.19723378012398030, 65.74487280419876356 ) ) ;
#17423=CARTESIAN_POINT ( 'NONE',  ( -12.23693665947836529, -20.15673230564203422, 65.06663674221491078 ) ) ;
#17424=CARTESIAN_POINT ( 'NONE',  ( -18.79049830835916524, -7.892586073225762000, 70.38540174208183942 ) ) ;
#17426=ORIENTED_EDGE ( 'NONE', *, *, #5394, .F. ) ;
#17428=CARTESIAN_POINT ( 'NONE',  ( -20.13360759725221882, -21.74902176548401300, 72.55478737390036770 ) ) ;
#17432=DIRECTION ( 'NONE',  ( 0.9629498065864428025, 0.2696806815386155187, -2.751890642837150366E-17 ) ) ;
#17433=CARTESIAN_POINT ( 'NONE',  ( -11.03124120290388532, -17.66077365132053956, 71.86718193465377169 ) ) ;
#17434=CARTESIAN_POINT ( 'NONE',  ( -11.05981229291193024, -11.89443034174749769, 71.19746914266430338 ) ) ;
#17435=B_SPLINE_CURVE_WITH_KNOTS ( 'NONE', 1,
 ( #38717, #43147 ),
 .UNSPECIFIED., .F., .F.,
 ( 2, 2 ),
 ( 0.000000000000000000, 1.000000000000000000 ),
 .UNSPECIFIED. ) ;
#17437=ORIENTED_EDGE ( 'NONE', *, *, #39279, .T. ) ;
#17438=CARTESIAN_POINT ( 'NONE',  ( -20.04849592361258104, -21.35284569240296548, 72.69006679631316103 ) ) ;
#17440=EDGE_CURVE ( 'NONE', #9885, #5635, #41153, .T. ) ;
#17441=CARTESIAN_POINT ( 'NONE',  ( -14.67111461712440601, -7.886426496449994161, 60.43500955848998757 ) ) ;
#17442=CARTESIAN_POINT ( 'NONE',  ( -10.10502314809590274, -16.20379097455708006, 68.09112436593052564 ) ) ;
#17446=EDGE_CURVE ( 'NONE', #43090, #15096, #8582, .T. ) ;
#17447=CARTESIAN_POINT ( 'NONE',  ( -10.38078069312423679, -14.50222183502507356, 68.00800126083242958 ) ) ;
#17448=CARTESIAN_POINT ( 'NONE',  ( -20.13271805750754950, -8.299978134201072777, 70.53628287813307907 ) ) ;
#17450=EDGE_CURVE ( 'NONE', #31116, #8437, #3763, .T. ) ;
#17453=CARTESIAN_POINT ( 'NONE',  ( -22.99017014647701984, -19.05426393579631750, 59.18410607220618402 ) ) ;
#17456=CARTESIAN_POINT ( 'NONE',  ( -11.28576306333344625, -19.03127759451936285, 68.37836181605487695 ) ) ;
#17457=ORIENTED_EDGE ( 'NONE', *, *, #13647, .F. ) ;
#17458=CARTESIAN_POINT ( 'NONE',  ( -13.71953088125924225, -21.27299755413469384, 68.63341999928891823 ) ) ;
#17461=VERTEX_POINT ( 'NONE', #39641 ) ;
#17462=CARTESIAN_POINT ( 'NONE',  ( -18.86498648104808495, -7.957467358499918042, 70.55995216654250157 ) ) ;
#17466=CARTESIAN_POINT ( 'NONE',  ( -19.89081357980290932, -21.83916422767060794, 69.07449100745587600 ) ) ;
#17468=CARTESIAN_POINT ( 'NONE',  ( -11.32638108541902788, -11.37148941047682627, 60.78771700233693309 ) ) ;
#17469=CARTESIAN_POINT ( 'NONE',  ( -20.19231657184298001, -8.325423463105359190, 70.25100341277899929 ) ) ;
#17470=VERTEX_POINT ( 'NONE', #1739 ) ;
#17471=EDGE_LOOP ( 'NONE', ( #45350, #20256 ) ) ;
#17472=CARTESIAN_POINT ( 'NONE',  ( -23.77312771997254615, -18.70709664074277612, 72.87872845841107505 ) ) ;
#17473=CARTESIAN_POINT ( 'NONE',  ( -13.22529448846758982, -9.145569705956512863, 64.19474388871357462 ) ) ;
#17474=VERTEX_POINT ( 'NONE', #9374 ) ;
#17477=CARTESIAN_POINT ( 'NONE',  ( -23.05195072219661512, -10.55808160950470409, 63.48674805708738234 ) ) ;
#17479=CARTESIAN_POINT ( 'NONE',  ( -13.89388974506275787, -21.36980381032900667, 72.11102993026078423 ) ) ;
#17480=CARTESIAN_POINT ( 'NONE',  ( -19.36683724782897897, -21.58655468785150688, 62.00975759738177118 ) ) ;
#17481=ORIENTED_EDGE ( 'NONE', *, *, #38261, .F. ) ;
#17482=CARTESIAN_POINT ( 'NONE',  ( -13.07136655094769750, -8.762923122256669473, 64.02451139116674028 ) ) ;
#17483=CARTESIAN_POINT ( 'NONE',  ( -24.08907074505709645, -11.48026357735065872, 63.13713704106291402 ) ) ;
#17485=( BOUNDED_CURVE ( )  B_SPLINE_CURVE ( 3, ( #9728, #46900, #2078, #43215 ),
 .UNSPECIFIED., .F., .F. ) 
 B_SPLINE_CURVE_WITH_KNOTS ( ( 4, 4 ),
 ( 0.4074455897393639559, 0.5000000000000000000 ),
 .UNSPECIFIED. ) 
 CURVE ( )  GEOMETRIC_REPRESENTATION_ITEM ( )  RATIONAL_B_SPLINE_CURVE ( ( 0.6983129098260867362, 0.7760317562606950936, 0.8765941196520002920, 1.000000000000003775 ) ) 
 REPRESENTATION_ITEM ( '' )  );
#17488=CARTESIAN_POINT ( 'NONE',  ( -24.46435014771442695, -14.30944682264569856, 62.86863794226144364 ) ) ;
#17489=EDGE_CURVE ( 'NONE', #18401, #35636, #5520, .T. ) ;
#17492=( BOUNDED_CURVE ( )  B_SPLINE_CURVE ( 3, ( #35032, #16560, #12157, #41957 ),
 .UNSPECIFIED., .F., .F. ) 
 B_SPLINE_CURVE_WITH_KNOTS ( ( 4, 4 ),
 ( 0.000000000000000000, 0.4074455897393675086 ),
 .UNSPECIFIED. ) 
 CURVE ( )  GEOMETRIC_REPRESENTATION_ITEM ( )  RATIONAL_B_SPLINE_CURVE ( ( 1.000000000000000000, 0.4567392136813269721, 0.3561768502900284350, 0.6983129098261046108 ) ) 
 REPRESENTATION_ITEM ( '' )  );
#17497=DIRECTION ( 'NONE',  ( 7.166348388238339064E-06, -1.030346078752312232E-05, -0.9999999999212410007 ) ) ;
#17498=EDGE_CURVE ( 'NONE', #31661, #29406, #3527, .T. ) ;
#17499=CARTESIAN_POINT ( 'NONE',  ( -17.87922771257724008, -21.79450505577156960, 61.87535931805457778 ) ) ;
#17500=CARTESIAN_POINT ( 'NONE',  ( -14.98249323814573941, -9.880861343182303358, 54.07175714974879099 ) ) ;
#17502=PLANE ( 'NONE',  #32284 ) ;
#17505=CARTESIAN_POINT ( 'NONE',  ( -10.71495605983455590, -12.81234157828920850, 64.26836111193937029 ) ) ;
#17506=CARTESIAN_POINT ( 'NONE',  ( -17.42539685990596254, -7.755594512365703963, 70.58215807128591734 ) ) ;
#17507=ORIENTED_EDGE ( 'NONE', *, *, #24884, .F. ) ;
#17508=CARTESIAN_POINT ( 'NONE',  ( -24.14695329351509656, -18.01973419914282104, 59.18191163003312028 ) ) ;
#17509=CARTESIAN_POINT ( 'NONE',  ( -10.25351306168449383, -12.78524163461458762, 64.38180785400611228 ) ) ;
#17510=VECTOR ( 'NONE', #36500, 1000.000000000000227 ) ;
#17511=CYLINDRICAL_SURFACE ( 'NONE', #31260, 0.1500000000000000222 ) ;
#17512=EDGE_CURVE ( 'NONE', #27648, #20725, #16729, .T. ) ;
#17513=CARTESIAN_POINT ( 'NONE',  ( -24.44757306576362410, -14.11227934896924374, 66.33859978849633876 ) ) ;
#17515=CARTESIAN_POINT ( 'NONE',  ( -10.39891438989669226, -17.28914431743334035, 61.26404815609701870 ) ) ;
#17516=VERTEX_POINT ( 'NONE', #35454 ) ;
#17517=CARTESIAN_POINT ( 'NONE',  ( -11.46875891826176819, -18.48806303968299858, 61.27710833525312495 ) ) ;
#17518=ADVANCED_FACE ( 'NONE', ( #16497 ), #46066, .T. ) ;
#17519=CARTESIAN_POINT ( 'NONE',  ( -11.73157977884637226, -10.00306985186507269, 67.75542791425031908 ) ) ;
#17520=CARTESIAN_POINT ( 'NONE',  ( -22.97398039646707701, -9.839151245828711367, 70.11204270335640842 ) ) ;
#17521=B_SPLINE_CURVE_WITH_KNOTS ( 'NONE', 1,
 ( #21030, #1835 ),
 .UNSPECIFIED., .F., .F.,
 ( 2, 2 ),
 ( 0.000000000000000000, 1.000000000000000000 ),
 .UNSPECIFIED. ) ;
#17522=FACE_OUTER_BOUND ( 'NONE', #40731, .T. ) ;
#17523=CARTESIAN_POINT ( 'NONE',  ( -18.67686240032185552, -7.922096350451282909, 70.37067976680781101 ) ) ;
#17524=EDGE_CURVE ( 'NONE', #15882, #21369, #16654, .T. ) ;
#17528=CARTESIAN_POINT ( 'NONE',  ( -21.64853795319383067, -9.164858462540919959, 66.95590184911722531 ) ) ;
#17530=ORIENTED_EDGE ( 'NONE', *, *, #35060, .F. ) ;
#17531=CARTESIAN_POINT ( 'NONE',  ( -11.33476804054750531, -19.10151225439055978, 68.40184904730287485 ) ) ;
#17532=CARTESIAN_POINT ( 'NONE',  ( -10.62793585389281326, -13.13198463278400041, 67.81120344634712183 ) ) ;
#17533=CARTESIAN_POINT ( 'NONE',  ( -11.79792781917550570, -18.97409009807959279, 71.68685885149984927 ) ) ;
#17536=CARTESIAN_POINT ( 'NONE',  ( -10.42492065060444872, -12.25670954885047692, 57.58503240040955262 ) ) ;
#17538=FACE_BOUND ( 'NONE', #25956, .T. ) ;
#17539=CARTESIAN_POINT ( 'NONE',  ( -10.79572441526863180, -11.40795732096215254, 67.80359905390240272 ) ) ;
#17541=CARTESIAN_POINT ( 'NONE',  ( -14.80637861323768334, -7.834189837989483429, 57.04274166530056078 ) ) ;
#17543=PLANE ( 'NONE',  #32177 ) ;
#17544=CARTESIAN_POINT ( 'NONE',  ( -11.50962084936622709, -18.55351502409101272, 61.29213219555924042 ) ) ;
#17545=CARTESIAN_POINT ( 'NONE',  ( -10.40948780249357597, -12.29963818034608813, 57.52846117370101098 ) ) ;
#17546=CARTESIAN_POINT ( 'NONE',  ( -22.56207008003183745, -19.63703213565221617, 72.92928497383269359 ) ) ;
#17547=CARTESIAN_POINT ( 'NONE',  ( -15.39389095703113952, -21.97733419268598709, 72.23070866474378704 ) ) ;
#17548=DIRECTION ( 'NONE',  ( -0.7364384864160969935, 0.6765045127160409510, 1.031360481960658298E-08 ) ) ;
#17549=ORIENTED_EDGE ( 'NONE', *, *, #45484, .T. ) ;
#17550=ORIENTED_EDGE ( 'NONE', *, *, #11132, .F. ) ;
#17552=CARTESIAN_POINT ( 'NONE',  ( -10.40174263535760524, -17.29725023780839166, 61.34238537770443855 ) ) ;
#17557=CARTESIAN_POINT ( 'NONE',  ( -10.37873872693602273, -15.23103030436339544, 74.95345861988057834 ) ) ;
#17559=CARTESIAN_POINT ( 'NONE',  ( -11.32522400900782067, -11.27219014254736074, 60.96413645226084554 ) ) ;
#17560=CARTESIAN_POINT ( 'NONE',  ( -22.07805708657739885, -20.69058616546009333, 53.49999999999994316 ) ) ;
#17564=ORIENTED_EDGE ( 'NONE', *, *, #9424, .T. ) ;
#17565=FACE_OUTER_BOUND ( 'NONE', #46796, .T. ) ;
#17566=CARTESIAN_POINT ( 'NONE',  ( -18.63483346095911131, -21.70376574273382175, 72.35798910450991173 ) ) ;
#17567=ORIENTED_EDGE ( 'NONE', *, *, #6881, .T. ) ;
#17568=DIRECTION ( 'NONE',  ( 4.615129112206533859E-07, -1.699487772732772144E-08, 0.9999999999998934186 ) ) ;
#17569=CARTESIAN_POINT ( 'NONE',  ( -24.83515292193595769, -14.04764123926324082, 73.23776205861604183 ) ) ;
#17570=( BOUNDED_SURFACE ( )  B_SPLINE_SURFACE ( 3, 1, ( 
 ( #15168, #14919 ),
 ( #44760, #19611 ),
 ( #4128, #26035 ),
 ( #7335, #33633 ),
 ( #48673, #29976 ),
 ( #34134, #33898 ),
 ( #426, #15406 ) ),
 .UNSPECIFIED., .T., .F., .F. ) 
 B_SPLINE_SURFACE_WITH_KNOTS ( ( 4, 3, 4 ),
 ( 2, 2 ),
 ( 0.000000000000000000, 0.5000000000000000000, 1.000000000000000000 ),
 ( 0.000000000000000000, 1.000000000000000000 ),
 .UNSPECIFIED. ) 
 GEOMETRIC_REPRESENTATION_ITEM ( )  RATIONAL_B_SPLINE_SURFACE ( (
 ( 1.000000000000000000, 1.000000000000000000),
 ( 0.3333333333333335369, 0.3333333333333330373),
 ( 0.3333333333333335369, 0.3333333333333330373),
 ( 1.000000000000000000, 1.000000000000000000),
 ( 0.3333333333333333703, 0.3333333333333333703),
 ( 0.3333333333333333703, 0.3333333333333333703),
 ( 1.000000000000000000, 1.000000000000000000) ) ) 
 REPRESENTATION_ITEM ( '' )  SURFACE ( )  );
#17571=CARTESIAN_POINT ( 'NONE',  ( -21.73099075187129614, -8.730192115828774746, 70.31627817507801126 ) ) ;
#17575=DIRECTION ( 'NONE',  ( 0.9862050927915948506, 0.1655279884246635136, 7.765682856207885122E-08 ) ) ;
#17576=EDGE_CURVE ( 'NONE', #17705, #2492, #45454, .T. ) ;
#17577=CARTESIAN_POINT ( 'NONE',  ( -11.96073139429061527, -19.87431630704028152, 57.97036459255868124 ) ) ;
#17579=EDGE_CURVE ( 'NONE', #6698, #8929, #13293, .T. ) ;
#17582=CIRCLE ( 'NONE', #15189, 7.000000000000000888 ) ;
#17583=CARTESIAN_POINT ( 'NONE',  ( -21.65914559189701194, -18.31838547852702348, 53.49999999999995026 ) ) ;
#17584=CARTESIAN_POINT ( 'NONE',  ( -23.27284462870851911, -18.74605969774991010, 66.10917289053097079 ) ) ;
#17585=ORIENTED_EDGE ( 'NONE', *, *, #36867, .T. ) ;
#17586=CARTESIAN_POINT ( 'NONE',  ( -23.46260370332431577, -11.17067683354235719, 73.66193301755811262 ) ) ;
#17587=CARTESIAN_POINT ( 'NONE',  ( -24.16515061560491162, -17.98105989040287866, 59.15378417205010209 ) ) ;
#17588=CARTESIAN_POINT ( 'NONE',  ( -24.08318141890305597, -17.12462156339858055, 72.88895803463330481 ) ) ;
#17589=ORIENTED_EDGE ( 'NONE', *, *, #27685, .T. ) ;
#17591=EDGE_LOOP ( 'NONE', ( #33456, #7710 ) ) ;
#17592=VERTEX_POINT ( 'NONE', #21890 ) ;
#17594=CARTESIAN_POINT ( 'NONE',  ( -10.03035368457962662, -15.72374687363213575, 61.22284448286259817 ) ) ;
#17598=ORIENTED_EDGE ( 'NONE', *, *, #46372, .T. ) ;
#17602=FACE_OUTER_BOUND ( 'NONE', #19121, .T. ) ;
#17603=DIRECTION ( 'NONE',  ( 0.8547111024021490921, 0.5191039697695417621, 7.472447835916433805E-08 ) ) ;
#17606=EDGE_LOOP ( 'NONE', ( #2016, #38814, #16001, #27538, #33628 ) ) ;
#17607=B_SPLINE_CURVE_WITH_KNOTS ( 'NONE', 3,
 ( #22450, #10876, #26149, #41160, #33256, #18002, #3734, #18744, #25646, #21716 ),
 .UNSPECIFIED., .F., .F.,
 ( 4, 2, 2, 2, 4 ),
 ( 0.6272669072877946617, 0.7522669073073083856, 0.8772669073268219986, 1.002266907346335723, 1.127266907365849447 ),
 .UNSPECIFIED. ) ;
#17608=EDGE_CURVE ( 'NONE', #14795, #12703, #30199, .T. ) ;
#17609=DIRECTION ( 'NONE',  ( 0.9375570856950865561, -0.3478314405900308492, 0.000000000000000000 ) ) ;
#17610=EDGE_CURVE ( 'NONE', #18615, #28180, #25352, .T. ) ;
#17611=DIRECTION ( 'NONE',  ( 0.4599824152910792496, 0.8879280250239794947, 2.250728352126283681E-08 ) ) ;
#17612=( BOUNDED_CURVE ( )  B_SPLINE_CURVE ( 3, ( #22258, #26200, #25701, #29402 ),
 .UNSPECIFIED., .F., .F. ) 
 B_SPLINE_CURVE_WITH_KNOTS ( ( 4, 4 ),
 ( 0.000000000000000000, 0.4074455897393676196 ),
 .UNSPECIFIED. ) 
 CURVE ( )  GEOMETRIC_REPRESENTATION_ITEM ( )  RATIONAL_B_SPLINE_CURVE ( ( 1.000000000000000000, 0.4567392136813364090, 0.3561768502900319322, 0.6983129098260865142 ) ) 
 REPRESENTATION_ITEM ( '' )  );
#17615=ORIENTED_EDGE ( 'NONE', *, *, #16638, .F. ) ;
#17616=B_SPLINE_CURVE_WITH_KNOTS ( 'NONE', 3,
 ( #47472, #27778, #42807, #34308, #37767, #30654, #29911, #11199, #3551, #10039 ),
 .UNSPECIFIED., .F., .F.,
 ( 4, 2, 2, 2, 4 ),
 ( 0.000000000000000000, 0.2500000000000000000, 0.5000000000000000000, 0.7500000000000000000, 1.000000000000000000 ),
 .UNSPECIFIED. ) ;
#17617=CARTESIAN_POINT ( 'NONE',  ( -10.70532053225239544, -12.67267096592666498, 61.08381491717225487 ) ) ;
#17618=CARTESIAN_POINT ( 'NONE',  ( -23.81024829756716343, -18.64597716098235836, 72.94863620959463901 ) ) ;
#17624=CARTESIAN_POINT ( 'NONE',  ( -24.83263378688676326, -15.59489965655864374, 73.18799144572807336 ) ) ;
#17625=( BOUNDED_CURVE ( )  B_SPLINE_CURVE ( 3, ( #1492, #16506, #24401, #5920 ),
 .UNSPECIFIED., .F., .F. ) 
 B_SPLINE_CURVE_WITH_KNOTS ( ( 4, 4 ),
 ( 0.000000000000000000, 0.4074455897393596260 ),
 .UNSPECIFIED. ) 
 CURVE ( )  GEOMETRIC_REPRESENTATION_ITEM ( )  RATIONAL_B_SPLINE_CURVE ( ( 1.000000000000000000, 0.4567392136813444026, 0.3561768502900348743, 0.6983129098260714152 ) ) 
 REPRESENTATION_ITEM ( '' )  );
#17626=CARTESIAN_POINT ( 'NONE',  ( -13.27770465421436796, -9.107456272842561873, 64.20946529204060482 ) ) ;
#17628=FACE_OUTER_BOUND ( 'NONE', #48731, .T. ) ;
#17629=FACE_OUTER_BOUND ( 'NONE', #12867, .T. ) ;
#17630=VERTEX_POINT ( 'NONE', #44088 ) ;
#17631=ADVANCED_FACE ( 'NONE', ( #10089 ), #37131, .T. ) ;
#17633=CARTESIAN_POINT ( 'NONE',  ( -11.02242957576233451, -11.85532881267382166, 74.57312195644870201 ) ) ;
#17635=CARTESIAN_POINT ( 'NONE',  ( -24.03161744405940325, -17.27608056677072312, 73.29824685711943744 ) ) ;
#17636=B_SPLINE_CURVE_WITH_KNOTS ( 'NONE', 3,
 ( #46949, #47202, #17858, #9295, #20853, #39322, #9782, #16895, #40054, #1895 ),
 .UNSPECIFIED., .F., .F.,
 ( 4, 2, 2, 2, 4 ),
 ( 0.000000000000000000, 0.2500000000000000000, 0.5000000000000000000, 0.7500000000000000000, 1.000000000000000000 ),
 .UNSPECIFIED. ) ;
#17637=LINE ( 'NONE', #6577, #24314 ) ;
#17638=EDGE_LOOP ( 'NONE', ( #30983, #22540 ) ) ;
#17641=CARTESIAN_POINT ( 'NONE',  ( -21.55304606329672623, -8.607909972211214011, 73.72315957790283392 ) ) ;
#17642=ORIENTED_EDGE ( 'NONE', *, *, #21206, .F. ) ;
#17643=CARTESIAN_POINT ( 'NONE',  ( -10.39538363539702104, -14.16717768424945412, 68.00232930279112509 ) ) ;
#17644=( BOUNDED_SURFACE ( )  B_SPLINE_SURFACE ( 3, 1, ( 
 ( #33774, #3262 ),
 ( #23376, #19686 ),
 ( #21978, #33272 ),
 ( #12288, #8610 ),
 ( #27309, #10894 ),
 ( #25917, #10656 ),
 ( #11145, #36974 ) ),
 .UNSPECIFIED., .T., .F., .F. ) 
 B_SPLINE_SURFACE_WITH_KNOTS ( ( 4, 3, 4 ),
 ( 2, 2 ),
 ( 0.000000000000000000, 0.5000000000000000000, 1.000000000000000000 ),
 ( 0.000000000000000000, 1.000000000000000000 ),
 .UNSPECIFIED. ) 
 GEOMETRIC_REPRESENTATION_ITEM ( )  RATIONAL_B_SPLINE_SURFACE ( (
 ( 1.000000000000000000, 1.000000000000000000),
 ( 0.3333333333333335369, 0.3333333333333330373),
 ( 0.3333333333333335369, 0.3333333333333330373),
 ( 1.000000000000000000, 1.000000000000000000),
 ( 0.3333333333333333703, 0.3333333333333333703),
 ( 0.3333333333333333703, 0.3333333333333333703),
 ( 1.000000000000000000, 1.000000000000000000) ) ) 
 REPRESENTATION_ITEM ( '' )  SURFACE ( )  );
#17645=EDGE_CURVE ( 'NONE', #918, #38805, #6632, .T. ) ;
#17646=ADVANCED_FACE ( 'NONE', ( #6637 ), #21653, .T. ) ;
#17647=CARTESIAN_POINT ( 'NONE',  ( -24.22122181710478017, -12.92668648255967234, 62.71775301689540782 ) ) ;
#17649=EDGE_LOOP ( 'NONE', ( #34463, #711 ) ) ;
#17650=VERTEX_POINT ( 'NONE', #36643 ) ;
#17653=CARTESIAN_POINT ( 'NONE',  ( -13.65948078749761585, -20.77935321253323053, 58.20216925893738846 ) ) ;
#17654=EDGE_CURVE ( 'NONE', #42072, #20668, #10164, .T. ) ;
#17655=CARTESIAN_POINT ( 'NONE',  ( -10.56409641782382813, -13.17052685802803680, 75.09306420679733662 ) ) ;
#17656=CARTESIAN_POINT ( 'NONE',  ( -19.44376929052122449, -7.638105555415076076, 60.07597592072836790 ) ) ;
#17657=CARTESIAN_POINT ( 'NONE',  ( -14.94536187920032333, -8.261047438867105797, 60.50923257244761544 ) ) ;
#17658=CARTESIAN_POINT ( 'NONE',  ( -12.40319033546273531, -19.76959921888892424, 68.48090162751329046 ) ) ;
#17659=FACE_OUTER_BOUND ( 'NONE', #412, .T. ) ;
#17660=EDGE_LOOP ( 'NONE', ( #9639, #14887, #37465, #32060, #8098 ) ) ;
#17661=ORIENTED_EDGE ( 'NONE', *, *, #47603, .T. ) ;
#17662=CARTESIAN_POINT ( 'NONE',  ( -10.43098718212803000, -15.70539730037032911, 61.32316937334011442 ) ) ;
#17663=EDGE_CURVE ( 'NONE', #39613, #5898, #24966, .T. ) ;
#17664=DIRECTION ( 'NONE',  ( -0.05957303659011965041, -0.9982239494779875377, 2.515684304538401650E-08 ) ) ;
#17665=CARTESIAN_POINT ( 'NONE',  ( -14.54176566789882585, -21.67913831930545854, 58.28122448549703449 ) ) ;
#17670=CARTESIAN_POINT ( 'NONE',  ( -14.73375663737576247, -21.75657035701089370, 61.75105113489106401 ) ) ;
#17671=CARTESIAN_POINT ( 'NONE',  ( -19.94550508065608341, -21.39305643010487756, 72.41038500746213913 ) ) ;
#17672=CARTESIAN_POINT ( 'NONE',  ( -14.66963140629840190, -7.887024584555132556, 60.57642187187276051 ) ) ;
#17673=CARTESIAN_POINT ( 'NONE',  ( -10.08052694344373812, -16.06451652471636748, 68.09272548404199199 ) ) ;
#17676=FACE_OUTER_BOUND ( 'NONE', #32913, .T. ) ;
#17677=CARTESIAN_POINT ( 'NONE',  ( -12.73449705190429881, -9.612314979486423994, 74.51026123490949260 ) ) ;
#17680=EDGE_CURVE ( 'NONE', #37170, #5421, #3145, .T. ) ;
#17681=PLANE ( 'NONE',  #39313 ) ;
#17682=ORIENTED_EDGE ( 'NONE', *, *, #17076, .F. ) ;
#17684=ORIENTED_EDGE ( 'NONE', *, *, #31504, .F. ) ;
#17685=CARTESIAN_POINT ( 'NONE',  ( -24.37683822056718697, -15.97618770311995640, 66.06324926631656069 ) ) ;
#17686=CARTESIAN_POINT ( 'NONE',  ( -11.29385027892729987, -19.04286830487734861, 68.33194243210506613 ) ) ;
#17687=ORIENTED_EDGE ( 'NONE', *, *, #44169, .T. ) ;
#17688=EDGE_CURVE ( 'NONE', #7043, #43099, #12036, .T. ) ;
#17689=CARTESIAN_POINT ( 'NONE',  ( -13.69271718318762154, -21.25742183927064488, 68.55601500167955464 ) ) ;
#17691=VERTEX_POINT ( 'NONE', #41096 ) ;
#17692=LINE ( 'NONE', #7619, #21320 ) ;
#17694=CARTESIAN_POINT ( 'NONE',  ( -23.92640620196626600, -11.17277965375445703, 70.14856683682155847 ) ) ;
#17696=CARTESIAN_POINT ( 'NONE',  ( -13.46596743574567867, -21.12091133008686938, 65.10912019092907599 ) ) ;
#17697=CARTESIAN_POINT ( 'NONE',  ( -24.22177629109872399, -13.13842424187848934, 63.13264177643409880 ) ) ;
#17698=CARTESIAN_POINT ( 'NONE',  ( -11.40127056704611519, -11.24191079892443135, 60.67885781060143557 ) ) ;
#17699=DIRECTION ( 'NONE',  ( 7.381188785182666071E-06, 5.670466977913946987E-06, 0.9999999999566818731 ) ) ;
#17703=CARTESIAN_POINT ( 'NONE',  ( -23.38832489838272011, -10.34464890867069542, 59.78016211506488986 ) ) ;
#17704=CARTESIAN_POINT ( 'NONE',  ( -17.00708550189658652, -7.821638742870105965, 73.96018273346899718 ) ) ;
#17705=VERTEX_POINT ( 'NONE', #44808 ) ;
#17706=CARTESIAN_POINT ( 'NONE',  ( -11.43603398054886711, -11.08795246958514547, 57.50343388809581313 ) ) ;
#17708=EDGE_CURVE ( 'NONE', #46221, #14849, #40347, .T. ) ;
#17709=CARTESIAN_POINT ( 'NONE',  ( -13.95528965362524332, -21.40322351219866093, 72.03952346373179694 ) ) ;
#17710=CARTESIAN_POINT ( 'NONE',  ( -19.21257558972570223, -21.63231285022588679, 62.08683831298252898 ) ) ;
#17712=VERTEX_POINT ( 'NONE', #37884 ) ;
#17713=DIRECTION ( 'NONE',  ( 0.9968684284758858594, -0.07907803935364897396, 1.831731161803828584E-08 ) ) ;
#17717=ADVANCED_FACE ( 'NONE', ( #7379 ), #45540, .F. ) ;
#17718=EDGE_LOOP ( 'NONE', ( #42381, #40308 ) ) ;
#17719=ORIENTED_EDGE ( 'NONE', *, *, #36326, .T. ) ;
#17720=CARTESIAN_POINT ( 'NONE',  ( -20.66572514793045912, -8.604890110293021976, 59.84125219026921627 ) ) ;
#17721=CARTESIAN_POINT ( 'NONE',  ( -12.34589673948493171, -19.70464915359104907, 64.95854842562067688 ) ) ;
#17722=CARTESIAN_POINT ( 'NONE',  ( -10.72552571836178181, -12.61109718544098790, 60.79853568372239891 ) ) ;
#17724=ORIENTED_EDGE ( 'NONE', *, *, #9077, .F. ) ;
#17725=B_SPLINE_CURVE_WITH_KNOTS ( 'NONE', 3,
 ( #21458, #21926, #2723, #17729, #13311, #40630, #43390, #36212, #21215, #17971 ),
 .UNSPECIFIED., .F., .F.,
 ( 4, 2, 2, 2, 4 ),
 ( 0.6272669072877782304, 0.7522669073072908441, 0.8772669073268035689, 1.002266907346316183, 1.127266907365828796 ),
 .UNSPECIFIED. ) ;
#17726=CARTESIAN_POINT ( 'NONE',  ( -24.23259748711979356, -13.18308280478570005, 59.55370993033776728 ) ) ;
#17727=CARTESIAN_POINT ( 'NONE',  ( -12.56076107774658723, -9.694232635630330108, 74.47489936300191005 ) ) ;
#17729=CARTESIAN_POINT ( 'NONE',  ( -12.57238404326915315, -20.46304599113934941, 71.94507178006293202 ) ) ;
#17730=CARTESIAN_POINT ( 'NONE',  ( -21.96079975839714038, -8.899669644523443779, 66.83962766284624024 ) ) ;
#17731=EDGE_CURVE ( 'NONE', #30525, #46554, #45394, .T. ) ;
#17733=DIRECTION ( 'NONE',  ( 0.3688590060343601706, -0.9294853595766551235, 1.901466464867618399E-17 ) ) ;
#17736=LINE ( 'NONE', #32765, #25264 ) ;
#17737=CARTESIAN_POINT ( 'NONE',  ( -22.87929373774275632, -19.88409160966729772, 72.75745300618787326 ) ) ;
#17738=CARTESIAN_POINT ( 'NONE',  ( -19.35628891158445342, -21.53731772049657067, 58.75180642434932565 ) ) ;
#17739=ORIENTED_EDGE ( 'NONE', *, *, #42119, .F. ) ;
#17740=CARTESIAN_POINT ( 'NONE',  ( -24.14391077536845032, -18.02620038539897962, 59.16524916619123786 ) ) ;
#17741=CARTESIAN_POINT ( 'NONE',  ( -10.76270079184834749, -12.47665168726528506, 64.41269048358307714 ) ) ;
#17743=CARTESIAN_POINT ( 'NONE',  ( -10.56816478614453381, -13.15098976910933537, 74.76997804572182815 ) ) ;
#17744=CARTESIAN_POINT ( 'NONE',  ( -11.89179040387956832, -10.43929601004734486, 70.96893105543333036 ) ) ;
#17747=CARTESIAN_POINT ( 'NONE',  ( -16.90444465785252959, -22.24122871430926196, 72.32689728778339600 ) ) ;
#17748=CARTESIAN_POINT ( 'NONE',  ( -11.25989573505624364, -11.38792594226331012, 64.14882039369129529 ) ) ;
#17749=CARTESIAN_POINT ( 'NONE',  ( -22.64102959707144791, -20.12774700627143076, 69.28143819862634700 ) ) ;
#17750=CARTESIAN_POINT ( 'NONE',  ( -10.40277079310570052, -15.44444055846370745, 57.71792809063055785 ) ) ;
#17751=FACE_OUTER_BOUND ( 'NONE', #5106, .T. ) ;
#17752=CARTESIAN_POINT ( 'NONE',  ( -16.07865109465781117, -7.939724484389961034, 63.97011030347106697 ) ) ;
#17753=ORIENTED_EDGE ( 'NONE', *, *, #16821, .F. ) ;
#17754=VERTEX_POINT ( 'NONE', #29776 ) ;
#17755=EDGE_CURVE ( 'NONE', #34024, #22189, #1672, .T. ) ;
#17756=CARTESIAN_POINT ( 'NONE',  ( -19.09949158415725634, -8.012660229328147921, 63.43089235425713923 ) ) ;
#17757=CARTESIAN_POINT ( 'NONE',  ( -19.42896615819153538, -21.56812558881098241, 62.14503644571260565 ) ) ;
#17758=EDGE_LOOP ( 'NONE', ( #10567, #2074, #40116, #16200, #34489 ) ) ;
#17760=CARTESIAN_POINT ( 'NONE',  ( -14.37682202087475680, -19.38786730597468022, 54.07175714974878389 ) ) ;
#17763=EDGE_CURVE ( 'NONE', #25767, #19668, #6707, .T. ) ;
#17764=CARTESIAN_POINT ( 'NONE',  ( -22.04114742393716142, -9.481025248639415537, 59.73643293354757589 ) ) ;
#17767=FACE_BOUND ( 'NONE', #14596, .T. ) ;
#17768=CARTESIAN_POINT ( 'NONE',  ( -24.09792875595537964, -17.08130417324981565, 72.88336032035921619 ) ) ;
#17769=CARTESIAN_POINT ( 'NONE',  ( -24.27033155520888030, -13.12649183948492393, 62.98264177272948672 ) ) ;
#17770=EDGE_CURVE ( 'NONE', #22085, #12430, #44762, .T. ) ;
#17771=CARTESIAN_POINT ( 'NONE',  ( -20.75918656682226171, -8.147304802054664563, 63.42626204841099735 ) ) ;
#17772=ORIENTED_EDGE ( 'NONE', *, *, #45422, .F. ) ;
#17773=PLANE ( 'NONE',  #32925 ) ;
#17774=CARTESIAN_POINT ( 'NONE',  ( -10.21805405031902225, -12.91800167290361578, 67.78186406512817541 ) ) ;
#17776=CARTESIAN_POINT ( 'NONE',  ( -24.13185811504778755, -12.61356036044664464, 66.45813649863244166 ) ) ;
#17777=ADVANCED_FACE ( 'NONE', ( #45295 ), #23386, .T. ) ;
#17778=CARTESIAN_POINT ( 'NONE',  ( -11.10681587527927938, -11.67891925637714401, 71.10332952723315714 ) ) ;
#17779=CARTESIAN_POINT ( 'NONE',  ( -11.54449430114617137, -11.00967495709500810, 57.22519909113746905 ) ) ;
#17780=( BOUNDED_CURVE ( )  B_SPLINE_CURVE ( 3, ( #15538, #30598, #26901, #41910 ),
 .UNSPECIFIED., .F., .F. ) 
 B_SPLINE_CURVE_WITH_KNOTS ( ( 4, 4 ),
 ( 0.5000000000000000000, 0.9074455897393627346 ),
 .UNSPECIFIED. ) 
 CURVE ( )  GEOMETRIC_REPRESENTATION_ITEM ( )  RATIONAL_B_SPLINE_CURVE ( ( 1.000000000000048628, 0.4567392136813446801, 0.3561768502900010680, 0.6983129098260700829 ) ) 
 REPRESENTATION_ITEM ( '' )  );
#17781=EDGE_LOOP ( 'NONE', ( #42215, #25329, #8877, #16386, #28819 ) ) ;
#17783=ORIENTED_EDGE ( 'NONE', *, *, #35710, .F. ) ;
#17786=ORIENTED_EDGE ( 'NONE', *, *, #30655, .F. ) ;
#17787=CARTESIAN_POINT ( 'NONE',  ( -16.91855014848012928, -22.24212009645463439, 72.28047803099305213 ) ) ;
#17788=B_SPLINE_CURVE_WITH_KNOTS ( 'NONE', 3,
 ( #9234, #21035, #5548, #39747, #17325, #47391, #20567, #1839, #16836, #28668 ),
 .UNSPECIFIED., .F., .F.,
 ( 4, 2, 2, 2, 4 ),
 ( 0.000000000000000000, 0.2500000000000000000, 0.5000000000000000000, 0.7500000000000000000, 1.000000000000000000 ),
 .UNSPECIFIED. ) ;
#17789=CARTESIAN_POINT ( 'NONE',  ( -15.41904748403203484, -7.634001509309876532, 74.19490257054667381 ) ) ;
#17790=CARTESIAN_POINT ( 'NONE',  ( -16.26195973558533936, -21.76306465430365122, 58.57113428431811997 ) ) ;
#17791=EDGE_LOOP ( 'NONE', ( #10260, #44693, #22601, #43081, #40415 ) ) ;
#17792=CARTESIAN_POINT ( 'NONE',  ( -10.99197923738610250, -11.04991372156584006, 60.85602641044604155 ) ) ;
#17794=ORIENTED_EDGE ( 'NONE', *, *, #48333, .F. ) ;
#17795=DIRECTION ( 'NONE',  ( -0.09077643883959130022, 0.9958712959773466933, 4.338678762321648003E-08 ) ) ;
#17799=CARTESIAN_POINT ( 'NONE',  ( -17.79929111768229433, -7.368650117109674547, 60.18037143928950172 ) ) ;
#17800=CARTESIAN_POINT ( 'NONE',  ( -21.23484681875272884, -20.74088929683185611, 69.33978048267414351 ) ) ;
#17802=ORIENTED_EDGE ( 'NONE', *, *, #42402, .T. ) ;
#17803=CARTESIAN_POINT ( 'NONE',  ( -10.70297003644833644, -11.59513240183115279, 71.27356180636090244 ) ) ;
#17804=CARTESIAN_POINT ( 'NONE',  ( -24.41897112398753933, -17.37347453850100720, 69.59835118672229726 ) ) ;
#17806=ORIENTED_EDGE ( 'NONE', *, *, #4444, .F. ) ;
#17807=DIRECTION ( 'NONE',  ( -0.5589780652556125551, 0.8291824422665291516, -7.938832475108110126E-08 ) ) ;
#17812=CARTESIAN_POINT ( 'NONE',  ( -11.70966707598573819, -10.02926654750783975, 67.64896868923555928 ) ) ;
#17814=CARTESIAN_POINT ( 'NONE',  ( -16.64258257546838138, -22.21885596081591174, 68.88215988439684168 ) ) ;
#17816=ORIENTED_EDGE ( 'NONE', *, *, #2791, .F. ) ;
#17817=CARTESIAN_POINT ( 'NONE',  ( -17.74348949963705024, -22.25235684858374796, 58.55553378380137985 ) ) ;
#17819=DIRECTION ( 'NONE',  ( -0.9048399035850771543, -0.4257519804770707461, -1.330923645920820637E-08 ) ) ;
#17821=ORIENTED_EDGE ( 'NONE', *, *, #34271, .F. ) ;
#17822=DIRECTION ( 'NONE',  ( 0.9562635972186038780, -0.2925062950340272527, 4.666065131241567634E-08 ) ) ;
#17823=B_SPLINE_CURVE_WITH_KNOTS ( 'NONE', 3,
 ( #37521, #11944, #26223, #44958, #139, #4078, #26716, #607, #41236, #38513 ),
 .UNSPECIFIED., .F., .F.,
 ( 4, 2, 2, 2, 4 ),
 ( 0.000000000000000000, 0.2500000000000000000, 0.5000000000000000000, 0.7500000000000000000, 1.000000000000000000 ),
 .UNSPECIFIED. ) ;
#17824=EDGE_CURVE ( 'NONE', #12655, #39442, #23615, .T. ) ;
#17826=ORIENTED_EDGE ( 'NONE', *, *, #43874, .T. ) ;
#17828=EDGE_CURVE ( 'NONE', #31288, #34613, #42575, .T. ) ;
#17829=CARTESIAN_POINT ( 'NONE',  ( -13.96006829630253776, -20.89348458149306964, 72.15437620276698283 ) ) ;
#17830=CARTESIAN_POINT ( 'NONE',  ( -22.66727079836811853, -10.09628861529951216, 70.16178520457069112 ) ) ;
#17831=DIRECTION ( 'NONE',  ( 0.8083598999316397027, 0.5886886037477749856, 6.671815825018552065E-08 ) ) ;
#17832=ORIENTED_EDGE ( 'NONE', *, *, #24330, .T. ) ;
#17841=ORIENTED_EDGE ( 'NONE', *, *, #40832, .T. ) ;
#17842=ADVANCED_FACE ( 'NONE', ( #39094 ), #35019, .T. ) ;
#17843=EDGE_CURVE ( 'NONE', #35459, #41905, #43619, .T. ) ;
#17846=CARTESIAN_POINT ( 'NONE',  ( -12.55198883488284878, -12.25722835735234639, 53.49899999999994549 ) ) ;
#17847=( BOUNDED_CURVE ( )  B_SPLINE_CURVE ( 3, ( #24157, #31294, #17231, #27602 ),
 .UNSPECIFIED., .F., .F. ) 
 B_SPLINE_CURVE_WITH_KNOTS ( ( 4, 4 ),
 ( 0.000000000000000000, 0.4074455897393622905 ),
 .UNSPECIFIED. ) 
 CURVE ( )  GEOMETRIC_REPRESENTATION_ITEM ( )  RATIONAL_B_SPLINE_CURVE ( ( 1.000000000000000000, 0.4567392136813342995, 0.3561768502900312106, 0.6983129098260907330 ) ) 
 REPRESENTATION_ITEM ( '' )  );
#17849=EDGE_LOOP ( 'NONE', ( #12554, #41617, #18868, #36453 ) ) ;
#17851=ORIENTED_EDGE ( 'NONE', *, *, #16638, .T. ) ;
#17852=CARTESIAN_POINT ( 'NONE',  ( -14.48548941065489970, -8.400516866317895293, 67.27447142263336843 ) ) ;
#17853=CARTESIAN_POINT ( 'NONE',  ( -19.52605052145376874, -21.48662438560833365, 65.48102853648620680 ) ) ;
#17854=CARTESIAN_POINT ( 'NONE',  ( -10.39890676938329150, -12.32907080782536191, 57.45044596432388317 ) ) ;
#17855=VERTEX_POINT ( 'NONE', #9316 ) ;
#17856=FACE_OUTER_BOUND ( 'NONE', #32643, .T. ) ;
#17858=CARTESIAN_POINT ( 'NONE',  ( -18.03604760049577393, -21.78284572725946333, 65.36148796969293073 ) ) ;
#17860=CARTESIAN_POINT ( 'NONE',  ( -24.83347472307691817, -15.58731732267899694, 73.18020620047872171 ) ) ;
#17864=CARTESIAN_POINT ( 'NONE',  ( -13.37636250268599092, -20.58507941322447365, 61.93135214938352107 ) ) ;
#17865=EDGE_LOOP ( 'NONE', ( #15154, #6137, #42023, #7520, #354 ) ) ;
#17866=CARTESIAN_POINT ( 'NONE',  ( -13.18362795047878144, -8.683667697493742565, 60.62445659250467145 ) ) ;
#17867=DIRECTION ( 'NONE',  ( -0.06357898915123239014, 0.9979768094191906469, 2.064515410283096215E-19 ) ) ;
#17868=EDGE_CURVE ( 'NONE', #21243, #39081, #1914, .T. ) ;
#17870=ORIENTED_EDGE ( 'NONE', *, *, #44515, .F. ) ;
#17871=CARTESIAN_POINT ( 'NONE',  ( -22.09234465700630423, -20.09219189623108548, 62.23439162498055310 ) ) ;
#17872=CARTESIAN_POINT ( 'NONE',  ( -10.92672688430831229, -11.16395088679539249, 64.40527978002718612 ) ) ;
#17875=CARTESIAN_POINT ( 'NONE',  ( -23.73621606195537481, -11.66110265205040974, 59.69055757226052350 ) ) ;
#17878=CARTESIAN_POINT ( 'NONE',  ( -24.76903642440577258, -16.05600587708614668, 66.16350687787337392 ) ) ;
#17879=ORIENTED_EDGE ( 'NONE', *, *, #39631, .F. ) ;
#17882=CARTESIAN_POINT ( 'NONE',  ( -19.41474593944376537, -21.52019035999878938, 61.99503644832097393 ) ) ;
#17885=CARTESIAN_POINT ( 'NONE',  ( -23.92640620196626600, -11.17277965375445703, 70.14856683682155847 ) ) ;
#17886=CARTESIAN_POINT ( 'NONE',  ( -12.29927561225700750, -19.57981844400423910, 61.58605613336224849 ) ) ;
#17891=ORIENTED_EDGE ( 'NONE', *, *, #45634, .F. ) ;
#17892=CARTESIAN_POINT ( 'NONE',  ( -19.42896615819153538, -21.56812558881098241, 62.14503644571260565 ) ) ;
#17894=CARTESIAN_POINT ( 'NONE',  ( -10.38078070663892660, -14.50222156296673148, 67.85800126083267969 ) ) ;
#17895=CARTESIAN_POINT ( 'NONE',  ( -19.01896746559008733, -7.531908412828363097, 67.00097544457088361 ) ) ;
#17898=( BOUNDED_CURVE ( )  B_SPLINE_CURVE ( 3, ( #4015, #7962, #37967, #11884 ),
 .UNSPECIFIED., .F., .F. ) 
 B_SPLINE_CURVE_WITH_KNOTS ( ( 4, 4 ),
 ( 4.712388980384689674, 4.921828490624008623 ),
 .UNSPECIFIED. ) 
 CURVE ( )  GEOMETRIC_REPRESENTATION_ITEM ( )  RATIONAL_B_SPLINE_CURVE ( ( 1.000000000000000000, 0.9963479302455156006, 0.9963479302455156006, 1.000000000000000000 ) ) 
 REPRESENTATION_ITEM ( '' )  );
#17900=EDGE_LOOP ( 'NONE', ( #43825, #44999 ) ) ;
#17901=EDGE_CURVE ( 'NONE', #15165, #26529, #18620, .T. ) ;
#17902=ADVANCED_FACE ( 'NONE', ( #17153 ), #36588, .T. ) ;
#17903=CARTESIAN_POINT ( 'NONE',  ( -22.37985696210566999, -19.82347738784875801, 69.32417989525721680 ) ) ;
#17904=CARTESIAN_POINT ( 'NONE',  ( -11.96181355942711910, -19.87549434724351727, 58.11177690156993947 ) ) ;
#17906=CARTESIAN_POINT ( 'NONE',  ( -10.09263637371726041, -16.13336529236863015, 68.02121877882343881 ) ) ;
#17908=ORIENTED_EDGE ( 'NONE', *, *, #36170, .F. ) ;
#17909=( BOUNDED_CURVE ( )  B_SPLINE_CURVE ( 3, ( #712, #7624, #48724, #7377 ),
 .UNSPECIFIED., .F., .F. ) 
 B_SPLINE_CURVE_WITH_KNOTS ( ( 4, 4 ),
 ( 0.4074455897393636228, 0.5000000000000000000 ),
 .UNSPECIFIED. ) 
 CURVE ( )  GEOMETRIC_REPRESENTATION_ITEM ( )  RATIONAL_B_SPLINE_CURVE ( ( 0.6983129098260894008, 0.7760317562606912078, 0.8765941196519937417, 0.9999999999999938938 ) ) 
 REPRESENTATION_ITEM ( '' )  );
#17912=ADVANCED_FACE ( 'NONE', ( #10282 ), #2943, .T. ) ;
#17913=B_SPLINE_CURVE_WITH_KNOTS ( 'NONE', 3,
 ( #33384, #425, #4353, #14654, #19361, #44759, #26033, #41050, #14917, #29974 ),
 .UNSPECIFIED., .F., .F.,
 ( 4, 2, 2, 2, 4 ),
 ( 0.000000000000000000, 0.2500000000000000000, 0.5000000000000000000, 0.7500000000000000000, 1.000000000000000000 ),
 .UNSPECIFIED. ) ;
#17914=CARTESIAN_POINT ( 'NONE',  ( -22.18998830427770841, -20.00468049915955859, 65.71893796558269685 ) ) ;
#17915=CARTESIAN_POINT ( 'NONE',  ( -12.74558454090558257, -9.602248860578644241, 74.54596281605876129 ) ) ;
#17917=CARTESIAN_POINT ( 'NONE',  ( -17.19980212172655953, -7.762775302065858085, 70.79035839668003405 ) ) ;
#17918=DIRECTION ( 'NONE',  ( -0.7489133456531319455, -0.6626679415081375701, 6.686399169904807035E-09 ) ) ;
#17921=( BOUNDED_CURVE ( )  B_SPLINE_CURVE ( 3, ( #46464, #42995, #42526, #9270 ),
 .UNSPECIFIED., .F., .F. ) 
 B_SPLINE_CURVE_WITH_KNOTS ( ( 4, 4 ),
 ( 0.5000000000000000000, 0.9074455897393698400 ),
 .UNSPECIFIED. ) 
 CURVE ( )  GEOMETRIC_REPRESENTATION_ITEM ( )  RATIONAL_B_SPLINE_CURVE ( ( 1.000000000000002220, 0.4567392136813248626, 0.3561768502900259925, 0.6983129098261080525 ) ) 
 REPRESENTATION_ITEM ( '' )  );
#17923=DIRECTION ( 'NONE',  ( 0.8398192074808118468, 0.5428661886195297326, 7.907900705247677662E-08 ) ) ;
#17926=ADVANCED_FACE ( 'NONE', ( #44031 ), #45124, .T. ) ;
#17928=ORIENTED_EDGE ( 'NONE', *, *, #8995, .T. ) ;
#17932=CARTESIAN_POINT ( 'NONE',  ( -24.86169257816691314, -14.37661386440606037, 66.34326115264040880 ) ) ;
#17933=EDGE_LOOP ( 'NONE', ( #42088, #21983, #46711, #42133, #43217 ) ) ;
#17944=CARTESIAN_POINT ( 'NONE',  ( -24.12000719736520438, -11.54295319193055214, 63.20864192093194589 ) ) ;
#17946=LINE ( 'NONE', #25841, #44806 ) ;
#17947=CARTESIAN_POINT ( 'NONE',  ( -23.66547331395526044, -18.87718802671421159, 69.40097851167932674 ) ) ;
#17950=CARTESIAN_POINT ( 'NONE',  ( -14.76438121721707830, -8.332445897900056409, 63.90051825552988873 ) ) ;
#17951=ORIENTED_EDGE ( 'NONE', *, *, #25702, .T. ) ;
#17952=CARTESIAN_POINT ( 'NONE',  ( -20.81971067820157728, -8.177204663279967534, 59.95469905373763453 ) ) ;
#17953=CARTESIAN_POINT ( 'NONE',  ( -13.46747890590686403, -9.034676489092227314, 60.43950277890026967 ) ) ;
#17954=CARTESIAN_POINT ( 'NONE',  ( -24.05845762361657947, -12.57644656616312773, 73.24225570276865938 ) ) ;
#17955=CARTESIAN_POINT ( 'NONE',  ( -13.49987067987283673, -9.012482076563856026, 60.73950329009904436 ) ) ;
#17956=VERTEX_POINT ( 'NONE', #36116 ) ;
#17958=EDGE_CURVE ( 'NONE', #42977, #36746, #23652, .T. ) ;
#17959=CYLINDRICAL_SURFACE ( 'NONE', #26477, 0.1499999999999953038 ) ;
#17960=CARTESIAN_POINT ( 'NONE',  ( -19.67760665824181388, -21.48965406232008490, 65.75014118398131302 ) ) ;
#17961=CARTESIAN_POINT ( 'NONE',  ( -23.31260078967427063, -19.37299621621055579, 58.98436398315890727 ) ) ;
#17963=EDGE_LOOP ( 'NONE', ( #41774, #27313 ) ) ;
#17966=CARTESIAN_POINT ( 'NONE',  ( -23.81432972337535858, -17.66677937220956451, 59.07666504472891233 ) ) ;
#17967=ORIENTED_EDGE ( 'NONE', *, *, #19086, .T. ) ;
#17968=EDGE_CURVE ( 'NONE', #39713, #24660, #6821, .T. ) ;
#17969=CARTESIAN_POINT ( 'NONE',  ( -13.65852477070391480, -21.23755994396627145, 68.64963458044397271 ) ) ;
#17971=CARTESIAN_POINT ( 'NONE',  ( -12.50776634899986384, -20.40684016789016297, 71.92158251742569064 ) ) ;
#17974=EDGE_LOOP ( 'NONE', ( #36735, #15817, #5726, #1952, #34356 ) ) ;
#17975=CARTESIAN_POINT ( 'NONE',  ( -11.86969123986252406, -10.46139627614129708, 67.49896775950338679 ) ) ;
#17978=CARTESIAN_POINT ( 'NONE',  ( -19.75048190521760461, -21.47275536819973141, 62.15070614013394135 ) ) ;
#17979=DIRECTION ( 'NONE',  ( -0.3478314405900309603, -0.9375570856950864451, 9.567072274253696421E-17 ) ) ;
#17980=ORIENTED_EDGE ( 'NONE', *, *, #40896, .T. ) ;
#17981=CARTESIAN_POINT ( 'NONE',  ( -24.43392429566424440, -14.02363658386207668, 69.65275204483315008 ) ) ;
#17982=CARTESIAN_POINT ( 'NONE',  ( -24.49584582974870628, -12.46528025919705485, 73.49871492906470394 ) ) ;
#17983=EDGE_CURVE ( 'NONE', #45657, #45009, #16462, .T. ) ;
#17984=DIRECTION ( 'NONE',  ( 0.9477661110324760996, -0.3189661404888857188, 2.738326501554841424E-08 ) ) ;
#17986=B_SPLINE_CURVE_WITH_KNOTS ( 'NONE', 3,
 ( #6910, #45092, #26356, #30069, #48509, #3453, #21927, #29816, #7910, #273 ),
 .UNSPECIFIED., .F., .F.,
 ( 4, 2, 2, 2, 4 ),
 ( 0.000000000000000000, 0.2500000000000000000, 0.5000000000000000000, 0.7500000000000000000, 1.000000000000000000 ),
 .UNSPECIFIED. ) ;
#17988=DIRECTION ( 'NONE',  ( -4.133538128552115272E-06, 2.214839418041148178E-07, -0.9999999999914322979 ) ) ;
#17991=CARTESIAN_POINT ( 'NONE',  ( -16.90422089642926906, -22.24121457338818431, 72.30509853249346008 ) ) ;
#17993=DIRECTION ( 'NONE',  ( 2.699622411496199987E-06, -1.161037829314838553E-05, -0.9999999999289554964 ) ) ;
#17994=PLANE ( 'NONE',  #11651 ) ;
#17995=CARTESIAN_POINT ( 'NONE',  ( -13.54823245630066175, -20.69819609872914157, 61.81646323537678001 ) ) ;
#17997=EDGE_LOOP ( 'NONE', ( #46877, #34385, #46129, #6074, #45023 ) ) ;
#17999=CARTESIAN_POINT ( 'NONE',  ( -11.06796828401846078, -18.69550736580278993, 61.53356777548469125 ) ) ;
#18000=CARTESIAN_POINT ( 'NONE',  ( -11.03230881600246427, -10.98182333549695322, 60.79390388117851529 ) ) ;
#18002=CARTESIAN_POINT ( 'NONE',  ( -15.35852799358099929, -7.651226727379689230, 74.18647339208507674 ) ) ;
#18004=CARTESIAN_POINT ( 'NONE',  ( -14.01837044221388417, -8.636059239884620098, 74.48482605064899076 ) ) ;
#18005=CARTESIAN_POINT ( 'NONE',  ( -12.44869005970189058, -9.885249076858732664, 57.08935532200567309 ) ) ;
#18006=CARTESIAN_POINT ( 'NONE',  ( -12.05727448861903639, -19.97649948735875114, 61.65324539733175868 ) ) ;
#18007=CARTESIAN_POINT ( 'NONE',  ( -22.07241914523459769, -20.11453564365663027, 65.79601743996857977 ) ) ;
#18008=CARTESIAN_POINT ( 'NONE',  ( -23.91439714532632621, -17.43141235356291574, 65.94357239632037704 ) ) ;
#18009=CARTESIAN_POINT ( 'NONE',  ( -12.64995474452274138, -19.99670071527213366, 68.63657438322856308 ) ) ;
#18011=ORIENTED_EDGE ( 'NONE', *, *, #25091, .T. ) ;
#18013=CARTESIAN_POINT ( 'NONE',  ( -11.60439305645412844, -10.15781863991614031, 71.14705871384585123 ) ) ;
#18014=CARTESIAN_POINT ( 'NONE',  ( -16.91855125566938511, -22.24212016642244905, 72.28047911973106920 ) ) ;
#18015=CARTESIAN_POINT ( 'NONE',  ( -15.28291064399146215, -21.52618758091310980, 68.57592918174772478 ) ) ;
#18016=CARTESIAN_POINT ( 'NONE',  ( -24.61562913124599916, -12.86357381044341430, 66.55892682786348757 ) ) ;
#18018=DIRECTION ( 'NONE',  ( -2.430360958779124298E-06, -9.751098539734333949E-07, 0.9999999999965712982 ) ) ;
#18019=CYLINDRICAL_SURFACE ( 'NONE', #40127, 0.1500000000000047407 ) ;
#18022=VERTEX_POINT ( 'NONE', #37085 ) ;
#18023=ORIENTED_EDGE ( 'NONE', *, *, #33642, .T. ) ;
#18026=CARTESIAN_POINT ( 'NONE',  ( -23.54173688680538135, -19.06112029705675681, 66.00202217072055078 ) ) ;
#18027=CARTESIAN_POINT ( 'NONE',  ( -20.06397283958904865, -8.325598795413901243, 74.00479983096190040 ) ) ;
#18030=FACE_OUTER_BOUND ( 'NONE', #46562, .T. ) ;
#18031=ORIENTED_EDGE ( 'NONE', *, *, #9992, .T. ) ;
#18034=CARTESIAN_POINT ( 'NONE',  ( -13.76849323099554567, -20.83774554052356365, 65.27156739751333703 ) ) ;
#18035=CARTESIAN_POINT ( 'NONE',  ( -21.00520398765801744, -21.34214743040633167, 62.37117330845665464 ) ) ;
#18036=EDGE_CURVE ( 'NONE', #23317, #6093, #7159, .T. ) ;
#18037=( BOUNDED_CURVE ( )  B_SPLINE_CURVE ( 3, ( #46024, #19424, #26095, #19187 ),
 .UNSPECIFIED., .F., .F. ) 
 B_SPLINE_CURVE_WITH_KNOTS ( ( 4, 4 ),
 ( 0.000000000000000000, 0.4074455897393680082 ),
 .UNSPECIFIED. ) 
 CURVE ( )  GEOMETRIC_REPRESENTATION_ITEM ( )  RATIONAL_B_SPLINE_CURVE ( ( 1.000000000000000000, 0.4567392136813361314, 0.3561768502900318767, 0.6983129098260871803 ) ) 
 REPRESENTATION_ITEM ( '' )  );
#18038=EDGE_LOOP ( 'NONE', ( #39339, #33879, #21411, #48516, #47409 ) ) ;
#18039=CARTESIAN_POINT ( 'NONE',  ( -18.50932193227059841, -21.77517953109191495, 72.58510940649489385 ) ) ;
#18041=ORIENTED_EDGE ( 'NONE', *, *, #38886, .T. ) ;
#18042=ADVANCED_FACE ( 'NONE', ( #18612 ), #26509, .T. ) ;
#18043=CARTESIAN_POINT ( 'NONE',  ( -23.00441930688031889, -19.11762475274336737, 59.03410642058399560 ) ) ;
#18045=DIRECTION ( 'NONE',  ( -0.4251432040024066272, -0.9051260995521939190, -1.185120001106687566E-09 ) ) ;
#18046=ORIENTED_EDGE ( 'NONE', *, *, #12128, .T. ) ;
#18047=CARTESIAN_POINT ( 'NONE',  ( -10.98892314574976226, -11.92244160250971419, 70.97372176798174337 ) ) ;
#18048=CARTESIAN_POINT ( 'NONE',  ( -23.38668188022877814, -18.47650611194418957, 72.76368285100856781 ) ) ;
#18049=AXIS2_PLACEMENT_3D ( 'NONE', #27446, #42231, #11283 ) ;
#18050=EDGE_CURVE ( 'NONE', #48039, #4198, #18927, .T. ) ;
#18051=( BOUNDED_SURFACE ( )  B_SPLINE_SURFACE ( 3, 1, ( 
 ( #24094, #43042 ),
 ( #32448, #16442 ),
 ( #2405, #12515 ),
 ( #20644, #46511 ),
 ( #27540, #42583 ),
 ( #8845, #23861 ),
 ( #5141, #31475 ) ),
 .UNSPECIFIED., .T., .F., .F. ) 
 B_SPLINE_SURFACE_WITH_KNOTS ( ( 4, 3, 4 ),
 ( 2, 2 ),
 ( 0.000000000000000000, 0.5000000000000000000, 1.000000000000000000 ),
 ( 0.000000000000000000, 1.000000000000000000 ),
 .UNSPECIFIED. ) 
 GEOMETRIC_REPRESENTATION_ITEM ( )  RATIONAL_B_SPLINE_SURFACE ( (
 ( 1.000000000000000000, 1.000000000000000000),
 ( 0.3333333333333335369, 0.3333333333333330373),
 ( 0.3333333333333335369, 0.3333333333333330373),
 ( 1.000000000000000000, 1.000000000000000000),
 ( 0.3333333333333333703, 0.3333333333333333703),
 ( 0.3333333333333333703, 0.3333333333333333703),
 ( 1.000000000000000000, 1.000000000000000000) ) ) 
 REPRESENTATION_ITEM ( '' )  SURFACE ( )  );
#18052=CARTESIAN_POINT ( 'NONE',  ( -14.01837044221388417, -8.636059239884620098, 74.48482605064899076 ) ) ;
#18053=CARTESIAN_POINT ( 'NONE',  ( -12.22871965896205460, -20.14873714605892019, 65.01674887276816150 ) ) ;
#18054=EDGE_LOOP ( 'NONE', ( #161, #6123 ) ) ;
#18055=CARTESIAN_POINT ( 'NONE',  ( -13.88293547364789404, -20.90532801101632998, 68.75625136993008368 ) ) ;
#18057=CARTESIAN_POINT ( 'NONE',  ( -10.72769102952926978, -12.77004266858777726, 60.98956792496692714 ) ) ;
#18058=CARTESIAN_POINT ( 'NONE',  ( -23.16275847746607752, -18.91806288495012112, 69.43805163930900903 ) ) ;
#18059=CARTESIAN_POINT ( 'NONE',  ( -11.47236147394688111, -10.32806163424019985, 74.55389795262664165 ) ) ;
#18060=LINE ( 'NONE', #14585, #6251 ) ;
#18061=DIRECTION ( 'NONE',  ( -0.07061531369766042843, -0.9975036227860933913, -1.268851337311104735E-08 ) ) ;
#18066=CARTESIAN_POINT ( 'NONE',  ( -18.59601872632196873, -7.856991649524070809, 73.85536540707786912 ) ) ;
#18067=ORIENTED_EDGE ( 'NONE', *, *, #25606, .F. ) ;
#18069=( BOUNDED_CURVE ( )  B_SPLINE_CURVE ( 3, ( #8163, #15505, #45597, #38166 ),
 .UNSPECIFIED., .F., .F. ) 
 B_SPLINE_CURVE_WITH_KNOTS ( ( 4, 4 ),
 ( 0.000000000000000000, 0.4074455897393648440 ),
 .UNSPECIFIED. ) 
 CURVE ( )  GEOMETRIC_REPRESENTATION_ITEM ( )  RATIONAL_B_SPLINE_CURVE ( ( 1.000000000000000000, 0.4567392136813316905, 0.3561768502900302114, 0.6983129098260953960 ) ) 
 REPRESENTATION_ITEM ( '' )  );
#18070=ORIENTED_EDGE ( 'NONE', *, *, #24031, .F. ) ;
#18071=ORIENTED_EDGE ( 'NONE', *, *, #20670, .F. ) ;
#18072=ORIENTED_EDGE ( 'NONE', *, *, #30419, .F. ) ;
#18073=CARTESIAN_POINT ( 'NONE',  ( -22.37985709289073455, -19.82347726015160205, 69.17417989525732480 ) ) ;
#18075=FACE_OUTER_BOUND ( 'NONE', #12890, .T. ) ;
#18076=ORIENTED_EDGE ( 'NONE', *, *, #429, .F. ) ;
#18080=B_SPLINE_CURVE_WITH_KNOTS ( 'NONE', 1,
 ( #8300, #20346 ),
 .UNSPECIFIED., .F., .F.,
 ( 2, 2 ),
 ( 0.000000000000000000, 1.000000000000000000 ),
 .UNSPECIFIED. ) ;
#18081=CARTESIAN_POINT ( 'NONE',  ( -10.86589828222802545, -17.25666868831298828, 61.34846333097007687 ) ) ;
#18087=DIRECTION ( 'NONE',  ( 1.277734862359329272E-05, 2.482875502418557358E-06, 0.9999999999152874297 ) ) ;
#18088=EDGE_CURVE ( 'NONE', #12513, #20130, #19542, .T. ) ;
#18089=FACE_OUTER_BOUND ( 'NONE', #4582, .T. ) ;
#18090=AXIS2_PLACEMENT_3D ( 'NONE', #30256, #26545, #41821 ) ;
#18091=FACE_OUTER_BOUND ( 'NONE', #28266, .T. ) ;
#18093=FACE_OUTER_BOUND ( 'NONE', #27330, .T. ) ;
#18094=VERTEX_POINT ( 'NONE', #26761 ) ;
#18095=EDGE_CURVE ( 'NONE', #42959, #34898, #4803, .T. ) ;
#18097=CARTESIAN_POINT ( 'NONE',  ( -15.22116837037893866, -21.50650591823945845, 68.59065000974109694 ) ) ;
#18099=VERTEX_POINT ( 'NONE', #4348 ) ;
#18100=CARTESIAN_POINT ( 'NONE',  ( -14.79207564484453563, -7.839496205118279271, 57.02716913942106913 ) ) ;
#18102=EDGE_CURVE ( 'NONE', #26191, #39816, #35908, .T. ) ;
#18103=DIRECTION ( 'NONE',  ( -1.896855589470121649E-06, -2.136244919983285370E-06, -0.9999999999959192643 ) ) ;
#18104=CARTESIAN_POINT ( 'NONE',  ( -19.82546683696349277, -21.43766614373956259, 69.23482471120810544 ) ) ;
#18106=CARTESIAN_POINT ( 'NONE',  ( -17.42409385541300892, -14.80920654474439502, 75.49999999999994316 ) ) ;
#18107=CARTESIAN_POINT ( 'NONE',  ( -21.38384743419493361, -20.64229702430353086, 72.81886605551670755 ) ) ;
#18108=CARTESIAN_POINT ( 'NONE',  ( -21.50786275526073510, -9.062390040748779185, 70.43132511361099546 ) ) ;
#18109=EDGE_LOOP ( 'NONE', ( #24543, #7926, #19769, #43075 ) ) ;
#18110=FACE_BOUND ( 'NONE', #42430, .T. ) ;
#18111=VERTEX_POINT ( 'NONE', #42511 ) ;
#18112=DIRECTION ( 'NONE',  ( 2.662580029140978055E-06, -1.091441817711415488E-05, 0.9999999999368930359 ) ) ;
#18113=CARTESIAN_POINT ( 'NONE',  ( -11.45752044641470668, -19.27057170535650954, 71.87181270239314301 ) ) ;
#18114=CARTESIAN_POINT ( 'NONE',  ( -13.11945872550529835, -9.225962324091906197, 67.67942785705487552 ) ) ;
#18116=CARTESIAN_POINT ( 'NONE',  ( -22.63008487438422733, -10.12971324841507581, 70.31178520543817001 ) ) ;
#18118=DIRECTION ( 'NONE',  ( 0.09855345062332551698, 0.9951317587989213509, 3.188559572831062401E-08 ) ) ;
#18120=CARTESIAN_POINT ( 'NONE',  ( -10.92750371411227128, -11.16255126880030701, 64.26386748351472988 ) ) ;
#18121=CARTESIAN_POINT ( 'NONE',  ( -23.34440357289541979, -18.54427947304066038, 69.30874357600073665 ) ) ;
#18122=EDGE_CURVE ( 'NONE', #41418, #30144, #31583, .T. ) ;
#18123=ORIENTED_EDGE ( 'NONE', *, *, #2846, .F. ) ;
#18126=EDGE_CURVE ( 'NONE', #39502, #22557, #33543, .T. ) ;
#18127=CARTESIAN_POINT ( 'NONE',  ( -24.65023673758593148, -12.99629830290576038, 63.01759453279318279 ) ) ;
#18128=ADVANCED_FACE ( 'NONE', ( #12702, #27720, #8784, #23557, #17538, #35094, #9923, #24940, #8527, #38552, #45955, #12453, #19859, #34859, #36250, #19606, #46683, #12929, #1362, #39957, #12217, #15898, #42750, #1126, #45735, #34612, #43670, #16128, #23305, #24041, #2533, #31174, #39037, #30944, #23800, #38802, #5318, #16627, #26994, #31663, #38295, #4587, #46195, #27477, #5081, #20090, #10644, #44165, #41165, #29355, #25904, #2759, #3739, #17767, #7449, #44386, #22213, #47595, #25652, #6475, #32563, #40666, #33261, #18253, #6949, #10415, #32796, #22455, #21966, #37201, #13828 ), #44880, .T. ) ;
#18129=ORIENTED_EDGE ( 'NONE', *, *, #24223, .T. ) ;
#18130=ORIENTED_EDGE ( 'NONE', *, *, #4779, .T. ) ;
#18131=CARTESIAN_POINT ( 'NONE',  ( -14.90123591195245112, -21.39555782113924209, 65.52085318447059592 ) ) ;
#18133=AXIS2_PLACEMENT_3D ( 'NONE', #41064, #10538, #14426 ) ;
#18134=CARTESIAN_POINT ( 'NONE',  ( -10.50893933415051507, -13.43540278197274063, 74.96345540680638919 ) ) ;
#18135=DIRECTION ( 'NONE',  ( -0.3478314405900307937, -0.9375570856950865561, 0.000000000000000000 ) ) ;
#18137=FACE_OUTER_BOUND ( 'NONE', #17718, .T. ) ;
#18139=VERTEX_POINT ( 'NONE', #14782 ) ;
#18140=ORIENTED_EDGE ( 'NONE', *, *, #38869, .T. ) ;
#18141=B_SPLINE_CURVE_WITH_KNOTS ( 'NONE', 1,
 ( #2192, #24619 ),
 .UNSPECIFIED., .F., .F.,
 ( 2, 2 ),
 ( 0.000000000000000000, 1.000000000000000000 ),
 .UNSPECIFIED. ) ;
#18144=LINE ( 'NONE', #47487, #8706 ) ;
#18145=CARTESIAN_POINT ( 'NONE',  ( -21.87050228503520799, -9.402212662412775757, 63.47537209186675256 ) ) ;
#18146=CARTESIAN_POINT ( 'NONE',  ( -12.46122051107220230, -19.81685944811288635, 64.88146935704573082 ) ) ;
#18147=( BOUNDED_CURVE ( )  B_SPLINE_CURVE ( 3, ( #5807, #2095, #32146, #29653 ),
 .UNSPECIFIED., .F., .F. ) 
 B_SPLINE_CURVE_WITH_KNOTS ( ( 4, 4 ),
 ( 0.5000000000000000000, 0.9074455897393565174 ),
 .UNSPECIFIED. ) 
 CURVE ( )  GEOMETRIC_REPRESENTATION_ITEM ( )  RATIONAL_B_SPLINE_CURVE ( ( 1.000000000000062395, 0.4567392136813611669, 0.3561768502899974043, 0.6983129098260387746 ) ) 
 REPRESENTATION_ITEM ( '' )  );
#18148=CARTESIAN_POINT ( 'NONE',  ( -24.40591063191072152, -15.81373627858385866, 73.30303958064588699 ) ) ;
#18151=ORIENTED_EDGE ( 'NONE', *, *, #48000, .T. ) ;
#18152=VECTOR ( 'NONE', #15671, 1000.000000000000114 ) ;
#18154=FACE_OUTER_BOUND ( 'NONE', #36156, .T. ) ;
#18155=VECTOR ( 'NONE', #24809, 1000.000000000000227 ) ;
#18156=CARTESIAN_POINT ( 'NONE',  ( -11.79904658571650877, -10.55909629022110963, 74.44444907532985667 ) ) ;
#18157=CARTESIAN_POINT ( 'NONE',  ( -18.20084761934894146, -22.21872609085398764, 65.46719399146324747 ) ) ;
#18158=ORIENTED_EDGE ( 'NONE', *, *, #2059, .T. ) ;
#18159=B_SPLINE_CURVE_WITH_KNOTS ( 'NONE', 3,
 ( #31703, #20629, #31457, #30750, #19659, #5619, #16174, #9063, #27281, #4632 ),
 .UNSPECIFIED., .F., .F.,
 ( 4, 2, 2, 2, 4 ),
 ( 0.1272669073658515837, 0.2522669073439512966, 0.3772669073220510372, 0.5022669073001506668, 0.6272669072782504074 ),
 .UNSPECIFIED. ) ;
#18160=AXIS2_PLACEMENT_3D ( 'NONE', #21530, #17324, #9954 ) ;
#18162=CARTESIAN_POINT ( 'NONE',  ( -12.14425517392406917, -10.13739710456042964, 64.17914326607970565 ) ) ;
#18163=CARTESIAN_POINT ( 'NONE',  ( -11.91343869374197695, -19.82283377674160718, 58.04186948019505365 ) ) ;
#18164=ORIENTED_EDGE ( 'NONE', *, *, #44104, .F. ) ;
#18166=CARTESIAN_POINT ( 'NONE',  ( -11.35719102664687874, -18.40077844947705188, 58.09242476654641507 ) ) ;
#18167=CARTESIAN_POINT ( 'NONE',  ( -16.11395021683892281, -7.881860907381922132, 63.67570853548351550 ) ) ;
#18168=ORIENTED_EDGE ( 'NONE', *, *, #21422, .F. ) ;
#18169=CARTESIAN_POINT ( 'NONE',  ( -18.31357640787765462, -21.80286941108919763, 68.81514702304139064 ) ) ;
#18172=CARTESIAN_POINT ( 'NONE',  ( -24.87230691347358302, -14.64571622948453111, 62.91307683260841088 ) ) ;
#18174=CARTESIAN_POINT ( 'NONE',  ( -18.42426029547229405, -21.73782819656517873, 72.56894429655113754 ) ) ;
#18176=CARTESIAN_POINT ( 'NONE',  ( -10.40277073914389661, -15.44443991871667343, 57.56792809063193772 ) ) ;
#18177=VERTEX_POINT ( 'NONE', #21496 ) ;
#18178=CARTESIAN_POINT ( 'NONE',  ( -13.60236376389480384, -20.73382277062339085, 61.80174179654961364 ) ) ;
#18179=FACE_OUTER_BOUND ( 'NONE', #26918, .T. ) ;
#18180=CARTESIAN_POINT ( 'NONE',  ( -23.39635208968330105, -11.04794396834914494, 70.04777744521437910 ) ) ;
#18181=ORIENTED_EDGE ( 'NONE', *, *, #35108, .T. ) ;
#18182=DIRECTION ( 'NONE',  ( -2.027460363947684990E-06, -1.195255637520530846E-05, 0.9999999999265128947 ) ) ;
#18183=ADVANCED_FACE ( 'NONE', ( #43913 ), #8024, .T. ) ;
#18184=CARTESIAN_POINT ( 'NONE',  ( -11.40126873537406205, -11.24191379345135999, 60.97885781058090515 ) ) ;
#18187=EDGE_CURVE ( 'NONE', #39328, #43944, #37157, .T. ) ;
#18188=EDGE_CURVE ( 'NONE', #4721, #21230, #38182, .T. ) ;
#18189=ORIENTED_EDGE ( 'NONE', *, *, #6420, .T. ) ;
#18192=CARTESIAN_POINT ( 'NONE',  ( -16.85779285108784009, -7.832151056010677515, 74.06904305648112086 ) ) ;
#18193=DIRECTION ( 'NONE',  ( -0.2393415023380396633, 0.9709354485539016810, -6.438601123826609832E-08 ) ) ;
#18195=PLANE ( 'NONE',  #32106 ) ;
#18196=( BOUNDED_SURFACE ( )  B_SPLINE_SURFACE ( 3, 1, ( 
 ( #25258, #10483 ),
 ( #3075, #23268 ),
 ( #15358, #45436 ),
 ( #41479, #7772 ),
 ( #27196, #26466 ),
 ( #41980, #8252 ),
 ( #34084, #11690 ) ),
 .UNSPECIFIED., .T., .F., .F. ) 
 B_SPLINE_SURFACE_WITH_KNOTS ( ( 4, 3, 4 ),
 ( 2, 2 ),
 ( 0.000000000000000000, 0.5000000000000000000, 1.000000000000000000 ),
 ( 0.000000000000000000, 1.000000000000000000 ),
 .UNSPECIFIED. ) 
 GEOMETRIC_REPRESENTATION_ITEM ( )  RATIONAL_B_SPLINE_SURFACE ( (
 ( 1.000000000000000000, 1.000000000000000000),
 ( 0.3333333333333335369, 0.3333333333333330373),
 ( 0.3333333333333335369, 0.3333333333333330373),
 ( 1.000000000000000000, 1.000000000000000000),
 ( 0.3333333333333333703, 0.3333333333333333703),
 ( 0.3333333333333333703, 0.3333333333333333703),
 ( 1.000000000000000000, 1.000000000000000000) ) ) 
 REPRESENTATION_ITEM ( '' )  SURFACE ( )  );
#18197=CARTESIAN_POINT ( 'NONE',  ( -13.89248387370423110, -21.36903859207333412, 71.96961763246901000 ) ) ;
#18198=CARTESIAN_POINT ( 'NONE',  ( -12.34063849734112850, -9.996720310667569720, 60.55918082403523073 ) ) ;
#18199=CARTESIAN_POINT ( 'NONE',  ( -10.62027216904274241, -17.84408883714660732, 71.71718193840895594 ) ) ;
#18200=EDGE_LOOP ( 'NONE', ( #8418, #17851 ) ) ;
#18201=CARTESIAN_POINT ( 'NONE',  ( -10.01440787728688520, -14.03439562150409969, 61.03325889150411143 ) ) ;
#18202=CARTESIAN_POINT ( 'NONE',  ( -14.06695675121984301, -8.606427752881131710, 70.61468953885895417 ) ) ;
#18205=CARTESIAN_POINT ( 'NONE',  ( -10.61641583932764910, -11.78277314028518319, 74.74335662173743344 ) ) ;
#18206=( BOUNDED_CURVE ( )  B_SPLINE_CURVE ( 3, ( #407, #8513, #11724, #34353 ),
 .UNSPECIFIED., .F., .F. ) 
 B_SPLINE_CURVE_WITH_KNOTS ( ( 4, 4 ),
 ( 0.000000000000000000, 0.4074455897393702841 ),
 .UNSPECIFIED. ) 
 CURVE ( )  GEOMETRIC_REPRESENTATION_ITEM ( )  RATIONAL_B_SPLINE_CURVE ( ( 1.000000000000000000, 0.4567392136813254733, 0.3561768502900278799, 0.6983129098261073864 ) ) 
 REPRESENTATION_ITEM ( '' )  );
#18207=ORIENTED_EDGE ( 'NONE', *, *, #27152, .T. ) ;
#18208=VERTEX_POINT ( 'NONE', #14305 ) ;
#18209=EDGE_CURVE ( 'NONE', #32937, #37435, #27127, .T. ) ;
#18211=CARTESIAN_POINT ( 'NONE',  ( -10.71808830285582914, -12.63376213818331628, 61.09853562115718262 ) ) ;
#18212=CARTESIAN_POINT ( 'NONE',  ( -13.93897074462874919, -20.93787812888889377, 68.74153005185598886 ) ) ;
#18213=ORIENTED_EDGE ( 'NONE', *, *, #23639, .T. ) ;
#18215=B_SPLINE_CURVE_WITH_KNOTS ( 'NONE', 3,
 ( #34124, #8717, #35033, #12637, #11002, #27659, #5254, #42692, #22568, #45239 ),
 .UNSPECIFIED., .F., .F.,
 ( 4, 2, 2, 2, 4 ),
 ( 0.6272669072877217200, 0.7522669073072643098, 0.8772669073268068995, 1.002266907346349489, 1.127266907365892079 ),
 .UNSPECIFIED. ) ;
#18216=CARTESIAN_POINT ( 'NONE',  ( -12.52712847051791378, -9.194636617869647921, 74.36277061998997340 ) ) ;
#18218=AXIS2_PLACEMENT_3D ( 'NONE', #7398, #14988, #22400 ) ;
#18219=CARTESIAN_POINT ( 'NONE',  ( -13.63887963148984817, -21.22614835001067490, 68.61771678319368561 ) ) ;
#18220=CARTESIAN_POINT ( 'NONE',  ( -24.86960059988683014, -14.52975442119237748, 62.82641240410487171 ) ) ;
#18221=CARTESIAN_POINT ( 'NONE',  ( -23.34288328645119037, -19.33377384263253873, 59.06905932422779415 ) ) ;
#18222=ORIENTED_EDGE ( 'NONE', *, *, #20900, .F. ) ;
#18223=CARTESIAN_POINT ( 'NONE',  ( -24.14084320357540747, -12.83654105174326077, 69.78859659034802121 ) ) ;
#18224=VERTEX_POINT ( 'NONE', #18751 ) ;
#18225=CARTESIAN_POINT ( 'NONE',  ( -19.50844099596679371, -21.96177777289817357, 62.11008350414853396 ) ) ;
#18226=CARTESIAN_POINT ( 'NONE',  ( -24.39574017056938615, -14.17912290068383108, 69.93809931784123535 ) ) ;
#18229=CARTESIAN_POINT ( 'NONE',  ( -24.08517543038346531, -12.49907855475201579, 73.52753481283211556 ) ) ;
#18231=B_SPLINE_CURVE_WITH_KNOTS ( 'NONE', 1,
 ( #29738, #44774 ),
 .UNSPECIFIED., .F., .F.,
 ( 2, 2 ),
 ( 0.000000000000000000, 1.000000000000000000 ),
 .UNSPECIFIED. ) ;
#18233=CARTESIAN_POINT ( 'NONE',  ( -10.75331705403316818, -16.93070056221711184, 57.98760548944069626 ) ) ;
#18235=FACE_OUTER_BOUND ( 'NONE', #45788, .T. ) ;
#18236=ORIENTED_EDGE ( 'NONE', *, *, #47916, .F. ) ;
#18237=CARTESIAN_POINT ( 'NONE',  ( -24.87106857282577721, -14.59265502392501546, 62.83483757625009503 ) ) ;
#18238=DIRECTION ( 'NONE',  ( -5.731567514496413899E-31, -1.020425574103664789E-16, -1.000000000000000000 ) ) ;
#18241=CARTESIAN_POINT ( 'NONE',  ( -11.32522400900782067, -11.27219014254736074, 60.96413645226084554 ) ) ;
#18242=EDGE_CURVE ( 'NONE', #16383, #31039, #30727, .T. ) ;
#18243=EDGE_LOOP ( 'NONE', ( #45675, #11557 ) ) ;
#18244=ORIENTED_EDGE ( 'NONE', *, *, #41305, .T. ) ;
#18245=CARTESIAN_POINT ( 'NONE',  ( -11.31808814922340822, -18.33929587155208552, 61.69199689979424051 ) ) ;
#18246=CARTESIAN_POINT ( 'NONE',  ( -14.98927377128267047, -8.246306944878837086, 57.14999999999994884 ) ) ;
#18247=EDGE_LOOP ( 'NONE', ( #5433, #13171, #22930, #40031, #48620 ) ) ;
#18248=CARTESIAN_POINT ( 'NONE',  ( -24.11793993921729395, -12.76166543249827434, 70.07243002473258286 ) ) ;
#18249=CARTESIAN_POINT ( 'NONE',  ( -12.55411140858086760, -19.90724249994213935, 65.15202838036978505 ) ) ;
#18252=CARTESIAN_POINT ( 'NONE',  ( -22.14851325272248062, -9.572347091288939680, 60.13659902389549927 ) ) ;
#18253=FACE_BOUND ( 'NONE', #35961, .T. ) ;
#18255=CARTESIAN_POINT ( 'NONE',  ( -10.42462062702805703, -14.89507852762941198, 74.79778901763455679 ) ) ;
#18256=EDGE_CURVE ( 'NONE', #12881, #2612, #37702, .T. ) ;
#18258=CARTESIAN_POINT ( 'NONE',  ( -24.28619334359350290, -16.42731978468327014, 59.13804568661029037 ) ) ;
#18260=CYLINDRICAL_SURFACE ( 'NONE', #15635, 0.1500000000000031586 ) ;
#18261=CARTESIAN_POINT ( 'NONE',  ( -21.63336539757928634, -9.153348366551478321, 66.94677872351418557 ) ) ;
#18262=ADVANCED_FACE ( 'NONE', ( #31061 ), #9597, .T. ) ;
#18263=CARTESIAN_POINT ( 'NONE',  ( -17.04413539470109740, -21.84925844046378174, 72.45071136019464575 ) ) ;
#18264=EDGE_CURVE ( 'NONE', #26255, #17956, #43243, .T. ) ;
#18267=CARTESIAN_POINT ( 'NONE',  ( -11.89177157637785598, -10.51836466457079844, 74.51055518672704636 ) ) ;
#18268=CARTESIAN_POINT ( 'NONE',  ( -21.99178428503401861, -9.439038574390064440, 60.02171213140443484 ) ) ;
#18270=ORIENTED_EDGE ( 'NONE', *, *, #8960, .F. ) ;
#18272=VERTEX_POINT ( 'NONE', #26892 ) ;
#18273=EDGE_CURVE ( 'NONE', #30917, #29274, #23431, .T. ) ;
#18275=CARTESIAN_POINT ( 'NONE',  ( -23.98474799315784978, -17.25007060033011896, 69.41339792561625188 ) ) ;
#18277=CARTESIAN_POINT ( 'NONE',  ( -16.23263389423368963, -22.16407464444966280, 58.39930168947970657 ) ) ;
#18278=EDGE_LOOP ( 'NONE', ( #47990, #40107, #16328, #28314, #5723 ) ) ;
#18279=CARTESIAN_POINT ( 'NONE',  ( -13.76849323099554567, -20.83774554052356365, 65.27156739751333703 ) ) ;
#18280=CARTESIAN_POINT ( 'NONE',  ( -21.06634951290973845, -21.30826427787840771, 62.29966696806321380 ) ) ;
#18281=ORIENTED_EDGE ( 'NONE', *, *, #9768, .T. ) ;
#18283=CARTESIAN_POINT ( 'NONE',  ( -12.94360638298142163, -11.59623166875815237, 53.69233794759168177 ) ) ;
#18284=ORIENTED_EDGE ( 'NONE', *, *, #24293, .F. ) ;
#18285=CARTESIAN_POINT ( 'NONE',  ( -17.76896499593897261, -7.367070395244857295, 60.20248019549192975 ) ) ;
#18286=CARTESIAN_POINT ( 'NONE',  ( -11.09636557211808849, -11.81291458199088495, 74.78669872099975180 ) ) ;
#18288=ORIENTED_EDGE ( 'NONE', *, *, #32254, .F. ) ;
#18289=CARTESIAN_POINT ( 'NONE',  ( -11.95600649777366264, -19.86917281586842066, 58.03344075405964020 ) ) ;
#18290=PLANE ( 'NONE',  #7704 ) ;
#18291=EDGE_CURVE ( 'NONE', #45009, #35691, #41873, .T. ) ;
#18292=FACE_OUTER_BOUND ( 'NONE', #39769, .T. ) ;
#18293=CARTESIAN_POINT ( 'NONE',  ( -15.34465393633500518, -21.54586957516256263, 68.86120835375241711 ) ) ;
#18294=EDGE_LOOP ( 'NONE', ( #23987, #3492 ) ) ;
#18295=CARTESIAN_POINT ( 'NONE',  ( -24.30048588269890431, -16.36411231998812710, 59.12332431758469653 ) ) ;
#18296=DIRECTION ( 'NONE',  ( -7.623677603559713149E-06, -4.209792907790860808E-06, 0.9999999999620784452 ) ) ;
#18297=CARTESIAN_POINT ( 'NONE',  ( -17.73224099643095286, -22.30287356026373047, 54.27966884056655061 ) ) ;
#18298=FACE_OUTER_BOUND ( 'NONE', #17167, .T. ) ;
#18299=EDGE_CURVE ( 'NONE', #30729, #35243, #21886, .T. ) ;
#18300=ORIENTED_EDGE ( 'NONE', *, *, #10005, .T. ) ;
#18301=CARTESIAN_POINT ( 'NONE',  ( -16.46477641927899782, -7.821750181629138154, 60.61517342399707076 ) ) ;
#18303=EDGE_LOOP ( 'NONE', ( #17354, #48216, #31563, #32263, #22412 ) ) ;
#18305=CARTESIAN_POINT ( 'NONE',  ( -15.37798316477759109, -8.114859020620054153, 74.30658946014833077 ) ) ;
#18306=CARTESIAN_POINT ( 'NONE',  ( -10.51729459156483237, -16.22293329152201480, 71.59750383216309899 ) ) ;
#18310=ORIENTED_EDGE ( 'NONE', *, *, #4432, .F. ) ;
#18311=ORIENTED_EDGE ( 'NONE', *, *, #26295, .T. ) ;
#18312=ORIENTED_EDGE ( 'NONE', *, *, #43442, .F. ) ;
#18315=EDGE_CURVE ( 'NONE', #44745, #24840, #48248, .T. ) ;
#18317=CARTESIAN_POINT ( 'NONE',  ( -11.25339550917664333, -11.39346175823023088, 60.56396915994215391 ) ) ;
#18318=CARTESIAN_POINT ( 'NONE',  ( -24.42398663107514523, -15.65075326911586906, 73.01775867260030850 ) ) ;
#18319=CARTESIAN_POINT ( 'NONE',  ( -24.85291224181648317, -14.24716073839753250, 69.84613574404021108 ) ) ;
#18320=CARTESIAN_POINT ( 'NONE',  ( -13.71586683582447819, -8.803873544643577631, 60.58383457371648717 ) ) ;
#18322=ORIENTED_EDGE ( 'NONE', *, *, #40487, .F. ) ;
#18327=EDGE_CURVE ( 'NONE', #10986, #43000, #4539, .T. ) ;
#18328=( BOUNDED_CURVE ( )  B_SPLINE_CURVE ( 3, ( #26386, #22453, #40664, #10641 ),
 .UNSPECIFIED., .F., .F. ) 
 B_SPLINE_CURVE_WITH_KNOTS ( ( 4, 4 ),
 ( 0.9074455897393624015, 1.000000000000000000 ),
 .UNSPECIFIED. ) 
 CURVE ( )  GEOMETRIC_REPRESENTATION_ITEM ( )  RATIONAL_B_SPLINE_CURVE ( ( 0.6983129098260856260, 0.7760317562606918740, 0.8765941196519966283, 1.000000000000000000 ) ) 
 REPRESENTATION_ITEM ( '' )  );
#18330=VERTEX_POINT ( 'NONE', #13049 ) ;
#18331=CARTESIAN_POINT ( 'NONE',  ( -10.81170448216924740, -12.36318809540519048, 57.34329390664808557 ) ) ;
#18332=PRODUCT_DEFINITION ( 'UNKNOWN', '', #36852, #19409 ) ;
#18334=CARTESIAN_POINT ( 'NONE',  ( -23.55638786360989911, -11.43265490025598119, 70.17594215464632157 ) ) ;
#18336=( BOUNDED_SURFACE ( )  B_SPLINE_SURFACE ( 3, 1, ( 
 ( #3092, #33118 ),
 ( #14389, #29447 ),
 ( #44478, #19333 ),
 ( #34340, #8271 ),
 ( #15878, #37294 ),
 ( #628, #4098 ),
 ( #26738, #30682 ) ),
 .UNSPECIFIED., .T., .F., .F. ) 
 B_SPLINE_SURFACE_WITH_KNOTS ( ( 4, 3, 4 ),
 ( 2, 2 ),
 ( 0.000000000000000000, 0.5000000000000000000, 1.000000000000000000 ),
 ( 0.000000000000000000, 1.000000000000000000 ),
 .UNSPECIFIED. ) 
 GEOMETRIC_REPRESENTATION_ITEM ( )  RATIONAL_B_SPLINE_SURFACE ( (
 ( 1.000000000000000000, 1.000000000000000000),
 ( 0.3333333333333335369, 0.3333333333333330373),
 ( 0.3333333333333335369, 0.3333333333333330373),
 ( 1.000000000000000000, 1.000000000000000000),
 ( 0.3333333333333333703, 0.3333333333333333703),
 ( 0.3333333333333333703, 0.3333333333333333703),
 ( 1.000000000000000000, 1.000000000000000000) ) ) 
 REPRESENTATION_ITEM ( '' )  SURFACE ( )  );
#18337=CARTESIAN_POINT ( 'NONE',  ( -24.47751270253307609, -14.87344405244085443, 63.01296453033411638 ) ) ;
#18338=B_SPLINE_CURVE_WITH_KNOTS ( 'NONE', 3,
 ( #16219, #5170, #46545, #1457, #12787, #39381, #24124, #9353, #13019, #16469 ),
 .UNSPECIFIED., .F., .F.,
 ( 4, 2, 2, 2, 4 ),
 ( 0.1272669073658746208, 0.2522669073488398861, 0.3772669073318051236, 0.5022669073147704166, 0.6272669072977357096 ),
 .UNSPECIFIED. ) ;
#18339=( BOUNDED_CURVE ( )  B_SPLINE_CURVE ( 3, ( #15071, #18781, #22480, #26914 ),
 .UNSPECIFIED., .F., .F. ) 
 B_SPLINE_CURVE_WITH_KNOTS ( ( 4, 4 ),
 ( 0.4074455897393629011, 0.5000000000000000000 ),
 .UNSPECIFIED. ) 
 CURVE ( )  GEOMETRIC_REPRESENTATION_ITEM ( )  RATIONAL_B_SPLINE_CURVE ( ( 0.6983129098260921763, 0.7760317562606997566, 0.8765941196520031786, 1.000000000000003775 ) ) 
 REPRESENTATION_ITEM ( '' )  );
#18340=VERTEX_POINT ( 'NONE', #42871 ) ;
#18341=B_SPLINE_CURVE_WITH_KNOTS ( 'NONE', 1,
 ( #14207, #6367 ),
 .UNSPECIFIED., .F., .F.,
 ( 2, 2 ),
 ( 0.000000000000000000, 1.000000000000000000 ),
 .UNSPECIFIED. ) ;
#18342=CARTESIAN_POINT ( 'NONE',  ( -21.31800817620502286, -20.62620158190326336, 72.82446429882371319 ) ) ;
#18345=CARTESIAN_POINT ( 'NONE',  ( -10.40918007552567914, -12.30049416576506083, 57.42833712013332814 ) ) ;
#18346=AXIS2_PLACEMENT_3D ( 'NONE', #19459, #34224, #15753 ) ;
#18348=CARTESIAN_POINT ( 'NONE',  ( -23.04367560227575140, -10.55211830211007396, 59.60203429193362012 ) ) ;
#18351=CARTESIAN_POINT ( 'NONE',  ( -10.08201403285261577, -16.07297148251123531, 68.17106154205173141 ) ) ;
#18352=ORIENTED_EDGE ( 'NONE', *, *, #12834, .T. ) ;
#18353=CARTESIAN_POINT ( 'NONE',  ( -22.66727108289645543, -10.09628893573625064, 70.01178520457129650 ) ) ;
#18354=DIRECTION ( 'NONE',  ( 0.9477661110324762106, -0.3189661404888857743, 2.738326501554842086E-08 ) ) ;
#18355=CARTESIAN_POINT ( 'NONE',  ( -19.05639634586962572, -7.942579960324152921, 70.51501210008177623 ) ) ;
#18356=( BOUNDED_CURVE ( )  B_SPLINE_CURVE ( 3, ( #32899, #10520, #17408, #39819 ),
 .UNSPECIFIED., .F., .F. ) 
 B_SPLINE_CURVE_WITH_KNOTS ( ( 4, 4 ),
 ( 0.9074455897393565174, 1.000000000000000000 ),
 .UNSPECIFIED. ) 
 CURVE ( )  GEOMETRIC_REPRESENTATION_ITEM ( )  RATIONAL_B_SPLINE_CURVE ( ( 0.6983129098260613121, 0.7760317562606708908, 0.8765941196519837497, 1.000000000000000000 ) ) 
 REPRESENTATION_ITEM ( '' )  );
#18359=ORIENTED_EDGE ( 'NONE', *, *, #3689, .F. ) ;
#18360=CARTESIAN_POINT ( 'NONE',  ( -22.05923648098858791, -20.05472392750071720, 62.23439162613904330 ) ) ;
#18361=CARTESIAN_POINT ( 'NONE',  ( -13.71154894328531704, -21.26836094557570433, 68.49979187789318757 ) ) ;
#18362=CARTESIAN_POINT ( 'NONE',  ( -16.93379202924731430, -21.84228538806570796, 72.17103004438159530 ) ) ;
#18366=ORIENTED_EDGE ( 'NONE', *, *, #41390, .F. ) ;
#18367=CARTESIAN_POINT ( 'NONE',  ( -22.01615059517208906, -8.856209313517616977, 54.02312124697528617 ) ) ;
#18368=CARTESIAN_POINT ( 'NONE',  ( -23.30282330091471366, -18.60927750845715067, 69.29371984660140527 ) ) ;
#18371=CARTESIAN_POINT ( 'NONE',  ( -13.41327670018355001, -20.54622194888242603, 58.34650078082590596 ) ) ;
#18372=VERTEX_POINT ( 'NONE', #27842 ) ;
#18375=ADVANCED_FACE ( 'NONE', ( #28580 ), #14562, .T. ) ;
#18376=CARTESIAN_POINT ( 'NONE',  ( -19.11145711862998553, -7.964113067175272676, 63.58089235102941217 ) ) ;
#18377=CARTESIAN_POINT ( 'NONE',  ( -21.89826263122328953, -8.852228171720549099, 66.84645388252840803 ) ) ;
#18379=CARTESIAN_POINT ( 'NONE',  ( -17.42409385541300892, -14.80920654474439502, 77.49999999999994316 ) ) ;
#18380=CARTESIAN_POINT ( 'NONE',  ( -21.19055157706816672, -21.23704344223776985, 65.69179803007084217 ) ) ;
#18381=CARTESIAN_POINT ( 'NONE',  ( -14.10113443798904065, -8.141252799482343150, 70.98603544959661349 ) ) ;
#18382=CARTESIAN_POINT ( 'NONE',  ( -17.85433243000881376, -7.371517279143424695, 60.25873515745463038 ) ) ;
#18384=ORIENTED_EDGE ( 'NONE', *, *, #41920, .F. ) ;
#18387=CARTESIAN_POINT ( 'NONE',  ( -17.00410561000564513, -7.771727611841389383, 74.26018273220857679 ) ) ;
#18391=CARTESIAN_POINT ( 'NONE',  ( -10.99934536236922611, -17.58926721141864746, 71.58334779160672667 ) ) ;
#18393=DIRECTION ( 'NONE',  ( 0.1571515419521612722, -0.9875744999047174622, 7.433889655140131751E-08 ) ) ;
#18397=CARTESIAN_POINT ( 'NONE',  ( -24.33635513415894280, -15.92417079501564459, 69.72234651700993879 ) ) ;
#18398=DIRECTION ( 'NONE',  ( 5.408674103422956756E-06, -4.460197091461694596E-06, -0.9999999999754264346 ) ) ;
#18399=CARTESIAN_POINT ( 'NONE',  ( -10.03904583415351581, -13.82694187778184158, 57.56329747881408565 ) ) ;
#18400=EDGE_CURVE ( 'NONE', #7211, #31812, #1981, .T. ) ;
#18401=VERTEX_POINT ( 'NONE', #32025 ) ;
#18403=B_SPLINE_CURVE_WITH_KNOTS ( 'NONE', 1,
 ( #38772, #388 ),
 .UNSPECIFIED., .F., .F.,
 ( 2, 2 ),
 ( 0.000000000000000000, 1.000000000000000000 ),
 .UNSPECIFIED. ) ;
#18404=CARTESIAN_POINT ( 'NONE',  ( -18.89726480061343494, -7.914800429535790549, 67.20071754334654202 ) ) ;
#18405=CARTESIAN_POINT ( 'NONE',  ( -19.98813031515369332, -21.37641424997302053, 72.70478737316020101 ) ) ;
#18407=CARTESIAN_POINT ( 'NONE',  ( -10.43125892716163960, -13.91323834088958122, 57.44825034920751960 ) ) ;
#18409=ORIENTED_EDGE ( 'NONE', *, *, #3322, .T. ) ;
#18410=CARTESIAN_POINT ( 'NONE',  ( -10.51950677724785166, -15.96138457174308556, 64.58059568819477647 ) ) ;
#18411=EDGE_LOOP ( 'NONE', ( #35955, #7622 ) ) ;
#18412=DIRECTION ( 'NONE',  ( 0.9998756790481365675, 0.01576789294826319576, 3.907472227867916492E-09 ) ) ;
#18415=CARTESIAN_POINT ( 'NONE',  ( -23.98503169607928953, -17.39005800936845603, 66.22885190747201989 ) ) ;
#18417=CARTESIAN_POINT ( 'NONE',  ( -18.61312572184442615, -22.16383290914719595, 72.40698155103602573 ) ) ;
#18418=ORIENTED_EDGE ( 'NONE', *, *, #23706, .F. ) ;
#18419=CARTESIAN_POINT ( 'NONE',  ( -20.38226146016681994, -7.971588334861294811, 70.36604906519886526 ) ) ;
#18420=CARTESIAN_POINT ( 'NONE',  ( -19.70791841144649581, -21.90059652173849969, 65.72132139802793915 ) ) ;
#18422=VERTEX_POINT ( 'NONE', #46805 ) ;
#18423=CARTESIAN_POINT ( 'NONE',  ( -13.46651328273216031, -21.12124922736007449, 65.16441668658305275 ) ) ;
#18424=CARTESIAN_POINT ( 'NONE',  ( -12.64372748113232703, -9.622537150800651418, 74.52742792958225948 ) ) ;
#18425=DIRECTION ( 'NONE',  ( 0.04086606279946446846, 0.9938001236776478065, 0.1033986416233887984 ) ) ;
#18426=VERTEX_POINT ( 'NONE', #28081 ) ;
#18427=EDGE_LOOP ( 'NONE', ( #35939, #7341, #4497, #10081, #12005 ) ) ;
#18428=CARTESIAN_POINT ( 'NONE',  ( -22.80070500595625660, -9.652102806524988310, 73.52515182072782807 ) ) ;
#18430=PLANE ( 'NONE',  #16223 ) ;
#18431=( BOUNDED_CURVE ( )  B_SPLINE_CURVE ( 3, ( #25103, #9843, #36632, #10079 ),
 .UNSPECIFIED., .F., .F. ) 
 B_SPLINE_CURVE_WITH_KNOTS ( ( 4, 4 ),
 ( 0.000000000000000000, 0.4074455897393585158 ),
 .UNSPECIFIED. ) 
 CURVE ( )  GEOMETRIC_REPRESENTATION_ITEM ( )  RATIONAL_B_SPLINE_CURVE ( ( 1.000000000000000000, 0.4567392136813423487, 0.3561768502900341526, 0.6983129098260754120 ) ) 
 REPRESENTATION_ITEM ( '' )  );
#18433=CARTESIAN_POINT ( 'NONE',  ( -10.56627932147773308, -16.21290872759732693, 71.74750383609593030 ) ) ;
#18434=CARTESIAN_POINT ( 'NONE',  ( -12.85387012802420514, -9.430729208696401855, 67.53509681483876648 ) ) ;
#18435=CARTESIAN_POINT ( 'NONE',  ( -17.19980177718173664, -7.762775310937220397, 70.49035839668022163 ) ) ;
#18436=B_SPLINE_CURVE_WITH_KNOTS ( 'NONE', 1,
 ( #32231, #37347 ),
 .UNSPECIFIED., .F., .F.,
 ( 2, 2 ),
 ( 0.000000000000000000, 1.000000000000000000 ),
 .UNSPECIFIED. ) ;
#18437=CARTESIAN_POINT ( 'NONE',  ( -14.76438133403450692, -8.332445847819730744, 63.97905807186954519 ) ) ;
#18439=B_SPLINE_CURVE_WITH_KNOTS ( 'NONE', 3,
 ( #9761, #42996, #20601, #31677, #43739, #5823, #20835, #42766, #28701, #16398 ),
 .UNSPECIFIED., .F., .F.,
 ( 4, 2, 2, 2, 4 ),
 ( 0.1272669073658294903, 0.2522669073463160716, 0.3772669073268026807, 0.5022669073072892898, 0.6272669072877758989 ),
 .UNSPECIFIED. ) ;
#18441=CARTESIAN_POINT ( 'NONE',  ( -24.32449541900864176, -13.36385115766270637, 59.36827749005163213 ) ) ;
#18445=CARTESIAN_POINT ( 'NONE',  ( -13.46747565276156422, -9.034678650756244878, 60.73950277887485072 ) ) ;
#18448=ORIENTED_EDGE ( 'NONE', *, *, #15530, .F. ) ;
#18449=CARTESIAN_POINT ( 'NONE',  ( -17.02358301252079542, -7.369853539629952266, 74.08301376234730640 ) ) ;
#18452=CARTESIAN_POINT ( 'NONE',  ( -11.68672710392437608, -10.05669134056747005, 67.68392285705759548 ) ) ;
#18453=CARTESIAN_POINT ( 'NONE',  ( -15.22116837037893866, -21.50650591823945845, 68.59065000974109694 ) ) ;
#18454=EDGE_CURVE ( 'NONE', #21691, #29632, #17946, .T. ) ;
#18455=ORIENTED_EDGE ( 'NONE', *, *, #40850, .T. ) ;
#18457=CARTESIAN_POINT ( 'NONE',  ( -23.59266626310239090, -11.50006285152738705, 66.72214495366867482 ) ) ;
#18458=CARTESIAN_POINT ( 'NONE',  ( -11.16004581379495342, -11.56782820372427167, 64.03393219759587396 ) ) ;
#18460=ADVANCED_FACE ( 'NONE', ( #14716 ), #19646, .T. ) ;
#18463=DIRECTION ( 'NONE',  ( -5.731567514496413899E-31, -1.020425574103664789E-16, -1.000000000000000000 ) ) ;
#18464=CARTESIAN_POINT ( 'NONE',  ( -10.90314314408274399, -12.12021994783307299, 74.76660409782968486 ) ) ;
#18465=CARTESIAN_POINT ( 'NONE',  ( -10.43125892716163960, -13.91323834088957945, 57.44825034920751960 ) ) ;
#18466=ORIENTED_EDGE ( 'NONE', *, *, #25989, .T. ) ;
#18467=CARTESIAN_POINT ( 'NONE',  ( -21.77427962766001812, -9.323007061219151126, 66.85077123041597247 ) ) ;
#18468=EDGE_LOOP ( 'NONE', ( #4731, #42395, #18925, #6654, #30341 ) ) ;
#18469=CARTESIAN_POINT ( 'NONE',  ( -22.37499513144005903, -19.83249348569362880, 73.05889139438880875 ) ) ;
#18470=ORIENTED_EDGE ( 'NONE', *, *, #37251, .F. ) ;
#18471=DIRECTION ( 'NONE',  ( -1.653275063147722522E-06, 1.135554159962570470E-05, 0.9999999999341591117 ) ) ;
#18473=FACE_OUTER_BOUND ( 'NONE', #32664, .T. ) ;
#18474=B_SPLINE_CURVE_WITH_KNOTS ( 'NONE', 3,
 ( #1357, #46191, #23550, #42746, #31895, #12696, #38797, #39285, #15894, #39034 ),
 .UNSPECIFIED., .F., .F.,
 ( 4, 2, 2, 2, 4 ),
 ( 0.000000000000000000, 0.2500000000000000000, 0.5000000000000000000, 0.7500000000000000000, 1.000000000000000000 ),
 .UNSPECIFIED. ) ;
#18477=CARTESIAN_POINT ( 'NONE',  ( -14.97188219925329378, -8.199429090594037461, 56.99999999999994316 ) ) ;
#18478=FACE_OUTER_BOUND ( 'NONE', #46579, .T. ) ;
#18480=CARTESIAN_POINT ( 'NONE',  ( -12.14425528403576848, -10.13739698163135117, 64.02914326607979945 ) ) ;
#18481=CARTESIAN_POINT ( 'NONE',  ( -9.990623107247818879, -14.31192343302863179, 64.57299167182827659 ) ) ;
#18482=CARTESIAN_POINT ( 'NONE',  ( -14.43654735092019514, -7.984457654175056263, 63.98967627971388339 ) ) ;
#18483=CARTESIAN_POINT ( 'NONE',  ( -23.56697050129053750, -18.27597851715990984, 72.97187965531796294 ) ) ;
#18484=CARTESIAN_POINT ( 'NONE',  ( -10.79744546256606341, -12.55229233887115114, 61.08236992542625643 ) ) ;
#18485=CARTESIAN_POINT ( 'NONE',  ( -17.12463553450013265, -7.815553531953688626, 70.77570529858661530 ) ) ;
#18486=EDGE_CURVE ( 'NONE', #5788, #26302, #42401, .T. ) ;
#18488=ORIENTED_EDGE ( 'NONE', *, *, #10210, .T. ) ;
#18491=CARTESIAN_POINT ( 'NONE',  ( -17.69678476813674095, -21.85754569590755736, 61.96715964058037684 ) ) ;
#18492=ORIENTED_EDGE ( 'NONE', *, *, #38689, .T. ) ;
#18494=CARTESIAN_POINT ( 'NONE',  ( -10.11824970337647223, -16.26811690260224452, 71.56254994910038647 ) ) ;
#18495=CARTESIAN_POINT ( 'NONE',  ( -13.30711473254145716, -9.147892019113847084, 63.90946529584681457 ) ) ;
#18496=CARTESIAN_POINT ( 'NONE',  ( -12.44869033171645611, -9.885248809711741913, 57.38935532200543577 ) ) ;
#18497=CARTESIAN_POINT ( 'NONE',  ( -14.91789657710648598, -21.40191547797545724, 58.05129291223532562 ) ) ;
#18498=B_SPLINE_CURVE_WITH_KNOTS ( 'NONE', 3,
 ( #18377, #43545, #9809, #24821, #40080, #26768, #27000, #22331, #11990, #37575 ),
 .UNSPECIFIED., .F., .F.,
 ( 4, 2, 2, 2, 4 ),
 ( 0.6272669072877582463, 0.7522669073072830725, 0.8772669073268077877, 1.002266907346332614, 1.127266907365857440 ),
 .UNSPECIFIED. ) ;
#18499=CARTESIAN_POINT ( 'NONE',  ( -24.38811251953670478, -14.09928673046249159, 73.12271532470063562 ) ) ;
#18500=CARTESIAN_POINT ( 'NONE',  ( -11.43009896910331413, -19.23352928037464693, 71.88697091451700771 ) ) ;
#18501=( BOUNDED_CURVE ( )  B_SPLINE_CURVE ( 3, ( #19287, #15824, #8707, #23004 ),
 .UNSPECIFIED., .F., .F. ) 
 B_SPLINE_CURVE_WITH_KNOTS ( ( 4, 4 ),
 ( 0.4074455897393687853, 0.5000000000000000000 ),
 .UNSPECIFIED. ) 
 CURVE ( )  GEOMETRIC_REPRESENTATION_ITEM ( )  RATIONAL_B_SPLINE_CURVE ( ( 0.6983129098261011691, 0.7760317562606855457, 0.8765941196519793088, 0.9999999999999688027 ) ) 
 REPRESENTATION_ITEM ( '' )  );
#18502=CARTESIAN_POINT ( 'NONE',  ( -10.42413886794138556, -14.85581422461645396, 75.09778936447564490 ) ) ;
#18504=CARTESIAN_POINT ( 'NONE',  ( -16.19813999035177332, -21.75179513556690480, 58.28585572029249562 ) ) ;
#18505=EDGE_LOOP ( 'NONE', ( #44178, #40351, #37662, #21100, #25276 ) ) ;
#18506=CARTESIAN_POINT ( 'NONE',  ( -20.31413516131974717, -8.378470924821744603, 67.06632013881642251 ) ) ;
#18507=CARTESIAN_POINT ( 'NONE',  ( -11.46876066122178095, -18.48806595306161071, 61.57710833523393035 ) ) ;
#18508=ADVANCED_FACE ( 'NONE', ( #6409 ), #24688, .T. ) ;
#18510=CARTESIAN_POINT ( 'NONE',  ( -24.27556694116850977, -13.13524334109580671, 66.71735578995932769 ) ) ;
#18511=CARTESIAN_POINT ( 'NONE',  ( -16.58751391467172098, -21.80939466075598077, 65.52564390317479592 ) ) ;
#18512=CARTESIAN_POINT ( 'NONE',  ( -12.10369268100898132, -9.594121713099781346, 57.27430968559156810 ) ) ;
#18514=ORIENTED_EDGE ( 'NONE', *, *, #34209, .T. ) ;
#18516=ORIENTED_EDGE ( 'NONE', *, *, #35444, .T. ) ;
#18517=CARTESIAN_POINT ( 'NONE',  ( -17.02397506063647015, -21.79788470884169627, 72.46543205081314909 ) ) ;
#18518=CARTESIAN_POINT ( 'NONE',  ( -10.43949455435184603, -13.84896052950683298, 57.46297163929641982 ) ) ;
#18520=CARTESIAN_POINT ( 'NONE',  ( -15.39459761884875100, -7.640960489892825613, 74.27996863187141230 ) ) ;
#18521=ADVANCED_FACE ( 'NONE', ( #44820 ), #29709, .T. ) ;
#18522=EDGE_CURVE ( 'NONE', #10266, #10553, #22411, .T. ) ;
#18523=DIRECTION ( 'NONE',  ( 0.5589780652556124441, -0.8291824422665291516, 7.938832475108296738E-08 ) ) ;
#18525=CARTESIAN_POINT ( 'NONE',  ( -23.12987884181161391, -10.01876350439231977, 66.71995018326251170 ) ) ;
#18526=DIRECTION ( 'NONE',  ( -1.277734862951525411E-05, -2.482875507175237739E-06, -0.9999999999152874297 ) ) ;
#18528=CARTESIAN_POINT ( 'NONE',  ( -22.32518170918469380, -20.42023717105881175, 62.41251914304209691 ) ) ;
#18529=CARTESIAN_POINT ( 'NONE',  ( -24.43362379028604536, -14.05489247495133753, 73.12271507725591846 ) ) ;
#18530=ORIENTED_EDGE ( 'NONE', *, *, #39104, .T. ) ;
#18532=ADVANCED_FACE ( 'NONE', ( #7392 ), #13011, .T. ) ;
#18533=CARTESIAN_POINT ( 'NONE',  ( -19.62622408449249178, -21.50961356628077326, 61.88014844347227950 ) ) ;
#18534=CARTESIAN_POINT ( 'NONE',  ( -15.38020936669038008, -6.822612233742264110, 53.49999999999995026 ) ) ;
#18535=CARTESIAN_POINT ( 'NONE',  ( -9.982716954774490503, -14.44908413001617298, 67.97304700561097945 ) ) ;
#18537=CARTESIAN_POINT ( 'NONE',  ( -24.22092373047179237, -12.93688097883364385, 66.30246741375938768 ) ) ;
#18539=CARTESIAN_POINT ( 'NONE',  ( -14.97037710525490262, -21.36678034756659272, 65.29523681788728595 ) ) ;
#18540=CARTESIAN_POINT ( 'NONE',  ( -21.89264518680100835, -20.26253109894388160, 58.77915004610761684 ) ) ;
#18541=ORIENTED_EDGE ( 'NONE', *, *, #44676, .T. ) ;
#18542=CARTESIAN_POINT ( 'NONE',  ( -10.96921284960095555, -11.97350354382807680, 74.84368195529052059 ) ) ;
#18545=CARTESIAN_POINT ( 'NONE',  ( -17.20812589326699182, -22.32442570159451734, 54.02312124697527906 ) ) ;
#18547=EDGE_CURVE ( 'NONE', #8929, #35456, #18037, .T. ) ;
#18548=VERTEX_POINT ( 'NONE', #45070 ) ;
#18549=CARTESIAN_POINT ( 'NONE',  ( -17.71634532009226248, -22.25352164097983376, 58.59891670633793126 ) ) ;
#18551=ORIENTED_EDGE ( 'NONE', *, *, #24588, .F. ) ;
#18553=CARTESIAN_POINT ( 'NONE',  ( -22.49805058420730219, -9.986866540729424813, 73.78161091687563555 ) ) ;
#18554=CARTESIAN_POINT ( 'NONE',  ( -11.68672710392437608, -10.05669134056747005, 67.68392285705759548 ) ) ;
#18555=EDGE_LOOP ( 'NONE', ( #23422, #34609, #28211, #44690, #4781 ) ) ;
#18558=DIRECTION ( 'NONE',  ( -0.9930145540378111368, 0.1179919296777755672, 4.526730167978065139E-08 ) ) ;
#18560=ORIENTED_EDGE ( 'NONE', *, *, #10235, .T. ) ;
#18562=CARTESIAN_POINT ( 'NONE',  ( -11.36795091080559850, -18.31963851737709348, 58.10714594516144871 ) ) ;
#18564=CARTESIAN_POINT ( 'NONE',  ( -14.02588861851693380, -8.179183006140712919, 70.88991002814806563 ) ) ;
#18566=ORIENTED_EDGE ( 'NONE', *, *, #42891, .T. ) ;
#18567=VERTEX_POINT ( 'NONE', #31003 ) ;
#18569=CARTESIAN_POINT ( 'NONE',  ( -11.45716883000597086, -10.34844295181603790, 74.63896264531059899 ) ) ;
#18572=VERTEX_POINT ( 'NONE', #3677 ) ;
#18573=EDGE_CURVE ( 'NONE', #15587, #29512, #27627, .T. ) ;
#18574=CARTESIAN_POINT ( 'NONE',  ( -16.59344707466788549, -21.75974795715521282, 65.52564390620075585 ) ) ;
#18575=CARTESIAN_POINT ( 'NONE',  ( -13.79242041809915875, -8.303469675591347965, 74.31299407998417905 ) ) ;
#18576=CYLINDRICAL_SURFACE ( 'NONE', #17042, 0.1500000000000017708 ) ;
#18577=VERTEX_POINT ( 'NONE', #41344 ) ;
#18578=CARTESIAN_POINT ( 'NONE',  ( -9.905916914905521509, -14.85586088411330330, 53.76227901944321985 ) ) ;
#18581=ORIENTED_EDGE ( 'NONE', *, *, #26864, .F. ) ;
#18583=CARTESIAN_POINT ( 'NONE',  ( -12.58530871590044242, -9.144360103953445673, 74.49735781771244092 ) ) ;
#18584=CARTESIAN_POINT ( 'NONE',  ( -24.82831796749689701, -13.98412716734901373, 73.31545655147931484 ) ) ;
#18586=ADVANCED_FACE ( 'NONE', ( #7637 ), #33690, .T. ) ;
#18589=DIRECTION ( 'NONE',  ( -0.8017593358536259096, -0.5976470257363776240, 1.209213344977627713E-07 ) ) ;
#18590=AXIS2_PLACEMENT_3D ( 'NONE', #8812, #46222, #31925 ) ;
#18592=FACE_OUTER_BOUND ( 'NONE', #25602, .T. ) ;
#18593=CARTESIAN_POINT ( 'NONE',  ( -10.08052675126636721, -16.06451543208143917, 68.09272439531302723 ) ) ;
#18594=ORIENTED_EDGE ( 'NONE', *, *, #5745, .F. ) ;
#18595=CARTESIAN_POINT ( 'NONE',  ( -10.55417862675165175, -17.69166933648559592, 68.21909214388388421 ) ) ;
#18596=CARTESIAN_POINT ( 'NONE',  ( -17.20086775249401612, -7.362538796574944477, 70.59061584993096972 ) ) ;
#18597=CARTESIAN_POINT ( 'NONE',  ( -10.73745268310985246, -11.52390413789708568, 71.21143970991980154 ) ) ;
#18598=FACE_BOUND ( 'NONE', #28636, .T. ) ;
#18599=ORIENTED_EDGE ( 'NONE', *, *, #19543, .T. ) ;
#18602=CARTESIAN_POINT ( 'NONE',  ( -16.78865379391102408, -21.78030513117466072, 68.69560651887046276 ) ) ;
#18603=CARTESIAN_POINT ( 'NONE',  ( -16.02724665508026192, -7.491242618400526077, 63.78515750052793010 ) ) ;
#18604=EDGE_LOOP ( 'NONE', ( #17242, #40639, #47470, #48370, #44223 ) ) ;
#18605=CARTESIAN_POINT ( 'NONE',  ( -10.44762891037015962, -14.23035630910777627, 64.67187305841532918 ) ) ;
#18607=CARTESIAN_POINT ( 'NONE',  ( -12.23358651314992152, -10.11189197570513443, 64.04530931701648910 ) ) ;
#18608=CARTESIAN_POINT ( 'NONE',  ( -23.56138404952065457, -11.33988834032952830, 70.19210750372964469 ) ) ;
#18611=CARTESIAN_POINT ( 'NONE',  ( -12.91576191806997542, -9.388722997169708151, 71.13453240065665284 ) ) ;
#18612=FACE_OUTER_BOUND ( 'NONE', #10511, .T. ) ;
#18615=VERTEX_POINT ( 'NONE', #42329 ) ;
#18617=DIRECTION ( 'NONE',  ( 0.9163203205182085531, 0.4004460890125010053, -2.380681616944615956E-09 ) ) ;
#18620=( BOUNDED_CURVE ( )  B_SPLINE_CURVE ( 3, ( #14411, #13936, #39824, #28512 ),
 .UNSPECIFIED., .F., .F. ) 
 B_SPLINE_CURVE_WITH_KNOTS ( ( 4, 4 ),
 ( 0.4074455897393655102, 0.5000000000000000000 ),
 .UNSPECIFIED. ) 
 CURVE ( )  GEOMETRIC_REPRESENTATION_ITEM ( )  RATIONAL_B_SPLINE_CURVE ( ( 0.6983129098261007250, 0.7760317562606782182, 0.8765941196519702050, 0.9999999999999577005 ) ) 
 REPRESENTATION_ITEM ( '' )  );
#18622=CARTESIAN_POINT ( 'NONE',  ( -14.19282086353638839, -8.542981675383003903, 71.01485553001869278 ) ) ;
#18626=VERTEX_POINT ( 'NONE', #8849 ) ;
#18627=CARTESIAN_POINT ( 'NONE',  ( -17.63706249495991685, -7.362172851917661909, 63.80702937774674410 ) ) ;
#18628=CARTESIAN_POINT ( 'NONE',  ( -11.87301334638075545, -9.840320147444462151, 64.20727067481126937 ) ) ;
#18631=CARTESIAN_POINT ( 'NONE',  ( -18.53201708017407157, -7.846807123103141102, 74.14064401780549929 ) ) ;
#18632=ORIENTED_EDGE ( 'NONE', *, *, #20786, .T. ) ;
#18633=ADVANCED_FACE ( 'NONE', ( #9087 ), #1191, .F. ) ;
#18634=( BOUNDED_SURFACE ( )  B_SPLINE_SURFACE ( 3, 1, ( 
 ( #19227, #34229 ),
 ( #15504, #42123 ),
 ( #30570, #15999 ),
 ( #8162, #46059 ),
 ( #27098, #8391 ),
 ( #31276, #12800 ),
 ( #1962, #23905 ) ),
 .UNSPECIFIED., .T., .F., .F. ) 
 B_SPLINE_SURFACE_WITH_KNOTS ( ( 4, 3, 4 ),
 ( 2, 2 ),
 ( 0.000000000000000000, 0.5000000000000000000, 1.000000000000000000 ),
 ( 0.000000000000000000, 1.000000000000000000 ),
 .UNSPECIFIED. ) 
 GEOMETRIC_REPRESENTATION_ITEM ( )  RATIONAL_B_SPLINE_SURFACE ( (
 ( 1.000000000000000000, 1.000000000000000000),
 ( 0.3333333333333335369, 0.3333333333333330373),
 ( 0.3333333333333335369, 0.3333333333333330373),
 ( 1.000000000000000000, 1.000000000000000000),
 ( 0.3333333333333333703, 0.3333333333333333703),
 ( 0.3333333333333333703, 0.3333333333333333703),
 ( 1.000000000000000000, 1.000000000000000000) ) ) 
 REPRESENTATION_ITEM ( '' )  SURFACE ( )  );
#18636=( BOUNDED_SURFACE ( )  B_SPLINE_SURFACE ( 3, 1, ( 
 ( #7763, #14123 ),
 ( #3315, #26215 ),
 ( #18317, #22780 ),
 ( #26459, #32851 ),
 ( #25479, #36774 ),
 ( #45190, #7515 ),
 ( #3064, #14600 ) ),
 .UNSPECIFIED., .T., .F., .F. ) 
 B_SPLINE_SURFACE_WITH_KNOTS ( ( 4, 3, 4 ),
 ( 2, 2 ),
 ( 0.000000000000000000, 0.5000000000000000000, 1.000000000000000000 ),
 ( 0.000000000000000000, 1.000000000000000000 ),
 .UNSPECIFIED. ) 
 GEOMETRIC_REPRESENTATION_ITEM ( )  RATIONAL_B_SPLINE_SURFACE ( (
 ( 1.000000000000000000, 1.000000000000000000),
 ( 0.3333333333333335369, 0.3333333333333330373),
 ( 0.3333333333333335369, 0.3333333333333330373),
 ( 1.000000000000000000, 1.000000000000000000),
 ( 0.3333333333333333703, 0.3333333333333333703),
 ( 0.3333333333333333703, 0.3333333333333333703),
 ( 1.000000000000000000, 1.000000000000000000) ) ) 
 REPRESENTATION_ITEM ( '' )  SURFACE ( )  );
#18638=FACE_OUTER_BOUND ( 'NONE', #35195, .T. ) ;
#18639=FACE_OUTER_BOUND ( 'NONE', #27559, .T. ) ;
#18640=CARTESIAN_POINT ( 'NONE',  ( -15.17058493111871975, -21.43790244863053118, 68.80422765957334263 ) ) ;
#18642=B_SPLINE_CURVE_WITH_KNOTS ( 'NONE', 3,
 ( #33233, #40178, #2732, #40891, #47796, #21467, #29085, #29567, #21224, #44597 ),
 .UNSPECIFIED., .F., .F.,
 ( 4, 2, 2, 2, 4 ),
 ( 0.6272669072877683494, 0.7522669073072896229, 0.8772669073268110074, 1.002266907346332392, 1.127266907365853665 ),
 .UNSPECIFIED. ) ;
#18645=CARTESIAN_POINT ( 'NONE',  ( -10.52207825420198439, -16.24630393939493800, 71.74750352243894724 ) ) ;
#18649=CARTESIAN_POINT ( 'NONE',  ( -18.70336468933619045, -7.876203269624392433, 70.67067999151545621 ) ) ;
#18651=CARTESIAN_POINT ( 'NONE',  ( -10.47910621644337326, -16.03883162486972935, 64.39282756246913664 ) ) ;
#18652=DIRECTION ( 'NONE',  ( -5.731567514496413899E-31, -1.020425574103664789E-16, -1.000000000000000000 ) ) ;
#18654=CARTESIAN_POINT ( 'NONE',  ( -10.52199164562254197, -15.97581925089275678, 64.61657531926886122 ) ) ;
#18657=VERTEX_POINT ( 'NONE', #27783 ) ;
#18658=CARTESIAN_POINT ( 'NONE',  ( -24.47412807302115212, -14.81851119574499975, 59.54300240094892160 ) ) ;
#18659=CARTESIAN_POINT ( 'NONE',  ( -19.17988342541450209, -7.569006731055750947, 63.62363369258376622 ) ) ;
#18662=CARTESIAN_POINT ( 'NONE',  ( -12.95651447042595095, -9.351591191262567548, 67.26453940287311184 ) ) ;
#18665=CARTESIAN_POINT ( 'NONE',  ( -21.44147796085869118, -20.54162532479978509, 72.63332330819365268 ) ) ;
#18667=EDGE_CURVE ( 'NONE', #6775, #42405, #23106, .T. ) ;
#18668=CARTESIAN_POINT ( 'NONE',  ( -12.77013062424865630, -8.927826924028671840, 54.27966884056655061 ) ) ;
#18669=CARTESIAN_POINT ( 'NONE',  ( -10.89657404688168363, -17.34179118677383613, 68.20794932300812263 ) ) ;
#18670=ORIENTED_EDGE ( 'NONE', *, *, #30494, .F. ) ;
#18671=CARTESIAN_POINT ( 'NONE',  ( -17.79108452803360763, -21.84994637594637368, 58.69081321602850920 ) ) ;
#18672=CARTESIAN_POINT ( 'NONE',  ( -11.74108458883011963, -23.16273580036827440, 54.49999999999995026 ) ) ;
#18673=FACE_OUTER_BOUND ( 'NONE', #13816, .T. ) ;
#18674=EDGE_LOOP ( 'NONE', ( #17254, #38269, #15792, #134, #25571 ) ) ;
#18675=ORIENTED_EDGE ( 'NONE', *, *, #19302, .F. ) ;
#18678=CARTESIAN_POINT ( 'NONE',  ( -23.24415167771102020, -18.79314401478295338, 62.23918030722157368 ) ) ;
#18681=CARTESIAN_POINT ( 'NONE',  ( -24.84263255441417328, -14.11714595057820354, 73.30926835346492965 ) ) ;
#18682=CARTESIAN_POINT ( 'NONE',  ( -11.42587710518540334, -11.10406226247761019, 57.49431069621225276 ) ) ;
#18683=CARTESIAN_POINT ( 'NONE',  ( -16.93697101831087792, -7.375022458023401839, 74.13735168198904546 ) ) ;
#18684=CARTESIAN_POINT ( 'NONE',  ( -16.49697044570162774, -22.20142030250349663, 65.34847517160625330 ) ) ;
#18687=B_SPLINE_CURVE_WITH_KNOTS ( 'NONE', 3,
 ( #37475, #44652, #45152, #4023, #10913, #19028, #25933, #7233, #48575, #22238 ),
 .UNSPECIFIED., .F., .F.,
 ( 4, 2, 2, 2, 4 ),
 ( 0.000000000000000000, 0.2500000000000000000, 0.5000000000000000000, 0.7500000000000000000, 1.000000000000000000 ),
 .UNSPECIFIED. ) ;
#18688=CARTESIAN_POINT ( 'NONE',  ( -14.03871066829747249, -8.172719617054283958, 70.91452941929576070 ) ) ;
#18689=PLANE ( 'NONE',  #37415 ) ;
#18690=DIRECTION ( 'NONE',  ( 6.865757730863489906E-07, 1.412849154798944614E-06, 0.9999999999987662092 ) ) ;
#18692=AXIS2_PLACEMENT_3D ( 'NONE', #17812, #17085, #24520 ) ;
#18693=ORIENTED_EDGE ( 'NONE', *, *, #41061, .F. ) ;
#18695=ORIENTED_EDGE ( 'NONE', *, *, #18963, .T. ) ;
#18696=CARTESIAN_POINT ( 'NONE',  ( -16.99059232606724734, -7.371822389834469469, 74.16029473639015634 ) ) ;
#18697=DIRECTION ( 'NONE',  ( 0.9999247414263408018, -0.01226831216845470154, -5.367905339470937357E-08 ) ) ;
#18698=B_SPLINE_CURVE_WITH_KNOTS ( 'NONE', 3,
 ( #12280, #5389, #28525, #32455, #25539, #24824, #2412, #17423, #36130, #31963 ),
 .UNSPECIFIED., .F., .F.,
 ( 4, 2, 2, 2, 4 ),
 ( 0.1272669073658538319, 0.2522669073463127409, 0.3772669073267717055, 0.5022669073072305590, 0.6272669072876895235 ),
 .UNSPECIFIED. ) ;
#18699=CARTESIAN_POINT ( 'NONE',  ( -15.55648817577099585, -8.010769314271311003, 74.09457776258329886 ) ) ;
#18700=CARTESIAN_POINT ( 'NONE',  ( -13.81866929095069096, -21.32886163922821154, 72.08754233397257849 ) ) ;
#18701=VECTOR ( 'NONE', #13335, 1000.000000000000114 ) ;
#18702=ORIENTED_EDGE ( 'NONE', *, *, #27553, .F. ) ;
#18704=AXIS2_PLACEMENT_3D ( 'NONE', #17285, #6218, #35997 ) ;
#18705=CARTESIAN_POINT ( 'NONE',  ( -13.58233848012166511, -8.897862878211833859, 57.26967725704754741 ) ) ;
#18706=CARTESIAN_POINT ( 'NONE',  ( -14.73037927113499812, -8.285490617698924254, 67.40407820626249702 ) ) ;
#18707=ORIENTED_EDGE ( 'NONE', *, *, #42284, .F. ) ;
#18710=CARTESIAN_POINT ( 'NONE',  ( -24.38756562526642213, -15.91227465074932290, 66.34852784166324113 ) ) ;
#18712=CARTESIAN_POINT ( 'NONE',  ( -12.20424117383341311, -20.12491952255346206, 65.12320790045656338 ) ) ;
#18713=ORIENTED_EDGE ( 'NONE', *, *, #13490, .F. ) ;
#18714=CARTESIAN_POINT ( 'NONE',  ( -19.57699507595987143, -21.94144279212693860, 62.17998934563075153 ) ) ;
#18715=EDGE_CURVE ( 'NONE', #18422, #32374, #35164, .T. ) ;
#18716=CARTESIAN_POINT ( 'NONE',  ( -20.40606020541642707, -8.476062491149917832, 63.38409570189014630 ) ) ;
#18717=ORIENTED_EDGE ( 'NONE', *, *, #33265, .T. ) ;
#18719=CARTESIAN_POINT ( 'NONE',  ( -16.78411710364782650, -21.83009890335197767, 68.99560651669348488 ) ) ;
#18724=( BOUNDED_SURFACE ( )  B_SPLINE_SURFACE ( 3, 1, ( 
 ( #36278, #6736 ),
 ( #13850, #28660 ),
 ( #43693, #10914 ),
 ( #25211, #33286 ),
 ( #40233, #21750 ),
 ( #6502, #18035 ),
 ( #14090, #18280 ) ),
 .UNSPECIFIED., .T., .F., .F. ) 
 B_SPLINE_SURFACE_WITH_KNOTS ( ( 4, 3, 4 ),
 ( 2, 2 ),
 ( 0.000000000000000000, 0.5000000000000000000, 1.000000000000000000 ),
 ( 0.000000000000000000, 1.000000000000000000 ),
 .UNSPECIFIED. ) 
 GEOMETRIC_REPRESENTATION_ITEM ( )  RATIONAL_B_SPLINE_SURFACE ( (
 ( 1.000000000000000000, 1.000000000000000000),
 ( 0.3333333333333335369, 0.3333333333333330373),
 ( 0.3333333333333335369, 0.3333333333333330373),
 ( 1.000000000000000000, 1.000000000000000000),
 ( 0.3333333333333333703, 0.3333333333333333703),
 ( 0.3333333333333333703, 0.3333333333333333703),
 ( 1.000000000000000000, 1.000000000000000000) ) ) 
 REPRESENTATION_ITEM ( '' )  SURFACE ( )  );
#18725=EDGE_CURVE ( 'NONE', #10981, #38205, #26496, .T. ) ;
#18726=AXIS2_PLACEMENT_3D ( 'NONE', #18813, #33823, #15103 ) ;
#18727=CARTESIAN_POINT ( 'NONE',  ( -10.06068050546405246, -15.94284296925492939, 64.64625047982192996 ) ) ;
#18729=CARTESIAN_POINT ( 'NONE',  ( -15.75291993497911136, -20.06326719075875076, 53.69233794759168177 ) ) ;
#18730=EDGE_LOOP ( 'NONE', ( #10487, #39015 ) ) ;
#18735=CARTESIAN_POINT ( 'NONE',  ( -12.55411140858086760, -19.90724249994213935, 65.15202838036978505 ) ) ;
#18736=DIRECTION ( 'NONE',  ( -6.312331220146435760E-07, -6.220915576521675503E-06, -0.9999999999804509709 ) ) ;
#18737=DIRECTION ( 'NONE',  ( -1.916827911674356108E-06, -6.156520247306097078E-06, 0.9999999999792114069 ) ) ;
#18738=CARTESIAN_POINT ( 'NONE',  ( -24.18450351543707555, -12.99348042298125883, 62.94150088911103325 ) ) ;
#18739=VERTEX_POINT ( 'NONE', #5640 ) ;
#18740=VERTEX_POINT ( 'NONE', #16926 ) ;
#18742=CARTESIAN_POINT ( 'NONE',  ( -9.975704095843513031, -14.64835857301500255, 71.45065776245529321 ) ) ;
#18744=CARTESIAN_POINT ( 'NONE',  ( -15.39793084389211764, -7.640011784162778596, 74.18011415750440563 ) ) ;
#18746=CARTESIAN_POINT ( 'NONE',  ( -11.30083408395673317, -18.20384969151142940, 58.03544514041180946 ) ) ;
#18748=CARTESIAN_POINT ( 'NONE',  ( -14.30855566557790404, -8.484641631233271752, 70.74429704309763167 ) ) ;
#18749=CARTESIAN_POINT ( 'NONE',  ( -21.83505603848428933, -9.305730678460758298, 59.60682523891489382 ) ) ;
#18750=ADVANCED_FACE ( 'NONE', ( #42587 ), #28124, .T. ) ;
#18751=CARTESIAN_POINT ( 'NONE',  ( -15.87557863975121819, -7.931372594209569193, 67.14007279017359053 ) ) ;
#18754=CARTESIAN_POINT ( 'NONE',  ( -23.88415217903648724, -17.63235132829416685, 62.77360984996715842 ) ) ;
#18755=CARTESIAN_POINT ( 'NONE',  ( -16.63927388632151505, -21.76668874189256542, 68.80633768154915231 ) ) ;
#18756=DIRECTION ( 'NONE',  ( 1.274157597653189794E-05, 2.329884815184971665E-06, -0.9999999999161119923 ) ) ;
#18757=EDGE_CURVE ( 'NONE', #40480, #17650, #5307, .T. ) ;
#18758=ADVANCED_FACE ( 'NONE', ( #9811 ), #25065, .T. ) ;
#18760=DIRECTION ( 'NONE',  ( 0.9753750245375037986, 0.2205528542287732707, 7.244220459260263973E-08 ) ) ;
#18761=CARTESIAN_POINT ( 'NONE',  ( -10.25416474409032652, -12.78293385988982678, 67.92487701448251869 ) ) ;
#18763=CARTESIAN_POINT ( 'NONE',  ( -11.13733870171179596, -11.61806121328041996, 67.90392505421056057 ) ) ;
#18764=CARTESIAN_POINT ( 'NONE',  ( -21.99213670719075253, -20.17946569659695299, 59.04970794435396897 ) ) ;
#18765=CARTESIAN_POINT ( 'NONE',  ( -14.47717485532954029, -21.65240259781455023, 58.35273132940589136 ) ) ;
#18766=CARTESIAN_POINT ( 'NONE',  ( -18.19389323530821301, -22.21941482433020809, 65.53027461949925225 ) ) ;
#18767=ORIENTED_EDGE ( 'NONE', *, *, #25485, .F. ) ;
#18770=B_SPLINE_CURVE_WITH_KNOTS ( 'NONE', 3,
 ( #22895, #8844, #11546, #45791, #38359, #23621, #4400, #34920, #30997, #19674 ),
 .UNSPECIFIED., .F., .F.,
 ( 4, 2, 2, 2, 4 ),
 ( 0.000000000000000000, 0.2500000000000000000, 0.5000000000000000000, 0.7500000000000000000, 1.000000000000000000 ),
 .UNSPECIFIED. ) ;
#18772=CARTESIAN_POINT ( 'NONE',  ( -17.05964169383668150, -21.79977244010465753, 72.18045664228594660 ) ) ;
#18775=FACE_OUTER_BOUND ( 'NONE', #18109, .T. ) ;
#18777=CARTESIAN_POINT ( 'NONE',  ( -17.99631655628617466, -7.779455715877602984, 60.49549448422539655 ) ) ;
#18781=CARTESIAN_POINT ( 'NONE',  ( -21.85939164964043613, -9.329133344058289978, 63.19153770872092224 ) ) ;
#18783=( BOUNDED_CURVE ( )  B_SPLINE_CURVE ( 3, ( #45138, #11381, #21389, #27129 ),
 .UNSPECIFIED., .F., .F. ) 
 B_SPLINE_CURVE_WITH_KNOTS ( ( 4, 4 ),
 ( 0.5000000000000000000, 0.9074455897393582937 ),
 .UNSPECIFIED. ) 
 CURVE ( )  GEOMETRIC_REPRESENTATION_ITEM ( )  RATIONAL_B_SPLINE_CURVE ( ( 0.9999999999999932276, 0.4567392136813395176, 0.3561768502900377054, 0.6983129098260805190 ) ) 
 REPRESENTATION_ITEM ( '' )  );
#18785=CARTESIAN_POINT ( 'NONE',  ( -23.75674853543430842, -11.71073052589263774, 62.95218282383657993 ) ) ;
#18786=VERTEX_POINT ( 'NONE', #39834 ) ;
#18787=DIRECTION ( 'NONE',  ( 0.7915359335728471279, 0.6111226275167354061, 5.146443701300904349E-08 ) ) ;
#18789=EDGE_CURVE ( 'NONE', #46893, #9283, #22934, .T. ) ;
#18790=CARTESIAN_POINT ( 'NONE',  ( -12.93827254315284669, -9.365655574729560229, 67.37942539479081461 ) ) ;
#18792=CARTESIAN_POINT ( 'NONE',  ( -10.60714174419670464, -13.01136550127550606, 68.03832326220812377 ) ) ;
#18793=DIRECTION ( 'NONE',  ( 0.9811758422909350186, 0.1931164583992469597, 7.863147543881891826E-08 ) ) ;
#18794=CARTESIAN_POINT ( 'NONE',  ( -24.27133562072960871, -13.11802050994479707, 59.24779033130878503 ) ) ;
#18795=DIRECTION ( 'NONE',  ( -0.5327540375067998379, -0.8462701315302333382, -7.203825861310614672E-08 ) ) ;
#18797=CARTESIAN_POINT ( 'NONE',  ( -24.31477923169101629, -16.30090137217950641, 59.40860294853779777 ) ) ;
#18798=CARTESIAN_POINT ( 'NONE',  ( -12.20309422964675150, -20.12380354524033521, 64.98179449731530610 ) ) ;
#18799=CARTESIAN_POINT ( 'NONE',  ( -15.44651063079976794, -21.52416795175674835, 72.34575487467760979 ) ) ;
#18800=( BOUNDED_CURVE ( )  B_SPLINE_CURVE ( 3, ( #34389, #677, #4145, #15922 ),
 .UNSPECIFIED., .F., .F. ) 
 B_SPLINE_CURVE_WITH_KNOTS ( ( 4, 4 ),
 ( 0.5000000000000000000, 0.9074455897393631787 ),
 .UNSPECIFIED. ) 
 CURVE ( )  GEOMETRIC_REPRESENTATION_ITEM ( )  RATIONAL_B_SPLINE_CURVE ( ( 0.9999999999999981126, 0.4567392136813338555, 0.3561768502900322098, 0.6983129098260911771 ) ) 
 REPRESENTATION_ITEM ( '' )  );
#18801=CARTESIAN_POINT ( 'NONE',  ( -19.09526777584694202, -9.555145898730048160, 53.69233794759168887 ) ) ;
#18802=CARTESIAN_POINT ( 'NONE',  ( -16.16063032598464133, -7.467038112641824377, 60.38523865926408263 ) ) ;
#18807=DIRECTION ( 'NONE',  ( 0.4683180279402422430, -0.8835599723313412035, 4.589753183357165928E-08 ) ) ;
#18808=CARTESIAN_POINT ( 'NONE',  ( -14.54749350918765671, -8.372447261038937327, 64.07506791522041567 ) ) ;
#18812=CARTESIAN_POINT ( 'NONE',  ( -15.46800725202396265, -8.087938728663994326, 74.07985622482316046 ) ) ;
#18813=CARTESIAN_POINT ( 'NONE',  ( -24.45670955521185164, -12.20012290887857098, 53.49999999999995026 ) ) ;
#18814=VERTEX_POINT ( 'NONE', #44278 ) ;
#18817=AXIS2_PLACEMENT_3D ( 'NONE', #31341, #5965, #5498 ) ;
#18818=EDGE_CURVE ( 'NONE', #45931, #36781, #40020, .T. ) ;
#18819=CARTESIAN_POINT ( 'NONE',  ( -10.00368807899092971, -15.89896712085359098, 53.49999999999994316 ) ) ;
#18822=ORIENTED_EDGE ( 'NONE', *, *, #48257, .T. ) ;
#18825=CARTESIAN_POINT ( 'NONE',  ( -18.84975023778164172, -7.496717724788733328, 70.53214580459695071 ) ) ;
#18826=CARTESIAN_POINT ( 'NONE',  ( -24.79900369310859531, -15.86464144874165072, 69.72645810305080261 ) ) ;
#18827=CARTESIAN_POINT ( 'NONE',  ( -24.84985713749398073, -14.20864767979305121, 69.85264054281394408 ) ) ;
#18828=CARTESIAN_POINT ( 'NONE',  ( -13.56484994756444173, -8.969080399747948462, 56.98470132832054702 ) ) ;
#18834=DIRECTION ( 'NONE',  ( -1.274157596560980788E-05, -2.329884826735012561E-06, 0.9999999999161118813 ) ) ;
#18836=VERTEX_POINT ( 'NONE', #47232 ) ;
#18837=EDGE_CURVE ( 'NONE', #37616, #946, #8890, .T. ) ;
#18838=FACE_OUTER_BOUND ( 'NONE', #8547, .T. ) ;
#18840=CARTESIAN_POINT ( 'NONE',  ( -13.85393748347032528, -8.270264590973253505, 74.38449983516251507 ) ) ;
#18841=FACE_OUTER_BOUND ( 'NONE', #15709, .T. ) ;
#18842=CARTESIAN_POINT ( 'NONE',  ( -11.17943887680513981, -18.87220427245064513, 65.00353025264104190 ) ) ;
#18843=ORIENTED_EDGE ( 'NONE', *, *, #26341, .F. ) ;
#18844=CARTESIAN_POINT ( 'NONE',  ( -23.05949278649137923, -18.96177454351483860, 62.65406924023815805 ) ) ;
#18846=EDGE_LOOP ( 'NONE', ( #13308, #30664, #37018, #6288, #5718 ) ) ;
#18848=CARTESIAN_POINT ( 'NONE',  ( -24.83590064562855559, -14.05458946445556201, 73.30084269368599337 ) ) ;
#18849=CARTESIAN_POINT ( 'NONE',  ( -11.82099675438171005, -9.899106633794131582, 64.21409753874590365 ) ) ;
#18850=CARTESIAN_POINT ( 'NONE',  ( -17.06879511326789256, -7.767867012253359071, 73.97490359703523666 ) ) ;
#18851=VERTEX_POINT ( 'NONE', #10045 ) ;
#18852=PLANE ( 'NONE',  #41460 ) ;
#18853=AXIS2_PLACEMENT_3D ( 'NONE', #45187, #18558, #4296 ) ;
#18854=CARTESIAN_POINT ( 'NONE',  ( -22.77158737830997026, -19.99662634883771517, 72.78367152623742697 ) ) ;
#18855=DIRECTION ( 'NONE',  ( -0.9132646967824439299, 0.4073666574609056124, -8.344532079829881716E-09 ) ) ;
#18856=CARTESIAN_POINT ( 'NONE',  ( -11.98246295270348405, -15.60836430055780433, 54.07175714974878389 ) ) ;
#18857=ORIENTED_EDGE ( 'NONE', *, *, #7357, .F. ) ;
#18858=CARTESIAN_POINT ( 'NONE',  ( -19.51667102011501953, -21.95933653056138013, 62.18841959269452246 ) ) ;
#18860=CARTESIAN_POINT ( 'NONE',  ( -18.66311988809301425, -7.868636481342422329, 70.65595886192740238 ) ) ;
#18861=FACE_BOUND ( 'NONE', #13302, .T. ) ;
#18862=ORIENTED_EDGE ( 'NONE', *, *, #36604, .F. ) ;
#18863=CARTESIAN_POINT ( 'NONE',  ( -13.14696836414372250, -20.90910850243368913, 58.24661284486880675 ) ) ;
#18864=CARTESIAN_POINT ( 'NONE',  ( -10.53619963070230625, -16.06595416482938887, 71.63677569188099881 ) ) ;
#18866=B_SPLINE_CURVE_WITH_KNOTS ( 'NONE', 3,
 ( #32863, #40277, #47658, #33580, #48627, #18081, #36547, #14861, #2604, #33335 ),
 .UNSPECIFIED., .F., .F.,
 ( 4, 2, 2, 2, 4 ),
 ( 0.000000000000000000, 0.2500000000000000000, 0.5000000000000000000, 0.7500000000000000000, 1.000000000000000000 ),
 .UNSPECIFIED. ) ;
#18867=CARTESIAN_POINT ( 'NONE',  ( -10.42302287260171312, -13.97751933429587012, 57.73352905910142852 ) ) ;
#18868=ORIENTED_EDGE ( 'NONE', *, *, #7438, .T. ) ;
#18869=CARTESIAN_POINT ( 'NONE',  ( -14.27401838705792159, -8.498068067913044032, 74.29134615490499982 ) ) ;
#18870=ORIENTED_EDGE ( 'NONE', *, *, #8199, .T. ) ;
#18872=CARTESIAN_POINT ( 'NONE',  ( -17.13503149044196405, -7.764836982087095052, 70.77563787455143540 ) ) ;
#18873=CARTESIAN_POINT ( 'NONE',  ( -14.41828383943595959, -8.428772226827717873, 63.67490250008367525 ) ) ;
#18874=ORIENTED_EDGE ( 'NONE', *, *, #6754, .F. ) ;
#18875=CARTESIAN_POINT ( 'NONE',  ( -10.59985822842712189, -17.79832335570924684, 71.70684799831278156 ) ) ;
#18876=CARTESIAN_POINT ( 'NONE',  ( -18.31455597897553389, -22.20596705496988221, 68.97661230289300249 ) ) ;
#18877=VERTEX_POINT ( 'NONE', #41791 ) ;
#18879=ORIENTED_EDGE ( 'NONE', *, *, #46416, .F. ) ;
#18883=CARTESIAN_POINT ( 'NONE',  ( -20.50928888383101167, -8.027964920953767347, 66.82458168832727097 ) ) ;
#18885=CARTESIAN_POINT ( 'NONE',  ( -20.49170831689750827, -8.461258797198503601, 63.59649424907591708 ) ) ;
#18887=CARTESIAN_POINT ( 'NONE',  ( -11.77169715766437008, -10.59578624409953207, 74.58885051661056309 ) ) ;
#18888=CARTESIAN_POINT ( 'NONE',  ( -19.04042241193164386, -7.536568769452434147, 67.01576393362593365 ) ) ;
#18892=ADVANCED_FACE ( 'NONE', ( #193 ), #45742, .T. ) ;
#18893=EDGE_CURVE ( 'NONE', #26956, #47302, #3620, .T. ) ;
#18894=CARTESIAN_POINT ( 'NONE',  ( -9.974456273375457371, -14.72748566909688073, 71.51278126739182994 ) ) ;
#18895=EDGE_CURVE ( 'NONE', #31648, #7640, #19428, .T. ) ;
#18896=CARTESIAN_POINT ( 'NONE',  ( -13.91686280105865947, -8.236299372188803147, 74.31459218752463869 ) ) ;
#18897=DIRECTION ( 'NONE',  ( 0.5263399769092094171, -0.8502742079512979334, -7.678741023867494836E-08 ) ) ;
#18901=ORIENTED_EDGE ( 'NONE', *, *, #24615, .F. ) ;
#18904=FACE_OUTER_BOUND ( 'NONE', #29254, .T. ) ;
#18906=CARTESIAN_POINT ( 'NONE',  ( -12.37139604325248499, -19.73008851950320519, 57.81193715039307079 ) ) ;
#18908=ORIENTED_EDGE ( 'NONE', *, *, #3759, .T. ) ;
#18909=CARTESIAN_POINT ( 'NONE',  ( -20.39546626481018876, -7.977226069863096569, 70.39066949591953914 ) ) ;
#18911=AXIS2_PLACEMENT_3D ( 'NONE', #10620, #17335, #9492 ) ;
#18912=EDGE_LOOP ( 'NONE', ( #30070, #38773 ) ) ;
#18913=CARTESIAN_POINT ( 'NONE',  ( -18.66311988809301425, -7.868636481342422329, 70.65595886192740238 ) ) ;
#18917=DIRECTION ( 'NONE',  ( -0.2466764125338440639, -0.9690979039805150963, 7.162324212089591066E-08 ) ) ;
#18919=ORIENTED_EDGE ( 'NONE', *, *, #47646, .F. ) ;
#18920=CARTESIAN_POINT ( 'NONE',  ( -18.19389434033494268, -22.21941471489327569, 65.53027570717884487 ) ) ;
#18922=ORIENTED_EDGE ( 'NONE', *, *, #34313, .F. ) ;
#18923=CARTESIAN_POINT ( 'NONE',  ( -24.47368665962210343, -14.70950332193510590, 62.72768537250228604 ) ) ;
#18924=DIRECTION ( 'NONE',  ( -0.9372362738803845517, -0.3486949482324240290, 5.386914174889910583E-09 ) ) ;
#18925=ORIENTED_EDGE ( 'NONE', *, *, #17498, .T. ) ;
#18926=CARTESIAN_POINT ( 'NONE',  ( -22.06946820259537390, -8.984793454286846170, 63.38427902854760987 ) ) ;
#18927=B_SPLINE_CURVE_WITH_KNOTS ( 'NONE', 3,
 ( #26028, #48667, #37322, #18876, #33626, #37826, #3611, #41280, #37568, #22088 ),
 .UNSPECIFIED., .F., .F.,
 ( 4, 2, 2, 2, 4 ),
 ( 0.1272669073657949346, 0.2522669073462943112, 0.3772669073267936324, 0.5022669073072929535, 0.6272669072877923302 ),
 .UNSPECIFIED. ) ;
#18928=( BOUNDED_CURVE ( )  B_SPLINE_CURVE ( 3, ( #26394, #34502, #31066, #12345 ),
 .UNSPECIFIED., .F., .F. ) 
 B_SPLINE_CURVE_WITH_KNOTS ( ( 4, 4 ),
 ( 0.4074455897393636228, 0.5000000000000000000 ),
 .UNSPECIFIED. ) 
 CURVE ( )  GEOMETRIC_REPRESENTATION_ITEM ( )  RATIONAL_B_SPLINE_CURVE ( ( 0.6983129098260818513, 0.7760317562606880992, 0.8765941196519940748, 0.9999999999999992228 ) ) 
 REPRESENTATION_ITEM ( '' )  );
#18929=EDGE_CURVE ( 'NONE', #45391, #43613, #16454, .T. ) ;
#18930=CARTESIAN_POINT ( 'NONE',  ( -16.40208609235968140, -7.882922330141489020, 60.27198835172391966 ) ) ;
#18931=LINE ( 'NONE', #33939, #11755 ) ;
#18933=EDGE_CURVE ( 'NONE', #14728, #30719, #12955, .T. ) ;
#18934=EDGE_LOOP ( 'NONE', ( #3413, #45696 ) ) ;
#18935=ORIENTED_EDGE ( 'NONE', *, *, #5816, .T. ) ;
#18938=CARTESIAN_POINT ( 'NONE',  ( -23.08487763607990928, -19.01185175973044039, 62.36879011380454330 ) ) ;
#18939=ORIENTED_EDGE ( 'NONE', *, *, #39494, .T. ) ;
#18941=CARTESIAN_POINT ( 'NONE',  ( -20.50074447585702941, -8.457105438040551704, 70.39533052524389234 ) ) ;
#18944=( BOUNDED_CURVE ( )  B_SPLINE_CURVE ( 3, ( #12588, #28086, #27611, #23928 ),
 .UNSPECIFIED., .F., .F. ) 
 B_SPLINE_CURVE_WITH_KNOTS ( ( 4, 4 ),
 ( 0.4074455897393611248, 0.5000000000000000000 ),
 .UNSPECIFIED. ) 
 CURVE ( )  GEOMETRIC_REPRESENTATION_ITEM ( )  RATIONAL_B_SPLINE_CURVE ( ( 0.6983129098260809631, 0.7760317562606844355, 0.8765941196519896339, 0.9999999999999945599 ) ) 
 REPRESENTATION_ITEM ( '' )  );
#18946=EDGE_LOOP ( 'NONE', ( #31232, #27391, #33410, #36646, #39457 ) ) ;
#18947=VECTOR ( 'NONE', #18393, 1000.000000000000000 ) ;
#18948=CARTESIAN_POINT ( 'NONE',  ( -13.07136655094769750, -8.762923122256669473, 64.02451139116674028 ) ) ;
#18951=CARTESIAN_POINT ( 'NONE',  ( -10.56492563526530759, -13.18000101695786341, 71.20828586226983248 ) ) ;
#18953=EDGE_CURVE ( 'NONE', #27537, #24743, #46477, .T. ) ;
#18955=ORIENTED_EDGE ( 'NONE', *, *, #227, .F. ) ;
#18956=( BOUNDED_CURVE ( )  B_SPLINE_CURVE ( 3, ( #39023, #41764, #5303, #46180 ),
 .UNSPECIFIED., .F., .F. ) 
 B_SPLINE_CURVE_WITH_KNOTS ( ( 4, 4 ),
 ( 0.4074455897393652881, 0.5000000000000000000 ),
 .UNSPECIFIED. ) 
 CURVE ( )  GEOMETRIC_REPRESENTATION_ITEM ( )  RATIONAL_B_SPLINE_CURVE ( ( 0.6983129098261153800, 0.7760317562607275121, 0.8765941196520252721, 1.000000000000015765 ) ) 
 REPRESENTATION_ITEM ( '' )  );
#18957=EDGE_CURVE ( 'NONE', #33529, #18814, #7903, .T. ) ;
#18961=CARTESIAN_POINT ( 'NONE',  ( -13.87255710869803593, -21.35819254899724484, 72.12596476508147703 ) ) ;
#18963=EDGE_CURVE ( 'NONE', #1317, #20165, #12627, .T. ) ;
#18965=CARTESIAN_POINT ( 'NONE',  ( -11.29219319990544079, -18.28864530752396433, 57.82186711835544912 ) ) ;
#18966=CARTESIAN_POINT ( 'NONE',  ( -13.33011785382929304, -9.069340661520646663, 63.92418669539090814 ) ) ;
#18969=CARTESIAN_POINT ( 'NONE',  ( -21.89130958583942288, -9.354787850460871468, 63.20625856529903075 ) ) ;
#18970=CARTESIAN_POINT ( 'NONE',  ( -17.78823904182716120, -7.818684512505932993, 60.38060768393231825 ) ) ;
#18971=CARTESIAN_POINT ( 'NONE',  ( -14.03512939856252295, -8.627013252941546639, 74.49394897105099744 ) ) ;
#18972=ORIENTED_EDGE ( 'NONE', *, *, #42402, .F. ) ;
#18975=CARTESIAN_POINT ( 'NONE',  ( -19.36683724782897897, -21.58655468785150688, 62.00975759738177118 ) ) ;
#18979=CARTESIAN_POINT ( 'NONE',  ( -13.41559392277415341, -8.529421005230245711, 57.08472474434080368 ) ) ;
#18984=EDGE_CURVE ( 'NONE', #44873, #11500, #79, .T. ) ;
#18986=CARTESIAN_POINT ( 'NONE',  ( -10.52155775835627161, -17.61265482900956414, 68.27534675147255427 ) ) ;
#18987=CARTESIAN_POINT ( 'NONE',  ( -17.20779274827556904, -21.85960060673416194, 72.16543130510109449 ) ) ;
#18991=CARTESIAN_POINT ( 'NONE',  ( -20.56282673992903653, -8.552218612421922828, 63.31121530278369391 ) ) ;
#18992=CARTESIAN_POINT ( 'NONE',  ( -22.38923928277987940, -20.36363336896080867, 62.35626408838342627 ) ) ;
#18993=CARTESIAN_POINT ( 'NONE',  ( -18.44104399304328012, -21.73500248025376536, 68.88802706434297818 ) ) ;
#18994=CARTESIAN_POINT ( 'NONE',  ( -23.76579110128109207, -18.71917648078158791, 72.92514783281183099 ) ) ;
#18995=VERTEX_POINT ( 'NONE', #39042 ) ;
#18996=ORIENTED_EDGE ( 'NONE', *, *, #10961, .F. ) ;
#18997=CARTESIAN_POINT ( 'NONE',  ( -23.99312320239454976, -11.29471777418100231, 66.60709819448160829 ) ) ;
#18998=CARTESIAN_POINT ( 'NONE',  ( -10.35393594074381163, -12.46056753982151122, 60.99191868369305780 ) ) ;
#18999=VERTEX_POINT ( 'NONE', #28215 ) ;
#19000=CARTESIAN_POINT ( 'NONE',  ( -10.00761937521931522, -15.51608998476985946, 57.75288115419267854 ) ) ;
#19003=CARTESIAN_POINT ( 'NONE',  ( -10.45256745270239307, -15.43993597667916795, 57.86792809192976961 ) ) ;
#19004=CARTESIAN_POINT ( 'NONE',  ( -21.57861252614732095, -20.99326887020048460, 72.62422790022243646 ) ) ;
#19005=CARTESIAN_POINT ( 'NONE',  ( -11.41497376296057098, -19.21309731666858411, 71.80190493362104576 ) ) ;
#19006=CARTESIAN_POINT ( 'NONE',  ( -20.54979551517892489, -8.489990701729437816, 63.31121512946744190 ) ) ;
#19008=CARTESIAN_POINT ( 'NONE',  ( -10.03117811545256366, -15.73068522104555100, 61.15976275176203103 ) ) ;
#19010=PLANE ( 'NONE',  #10131 ) ;
#19013=CARTESIAN_POINT ( 'NONE',  ( -12.11584165285342074, -20.03677265438916422, 61.53532148967806137 ) ) ;
#19014=CARTESIAN_POINT ( 'NONE',  ( -13.76849323099554567, -20.83774554052356009, 65.27156739751333703 ) ) ;
#19016=CARTESIAN_POINT ( 'NONE',  ( -23.49605051889219709, -11.22618518380361330, 73.37665428612797314 ) ) ;
#19018=VERTEX_POINT ( 'NONE', #5326 ) ;
#19021=VERTEX_POINT ( 'NONE', #12936 ) ;
#19022=CARTESIAN_POINT ( 'NONE',  ( -17.36015840614627592, -7.359395087992972151, 67.20535029649403214 ) ) ;
#19025=CARTESIAN_POINT ( 'NONE',  ( -13.67313190561211478, -20.71991002637085089, 65.00245577047650158 ) ) ;
#19026=CARTESIAN_POINT ( 'NONE',  ( -17.77594409791816688, -7.367433943401969998, 60.26556080592736464 ) ) ;
#19027=ORIENTED_EDGE ( 'NONE', *, *, #29043, .T. ) ;
#19028=CARTESIAN_POINT ( 'NONE',  ( -24.36490017465187208, -15.72991749304959441, 73.19230876869042390 ) ) ;
#19031=CARTESIAN_POINT ( 'NONE',  ( -22.34946685659131305, -20.39877785696383228, 62.43450362657586084 ) ) ;
#19033=CARTESIAN_POINT ( 'NONE',  ( -23.74619265052512418, -11.68934008440960426, 62.95218278636776432 ) ) ;
#19034=EDGE_CURVE ( 'NONE', #5705, #43753, #2565, .T. ) ;
#19035=VERTEX_POINT ( 'NONE', #19614 ) ;
#19036=CARTESIAN_POINT ( 'NONE',  ( -11.14880203912577983, -10.79352180864503552, 57.34869885996136674 ) ) ;
#19037=CARTESIAN_POINT ( 'NONE',  ( -20.31649657898477912, -7.943510300654241796, 70.43595776394847974 ) ) ;
#19038=CARTESIAN_POINT ( 'NONE',  ( -18.59601872632196518, -7.856991649524070809, 73.85536540707786912 ) ) ;
#19039=EDGE_CURVE ( 'NONE', #12740, #11221, #36410, .T. ) ;
#19040=ORIENTED_EDGE ( 'NONE', *, *, #45360, .F. ) ;
#19041=CARTESIAN_POINT ( 'NONE',  ( -23.21820299084679817, -10.12609468326883722, 63.17847675013702258 ) ) ;
#19042=DIRECTION ( 'NONE',  ( 2.575747226434838513E-06, -1.267954838932485449E-05, -0.9999999999162972886 ) ) ;
#19043=CARTESIAN_POINT ( 'NONE',  ( -19.97164353606484255, -21.81018995992316079, 69.11977899231902711 ) ) ;
#19044=CARTESIAN_POINT ( 'NONE',  ( -23.99887651489391871, -12.24265264118830387, 73.39792675737896843 ) ) ;
#19045=ORIENTED_EDGE ( 'NONE', *, *, #12866, .T. ) ;
#19048=CARTESIAN_POINT ( 'NONE',  ( -14.47983227664519212, -7.965588925009814858, 63.90483403727078837 ) ) ;
#19050=CYLINDRICAL_SURFACE ( 'NONE', #21931, 0.1500000000000034084 ) ;
#19051=CARTESIAN_POINT ( 'NONE',  ( -21.20819684703883468, -20.76197102398859329, 65.58453721533290093 ) ) ;
#19054=CARTESIAN_POINT ( 'NONE',  ( -24.28579947082789303, -13.18942387424446494, 62.84736316175410309 ) ) ;
#19055=CARTESIAN_POINT ( 'NONE',  ( -24.71334354870178274, -13.26952572216105075, 59.47772645308575790 ) ) ;
#19056=EDGE_LOOP ( 'NONE', ( #2369, #21355, #45458, #44933, #48690 ) ) ;
#19057=CARTESIAN_POINT ( 'NONE',  ( -24.43774544639958179, -15.55896182022801177, 69.74127236015951325 ) ) ;
#19058=CARTESIAN_POINT ( 'NONE',  ( -24.47509194515568964, -14.61357797254947677, 59.24300266175899310 ) ) ;
#19059=CARTESIAN_POINT ( 'NONE',  ( -10.67632725396948956, -12.73975884439864359, 57.48424594490033002 ) ) ;
#19062=FACE_OUTER_BOUND ( 'NONE', #11816, .T. ) ;
#19064=ORIENTED_EDGE ( 'NONE', *, *, #19964, .F. ) ;
#19066=CARTESIAN_POINT ( 'NONE',  ( -24.17966087195022595, -11.66819065304315117, 59.52589827039258097 ) ) ;
#19067=LINE ( 'NONE', #29663, #21387 ) ;
#19068=CARTESIAN_POINT ( 'NONE',  ( -15.36003256934816719, -8.059790721335600594, 70.76556701434653007 ) ) ;
#19070=ORIENTED_EDGE ( 'NONE', *, *, #12961, .F. ) ;
#19071=ORIENTED_EDGE ( 'NONE', *, *, #31718, .F. ) ;
#19074=EDGE_CURVE ( 'NONE', #24536, #12328, #28837, .T. ) ;
#19076=CARTESIAN_POINT ( 'NONE',  ( -11.97490362423377164, -10.33561459433851404, 67.78424783647008667 ) ) ;
#19077=( BOUNDED_SURFACE ( )  B_SPLINE_SURFACE ( 3, 1, ( 
 ( #7808, #175 ),
 ( #11477, #33616 ),
 ( #15153, #40782 ),
 ( #7067, #41773 ),
 ( #10744, #4341 ),
 ( #30453, #26019 ),
 ( #11727, #37311 ) ),
 .UNSPECIFIED., .T., .F., .F. ) 
 B_SPLINE_SURFACE_WITH_KNOTS ( ( 4, 3, 4 ),
 ( 2, 2 ),
 ( 0.000000000000000000, 0.5000000000000000000, 1.000000000000000000 ),
 ( 0.000000000000000000, 1.000000000000000000 ),
 .UNSPECIFIED. ) 
 GEOMETRIC_REPRESENTATION_ITEM ( )  RATIONAL_B_SPLINE_SURFACE ( (
 ( 1.000000000000000000, 1.000000000000000000),
 ( 0.3333333333333335369, 0.3333333333333330373),
 ( 0.3333333333333335369, 0.3333333333333330373),
 ( 1.000000000000000000, 1.000000000000000000),
 ( 0.3333333333333333703, 0.3333333333333333703),
 ( 0.3333333333333333703, 0.3333333333333333703),
 ( 1.000000000000000000, 1.000000000000000000) ) ) 
 REPRESENTATION_ITEM ( '' )  SURFACE ( )  );
#19080=CARTESIAN_POINT ( 'NONE',  ( -20.35208330028754631, -8.450993137587310855, 66.78104082230152017 ) ) ;
#19081=CARTESIAN_POINT ( 'NONE',  ( -18.90996479553717791, -7.968725069611966916, 66.90071784165556323 ) ) ;
#19082=ORIENTED_EDGE ( 'NONE', *, *, #6756, .T. ) ;
#19083=B_SPLINE_CURVE_WITH_KNOTS ( 'NONE', 3,
 ( #45104, #41144, #11351, #8388, #7425, #23412, #31043, #41885, #19225, #22430 ),
 .UNSPECIFIED., .F., .F.,
 ( 4, 2, 2, 2, 4 ),
 ( 0.1272669073658535543, 0.2522669073463322809, 0.3772669073268109519, 0.5022669073072896229, 0.6272669072877683494 ),
 .UNSPECIFIED. ) ;
#19085=( BOUNDED_CURVE ( )  B_SPLINE_CURVE ( 3, ( #7185, #13146, #33000, #43467 ),
 .UNSPECIFIED., .F., .F. ) 
 B_SPLINE_CURVE_WITH_KNOTS ( ( 4, 4 ),
 ( 0.9074455897393627346, 1.000000000000000000 ),
 .UNSPECIFIED. ) 
 CURVE ( )  GEOMETRIC_REPRESENTATION_ITEM ( )  RATIONAL_B_SPLINE_CURVE ( ( 0.6983129098260820733, 0.7760317562606887654, 0.8765941196519947409, 1.000000000000000000 ) ) 
 REPRESENTATION_ITEM ( '' )  );
#19086=EDGE_CURVE ( 'NONE', #21615, #26298, #5911, .T. ) ;
#19087=VERTEX_POINT ( 'NONE', #14366 ) ;
#19088=DIRECTION ( 'NONE',  ( 0.8565259173193582320, -0.5161040137028850561, 6.301967848571305848E-08 ) ) ;
#19089=LINE ( 'NONE', #15370, #39930 ) ;
#19090=ADVANCED_FACE ( 'NONE', ( #18075 ), #33085, .T. ) ;
#19091=CYLINDRICAL_SURFACE ( 'NONE', #10299, 0.1500000000000020206 ) ;
#19092=ADVANCED_FACE ( 'NONE', ( #36538 ), #40271, .T. ) ;
#19093=PLANE ( 'NONE',  #26213 ) ;
#19094=EDGE_CURVE ( 'NONE', #11362, #24536, #1818, .T. ) ;
#19095=EDGE_LOOP ( 'NONE', ( #25354, #9693, #3097, #1675, #27144, #643, #38186, #18448, #27078, #34299, #21985, #17642, #4790, #28464, #36441, #33655, #21872, #4881, #46053, #38297, #45814, #15685, #7400, #8270, #23208, #8317, #903, #15752, #36097, #13563, #26031, #13025, #21602, #17550 ) ) ;
#19097=CARTESIAN_POINT ( 'NONE',  ( -24.08517543038346531, -12.49907855475201579, 73.52753481283211556 ) ) ;
#19099=FACE_OUTER_BOUND ( 'NONE', #30055, .T. ) ;
#19100=ORIENTED_EDGE ( 'NONE', *, *, #34694, .T. ) ;
#19101=CARTESIAN_POINT ( 'NONE',  ( -19.57699614054808634, -21.94144247634149281, 62.17999043330664222 ) ) ;
#19102=CARTESIAN_POINT ( 'NONE',  ( -14.64884435835704757, -8.328266481489457362, 63.79538598111422942 ) ) ;
#19104=FACE_BOUND ( 'NONE', #38118, .T. ) ;
#19106=VERTEX_POINT ( 'NONE', #6773 ) ;
#19107=B_SPLINE_CURVE_WITH_KNOTS ( 'NONE', 3,
 ( #35654, #20421, #39112, #46991, #1933, #28033, #32226, #43316, #16457, #8857 ),
 .UNSPECIFIED., .F., .F.,
 ( 4, 2, 2, 2, 4 ),
 ( 0.000000000000000000, 0.2500000000000000000, 0.5000000000000000000, 0.7500000000000000000, 1.000000000000000000 ),
 .UNSPECIFIED. ) ;
#19108=CARTESIAN_POINT ( 'NONE',  ( -22.11681431073945703, -20.00335822171163258, 62.24941606537704786 ) ) ;
#19109=CARTESIAN_POINT ( 'NONE',  ( -16.06050865347321732, -9.480920197610746669, 53.49999999999995026 ) ) ;
#19111=CARTESIAN_POINT ( 'NONE',  ( -23.42597896001542424, -18.52301023162717897, 65.97956265853692059 ) ) ;
#19113=ORIENTED_EDGE ( 'NONE', *, *, #31418, .F. ) ;
#19115=ORIENTED_EDGE ( 'NONE', *, *, #6779, .T. ) ;
#19116=DIRECTION ( 'NONE',  ( -0.9629498065864410261, -0.2696806815386222911, 2.751890642837218776E-17 ) ) ;
#19119=ORIENTED_EDGE ( 'NONE', *, *, #17576, .F. ) ;
#19121=EDGE_LOOP ( 'NONE', ( #34994, #28494, #12312, #23842, #21835 ) ) ;
#19123=ORIENTED_EDGE ( 'NONE', *, *, #4644, .F. ) ;
#19126=CARTESIAN_POINT ( 'NONE',  ( -22.58065782673598676, -12.89613362149922438, 54.07175714974875547 ) ) ;
#19127=CARTESIAN_POINT ( 'NONE',  ( -23.19948571119275726, -18.85291137746750323, 65.83861571032234394 ) ) ;
#19128=CARTESIAN_POINT ( 'NONE',  ( -10.66703338591908690, -12.79807911521252883, 64.41836111017862265 ) ) ;
#19130=CARTESIAN_POINT ( 'NONE',  ( -14.19282086353638839, -8.542981675383003903, 71.01485553001869278 ) ) ;
#19131=CARTESIAN_POINT ( 'NONE',  ( -11.79630000206883977, -19.05592701419838519, 71.97213747039440079 ) ) ;
#19132=EDGE_LOOP ( 'NONE', ( #8765, #7197 ) ) ;
#19134=CARTESIAN_POINT ( 'NONE',  ( -17.56877512014188625, -7.360533253644350182, 63.59411120999686062 ) ) ;
#19135=ADVANCED_FACE ( 'NONE', ( #35825 ), #17359, .T. ) ;
#19136=CARTESIAN_POINT ( 'NONE',  ( -9.985622318910028383, -14.38165043598653980, 64.50148546807987771 ) ) ;
#19137=CYLINDRICAL_SURFACE ( 'NONE', #37005, 0.1499999999999954148 ) ;
#19138=LINE ( 'NONE', #30725, #19726 ) ;
#19141=ORIENTED_EDGE ( 'NONE', *, *, #11053, .F. ) ;
#19142=CARTESIAN_POINT ( 'NONE',  ( -16.12972974591750486, -21.68894147889758273, 58.30202270284849675 ) ) ;
#19145=CARTESIAN_POINT ( 'NONE',  ( -10.04792990808071984, -13.75760301026566523, 57.63480408467697913 ) ) ;
#19147=CARTESIAN_POINT ( 'NONE',  ( -23.46734565652671378, -18.44686360299153804, 69.50191697180839867 ) ) ;
#19151=CARTESIAN_POINT ( 'NONE',  ( -22.83623332803211881, -19.92908237830355134, 72.82117468064575405 ) ) ;
#19153=CARTESIAN_POINT ( 'NONE',  ( -10.38649001812422057, -14.33425944237064442, 61.12641118716408783 ) ) ;
#19154=CARTESIAN_POINT ( 'NONE',  ( -19.37616851487812752, -21.99900361761337919, 58.71002773933979313 ) ) ;
#19155=CARTESIAN_POINT ( 'NONE',  ( -10.72552546848295485, -12.61109793159036663, 61.09853568372136579 ) ) ;
#19157=CARTESIAN_POINT ( 'NONE',  ( -11.18894283504542564, -11.62402331817657775, 71.19933931412334971 ) ) ;
#19159=CARTESIAN_POINT ( 'NONE',  ( -10.51737753838112610, -13.38018574993044219, 71.09339731095114701 ) ) ;
#19163=B_SPLINE_CURVE_WITH_KNOTS ( 'NONE', 1,
 ( #10581, #35940 ),
 .UNSPECIFIED., .F., .F.,
 ( 2, 2 ),
 ( 0.000000000000000000, 1.000000000000000000 ),
 .UNSPECIFIED. ) ;
#19166=CARTESIAN_POINT ( 'NONE',  ( -24.55871690389112061, -12.66422819002857558, 69.88747705124970366 ) ) ;
#19167=ADVANCED_FACE ( 'NONE', ( #43981 ), #2107, .T. ) ;
#19168=CARTESIAN_POINT ( 'NONE',  ( -10.39241571269986331, -17.41794234916963191, 53.49999999999994316 ) ) ;
#19169=ORIENTED_EDGE ( 'NONE', *, *, #21755, .T. ) ;
#19170=CARTESIAN_POINT ( 'NONE',  ( -22.08245549401321028, -8.995232178987802030, 63.39142531933751457 ) ) ;
#19172=CARTESIAN_POINT ( 'NONE',  ( -11.97682588793020386, -9.726891629870488387, 60.65894467978176863 ) ) ;
#19174=CARTESIAN_POINT ( 'NONE',  ( -19.13762013005870699, -8.022059148145649132, 63.43089277029390161 ) ) ;
#19175=CARTESIAN_POINT ( 'NONE',  ( -21.67414471755420635, -8.689506427787394571, 70.24477150985708818 ) ) ;
#19176=EDGE_CURVE ( 'NONE', #38907, #36780, #2924, .T. ) ;
#19177=AXIS2_PLACEMENT_3D ( 'NONE', #13091, #5243, #6208 ) ;
#19178=ORIENTED_EDGE ( 'NONE', *, *, #38282, .F. ) ;
#19179=ORIENTED_EDGE ( 'NONE', *, *, #40106, .T. ) ;
#19185=CARTESIAN_POINT ( 'NONE',  ( -20.38154718419116662, -8.406214666052791884, 70.66588945595221105 ) ) ;
#19186=B_SPLINE_CURVE_WITH_KNOTS ( 'NONE', 3,
 ( #38470, #45164, #34285, #41694, #34532, #19041, #15818, #30869, #45883, #34045 ),
 .UNSPECIFIED., .F., .F.,
 ( 4, 2, 2, 2, 4 ),
 ( 0.6272669072979214500, 0.7522669073149003127, 0.8772669073318792865, 1.002266907348858149, 1.127266907365837012 ),
 .UNSPECIFIED. ) ;
#19187=CARTESIAN_POINT ( 'NONE',  ( -24.03160980685186843, -17.26750534774173929, 69.41339792588560442 ) ) ;
#19188=CARTESIAN_POINT ( 'NONE',  ( -10.71289789653228830, -16.96858549093376212, 57.98760533367797620 ) ) ;
#19190=ORIENTED_EDGE ( 'NONE', *, *, #8679, .F. ) ;
#19191=CARTESIAN_POINT ( 'NONE',  ( -16.26183941974026581, -7.855670460422400581, 60.35028478908645155 ) ) ;
#19194=EDGE_LOOP ( 'NONE', ( #46568, #16570, #18530, #28759, #4777 ) ) ;
#19195=ORIENTED_EDGE ( 'NONE', *, *, #46372, .F. ) ;
#19196=CARTESIAN_POINT ( 'NONE',  ( -19.86902678349231621, -21.36835431182334233, 69.20703478714260370 ) ) ;
#19197=FACE_OUTER_BOUND ( 'NONE', #33497, .T. ) ;
#19198=CARTESIAN_POINT ( 'NONE',  ( -11.67751508479469358, -10.06770433361378991, 67.65930235469357967 ) ) ;
#19199=CARTESIAN_POINT ( 'NONE',  ( -11.46043843694620179, -11.04924462883820802, 57.50903212149483323 ) ) ;
#19200=EDGE_CURVE ( 'NONE', #18139, #42076, #10705, .T. ) ;
#19201=B_SPLINE_CURVE_WITH_KNOTS ( 'NONE', 1,
 ( #33184, #10076 ),
 .UNSPECIFIED., .F., .F.,
 ( 2, 2 ),
 ( 0.000000000000000000, 1.000000000000000000 ),
 .UNSPECIFIED. ) ;
#19203=FACE_OUTER_BOUND ( 'NONE', #2319, .T. ) ;
#19205=CARTESIAN_POINT ( 'NONE',  ( -14.22586362203780652, -8.080537296073694975, 67.30329176109222544 ) ) ;
#19206=ADVANCED_FACE ( 'NONE', ( #9984 ), #25005, .T. ) ;
#19209=CARTESIAN_POINT ( 'NONE',  ( -22.84776207900630851, -9.701615188675109636, 73.73807001133110361 ) ) ;
#19210=LINE ( 'NONE', #44843, #43038 ) ;
#19211=( BOUNDED_CURVE ( )  B_SPLINE_CURVE ( 3, ( #6382, #36157, #20917, #10326 ),
 .UNSPECIFIED., .F., .F. ) 
 B_SPLINE_CURVE_WITH_KNOTS ( ( 4, 4 ),
 ( 0.9074455897393687298, 1.000000000000000000 ),
 .UNSPECIFIED. ) 
 CURVE ( )  GEOMETRIC_REPRESENTATION_ITEM ( )  RATIONAL_B_SPLINE_CURVE ( ( 0.6983129098261068313, 0.7760317562607100816, 0.8765941196520078416, 1.000000000000000000 ) ) 
 REPRESENTATION_ITEM ( '' )  );
#19212=CARTESIAN_POINT ( 'NONE',  ( -23.63484821195902441, -11.47287264873313184, 66.71654728383106203 ) ) ;
#19213=B_SPLINE_CURVE_WITH_KNOTS ( 'NONE', 3,
 ( #12449, #35091, #4346, #8522, #42505, #8779, #45731, #38798, #34608, #46442 ),
 .UNSPECIFIED., .F., .F.,
 ( 4, 2, 2, 2, 4 ),
 ( 0.000000000000000000, 0.2500000000000000000, 0.5000000000000000000, 0.7500000000000000000, 1.000000000000000000 ),
 .UNSPECIFIED. ) ;
#19214=ORIENTED_EDGE ( 'NONE', *, *, #20799, .T. ) ;
#19215=CARTESIAN_POINT ( 'NONE',  ( -12.15299190543910512, -20.07505386821981119, 65.05330132703942070 ) ) ;
#19216=EDGE_LOOP ( 'NONE', ( #7405, #29982, #45245, #42906, #276 ) ) ;
#19220=VERTEX_POINT ( 'NONE', #34078 ) ;
#19221=CARTESIAN_POINT ( 'NONE',  ( -23.23616624490289340, -18.79948399208958776, 66.12389430041484673 ) ) ;
#19222=CARTESIAN_POINT ( 'NONE',  ( -13.35819042472069107, -21.05197888995676436, 61.70141705377209007 ) ) ;
#19225=CARTESIAN_POINT ( 'NONE',  ( -21.41690965305989991, -21.09893724392033576, 69.24724315047997436 ) ) ;
#19226=EDGE_CURVE ( 'NONE', #9317, #8500, #26437, .T. ) ;
#19227=CARTESIAN_POINT ( 'NONE',  ( -19.04853579327176760, -7.948602568230340282, 63.71617106789811658 ) ) ;
#19228=CARTESIAN_POINT ( 'NONE',  ( -21.68499601416157674, -9.192516039336663169, 66.66149992327366647 ) ) ;
#19229=VERTEX_POINT ( 'NONE', #4302 ) ;
#19231=CARTESIAN_POINT ( 'NONE',  ( -24.86242983737997747, -14.39095285025967286, 66.36788159907001727 ) ) ;
#19232=CARTESIAN_POINT ( 'NONE',  ( -17.42409385541300892, -14.80920654474439502, 75.49999999999994316 ) ) ;
#19233=CARTESIAN_POINT ( 'NONE',  ( -22.33613286903973716, -20.41056029178123055, 62.34165005762706357 ) ) ;
#19234=CARTESIAN_POINT ( 'NONE',  ( -24.76828060908045614, -13.20045483505886352, 53.76227901944320564 ) ) ;
#19235=CARTESIAN_POINT ( 'NONE',  ( -22.78986551909422786, -9.640697744553680337, 73.62014601573351058 ) ) ;
#19236=VERTEX_POINT ( 'NONE', #37515 ) ;
#19237=EDGE_LOOP ( 'NONE', ( #2175, #36853, #42653, #29008, #11123 ) ) ;
#19238=CARTESIAN_POINT ( 'NONE',  ( -18.73521446872676322, -7.879141670414848697, 74.25553277440172906 ) ) ;
#19239=CARTESIAN_POINT ( 'NONE',  ( -14.47651980493331081, -8.396190447208750740, 60.47563573450432273 ) ) ;
#19241=CARTESIAN_POINT ( 'NONE',  ( -12.79725882921341373, -20.12850138265567068, 72.10653676770067477 ) ) ;
#19242=CARTESIAN_POINT ( 'NONE',  ( -15.34465393633500696, -21.54586957516256263, 68.86120835375241711 ) ) ;
#19244=CARTESIAN_POINT ( 'NONE',  ( -16.26184114368905043, -7.855670183028919062, 60.20028478909661374 ) ) ;
#19245=EDGE_CURVE ( 'NONE', #28015, #26442, #7516, .T. ) ;
#19246=CARTESIAN_POINT ( 'NONE',  ( -24.39996007374347542, -14.20938048761671446, 73.23344610889544981 ) ) ;
#19247=DIRECTION ( 'NONE',  ( -0.5510797171261976324, 0.8280216580999243403, 0.1033986416233888955 ) ) ;
#19248=CARTESIAN_POINT ( 'NONE',  ( -20.60788153932096023, -8.518722016582882972, 63.32593600985608617 ) ) ;
#19249=( BOUNDED_SURFACE ( )  B_SPLINE_SURFACE ( 3, 1, ( 
 ( #9225, #5284 ),
 ( #24249, #30670 ),
 ( #11953, #26963 ),
 ( #30912, #12183 ),
 ( #8490, #38519 ),
 ( #34822, #43202 ),
 ( #20558, #21522 ) ),
 .UNSPECIFIED., .T., .F., .F. ) 
 B_SPLINE_SURFACE_WITH_KNOTS ( ( 4, 3, 4 ),
 ( 2, 2 ),
 ( 0.000000000000000000, 0.5000000000000000000, 1.000000000000000000 ),
 ( 0.000000000000000000, 1.000000000000000000 ),
 .UNSPECIFIED. ) 
 GEOMETRIC_REPRESENTATION_ITEM ( )  RATIONAL_B_SPLINE_SURFACE ( (
 ( 1.000000000000000000, 1.000000000000000000),
 ( 0.3333333333333335369, 0.3333333333333330373),
 ( 0.3333333333333335369, 0.3333333333333330373),
 ( 1.000000000000000000, 1.000000000000000000),
 ( 0.3333333333333333703, 0.3333333333333333703),
 ( 0.3333333333333333703, 0.3333333333333333703),
 ( 1.000000000000000000, 1.000000000000000000) ) ) 
 REPRESENTATION_ITEM ( '' )  SURFACE ( )  );
#19254=CARTESIAN_POINT ( 'NONE',  ( -24.17783940236180840, -12.77441742776904299, 73.33405665229432202 ) ) ;
#19256=CARTESIAN_POINT ( 'NONE',  ( -11.82205746763155041, -9.897907871467767293, 64.07268414109491061 ) ) ;
#19258=ORIENTED_EDGE ( 'NONE', *, *, #11798, .F. ) ;
#19259=ORIENTED_EDGE ( 'NONE', *, *, #8291, .T. ) ;
#19263=CARTESIAN_POINT ( 'NONE',  ( -16.43985614576752852, -21.73979035755244382, 61.75568083065761016 ) ) ;
#19264=EDGE_CURVE ( 'NONE', #8282, #25938, #2332, .T. ) ;
#19265=CARTESIAN_POINT ( 'NONE',  ( -13.37515154783066862, -8.555510161798645541, 57.06944116666958422 ) ) ;
#19266=CARTESIAN_POINT ( 'NONE',  ( -16.84878425383806189, -22.23771130781744532, 72.35198525528087998 ) ) ;
#19268=CARTESIAN_POINT ( 'NONE',  ( -20.95734383732741080, -8.250155102951309161, 59.98091898960346668 ) ) ;
#19269=DIRECTION ( 'NONE',  ( -0.3506977235573949248, 0.2775087506578152174, 0.8944271909999157444 ) ) ;
#19270=ORIENTED_EDGE ( 'NONE', *, *, #5122, .F. ) ;
#19271=CARTESIAN_POINT ( 'NONE',  ( -12.26752988409003287, -16.72227946798956921, 53.49999999999995026 ) ) ;
#19272=PLANE ( 'NONE',  #40871 ) ;
#19275=CYLINDRICAL_SURFACE ( 'NONE', #9475, 0.1500000000000048794 ) ;
#19276=LINE ( 'NONE', #34283, #29704 ) ;
#19277=ORIENTED_EDGE ( 'NONE', *, *, #33297, .F. ) ;
#19278=DIRECTION ( 'NONE',  ( 0.9997277805376392212, -0.02333162706040292633, -9.101776391673708383E-09 ) ) ;
#19281=CARTESIAN_POINT ( 'NONE',  ( -14.98927377128279126, -8.246306944878790901, 56.84999999999994458 ) ) ;
#19283=CARTESIAN_POINT ( 'NONE',  ( -11.56105952661339487, -10.21267894317357516, 71.07554790443391823 ) ) ;
#19287=CARTESIAN_POINT ( 'NONE',  ( -20.19231657184298356, -8.325423463105360966, 70.25100341277898508 ) ) ;
#19290=EDGE_CURVE ( 'NONE', #38378, #19901, #48726, .T. ) ;
#19291=CARTESIAN_POINT ( 'NONE',  ( -21.94239175829699207, -20.22099772874085488, 59.06442899522711087 ) ) ;
#19293=VERTEX_POINT ( 'NONE', #22277 ) ;
#19294=B_SPLINE_CURVE_WITH_KNOTS ( 'NONE', 1,
 ( #45692, #19570 ),
 .UNSPECIFIED., .F., .F.,
 ( 2, 2 ),
 ( 0.000000000000000000, 1.000000000000000000 ),
 .UNSPECIFIED. ) ;
#19295=CARTESIAN_POINT ( 'NONE',  ( -14.01352161170464861, -20.97950563691217241, 71.93167508253637266 ) ) ;
#19298=CARTESIAN_POINT ( 'NONE',  ( -15.64068491485237367, -7.988352816650894361, 70.90430021208057099 ) ) ;
#19302=EDGE_CURVE ( 'NONE', #11292, #33252, #3448, .T. ) ;
#19303=CARTESIAN_POINT ( 'NONE',  ( -18.39792479006713677, -22.19536379348757293, 68.85868763382491409 ) ) ;
#19304=CARTESIAN_POINT ( 'NONE',  ( -16.87480544004084493, -7.378732441012598287, 74.07362965403005717 ) ) ;
#19305=CARTESIAN_POINT ( 'NONE',  ( -14.61488608402547129, -21.70940465152681398, 58.34334805677458746 ) ) ;
#19306=ORIENTED_EDGE ( 'NONE', *, *, #27149, .F. ) ;
#19308=CARTESIAN_POINT ( 'NONE',  ( -12.88615340579958790, -8.900756115988826878, 67.47968544571848781 ) ) ;
#19310=CARTESIAN_POINT ( 'NONE',  ( -22.53429319464570924, -9.952421322533329118, 73.48161091678163359 ) ) ;
#19311=ORIENTED_EDGE ( 'NONE', *, *, #19393, .T. ) ;
#19315=CARTESIAN_POINT ( 'NONE',  ( -22.95709159497877394, -9.820362260273858723, 70.21167301517006365 ) ) ;
#19318=ADVANCED_FACE ( 'NONE', ( #4071 ), #16059, .T. ) ;
#19321=CARTESIAN_POINT ( 'NONE',  ( -20.42320230239022294, -8.483743783821255491, 67.06487496235745027 ) ) ;
#19322=CARTESIAN_POINT ( 'NONE',  ( -20.83700022493355775, -19.12221826660256951, 54.07175714974878389 ) ) ;
#19324=VERTEX_POINT ( 'NONE', #19555 ) ;
#19328=DIRECTION ( 'NONE',  ( -0.7029450532227031756, -0.7112441579020041260, 7.405715380709763191E-09 ) ) ;
#19330=CARTESIAN_POINT ( 'NONE',  ( -12.54360673743864574, -9.180396906553989211, 74.41899371332708313 ) ) ;
#19331=PLANE ( 'NONE',  #44294 ) ;
#19333=CARTESIAN_POINT ( 'NONE',  ( -10.33481637538221243, -12.51883299443452202, 60.84207650303104487 ) ) ;
#19335=CARTESIAN_POINT ( 'NONE',  ( -10.33193864190904421, -12.52760266535700318, 60.97570470297297618 ) ) ;
#19336=CARTESIAN_POINT ( 'NONE',  ( -24.47066272824306665, -14.57993217219608972, 62.99824437345091610 ) ) ;
#19338=CARTESIAN_POINT ( 'NONE',  ( -14.78754730678460660, -8.270772302057270764, 60.46996282000571199 ) ) ;
#19339=CARTESIAN_POINT ( 'NONE',  ( -20.88270815654435353, -21.40782497263450068, 58.82970582236164603 ) ) ;
#19341=FACE_BOUND ( 'NONE', #15981, .T. ) ;
#19343=EDGE_CURVE ( 'NONE', #33991, #27147, #46289, .T. ) ;
#19345=CARTESIAN_POINT ( 'NONE',  ( -13.60238447927381777, -8.884931327198675177, 57.11967755504965538 ) ) ;
#19347=CARTESIAN_POINT ( 'NONE',  ( -23.58525830889974984, -18.99772868593042219, 65.86743475655129032 ) ) ;
#19348=EDGE_CURVE ( 'NONE', #21537, #24440, #5521, .T. ) ;
#19350=ORIENTED_EDGE ( 'NONE', *, *, #37408, .T. ) ;
#19351=LINE ( 'NONE', #30455, #11109 ) ;
#19352=ADVANCED_FACE ( 'NONE', ( #19814 ), #16576, .T. ) ;
#19355=DIRECTION ( 'NONE',  ( -0.2465957053274583366, -0.9635866743705473469, 0.1033986416233890621 ) ) ;
#19356=EDGE_LOOP ( 'NONE', ( #35569, #21337, #37116, #30234, #34080 ) ) ;
#19357=CARTESIAN_POINT ( 'NONE',  ( -23.04367560227575140, -10.55211830211007218, 59.60203429193362012 ) ) ;
#19358=VERTEX_POINT ( 'NONE', #23761 ) ;
#19359=ORIENTED_EDGE ( 'NONE', *, *, #7835, .F. ) ;
#19360=ORIENTED_EDGE ( 'NONE', *, *, #36660, .T. ) ;
#19361=CARTESIAN_POINT ( 'NONE',  ( -22.23802311999876480, -19.89335690450594996, 69.28490980393287657 ) ) ;
#19362=CARTESIAN_POINT ( 'NONE',  ( -17.28496127917699710, -14.43418371046636217, 54.49999999999994316 ) ) ;
#19364=( BOUNDED_CURVE ( )  B_SPLINE_CURVE ( 3, ( #37555, #3596, #18362, #7316 ),
 .UNSPECIFIED., .F., .F. ) 
 B_SPLINE_CURVE_WITH_KNOTS ( ( 4, 4 ),
 ( 0.4074455897393651216, 0.5000000000000000000 ),
 .UNSPECIFIED. ) 
 CURVE ( )  GEOMETRIC_REPRESENTATION_ITEM ( )  RATIONAL_B_SPLINE_CURVE ( ( 0.6983129098260971723, 0.7760317562607096376, 0.8765941196520130596, 1.000000000000012657 ) ) 
 REPRESENTATION_ITEM ( '' )  );
#19365=CARTESIAN_POINT ( 'NONE',  ( -24.13566541640272334, -12.82032643073200440, 66.37534717750864388 ) ) ;
#19368=LINE ( 'NONE', #37579, #42529 ) ;
#19369=EDGE_CURVE ( 'NONE', #33919, #38352, #11149, .T. ) ;
#19370=ORIENTED_EDGE ( 'NONE', *, *, #33689, .T. ) ;
#19371=VERTEX_POINT ( 'NONE', #12405 ) ;
#19372=B_SPLINE_CURVE_WITH_KNOTS ( 'NONE', 3,
 ( #21368, #36356, #44028, #2634, #17641, #32672, #25299, #41524, #7561, #33621 ),
 .UNSPECIFIED., .F., .F.,
 ( 4, 2, 2, 2, 4 ),
 ( 0.6272669072877536944, 0.7522669073072811852, 0.8772669073268085649, 1.002266907346335945, 1.127266907365863435 ),
 .UNSPECIFIED. ) ;
#19373=CARTESIAN_POINT ( 'NONE',  ( -15.32518304399999387, -21.95751765168108349, 72.16080051677664642 ) ) ;
#19374=ADVANCED_FACE ( 'NONE', ( #8244 ), #24234, .T. ) ;
#19376=CARTESIAN_POINT ( 'NONE',  ( -13.18148061888732414, -8.602323747283376676, 54.02312124697527906 ) ) ;
#19378=CARTESIAN_POINT ( 'NONE',  ( -23.23311957587295495, -18.80921362937865382, 69.70860875969677295 ) ) ;
#19379=VERTEX_POINT ( 'NONE', #35050 ) ;
#19381=( BOUNDED_CURVE ( )  B_SPLINE_CURVE ( 3, ( #15292, #25661, #21977, #11144 ),
 .UNSPECIFIED., .F., .F. ) 
 B_SPLINE_CURVE_WITH_KNOTS ( ( 4, 4 ),
 ( 0.000000000000000000, 0.4074455897393662873 ),
 .UNSPECIFIED. ) 
 CURVE ( )  GEOMETRIC_REPRESENTATION_ITEM ( )  RATIONAL_B_SPLINE_CURVE ( ( 1.000000000000000000, 0.4567392136813295256, 0.3561768502900293787, 0.6983129098260995038 ) ) 
 REPRESENTATION_ITEM ( '' )  );
#19382=VECTOR ( 'NONE', #25949, 1000.000000000000114 ) ;
#19384=B_SPLINE_CURVE_WITH_KNOTS ( 'NONE', 3,
 ( #1743, #35937, #47290, #42864, #13762, #32017, #36177, #9858, #28073, #17472 ),
 .UNSPECIFIED., .F., .F.,
 ( 4, 2, 2, 2, 4 ),
 ( 0.6272669072878153118, 0.7522669073073335877, 0.8772669073268517526, 1.002266907346370139, 1.127266907365888304 ),
 .UNSPECIFIED. ) ;
#19385=ORIENTED_EDGE ( 'NONE', *, *, #36266, .T. ) ;
#19386=CARTESIAN_POINT ( 'NONE',  ( -16.16816302088245649, -21.69572814894516100, 58.28585623287596462 ) ) ;
#19387=CARTESIAN_POINT ( 'NONE',  ( -23.25757785049868787, -10.17517560731475967, 63.18690593950643120 ) ) ;
#19388=B_SPLINE_CURVE_WITH_KNOTS ( 'NONE', 1,
 ( #25325, #36142 ),
 .UNSPECIFIED., .F., .F.,
 ( 2, 2 ),
 ( 0.000000000000000000, 1.000000000000000000 ),
 .UNSPECIFIED. ) ;
#19389=CARTESIAN_POINT ( 'NONE',  ( -15.26068241199881648, -21.46662293872147842, 68.87592932306560556 ) ) ;
#19392=CARTESIAN_POINT ( 'NONE',  ( -22.05233278088557825, -8.971020610563387621, 63.35187109495049640 ) ) ;
#19393=EDGE_CURVE ( 'NONE', #12430, #22085, #29371, .T. ) ;
#19394=CARTESIAN_POINT ( 'NONE',  ( -12.15399223456666178, -9.543296633619027247, 57.20440205305690995 ) ) ;
#19396=CARTESIAN_POINT ( 'NONE',  ( -23.61204096558246235, -11.53669824655086451, 66.72214514747398084 ) ) ;
#19398=ORIENTED_EDGE ( 'NONE', *, *, #46255, .F. ) ;
#19399=CARTESIAN_POINT ( 'NONE',  ( -11.12358220677134035, -11.75903396576748605, 71.08860871065073184 ) ) ;
#19401=CARTESIAN_POINT ( 'NONE',  ( -10.31152747832866545, -17.02635028487499724, 57.86573311178444357 ) ) ;
#19402=CARTESIAN_POINT ( 'NONE',  ( -24.40614610099494541, -15.84163519271677956, 62.74895499471147531 ) ) ;
#19403=ORIENTED_EDGE ( 'NONE', *, *, #11661, .T. ) ;
#19404=DIRECTION ( 'NONE',  ( 0.1922068328301544116, 0.9813544382196450755, -7.804899501647045773E-08 ) ) ;
#19406=EDGE_CURVE ( 'NONE', #15202, #48304, #38156, .T. ) ;
#19408=CARTESIAN_POINT ( 'NONE',  ( -21.35242735686129478, -20.60316130439240112, 72.52446376371732129 ) ) ;
#19409=PRODUCT_DEFINITION_CONTEXT ( 'detailed design', #42294, 'design' ) ;
#19410=CARTESIAN_POINT ( 'NONE',  ( -11.10681587527927938, -11.67891925637714401, 71.10332952723315714 ) ) ;
#19412=CARTESIAN_POINT ( 'NONE',  ( -12.55788482626217650, -9.703832430577184809, 57.50424130074089391 ) ) ;
#19415=CARTESIAN_POINT ( 'NONE',  ( -23.31471867911119489, -19.37025309988949573, 59.08421845897321845 ) ) ;
#19417=ORIENTED_EDGE ( 'NONE', *, *, #10488, .T. ) ;
#19418=CARTESIAN_POINT ( 'NONE',  ( -24.84738384818810175, -14.17746907932909295, 69.77462523386947169 ) ) ;
#19423=CARTESIAN_POINT ( 'NONE',  ( -14.05371270701021480, -21.00138147690670820, 71.92607703580544865 ) ) ;
#19424=CARTESIAN_POINT ( 'NONE',  ( -24.11031341057265465, -17.05596264031881759, 69.62159819203986899 ) ) ;
#19425=CARTESIAN_POINT ( 'NONE',  ( -17.52853272358826686, -7.759682304905023642, 63.83584969886392457 ) ) ;
#19426=CARTESIAN_POINT ( 'NONE',  ( -10.79646186035629540, -11.40653701787342200, 67.66218675276181216 ) ) ;
#19427=ORIENTED_EDGE ( 'NONE', *, *, #45921, .F. ) ;
#19428=B_SPLINE_CURVE_WITH_KNOTS ( 'NONE', 3,
 ( #15171, #45015, #45490, #4596, #34136, #7825, #11992, #37332, #11748, #29978 ),
 .UNSPECIFIED., .F., .F.,
 ( 4, 2, 2, 2, 4 ),
 ( 0.1272669073658183880, 0.2522669073463058576, 0.3772669073267932438, 0.5022669073072807411, 0.6272669072877681273 ),
 .UNSPECIFIED. ) ;
#19429=CARTESIAN_POINT ( 'NONE',  ( -22.94085508618206859, -9.802298960702817254, 70.19673832247809742 ) ) ;
#19430=EDGE_CURVE ( 'NONE', #14105, #20348, #22296, .T. ) ;
#19433=CARTESIAN_POINT ( 'NONE',  ( -24.53366638517183773, -12.58233285770469578, 69.91096473585081128 ) ) ;
#19434=CARTESIAN_POINT ( 'NONE',  ( -12.46122051107220230, -19.81685944811288635, 64.88146935704573082 ) ) ;
#19435=VERTEX_POINT ( 'NONE', #35773 ) ;
#19436=EDGE_CURVE ( 'NONE', #5003, #18340, #7117, .T. ) ;
#19437=ADVANCED_FACE ( 'NONE', ( #36260 ), #11044, .T. ) ;
#19440=CARTESIAN_POINT ( 'NONE',  ( -23.82366728017863622, -10.99486018697619372, 73.47698013610775547 ) ) ;
#19441=CARTESIAN_POINT ( 'NONE',  ( -15.34627850953772743, -21.96360194435002455, 72.14601215069538398 ) ) ;
#19444=CARTESIAN_POINT ( 'NONE',  ( -13.02800281770400659, -9.361645100181775092, 71.14925385330717234 ) ) ;
#19446=VECTOR ( 'NONE', #38590, 1000.000000000000114 ) ;
#19447=CYLINDRICAL_SURFACE ( 'NONE', #32755, 0.1500000000000054345 ) ;
#19451=CARTESIAN_POINT ( 'NONE',  ( -11.10300763040008398, -10.86615618544839457, 57.39398486019972268 ) ) ;
#19452=CARTESIAN_POINT ( 'NONE',  ( -13.78028125966771178, -8.764572710043150749, 74.35521961121672518 ) ) ;
#19454=CARTESIAN_POINT ( 'NONE',  ( -21.76140116446488193, -9.313237301066212837, 66.73320317296904136 ) ) ;
#19455=ORIENTED_EDGE ( 'NONE', *, *, #29887, .F. ) ;
#19456=DIRECTION ( 'NONE',  ( 0.1453014101478983799, 0.9893874368562763921, 1.082933083898391864E-18 ) ) ;
#19457=CARTESIAN_POINT ( 'NONE',  ( -11.57017261513264117, -10.87519553945718620, 57.62392099249677102 ) ) ;
#19458=VERTEX_POINT ( 'NONE', #17547 ) ;
#19459=CARTESIAN_POINT ( 'NONE',  ( -11.98528268197933322, -9.717857698500944608, 60.70918086974133843 ) ) ;
#19460=CARTESIAN_POINT ( 'NONE',  ( -24.43113015230203544, -15.58634353390661964, 73.15303748141660378 ) ) ;
#19462=CARTESIAN_POINT ( 'NONE',  ( -10.74573065459234478, -12.54952415110468422, 60.81325645027152405 ) ) ;
#19463=CARTESIAN_POINT ( 'NONE',  ( -22.21838695824825294, -9.106656223178038800, 59.84358462373373300 ) ) ;
#19464=ORIENTED_EDGE ( 'NONE', *, *, #16524, .T. ) ;
#19467=CARTESIAN_POINT ( 'NONE',  ( -12.50766578132126305, -19.86205079821699115, 65.16674886870754335 ) ) ;
#19469=CARTESIAN_POINT ( 'NONE',  ( -24.76306277605930717, -16.09159651786607625, 66.22471475759273574 ) ) ;
#19472=CARTESIAN_POINT ( 'NONE',  ( -18.20082364030551503, -7.794104720362528660, 73.99631248270939921 ) ) ;
#19473=CARTESIAN_POINT ( 'NONE',  ( -10.35899127153216881, -12.44516180055180143, 60.92136665175527099 ) ) ;
#19474=ORIENTED_EDGE ( 'NONE', *, *, #14401, .F. ) ;
#19475=AXIS2_PLACEMENT_3D ( 'NONE', #12191, #42483, #1334 ) ;
#19476=LINE ( 'NONE', #30585, #24129 ) ;
#19477=CARTESIAN_POINT ( 'NONE',  ( -14.57480141982250998, -21.69281262657844067, 58.31617885369491461 ) ) ;
#19479=DIRECTION ( 'NONE',  ( -0.3667195576449454042, 0.9303315355510073381, 1.591455084066143578E-08 ) ) ;
#19480=CARTESIAN_POINT ( 'NONE',  ( -12.07387405703792460, -19.99358258471635708, 61.59689830162205482 ) ) ;
#19481=CARTESIAN_POINT ( 'NONE',  ( -11.40643119260009364, -19.20155754982889817, 71.82652555106689363 ) ) ;
#19483=CARTESIAN_POINT ( 'NONE',  ( -24.25068033110073173, -17.79252971020026663, 62.62360985091944343 ) ) ;
#19485=ORIENTED_EDGE ( 'NONE', *, *, #47663, .F. ) ;
#19487=EDGE_CURVE ( 'NONE', #13527, #33162, #44047, .T. ) ;
#19490=CARTESIAN_POINT ( 'NONE',  ( -13.90792234543431327, -20.92405545593893379, 64.98628592218737765 ) ) ;
#19491=CARTESIAN_POINT ( 'NONE',  ( -12.83007281553047108, -20.09077549419061626, 71.80653676829817300 ) ) ;
#19492=CARTESIAN_POINT ( 'NONE',  ( -18.12273512012592747, -22.22646200727865917, 65.46036854067777710 ) ) ;
#19493=VECTOR ( 'NONE', #41592, 1000.000000000000000 ) ;
#19494=ORIENTED_EDGE ( 'NONE', *, *, #30819, .F. ) ;
#19497=B_SPLINE_CURVE_WITH_KNOTS ( 'NONE', 3,
 ( #28656, #13370, #27686, #9470, #47381, #24495, #39734, #28420, #1577, #31378 ),
 .UNSPECIFIED., .F., .F.,
 ( 4, 2, 2, 2, 4 ),
 ( 0.000000000000000000, 0.2500000000000000000, 0.5000000000000000000, 0.7500000000000000000, 1.000000000000000000 ),
 .UNSPECIFIED. ) ;
#19499=CARTESIAN_POINT ( 'NONE',  ( -11.96084830514426400, -9.743959610980004626, 60.74413522332266524 ) ) ;
#19500=EDGE_CURVE ( 'NONE', #32337, #8240, #21119, .T. ) ;
#19501=CARTESIAN_POINT ( 'NONE',  ( -16.47491545697456061, -21.74461699364392686, 62.04102722053536212 ) ) ;
#19503=( BOUNDED_CURVE ( )  B_SPLINE_CURVE ( 3, ( #21897, #25121, #21435, #40141 ),
 .UNSPECIFIED., .F., .F. ) 
 B_SPLINE_CURVE_WITH_KNOTS ( ( 4, 4 ),
 ( 0.4074455897393699511, 0.5000000000000000000 ),
 .UNSPECIFIED. ) 
 CURVE ( )  GEOMETRIC_REPRESENTATION_ITEM ( )  RATIONAL_B_SPLINE_CURVE ( ( 0.6983129098261027234, 0.7760317562607084163, 0.8765941196520080636, 1.000000000000002887 ) ) 
 REPRESENTATION_ITEM ( '' )  );
#19505=CARTESIAN_POINT ( 'NONE',  ( -13.73970650151387751, -20.76112128469266693, 64.98628881673506896 ) ) ;
#19506=FACE_OUTER_BOUND ( 'NONE', #33186, .T. ) ;
#19507=ADVANCED_FACE ( 'NONE', ( #5989 ), #3009, .T. ) ;
#19508=ORIENTED_EDGE ( 'NONE', *, *, #4504, .F. ) ;
#19509=CARTESIAN_POINT ( 'NONE',  ( -23.80321451250838649, -17.81075939459467961, 59.00378417737415049 ) ) ;
#19511=DIRECTION ( 'NONE',  ( 0.3109111061729914471, 0.9504389954427826526, 3.354176643444177759E-08 ) ) ;
#19512=VECTOR ( 'NONE', #30100, 1000.000000000000114 ) ;
#19514=( BOUNDED_CURVE ( )  B_SPLINE_CURVE ( 3, ( #47038, #13281, #43362, #8815 ),
 .UNSPECIFIED., .F., .F. ) 
 B_SPLINE_CURVE_WITH_KNOTS ( ( 4, 4 ),
 ( 0.000000000000000000, 0.4074455897393678416 ),
 .UNSPECIFIED. ) 
 CURVE ( )  GEOMETRIC_REPRESENTATION_ITEM ( )  RATIONAL_B_SPLINE_CURVE ( ( 1.000000000000000000, 0.4567392136813320791, 0.3561768502900303779, 0.6983129098260949519 ) ) 
 REPRESENTATION_ITEM ( '' )  );
#19515=CARTESIAN_POINT ( 'NONE',  ( -14.72744631621160494, -8.295007313424175521, 60.60524229057013201 ) ) ;
#19516=VECTOR ( 'NONE', #9734, 1000.000000000000227 ) ;
#19518=VERTEX_POINT ( 'NONE', #28411 ) ;
#19521=CARTESIAN_POINT ( 'NONE',  ( -24.05845762361657947, -12.57644656616312773, 73.24225570276865938 ) ) ;
#19522=ORIENTED_EDGE ( 'NONE', *, *, #1154, .F. ) ;
#19523=CARTESIAN_POINT ( 'NONE',  ( -12.74836358285320159, -20.08597126951521261, 71.82125749157572159 ) ) ;
#19526=CARTESIAN_POINT ( 'NONE',  ( -18.31357888663955080, -21.80286911112441217, 69.11514702303101387 ) ) ;
#19529=CARTESIAN_POINT ( 'NONE',  ( -20.54979434103954006, -8.489990112051950533, 63.61121512946457557 ) ) ;
#19530=( BOUNDED_CURVE ( )  B_SPLINE_CURVE ( 3, ( #31135, #8257, #42720, #27689 ),
 .UNSPECIFIED., .F., .F. ) 
 B_SPLINE_CURVE_WITH_KNOTS ( ( 4, 4 ),
 ( 0.000000000000000000, 0.4074455897393666204 ),
 .UNSPECIFIED. ) 
 CURVE ( )  GEOMETRIC_REPRESENTATION_ITEM ( )  RATIONAL_B_SPLINE_CURVE ( ( 1.000000000000000000, 0.4567392136813317460, 0.3561768502900302114, 0.6983129098260953960 ) ) 
 REPRESENTATION_ITEM ( '' )  );
#19531=DIRECTION ( 'NONE',  ( -9.880513536971593873E-06, -1.241746728590076822E-06, 0.9999999999504166626 ) ) ;
#19532=CARTESIAN_POINT ( 'NONE',  ( -23.93063274373519178, -11.18025648668110783, 70.07023518370729676 ) ) ;
#19535=ORIENTED_EDGE ( 'NONE', *, *, #4783, .T. ) ;
#19537=CARTESIAN_POINT ( 'NONE',  ( -21.84079884060555088, -9.314189094968263305, 63.34153755726884327 ) ) ;
#19538=VERTEX_POINT ( 'NONE', #21016 ) ;
#19540=CARTESIAN_POINT ( 'NONE',  ( -24.46601827249642014, -14.47102098010720006, 66.18292729753066794 ) ) ;
#19541=CARTESIAN_POINT ( 'NONE',  ( -18.73521446872676322, -7.879141670414848697, 74.25553277440172906 ) ) ;
#19542=B_SPLINE_CURVE_WITH_KNOTS ( 'NONE', 3,
 ( #26265, #15161, #44755, #29968, #45006, #7817, #11252, #22832, #38062, #11738 ),
 .UNSPECIFIED., .F., .F.,
 ( 4, 2, 2, 2, 4 ),
 ( 0.000000000000000000, 0.2500000000000000000, 0.5000000000000000000, 0.7500000000000000000, 1.000000000000000000 ),
 .UNSPECIFIED. ) ;
#19543=EDGE_CURVE ( 'NONE', #21555, #46504, #7609, .T. ) ;
#19544=ORIENTED_EDGE ( 'NONE', *, *, #5345, .F. ) ;
#19545=CARTESIAN_POINT ( 'NONE',  ( -18.37786432726835883, -21.79469297182707521, 69.10042588711679912 ) ) ;
#19546=LINE ( 'NONE', #34556, #21004 ) ;
#19547=CARTESIAN_POINT ( 'NONE',  ( -12.04811195874215812, -10.23604714248314629, 60.71485379904431312 ) ) ;
#19548=ADVANCED_FACE ( 'NONE', ( #2295 ), #17644, .T. ) ;
#19549=ORIENTED_EDGE ( 'NONE', *, *, #36273, .F. ) ;
#19550=CARTESIAN_POINT ( 'NONE',  ( -11.32469144785209103, -18.34471071427194389, 57.80714594245691273 ) ) ;
#19554=CARTESIAN_POINT ( 'NONE',  ( -10.00037608677762258, -14.17511115329010707, 61.03165943758897782 ) ) ;
#19555=CARTESIAN_POINT ( 'NONE',  ( -19.86569447268031041, -19.73755174630646891, 53.49999999999995026 ) ) ;
#19556=CARTESIAN_POINT ( 'NONE',  ( -23.16129546718040189, -18.81986427065789158, 62.58080139315423907 ) ) ;
#19558=VECTOR ( 'NONE', #44119, 999.9999999999998863 ) ;
#19560=EDGE_LOOP ( 'NONE', ( #22820, #47582, #40553, #15255, #18236 ) ) ;
#19563=EDGE_CURVE ( 'NONE', #15772, #39638, #44642, .T. ) ;
#19566=CARTESIAN_POINT ( 'NONE',  ( -17.73224099643095286, -22.30287356026373047, 53.49999999999994316 ) ) ;
#19567=EDGE_CURVE ( 'NONE', #43051, #20660, #22712, .T. ) ;
#19569=CARTESIAN_POINT ( 'NONE',  ( -11.81042834955647258, -10.54382735031610174, 74.45357240259568243 ) ) ;
#19570=CARTESIAN_POINT ( 'NONE',  ( -17.98584164848810474, -22.23808382151284491, 62.06031347038508983 ) ) ;
#19571=CARTESIAN_POINT ( 'NONE',  ( -12.26752988409003287, -16.72227946798956921, 53.49999999999995026 ) ) ;
#19575=CARTESIAN_POINT ( 'NONE',  ( -21.20678976440764885, -20.70065158789174475, 72.59616802899515164 ) ) ;
#19576=CARTESIAN_POINT ( 'NONE',  ( -22.06352374043166265, -8.980015506435984562, 63.37649162950052784 ) ) ;
#19577=ORIENTED_EDGE ( 'NONE', *, *, #41809, .T. ) ;
#19578=CARTESIAN_POINT ( 'NONE',  ( -11.06712629860931152, -18.69414434431124761, 61.39215439313597500 ) ) ;
#19579=CARTESIAN_POINT ( 'NONE',  ( -9.974215857974789046, -14.86484893678357544, 74.91283499353951925 ) ) ;
#19580=CARTESIAN_POINT ( 'NONE',  ( -10.55151165865014384, -17.68520938540437371, 68.28217272534745064 ) ) ;
#19581=CARTESIAN_POINT ( 'NONE',  ( -13.22529448846758982, -9.145569705956512863, 64.19474388871357462 ) ) ;
#19583=CARTESIAN_POINT ( 'NONE',  ( -10.78898398081525301, -17.19290454168847404, 61.44271037915215317 ) ) ;
#19585=FACE_OUTER_BOUND ( 'NONE', #21476, .T. ) ;
#19587=ORIENTED_EDGE ( 'NONE', *, *, #759, .F. ) ;
#19588=CARTESIAN_POINT ( 'NONE',  ( -10.33960071559749494, -17.11462300555371030, 57.82614026527284778 ) ) ;
#19591=CARTESIAN_POINT ( 'NONE',  ( -23.77312829587014420, -18.70709569252041859, 72.87872954713984086 ) ) ;
#19592=CARTESIAN_POINT ( 'NONE',  ( -18.78767905735283605, -20.13749289187802916, 53.49999999999995026 ) ) ;
#19594=DIRECTION ( 'NONE',  ( -0.9999247414263406908, 0.01226831216845469807, 5.367905339378914507E-08 ) ) ;
#19595=CARTESIAN_POINT ( 'NONE',  ( -22.57893663749957369, -9.999394138389961384, 73.49633153340955971 ) ) ;
#19598=CARTESIAN_POINT ( 'NONE',  ( -20.66696756681432134, -21.06910030335248507, 58.64475164910060556 ) ) ;
#19599=VECTOR ( 'NONE', #15890, 1000.000000000000114 ) ;
#19603=ADVANCED_FACE ( 'NONE', ( #14544 ), #3499, .T. ) ;
#19604=VERTEX_POINT ( 'NONE', #18511 ) ;
#19606=FACE_BOUND ( 'NONE', #3079, .T. ) ;
#19607=ORIENTED_EDGE ( 'NONE', *, *, #43642, .F. ) ;
#19609=ORIENTED_EDGE ( 'NONE', *, *, #33045, .T. ) ;
#19610=CARTESIAN_POINT ( 'NONE',  ( -18.05557233295238362, -22.23314744338585669, 61.98880637900742130 ) ) ;
#19611=CARTESIAN_POINT ( 'NONE',  ( -12.61446418420489124, -20.49964817803554595, 71.91998392462126333 ) ) ;
#19613=B_SPLINE_CURVE_WITH_KNOTS ( 'NONE', 3,
 ( #35813, #47880, #36055, #17346, #46914, #13154, #13402, #2093, #36300, #28202 ),
 .UNSPECIFIED., .F., .F.,
 ( 4, 2, 2, 2, 4 ),
 ( 0.6272669072877499197, 0.7522669073072704160, 0.8772669073267909123, 1.002266907346311520, 1.127266907365831905 ),
 .UNSPECIFIED. ) ;
#19614=CARTESIAN_POINT ( 'NONE',  ( -23.83043763270304538, -11.86620476845630101, 59.48235732590899261 ) ) ;
#19616=ADVANCED_FACE ( 'NONE', ( #48081 ), #4425, .T. ) ;
#19617=CARTESIAN_POINT ( 'NONE',  ( -19.36486374868428584, -8.083171814817379897, 59.97709656101385889 ) ) ;
#19621=EDGE_CURVE ( 'NONE', #3056, #36780, #6960, .T. ) ;
#19622=CARTESIAN_POINT ( 'NONE',  ( -13.71339271347209987, -20.80363700974685059, 65.28628881287177421 ) ) ;
#19623=VECTOR ( 'NONE', #41778, 1000.000000000000227 ) ;
#19624=CARTESIAN_POINT ( 'NONE',  ( -19.30272045617997634, -8.014115550771089502, 59.96092997145631642 ) ) ;
#19625=CARTESIAN_POINT ( 'NONE',  ( -20.75210801675527605, -8.590061315918145368, 63.40301605188658129 ) ) ;
#19626=EDGE_LOOP ( 'NONE', ( #2566, #44566, #5292, #40750 ) ) ;
#19628=VECTOR ( 'NONE', #34677, 1000.000000000000000 ) ;
#19629=VECTOR ( 'NONE', #29849, 1000.000000000000000 ) ;
#19632=B_SPLINE_CURVE_WITH_KNOTS ( 'NONE', 1,
 ( #20957, #25137 ),
 .UNSPECIFIED., .F., .F.,
 ( 2, 2 ),
 ( 0.000000000000000000, 1.000000000000000000 ),
 .UNSPECIFIED. ) ;
#19634=CARTESIAN_POINT ( 'NONE',  ( -15.44116676862596549, -21.52247700621390436, 68.68478959089048885 ) ) ;
#19635=CARTESIAN_POINT ( 'NONE',  ( -24.46783000807617370, -17.23593667955698905, 73.07674329114531986 ) ) ;
#19637=EDGE_CURVE ( 'NONE', #18422, #47966, #35888, .T. ) ;
#19638=B_SPLINE_CURVE_WITH_KNOTS ( 'NONE', 1,
 ( #33075, #26207 ),
 .UNSPECIFIED., .F., .F.,
 ( 2, 2 ),
 ( 0.000000000000000000, 1.000000000000000000 ),
 .UNSPECIFIED. ) ;
#19641=CARTESIAN_POINT ( 'NONE',  ( -10.44938425464750331, -17.42781160170326871, 64.88385290183622089 ) ) ;
#19644=ORIENTED_EDGE ( 'NONE', *, *, #41324, .F. ) ;
#19646=( BOUNDED_SURFACE ( )  B_SPLINE_SURFACE ( 3, 1, ( 
 ( #10584, #2470 ),
 ( #29052, #17709 ),
 ( #47762, #18197 ),
 ( #21664, #2935 ),
 ( #44099, #13768 ),
 ( #29534, #3186 ),
 ( #37142, #17479 ) ),
 .UNSPECIFIED., .T., .F., .F. ) 
 B_SPLINE_SURFACE_WITH_KNOTS ( ( 4, 3, 4 ),
 ( 2, 2 ),
 ( 0.000000000000000000, 0.5000000000000000000, 1.000000000000000000 ),
 ( 0.000000000000000000, 1.000000000000000000 ),
 .UNSPECIFIED. ) 
 GEOMETRIC_REPRESENTATION_ITEM ( )  RATIONAL_B_SPLINE_SURFACE ( (
 ( 1.000000000000000000, 1.000000000000000000),
 ( 0.3333333333333335369, 0.3333333333333330373),
 ( 0.3333333333333335369, 0.3333333333333330373),
 ( 1.000000000000000000, 1.000000000000000000),
 ( 0.3333333333333333703, 0.3333333333333333703),
 ( 0.3333333333333333703, 0.3333333333333333703),
 ( 1.000000000000000000, 1.000000000000000000) ) ) 
 REPRESENTATION_ITEM ( '' )  SURFACE ( )  );
#19647=EDGE_CURVE ( 'NONE', #3179, #8795, #4089, .T. ) ;
#19648=B_SPLINE_CURVE_WITH_KNOTS ( 'NONE', 1,
 ( #30874, #30146 ),
 .UNSPECIFIED., .F., .F.,
 ( 2, 2 ),
 ( 0.000000000000000000, 1.000000000000000000 ),
 .UNSPECIFIED. ) ;
#19649=CARTESIAN_POINT ( 'NONE',  ( -22.94084456310974574, -19.11815116408422810, 59.18410675569454327 ) ) ;
#19650=CARTESIAN_POINT ( 'NONE',  ( -12.41053161536432725, -20.31997060906338248, 68.45844704426498595 ) ) ;
#19651=ORIENTED_EDGE ( 'NONE', *, *, #14379, .F. ) ;
#19654=ORIENTED_EDGE ( 'NONE', *, *, #41324, .T. ) ;
#19657=ORIENTED_EDGE ( 'NONE', *, *, #6171, .F. ) ;
#19659=CARTESIAN_POINT ( 'NONE',  ( -22.16593877863229878, -20.55544301355402581, 58.94255664220460744 ) ) ;
#19660=FACE_OUTER_BOUND ( 'NONE', #17038, .T. ) ;
#19661=DIRECTION ( 'NONE',  ( -0.1738928961406289164, 0.9847645711904029486, 7.871847295470929299E-08 ) ) ;
#19663=ORIENTED_EDGE ( 'NONE', *, *, #13629, .F. ) ;
#19665=CARTESIAN_POINT ( 'NONE',  ( -13.26872317195175199, -21.05283485551296607, 54.27966884056655061 ) ) ;
#19666=( BOUNDED_CURVE ( )  B_SPLINE_CURVE ( 3, ( #7078, #28988, #28750, #48182 ),
 .UNSPECIFIED., .F., .F. ) 
 B_SPLINE_CURVE_WITH_KNOTS ( ( 4, 4 ),
 ( 0.5000000000000000000, 0.9074455897393729487 ),
 .UNSPECIFIED. ) 
 CURVE ( )  GEOMETRIC_REPRESENTATION_ITEM ( )  RATIONAL_B_SPLINE_CURVE ( ( 1.000000000000021538, 0.4567392136813241410, 0.3561768502900121702, 0.6983129098261091627 ) ) 
 REPRESENTATION_ITEM ( '' )  );
#19667=CARTESIAN_POINT ( 'NONE',  ( -22.48964968825576705, -9.905448439006629968, 73.76689030015370463 ) ) ;
#19668=VERTEX_POINT ( 'NONE', #9333 ) ;
#19669=CARTESIAN_POINT ( 'NONE',  ( -12.10481839165579565, -9.592984239578061789, 57.13289628414671739 ) ) ;
#19672=VERTEX_POINT ( 'NONE', #20162 ) ;
#19673=VERTEX_POINT ( 'NONE', #28531 ) ;
#19674=CARTESIAN_POINT ( 'NONE',  ( -22.75923480142028055, -10.27751027444597653, 66.84182257657300852 ) ) ;
#19675=CARTESIAN_POINT ( 'NONE',  ( -10.69681097496852473, -11.60785472431778942, 71.22714364629104011 ) ) ;
#19679=CARTESIAN_POINT ( 'NONE',  ( -10.43125892716163960, -13.91323834088958122, 57.44825034920751960 ) ) ;
#19680=CARTESIAN_POINT ( 'NONE',  ( -12.15890832635194485, -9.538329179646957812, 57.26748263554841856 ) ) ;
#19681=CARTESIAN_POINT ( 'NONE',  ( -18.60508437019847960, -7.453401506293143797, 74.04075608594855851 ) ) ;
#19682=( BOUNDED_CURVE ( )  B_SPLINE_CURVE ( 3, ( #7600, #18645, #25806, #41074 ),
 .UNSPECIFIED., .F., .F. ) 
 B_SPLINE_CURVE_WITH_KNOTS ( ( 4, 4 ),
 ( 0.9074455897393630677, 1.000000000000000000 ),
 .UNSPECIFIED. ) 
 CURVE ( )  GEOMETRIC_REPRESENTATION_ITEM ( )  RATIONAL_B_SPLINE_CURVE ( ( 0.6983129098260782985, 0.7760317562606855457, 0.8765941196519927425, 1.000000000000000000 ) ) 
 REPRESENTATION_ITEM ( '' )  );
#19683=EDGE_LOOP ( 'NONE', ( #48060, #44946, #9612, #8459, #397 ) ) ;
#19684=ORIENTED_EDGE ( 'NONE', *, *, #40027, .F. ) ;
#19686=CARTESIAN_POINT ( 'NONE',  ( -13.77338061488629073, -21.30427811955188844, 68.56969753575143045 ) ) ;
#19687=CARTESIAN_POINT ( 'NONE',  ( -12.41310947992116098, -19.76871611099698001, 61.68206578716802113 ) ) ;
#19688=CARTESIAN_POINT ( 'NONE',  ( -18.39722185058254311, -7.818642594244027855, 70.52634850392742294 ) ) ;
#19691=EDGE_CURVE ( 'NONE', #28180, #44222, #31118, .T. ) ;
#19692=CARTESIAN_POINT ( 'NONE',  ( -11.75774308769439003, -19.00384223356172697, 71.98685884781659183 ) ) ;
#19693=CARTESIAN_POINT ( 'NONE',  ( -23.82284107231174630, -10.99348899561931781, 73.61839243124092036 ) ) ;
#19695=CARTESIAN_POINT ( 'NONE',  ( -22.11801181964649388, -9.023811091936513762, 63.44799684341401047 ) ) ;
#19696=CARTESIAN_POINT ( 'NONE',  ( -11.06311696324566007, -18.68765404749363768, 61.39993965581383151 ) ) ;
#19698=EDGE_LOOP ( 'NONE', ( #43356, #27450, #31264, #44955, #22699 ) ) ;
#19699=AXIS2_PLACEMENT_3D ( 'NONE', #10425, #9458, #18018 ) ;
#19700=CARTESIAN_POINT ( 'NONE',  ( -10.54364274917572963, -16.09770547908457061, 67.99270210874573195 ) ) ;
#19702=EDGE_LOOP ( 'NONE', ( #5135, #42785 ) ) ;
#19703=B_SPLINE_CURVE_WITH_KNOTS ( 'NONE', 3,
 ( #6172, #31790, #35469, #39168, #43610, #20214, #1990, #24656, #13536, #17482 ),
 .UNSPECIFIED., .F., .F.,
 ( 4, 2, 2, 2, 4 ),
 ( 0.6272669072782244282, 0.7522669073001253537, 0.8772669073220261682, 1.002266907343926983, 1.127266907365827908 ),
 .UNSPECIFIED. ) ;
#19704=CARTESIAN_POINT ( 'NONE',  ( -11.14114413899577904, -10.80566798617789459, 57.32407932063995304 ) ) ;
#19705=CARTESIAN_POINT ( 'NONE',  ( -14.25645962476006368, -8.507545769726087670, 74.61443249008125633 ) ) ;
#19707=CARTESIAN_POINT ( 'NONE',  ( -17.42409385541300892, -14.80920654474439324, 54.49999999999995026 ) ) ;
#19711=CARTESIAN_POINT ( 'NONE',  ( -17.78823985852933731, -7.818684566706888717, 60.08060768393342954 ) ) ;
#19713=DIRECTION ( 'NONE',  ( -0.3926557917762825700, 0.9196855055857631189, 5.808111630006007955E-09 ) ) ;
#19716=CARTESIAN_POINT ( 'NONE',  ( -24.76540221579651302, -16.07765826482591365, 66.17829537637275905 ) ) ;
#19717=VECTOR ( 'NONE', #20910, 1000.000000000000227 ) ;
#19719=CARTESIAN_POINT ( 'NONE',  ( -17.57433505571471599, -21.80920136837260159, 58.59480362143565202 ) ) ;
#19720=CARTESIAN_POINT ( 'NONE',  ( -22.21789835343034269, -9.106240630544798265, 59.89888112549417798 ) ) ;
#19721=CARTESIAN_POINT ( 'NONE',  ( -13.42747132184446990, -8.521758955768165222, 57.13114303280060824 ) ) ;
#19722=ORIENTED_EDGE ( 'NONE', *, *, #38747, .F. ) ;
#19723=CARTESIAN_POINT ( 'NONE',  ( -24.47401588439613818, -14.84236418521736134, 59.54300237059216983 ) ) ;
#19725=CYLINDRICAL_SURFACE ( 'NONE', #36086, 0.1500000000000000777 ) ;
#19726=VECTOR ( 'NONE', #45751, 1000.000000000000227 ) ;
#19727=FACE_OUTER_BOUND ( 'NONE', #4959, .T. ) ;
#19728=ORIENTED_EDGE ( 'NONE', *, *, #9237, .F. ) ;
#19729=ORIENTED_EDGE ( 'NONE', *, *, #30967, .T. ) ;
#19730=B_SPLINE_CURVE_WITH_KNOTS ( 'NONE', 3,
 ( #42137, #8402, #32271, #21184, #39888, #28334, #31537, #39646, #6159, #1489 ),
 .UNSPECIFIED., .F., .F.,
 ( 4, 2, 2, 2, 4 ),
 ( 0.000000000000000000, 0.2500000000000000000, 0.5000000000000000000, 0.7500000000000000000, 1.000000000000000000 ),
 .UNSPECIFIED. ) ;
#19731=AXIS2_PLACEMENT_3D ( 'NONE', #15143, #29453, #15380 ) ;
#19732=CARTESIAN_POINT ( 'NONE',  ( -24.50086468078332658, -12.48019312587592999, 73.40372080011530898 ) ) ;
#19734=CARTESIAN_POINT ( 'NONE',  ( -24.02536259471169444, -17.13930990111214925, 73.16719446933997517 ) ) ;
#19735=CARTESIAN_POINT ( 'NONE',  ( -23.42915847708036736, -11.11517115755410146, 73.64721174900437006 ) ) ;
#19737=CARTESIAN_POINT ( 'NONE',  ( -24.74210650470650918, -16.20599442878457452, 62.71515881785720836 ) ) ;
#19738=B_SPLINE_CURVE_WITH_KNOTS ( 'NONE', 3,
 ( #9560, #33993, #46009, #27771, #27529, #12263, #23606, #38611, #23849, #4893 ),
 .UNSPECIFIED., .F., .F.,
 ( 4, 2, 2, 2, 4 ),
 ( 0.1272669073658014571, 0.2522669073462826539, 0.3772669073267638229, 0.5022669073072449919, 0.6272669072877261609 ),
 .UNSPECIFIED. ) ;
#19739=CARTESIAN_POINT ( 'NONE',  ( -14.16114181629738589, -8.110937519819053421, 67.37319822901852717 ) ) ;
#19740=CARTESIAN_POINT ( 'NONE',  ( -11.29219319990544079, -18.28864530752396433, 57.82186711835544912 ) ) ;
#19742=PLANE ( 'NONE',  #23225 ) ;
#19743=ORIENTED_EDGE ( 'NONE', *, *, #45577, .F. ) ;
#19745=CARTESIAN_POINT ( 'NONE',  ( -16.12858474313192048, -22.14570131352578741, 58.43585568879253600 ) ) ;
#19749=CARTESIAN_POINT ( 'NONE',  ( -15.63656890543763112, -8.039962338392246721, 74.15155978326677655 ) ) ;
#19750=CARTESIAN_POINT ( 'NONE',  ( -13.87409341786790762, -20.84236815287593103, 68.75625181053004553 ) ) ;
#19751=CARTESIAN_POINT ( 'NONE',  ( -11.91470689456726717, -9.793200236000155101, 64.21569601040394559 ) ) ;
#19752=CARTESIAN_POINT ( 'NONE',  ( -14.89095713150699218, -21.33490654319496116, 61.63600435359662555 ) ) ;
#19754=VERTEX_POINT ( 'NONE', #32223 ) ;
#19756=ORIENTED_EDGE ( 'NONE', *, *, #41804, .F. ) ;
#19757=B_SPLINE_CURVE_WITH_KNOTS ( 'NONE', 3,
 ( #40059, #16667, #47207, #9787, #46727, #27761, #16425, #35858, #13200, #5364 ),
 .UNSPECIFIED., .F., .F.,
 ( 4, 2, 2, 2, 4 ),
 ( 0.6272669072877503638, 0.7522669073072690837, 0.8772669073267878037, 1.002266907346306635, 1.127266907365825244 ),
 .UNSPECIFIED. ) ;
#19758=LINE ( 'NONE', #15793, #46878 ) ;
#19759=VECTOR ( 'NONE', #31883, 1000.000000000000227 ) ;
#19761=CARTESIAN_POINT ( 'NONE',  ( -24.07714866641017792, -12.63257625550829033, 69.99916305551172968 ) ) ;
#19766=CARTESIAN_POINT ( 'NONE',  ( -13.73970969606274473, -20.76112332560825990, 65.28628881671112083 ) ) ;
#19768=CARTESIAN_POINT ( 'NONE',  ( -10.46334769751556593, -14.06892751230320826, 57.63928137823284459 ) ) ;
#19769=ORIENTED_EDGE ( 'NONE', *, *, #29798, .T. ) ;
#19770=CARTESIAN_POINT ( 'NONE',  ( -11.34161041692636651, -11.34373020466420279, 64.16498710548324880 ) ) ;
#19772=CARTESIAN_POINT ( 'NONE',  ( -12.26447506468708681, -20.18352723774274793, 65.00528407122952501 ) ) ;
#19774=CARTESIAN_POINT ( 'NONE',  ( -23.70015292207183322, -18.82353835121273988, 69.47867366044893345 ) ) ;
#19777=ORIENTED_EDGE ( 'NONE', *, *, #36660, .F. ) ;
#19778=CARTESIAN_POINT ( 'NONE',  ( -19.66015618626893868, -21.44380804025676923, 69.16312308005014131 ) ) ;
#19780=CARTESIAN_POINT ( 'NONE',  ( -24.12071557656922494, -11.54438865435207795, 63.06722852297808402 ) ) ;
#19782=CARTESIAN_POINT ( 'NONE',  ( -11.58645319427940024, -10.18053053143523279, 71.06918860465941634 ) ) ;
#19783=CARTESIAN_POINT ( 'NONE',  ( -24.47354813883760016, -12.39902559715248032, 73.42720875634239519 ) ) ;
#19785=DIRECTION ( 'NONE',  ( 0.3667195576449454042, -0.9303315355510073381, -1.591455084066186922E-08 ) ) ;
#19787=CARTESIAN_POINT ( 'NONE',  ( -17.82203991332369597, -7.766729491495081739, 63.85057028805255186 ) ) ;
#19788=EDGE_CURVE ( 'NONE', #37220, #30787, #6435, .T. ) ;
#19790=CARTESIAN_POINT ( 'NONE',  ( -10.47679702054951534, -15.67959025947600971, 64.69698733612924002 ) ) ;
#19793=ORIENTED_EDGE ( 'NONE', *, *, #27405, .F. ) ;
#19794=EDGE_CURVE ( 'NONE', #42912, #12909, #18144, .T. ) ;
#19795=CYLINDRICAL_SURFACE ( 'NONE', #13310, 0.1499999999999963585 ) ;
#19796=CARTESIAN_POINT ( 'NONE',  ( -24.28330220718811105, -16.20608195347976022, 59.31435516383907469 ) ) ;
#19798=CARTESIAN_POINT ( 'NONE',  ( -21.39967327233876659, -20.63170314183283693, 72.80974286114339122 ) ) ;
#19800=CARTESIAN_POINT ( 'NONE',  ( -23.26656235495780578, -10.18637482697468677, 63.21152651401433786 ) ) ;
#19802=ORIENTED_EDGE ( 'NONE', *, *, #27758, .F. ) ;
#19803=CARTESIAN_POINT ( 'NONE',  ( -24.40557713429137365, -14.30039287845891671, 66.29178820325090271 ) ) ;
#19804=CARTESIAN_POINT ( 'NONE',  ( -17.24553756445192221, -7.761319519027048308, 70.49595599234443455 ) ) ;
#19806=CARTESIAN_POINT ( 'NONE',  ( -12.00971629994662493, -9.691756596678954949, 60.67422760384662439 ) ) ;
#19808=ORIENTED_EDGE ( 'NONE', *, *, #21495, .F. ) ;
#19809=CARTESIAN_POINT ( 'NONE',  ( -11.35719102664687874, -18.40077844947705188, 58.09242476654641507 ) ) ;
#19810=AXIS2_PLACEMENT_3D ( 'NONE', #17817, #25239, #32143 ) ;
#19812=CARTESIAN_POINT ( 'NONE',  ( -10.42930205768512941, -13.90492575851057211, 61.33310083575204885 ) ) ;
#19813=( BOUNDED_CURVE ( )  B_SPLINE_CURVE ( 3, ( #5886, #25556, #2430, #28773 ),
 .UNSPECIFIED., .F., .F. ) 
 B_SPLINE_CURVE_WITH_KNOTS ( ( 4, 4 ),
 ( 0.9074455897393592929, 1.000000000000000000 ),
 .UNSPECIFIED. ) 
 CURVE ( )  GEOMETRIC_REPRESENTATION_ITEM ( )  RATIONAL_B_SPLINE_CURVE ( ( 0.6983129098260664191, 0.7760317562606752206, 0.8765941196519864143, 1.000000000000000000 ) ) 
 REPRESENTATION_ITEM ( '' )  );
#19814=FACE_OUTER_BOUND ( 'NONE', #10652, .T. ) ;
#19817=ORIENTED_EDGE ( 'NONE', *, *, #24304, .F. ) ;
#19819=CARTESIAN_POINT ( 'NONE',  ( -10.72552571836178181, -12.61109718544098790, 60.79853568372240602 ) ) ;
#19820=LINE ( 'NONE', #22526, #37039 ) ;
#19822=( BOUNDED_SURFACE ( )  B_SPLINE_SURFACE ( 3, 1, ( 
 ( #21723, #17539 ),
 ( #32565, #8180 ),
 ( #7208, #37202 ),
 ( #782, #12104 ),
 ( #30834, #34496 ),
 ( #11866, #41404 ),
 ( #11370, #7696 ) ),
 .UNSPECIFIED., .T., .F., .F. ) 
 B_SPLINE_SURFACE_WITH_KNOTS ( ( 4, 3, 4 ),
 ( 2, 2 ),
 ( 0.000000000000000000, 0.5000000000000000000, 1.000000000000000000 ),
 ( 0.000000000000000000, 1.000000000000000000 ),
 .UNSPECIFIED. ) 
 GEOMETRIC_REPRESENTATION_ITEM ( )  RATIONAL_B_SPLINE_SURFACE ( (
 ( 1.000000000000000000, 1.000000000000000000),
 ( 0.3333333333333335369, 0.3333333333333330373),
 ( 0.3333333333333335369, 0.3333333333333330373),
 ( 1.000000000000000000, 1.000000000000000000),
 ( 0.3333333333333333703, 0.3333333333333333703),
 ( 0.3333333333333333703, 0.3333333333333333703),
 ( 1.000000000000000000, 1.000000000000000000) ) ) 
 REPRESENTATION_ITEM ( '' )  SURFACE ( )  );
#19823=CARTESIAN_POINT ( 'NONE',  ( -17.79108452803360763, -21.84994637594637723, 58.69081321602850920 ) ) ;
#19824=CARTESIAN_POINT ( 'NONE',  ( -20.66848101912799862, -8.549761622307151754, 60.12653141481577990 ) ) ;
#19825=CARTESIAN_POINT ( 'NONE',  ( -10.41631042766677417, -15.61196327047340304, 64.59951812971527829 ) ) ;
#19826=CARTESIAN_POINT ( 'NONE',  ( -18.12273512012592747, -22.22646200727865917, 65.46036854067777710 ) ) ;
#19828=ORIENTED_EDGE ( 'NONE', *, *, #7889, .T. ) ;
#19829=CARTESIAN_POINT ( 'NONE',  ( -21.31800492490012999, -20.62620369199774117, 72.52446429884872714 ) ) ;
#19830=CARTESIAN_POINT ( 'NONE',  ( -10.09291391017891115, -16.13494330055838333, 68.16263215882007387 ) ) ;
#19831=VERTEX_POINT ( 'NONE', #44516 ) ;
#19834=ORIENTED_EDGE ( 'NONE', *, *, #18209, .T. ) ;
#19836=EDGE_CURVE ( 'NONE', #44310, #40803, #39308, .T. ) ;
#19838=CYLINDRICAL_SURFACE ( 'NONE', #48507, 0.1500000000000022427 ) ;
#19839=CARTESIAN_POINT ( 'NONE',  ( -20.03442169439229303, -8.314116961584396392, 70.35986449788516950 ) ) ;
#19841=ORIENTED_EDGE ( 'NONE', *, *, #17731, .F. ) ;
#19842=CARTESIAN_POINT ( 'NONE',  ( -13.83108299072750391, -21.33561835983412891, 72.04112301026525245 ) ) ;
#19843=CARTESIAN_POINT ( 'NONE',  ( -17.79355539233428374, -22.25020845511654954, 58.56586767823151263 ) ) ;
#19845=FACE_BOUND ( 'NONE', #8247, .T. ) ;
#19848=CARTESIAN_POINT ( 'NONE',  ( -23.42915847708036736, -11.11517115755410146, 73.64721174900437006 ) ) ;
#19849=ADVANCED_FACE ( 'NONE', ( #2657 ), #28999, .T. ) ;
#19853=EDGE_CURVE ( 'NONE', #26529, #40716, #34583, .T. ) ;
#19856=CARTESIAN_POINT ( 'NONE',  ( -20.64377408635552769, -21.08512125173600893, 62.20651549696969340 ) ) ;
#19857=ORIENTED_EDGE ( 'NONE', *, *, #23751, .T. ) ;
#19858=CARTESIAN_POINT ( 'NONE',  ( -23.71751471349159601, -11.63122711669449494, 63.23746208799618529 ) ) ;
#19859=FACE_BOUND ( 'NONE', #14774, .T. ) ;
#19862=ORIENTED_EDGE ( 'NONE', *, *, #8873, .T. ) ;
#19863=DIRECTION ( 'NONE',  ( -0.9796876409582463419, 0.2005296141562636081, 7.890952370353029293E-08 ) ) ;
#19864=CARTESIAN_POINT ( 'NONE',  ( -19.45281838860202228, -9.697037067072804106, 53.49899999999994549 ) ) ;
#19865=CARTESIAN_POINT ( 'NONE',  ( -16.38321341446914658, -21.78497919871296062, 65.64053219190310529 ) ) ;
#19866=EDGE_CURVE ( 'NONE', #2243, #10578, #9481, .T. ) ;
#19867=CARTESIAN_POINT ( 'NONE',  ( -14.58386023763418926, -8.409552415680012771, 67.37048090121328414 ) ) ;
#19868=CARTESIAN_POINT ( 'NONE',  ( -10.76270079184834749, -12.47665168726528506, 64.41269048358307714 ) ) ;
#19869=CARTESIAN_POINT ( 'NONE',  ( -12.56172001024846452, -20.45377019276184427, 71.99149100736865137 ) ) ;
#19870=ORIENTED_EDGE ( 'NONE', *, *, #15478, .T. ) ;
#19871=EDGE_LOOP ( 'NONE', ( #17682, #21813, #16185, #7179, #16965 ) ) ;
#19872=B_SPLINE_CURVE_WITH_KNOTS ( 'NONE', 3,
 ( #20903, #32473, #13727, #44296, #39612, #10063, #14436, #25557, #25086, #44062 ),
 .UNSPECIFIED., .F., .F.,
 ( 4, 2, 2, 2, 4 ),
 ( 0.1272669073658340144, 0.2522669073463233991, 0.3772669073268128392, 0.5022669073073022794, 0.6272669072877916641 ),
 .UNSPECIFIED. ) ;
#19874=DIRECTION ( 'NONE',  ( -0.9990515194385544140, -0.04354378839186318073, 1.103613758316041049E-08 ) ) ;
#19875=CARTESIAN_POINT ( 'NONE',  ( -21.05884094699671039, -21.31242506687340210, 62.22133086525234091 ) ) ;
#19876=CARTESIAN_POINT ( 'NONE',  ( -19.72874733844480488, -21.41900457955616588, 65.69159546287741591 ) ) ;
#19877=ORIENTED_EDGE ( 'NONE', *, *, #17680, .T. ) ;
#19880=CARTESIAN_POINT ( 'NONE',  ( -12.10599122619147749, -20.02663529450013513, 61.58173959111590534 ) ) ;
#19881=CARTESIAN_POINT ( 'NONE',  ( -17.24727489946581116, -7.811440102727049251, 67.21142879207842213 ) ) ;
#19888=CARTESIAN_POINT ( 'NONE',  ( -10.44551245922705185, -15.36195639909390742, 57.85176246259045740 ) ) ;
#19889=LINE ( 'NONE', #34893, #20487 ) ;
#19890=CARTESIAN_POINT ( 'NONE',  ( -12.41578987685235980, -20.32480987677443807, 68.47510952779386173 ) ) ;
#19891=ORIENTED_EDGE ( 'NONE', *, *, #1705, .F. ) ;
#19892=EDGE_LOOP ( 'NONE', ( #40313, #34996 ) ) ;
#19893=CARTESIAN_POINT ( 'NONE',  ( -15.41198273355754900, -21.57429164360176799, 65.26163917071316689 ) ) ;
#19894=CARTESIAN_POINT ( 'NONE',  ( -14.86627003481517839, -7.811970263561289762, 56.96504677300865893 ) ) ;
#19895=ORIENTED_EDGE ( 'NONE', *, *, #22750, .F. ) ;
#19896=CARTESIAN_POINT ( 'NONE',  ( -13.33011785382929304, -9.069340661520646663, 63.92418669539090814 ) ) ;
#19897=CARTESIAN_POINT ( 'NONE',  ( -23.78500266573477262, -11.88707733699690827, 59.78235732566622573 ) ) ;
#19898=CARTESIAN_POINT ( 'NONE',  ( -14.24557640779922352, -8.071278081433945317, 67.35951463815518991 ) ) ;
#19899=EDGE_CURVE ( 'NONE', #3049, #31720, #26157, .T. ) ;
#19900=CARTESIAN_POINT ( 'NONE',  ( -14.25068826455714621, -8.513811653308138716, 70.87957628655816222 ) ) ;
#19901=VERTEX_POINT ( 'NONE', #8080 ) ;
#19902=CARTESIAN_POINT ( 'NONE',  ( -9.995738443926455830, -14.24059931954510816, 64.50308448303212572 ) ) ;
#19904=EDGE_CURVE ( 'NONE', #27633, #2092, #48144, .T. ) ;
#19905=CARTESIAN_POINT ( 'NONE',  ( -20.59780922738080378, -8.569522135318988987, 63.32738143816840903 ) ) ;
#19907=CARTESIAN_POINT ( 'NONE',  ( -23.46293004877725252, -19.17220411032675997, 62.54681013563286029 ) ) ;
#19908=ORIENTED_EDGE ( 'NONE', *, *, #41539, .F. ) ;
#19909=CARTESIAN_POINT ( 'NONE',  ( -23.96075626263749214, -17.45014286185010377, 66.24357239682278475 ) ) ;
#19910=ADVANCED_FACE ( 'NONE', ( #23319 ), #29986, .F. ) ;
#19911=CARTESIAN_POINT ( 'NONE',  ( -21.47456293661849713, -9.038556783377254433, 70.41660404402310292 ) ) ;
#19912=ORIENTED_EDGE ( 'NONE', *, *, #813, .T. ) ;
#19915=CARTESIAN_POINT ( 'NONE',  ( -10.18364478422453345, -13.05433800282328960, 71.46474530336836040 ) ) ;
#19916=B_SPLINE_CURVE_WITH_KNOTS ( 'NONE', 3,
 ( #36275, #16340, #46407, #31629, #12661, #2065, #46655, #5283, #1826, #16825 ),
 .UNSPECIFIED., .F., .F.,
 ( 4, 2, 2, 2, 4 ),
 ( 0.1272669073658204419, 0.2522669073439322562, 0.3772669073220440428, 0.5022669073001558848, 0.6272669072782677269 ),
 .UNSPECIFIED. ) ;
#19917=EDGE_CURVE ( 'NONE', #4870, #18548, #23447, .T. ) ;
#19919=CARTESIAN_POINT ( 'NONE',  ( -11.64235137327199610, -18.84330536064715034, 68.36689631560025759 ) ) ;
#19920=CARTESIAN_POINT ( 'NONE',  ( -12.26902398874117495, -19.54473763108856943, 58.22682373989366766 ) ) ;
#19921=CARTESIAN_POINT ( 'NONE',  ( -19.78100189160110389, -21.87668917967754112, 65.58673452452636354 ) ) ;
#19925=CARTESIAN_POINT ( 'NONE',  ( -11.02242957576233273, -11.85532881267382166, 74.57312195644870201 ) ) ;
#19926=VECTOR ( 'NONE', #18523, 1000.000000000000000 ) ;
#19928=DIRECTION ( 'NONE',  ( -0.3566357048164924270, 0.9342435303763380050, -8.054691247152028744E-09 ) ) ;
#19929=CYLINDRICAL_SURFACE ( 'NONE', #4017, 0.1500000000000004385 ) ;
#19930=ADVANCED_FACE ( 'NONE', ( #38081 ), #2833, .T. ) ;
#19932=ORIENTED_EDGE ( 'NONE', *, *, #25791, .F. ) ;
#19934=CARTESIAN_POINT ( 'NONE',  ( -23.35641471936834535, -10.99444570894131168, 73.24704464419542660 ) ) ;
#19935=CARTESIAN_POINT ( 'NONE',  ( -15.62847675160137406, -21.57498509099777095, 72.15461454263183327 ) ) ;
#19937=( BOUNDED_SURFACE ( )  B_SPLINE_SURFACE ( 3, 1, ( 
 ( #20140, #31466 ),
 ( #28742, #21600 ),
 ( #3113, #32671 ),
 ( #2145, #18120 ),
 ( #10519, #14407 ),
 ( #13931, #17872 ),
 ( #10748, #6335 ) ),
 .UNSPECIFIED., .T., .F., .F. ) 
 B_SPLINE_SURFACE_WITH_KNOTS ( ( 4, 3, 4 ),
 ( 2, 2 ),
 ( 0.000000000000000000, 0.5000000000000000000, 1.000000000000000000 ),
 ( 0.000000000000000000, 1.000000000000000000 ),
 .UNSPECIFIED. ) 
 GEOMETRIC_REPRESENTATION_ITEM ( )  RATIONAL_B_SPLINE_SURFACE ( (
 ( 1.000000000000000000, 1.000000000000000000),
 ( 0.3333333333333335369, 0.3333333333333330373),
 ( 0.3333333333333335369, 0.3333333333333330373),
 ( 1.000000000000000000, 1.000000000000000000),
 ( 0.3333333333333333703, 0.3333333333333333703),
 ( 0.3333333333333333703, 0.3333333333333333703),
 ( 1.000000000000000000, 1.000000000000000000) ) ) 
 REPRESENTATION_ITEM ( '' )  SURFACE ( )  );
#19938=EDGE_CURVE ( 'NONE', #42817, #18995, #31638, .T. ) ;
#19940=CARTESIAN_POINT ( 'NONE',  ( -24.85911909788007179, -14.32540520456757172, 69.83930567627945152 ) ) ;
#19942=ORIENTED_EDGE ( 'NONE', *, *, #6264, .T. ) ;
#19943=CARTESIAN_POINT ( 'NONE',  ( -11.28158159523816728, -11.33292898549803240, 57.36470039992773451 ) ) ;
#19944=CARTESIAN_POINT ( 'NONE',  ( -10.42462062702805703, -14.89507852762941198, 74.79778901763455679 ) ) ;
#19945=( BOUNDED_CURVE ( )  B_SPLINE_CURVE ( 3, ( #44214, #27530, #35811, #10222 ),
 .UNSPECIFIED., .F., .F. ) 
 B_SPLINE_CURVE_WITH_KNOTS ( ( 4, 4 ),
 ( 0.5000000000000000000, 0.9074455897393709503 ),
 .UNSPECIFIED. ) 
 CURVE ( )  GEOMETRIC_REPRESENTATION_ITEM ( )  RATIONAL_B_SPLINE_CURVE ( ( 1.000000000000007327, 0.4567392136813255288, 0.3561768502900227173, 0.6983129098261068313 ) ) 
 REPRESENTATION_ITEM ( '' )  );
#19946=ORIENTED_EDGE ( 'NONE', *, *, #30019, .F. ) ;
#19947=( BOUNDED_CURVE ( )  B_SPLINE_CURVE ( 3, ( #26856, #18464, #41871, #3706 ),
 .UNSPECIFIED., .F., .F. ) 
 B_SPLINE_CURVE_WITH_KNOTS ( ( 4, 4 ),
 ( 0.000000000000000000, 0.4074455897393629566 ),
 .UNSPECIFIED. ) 
 CURVE ( )  GEOMETRIC_REPRESENTATION_ITEM ( )  RATIONAL_B_SPLINE_CURVE ( ( 1.000000000000000000, 0.4567392136813387959, 0.3561768502900328204, 0.6983129098260820733 ) ) 
 REPRESENTATION_ITEM ( '' )  );
#19949=ORIENTED_EDGE ( 'NONE', *, *, #11598, .F. ) ;
#19950=CARTESIAN_POINT ( 'NONE',  ( -17.22281210278579167, -7.361840297529252730, 70.60540404266352255 ) ) ;
#19951=CARTESIAN_POINT ( 'NONE',  ( -21.31115985637654120, -8.927249709250721921, 73.88656608925673197 ) ) ;
#19952=EDGE_LOOP ( 'NONE', ( #42612, #47325, #42126, #31995 ) ) ;
#19953=LINE ( 'NONE', #17626, #40369 ) ;
#19954=FACE_OUTER_BOUND ( 'NONE', #8781, .T. ) ;
#19957=CARTESIAN_POINT ( 'NONE',  ( -17.78823904182716120, -7.818684512505932993, 60.38060768393231825 ) ) ;
#19961=( BOUNDED_CURVE ( )  B_SPLINE_CURVE ( 3, ( #18353, #29695, #23054, #7546 ),
 .UNSPECIFIED., .F., .F. ) 
 B_SPLINE_CURVE_WITH_KNOTS ( ( 4, 4 ),
 ( 0.4074455897393651771, 0.5000000000000000000 ),
 .UNSPECIFIED. ) 
 CURVE ( )  GEOMETRIC_REPRESENTATION_ITEM ( )  RATIONAL_B_SPLINE_CURVE ( ( 0.6983129098260844048, 0.7760317562606871000, 0.8765941196519911882, 0.9999999999999941158 ) ) 
 REPRESENTATION_ITEM ( '' )  );
#19964=EDGE_CURVE ( 'NONE', #30264, #47790, #32747, .T. ) ;
#19965=CARTESIAN_POINT ( 'NONE',  ( -23.68074301380292823, -18.85356566062577599, 69.44371981100314883 ) ) ;
#19966=FACE_OUTER_BOUND ( 'NONE', #28352, .T. ) ;
#19968=ORIENTED_EDGE ( 'NONE', *, *, #26539, .F. ) ;
#19969=EDGE_CURVE ( 'NONE', #24011, #15202, #8544, .T. ) ;
#19970=CARTESIAN_POINT ( 'NONE',  ( -21.44791825677726038, -9.079743230750363381, 73.82958728338842036 ) ) ;
#19971=CARTESIAN_POINT ( 'NONE',  ( -14.59672178607931414, -8.347720424474937673, 60.20507679337548979 ) ) ;
#19973=CARTESIAN_POINT ( 'NONE',  ( -22.53655392111809164, -20.22829597721307948, 65.88917050827579658 ) ) ;
#19974=CARTESIAN_POINT ( 'NONE',  ( -15.60243201887541709, -21.62804181911354817, 68.73160055118694345 ) ) ;
#19976=CARTESIAN_POINT ( 'NONE',  ( -13.08297840233603182, -8.754478813416307403, 64.04913201435263659 ) ) ;
#19977=CARTESIAN_POINT ( 'NONE',  ( -10.66331429883175019, -17.94058386735023802, 71.68062945273115361 ) ) ;
#19979=ORIENTED_EDGE ( 'NONE', *, *, #16105, .T. ) ;
#19980=CARTESIAN_POINT ( 'NONE',  ( -22.64922984081423252, -10.07076843310239589, 66.54182118905438870 ) ) ;
#19982=CARTESIAN_POINT ( 'NONE',  ( -23.21383278545907558, -10.12064720979650190, 63.11540053722242050 ) ) ;
#19983=CARTESIAN_POINT ( 'NONE',  ( -17.67039274234547364, -7.813102812368692085, 63.83440432737404535 ) ) ;
#19984=CARTESIAN_POINT ( 'NONE',  ( -21.49816216734858898, -9.116934002111024782, 70.13132539266752019 ) ) ;
#19986=ADVANCED_FACE ( 'NONE', ( #5337 ), #27729, .T. ) ;
#19987=VERTEX_POINT ( 'NONE', #27971 ) ;
#19988=ORIENTED_EDGE ( 'NONE', *, *, #2970, .T. ) ;
#19991=B_SPLINE_CURVE_WITH_KNOTS ( 'NONE', 1,
 ( #1301, #30461 ),
 .UNSPECIFIED., .F., .F.,
 ( 2, 2 ),
 ( 0.000000000000000000, 1.000000000000000000 ),
 .UNSPECIFIED. ) ;
#19992=ORIENTED_EDGE ( 'NONE', *, *, #34287, .T. ) ;
#19994=ADVANCED_FACE ( 'NONE', ( #46699 ), #46931, .T. ) ;
#19995=EDGE_CURVE ( 'NONE', #44029, #34579, #4601, .T. ) ;
#19996=DIRECTION ( 'NONE',  ( 0.7800143876985550229, -0.6257615799833393666, 5.505484597913564244E-08 ) ) ;
#19998=CARTESIAN_POINT ( 'NONE',  ( -10.96452110319877704, -18.52097308172938739, 57.91440450685169594 ) ) ;
#19999=ORIENTED_EDGE ( 'NONE', *, *, #47720, .T. ) ;
#20000=CARTESIAN_POINT ( 'NONE',  ( -10.43073328261085386, -14.50439875238632403, 67.85800126138448718 ) ) ;
#20001=CARTESIAN_POINT ( 'NONE',  ( -10.89280251029460622, -11.22507333849785027, 64.33377325762776877 ) ) ;
#20002=ORIENTED_EDGE ( 'NONE', *, *, #2986, .T. ) ;
#20003=CARTESIAN_POINT ( 'NONE',  ( -18.05440415122280839, -21.83127237841607027, 65.36004252941745563 ) ) ;
#20005=ORIENTED_EDGE ( 'NONE', *, *, #11737, .F. ) ;
#20006=CARTESIAN_POINT ( 'NONE',  ( -19.48731947536727915, -21.55887828695198039, 69.07915298548451233 ) ) ;
#20007=CARTESIAN_POINT ( 'NONE',  ( -13.53325622885376944, -21.16256470055228789, 65.17124264509627096 ) ) ;
#20008=ORIENTED_EDGE ( 'NONE', *, *, #44427, .T. ) ;
#20009=CARTESIAN_POINT ( 'NONE',  ( -23.42626641412206823, -19.22254892098468204, 62.61052823878424078 ) ) ;
#20010=CARTESIAN_POINT ( 'NONE',  ( -22.22619444978876757, -20.50513558618911958, 58.94938304221643222 ) ) ;
#20013=CARTESIAN_POINT ( 'NONE',  ( -13.54792730259346456, -8.920061342218058797, 57.25495614889487683 ) ) ;
#20014=EDGE_CURVE ( 'NONE', #15909, #18272, #17921, .T. ) ;
#20015=CARTESIAN_POINT ( 'NONE',  ( -22.11764131551248269, -20.59576654024708731, 58.95098234965121264 ) ) ;
#20016=DIRECTION ( 'NONE',  ( -5.731567514496413899E-31, -1.020425574103664789E-16, -1.000000000000000000 ) ) ;
#20017=CARTESIAN_POINT ( 'NONE',  ( -10.82908108634309663, -17.30933488606310178, 68.51210539238705621 ) ) ;
#20018=CARTESIAN_POINT ( 'NONE',  ( -12.79725860806972904, -20.12850118792689358, 71.95653676770096752 ) ) ;
#20022=VECTOR ( 'NONE', #24598, 999.9999999999998863 ) ;
#20023=CARTESIAN_POINT ( 'NONE',  ( -21.35673258969864818, -10.96416394607318878, 53.49999999999995026 ) ) ;
#20028=ORIENTED_EDGE ( 'NONE', *, *, #39444, .T. ) ;
#20030=CARTESIAN_POINT ( 'NONE',  ( -14.79551189520038967, -8.264331297124348552, 64.20467431377564083 ) ) ;
#20031=DIRECTION ( 'NONE',  ( 0.3374354101627464186, 0.9413486835218386473, 1.423378189492272593E-08 ) ) ;
#20032=CARTESIAN_POINT ( 'NONE',  ( -22.78003227265734765, -10.21913417830377036, 63.07185788080192879 ) ) ;
#20033=CARTESIAN_POINT ( 'NONE',  ( -10.40127108354264429, -12.32249413655887871, 57.51352655450988749 ) ) ;
#20035=CARTESIAN_POINT ( 'NONE',  ( -24.41485940220508510, -14.44976662329334616, 66.18292729254385165 ) ) ;
#20036=CARTESIAN_POINT ( 'NONE',  ( -10.45859239952313224, -15.89938452881993847, 64.79299464097340433 ) ) ;
#20037=CARTESIAN_POINT ( 'NONE',  ( -10.00761947527410634, -15.51609109068450465, 57.75288224187332276 ) ) ;
#20038=VERTEX_POINT ( 'NONE', #42278 ) ;
#20039=CARTESIAN_POINT ( 'NONE',  ( -12.64995486802317082, -19.99670083032576429, 68.33657438322859434 ) ) ;
#20040=( BOUNDED_SURFACE ( )  B_SPLINE_SURFACE ( 3, 1, ( 
 ( #18872, #15158 ),
 ( #40132, #13755 ),
 ( #11482, #29039 ),
 ( #21178, #26506 ),
 ( #32725, #10339 ),
 ( #22829, #6394 ),
 ( #36409, #37316 ) ),
 .UNSPECIFIED., .T., .F., .F. ) 
 B_SPLINE_SURFACE_WITH_KNOTS ( ( 4, 3, 4 ),
 ( 2, 2 ),
 ( 0.000000000000000000, 0.5000000000000000000, 1.000000000000000000 ),
 ( 0.000000000000000000, 1.000000000000000000 ),
 .UNSPECIFIED. ) 
 GEOMETRIC_REPRESENTATION_ITEM ( )  RATIONAL_B_SPLINE_SURFACE ( (
 ( 1.000000000000000000, 1.000000000000000000),
 ( 0.3333333333333335369, 0.3333333333333330373),
 ( 0.3333333333333335369, 0.3333333333333330373),
 ( 1.000000000000000000, 1.000000000000000000),
 ( 0.3333333333333333703, 0.3333333333333333703),
 ( 0.3333333333333333703, 0.3333333333333333703),
 ( 1.000000000000000000, 1.000000000000000000) ) ) 
 REPRESENTATION_ITEM ( '' )  SURFACE ( )  );
#20041=FACE_OUTER_BOUND ( 'NONE', #34604, .T. ) ;
#20042=CARTESIAN_POINT ( 'NONE',  ( -17.58247036098680027, -9.298045829720972932, 53.88362224778186516 ) ) ;
#20045=ORIENTED_EDGE ( 'NONE', *, *, #14278, .F. ) ;
#20048=EDGE_CURVE ( 'NONE', #10747, #43494, #12467, .T. ) ;
#20049=ADVANCED_FACE ( 'NONE', ( #34871 ), #6009, .T. ) ;
#20050=CARTESIAN_POINT ( 'NONE',  ( -19.96994574550859980, -21.32983827578761193, 72.40478737306770540 ) ) ;
#20051=CARTESIAN_POINT ( 'NONE',  ( -15.35027142736847239, -7.653576728715946409, 74.26480947788739684 ) ) ;
#20054=EDGE_CURVE ( 'NONE', #47542, #14105, #14449, .T. ) ;
#20055=CARTESIAN_POINT ( 'NONE',  ( -19.30706890485013005, -22.01740903849647069, 58.64011989901568711 ) ) ;
#20056=CARTESIAN_POINT ( 'NONE',  ( -20.88147674714181079, -8.209942860146695054, 60.02620543942160225 ) ) ;
#20058=CARTESIAN_POINT ( 'NONE',  ( -9.982716906467198115, -14.44908523835941594, 67.97304809435139816 ) ) ;
#20059=CARTESIAN_POINT ( 'NONE',  ( -24.23061318975584300, -17.83844832426134275, 62.61327595999730278 ) ) ;
#20060=ORIENTED_EDGE ( 'NONE', *, *, #46088, .T. ) ;
#20061=CARTESIAN_POINT ( 'NONE',  ( -23.66043351732632871, -18.11420823279021519, 59.14811234476497503 ) ) ;
#20064=CARTESIAN_POINT ( 'NONE',  ( -10.33483191699034265, -17.09962811228164270, 57.73114616685904110 ) ) ;
#20068=EDGE_CURVE ( 'NONE', #43006, #12881, #16351, .T. ) ;
#20069=CARTESIAN_POINT ( 'NONE',  ( -10.00117625416208433, -15.44487358686203571, 57.68297391752145842 ) ) ;
#20070=CARTESIAN_POINT ( 'NONE',  ( -21.84598475011588903, -8.812495317756813051, 70.31787921227815730 ) ) ;
#20071=CARTESIAN_POINT ( 'NONE',  ( -24.32752865423570654, -15.96790753223159598, 66.36324927017490438 ) ) ;
#20072=ORIENTED_EDGE ( 'NONE', *, *, #17610, .T. ) ;
#20075=CARTESIAN_POINT ( 'NONE',  ( -23.77395946432122997, -18.70572718374853594, 73.02014183918953449 ) ) ;
#20076=FACE_BOUND ( 'NONE', #15235, .T. ) ;
#20078=FACE_OUTER_BOUND ( 'NONE', #31587, .T. ) ;
#20079=CARTESIAN_POINT ( 'NONE',  ( -14.42683414290149813, -8.428067600363897682, 67.25975083869262505 ) ) ;
#20082=CARTESIAN_POINT ( 'NONE',  ( -10.70313947777602692, -12.85204326357734494, 64.26836087226253369 ) ) ;
#20083=EDGE_LOOP ( 'NONE', ( #10280, #45481, #20483, #30027, #12253 ) ) ;
#20085=CARTESIAN_POINT ( 'NONE',  ( -16.73406348812019928, -22.22719469671659809, 68.79586406416278521 ) ) ;
#20086=( BOUNDED_CURVE ( )  B_SPLINE_CURVE ( 3, ( #25481, #6538, #10957, #6292 ),
 .UNSPECIFIED., .F., .F. ) 
 B_SPLINE_CURVE_WITH_KNOTS ( ( 4, 4 ),
 ( 0.4074455897393650106, 0.5000000000000000000 ),
 .UNSPECIFIED. ) 
 CURVE ( )  GEOMETRIC_REPRESENTATION_ITEM ( )  RATIONAL_B_SPLINE_CURVE ( ( 0.6983129098260945078, 0.7760317562606938724, 0.8765941196519940748, 0.9999999999999911182 ) ) 
 REPRESENTATION_ITEM ( '' )  );
#20088=FACE_OUTER_BOUND ( 'NONE', #7834, .T. ) ;
#20090=FACE_BOUND ( 'NONE', #27769, .T. ) ;
#20091=ORIENTED_EDGE ( 'NONE', *, *, #1190, .T. ) ;
#20094=CARTESIAN_POINT ( 'NONE',  ( -10.43098718212803000, -15.70539730037032911, 61.32316937334011442 ) ) ;
#20097=CARTESIAN_POINT ( 'NONE',  ( -10.96921284960095377, -11.97350354382807680, 74.84368195529052059 ) ) ;
#20098=CARTESIAN_POINT ( 'NONE',  ( -16.29006019099003666, -22.17251760029243712, 61.87851267503305053 ) ) ;
#20099=( BOUNDED_CURVE ( )  B_SPLINE_CURVE ( 3, ( #47494, #43805, #17671, #35897 ),
 .UNSPECIFIED., .F., .F. ) 
 B_SPLINE_CURVE_WITH_KNOTS ( ( 4, 4 ),
 ( 0.4074455897393731707, 0.5000000000000000000 ),
 .UNSPECIFIED. ) 
 CURVE ( )  GEOMETRIC_REPRESENTATION_ITEM ( )  RATIONAL_B_SPLINE_CURVE ( ( 0.6983129098261171563, 0.7760317562606884323, 0.8765941196519738687, 0.9999999999999514833 ) ) 
 REPRESENTATION_ITEM ( '' )  );
#20100=VERTEX_POINT ( 'NONE', #8454 ) ;
#20104=CARTESIAN_POINT ( 'NONE',  ( -22.42594789675818845, -19.77792426076253918, 69.45945937764655298 ) ) ;
#20106=CARTESIAN_POINT ( 'NONE',  ( -21.49815937814055999, -9.116931945208399668, 70.43132539264750847 ) ) ;
#20107=ORIENTED_EDGE ( 'NONE', *, *, #29379, .F. ) ;
#20109=B_SPLINE_CURVE_WITH_KNOTS ( 'NONE', 1,
 ( #20911, #35907 ),
 .UNSPECIFIED., .F., .F.,
 ( 2, 2 ),
 ( 0.000000000000000000, 1.000000000000000000 ),
 .UNSPECIFIED. ) ;
#20111=VERTEX_POINT ( 'NONE', #8710 ) ;
#20112=CARTESIAN_POINT ( 'NONE',  ( -23.09439563802003903, -10.70187420503893883, 59.79130591064781441 ) ) ;
#20115=DIRECTION ( 'NONE',  ( -1.140458109893898545E-06, -1.256740822519431765E-06, 0.9999999999985598187 ) ) ;
#20117=EDGE_LOOP ( 'NONE', ( #45150, #39861, #7114, #4588, #14959 ) ) ;
#20120=CARTESIAN_POINT ( 'NONE',  ( -10.74628672884880309, -17.07053172313825939, 61.17215199736627795 ) ) ;
#20122=CARTESIAN_POINT ( 'NONE',  ( -24.20565986263710201, -11.72478542327168327, 59.58961564006824574 ) ) ;
#20123=VERTEX_POINT ( 'NONE', #30392 ) ;
#20124=B_SPLINE_CURVE_WITH_KNOTS ( 'NONE', 3,
 ( #17410, #8959, #18875, #27176, #7563, #8719, #38488, #30885, #12158, #46131 ),
 .UNSPECIFIED., .F., .F.,
 ( 4, 2, 2, 2, 4 ),
 ( 0.1272669073658516392, 0.2522669073439419707, 0.3772669073220322744, 0.5022669073001225781, 0.6272669072782128818 ),
 .UNSPECIFIED. ) ;
#20125=CARTESIAN_POINT ( 'NONE',  ( -10.44902906966473388, -15.40082580494429365, 57.86792826000680634 ) ) ;
#20126=CARTESIAN_POINT ( 'NONE',  ( -24.82319332931276179, -15.68001985351029681, 73.16450280174184684 ) ) ;
#20127=CARTESIAN_POINT ( 'NONE',  ( -12.41595477954341575, -20.32496163943406842, 68.49690828407896959 ) ) ;
#20128=ORIENTED_EDGE ( 'NONE', *, *, #28355, .F. ) ;
#20130=VERTEX_POINT ( 'NONE', #15827 ) ;
#20132=CARTESIAN_POINT ( 'NONE',  ( -15.16478962180274870, -8.127860897350485558, 57.26488623981089177 ) ) ;
#20133=VERTEX_POINT ( 'NONE', #11662 ) ;
#20136=CARTESIAN_POINT ( 'NONE',  ( -15.12736045941317897, -21.89643407171298151, 68.69097498501147925 ) ) ;
#20137=CARTESIAN_POINT ( 'NONE',  ( -11.55897615675186785, -7.397247749063358135, 53.49999999999995026 ) ) ;
#20138=ORIENTED_EDGE ( 'NONE', *, *, #39785, .T. ) ;
#20139=DIRECTION ( 'NONE',  ( -5.731567514496413899E-31, -1.020425574103664789E-16, -1.000000000000000000 ) ) ;
#20140=CARTESIAN_POINT ( 'NONE',  ( -11.22844613476422460, -11.44458948612160043, 64.43409918096024569 ) ) ;
#20142=CARTESIAN_POINT ( 'NONE',  ( -22.28894518008692316, -9.166670731632796887, 59.88317716683520331 ) ) ;
#20143=ORIENTED_EDGE ( 'NONE', *, *, #16939, .T. ) ;
#20144=CARTESIAN_POINT ( 'NONE',  ( -10.38752013045322009, -14.36951432065623813, 64.67331771650336236 ) ) ;
#20145=CARTESIAN_POINT ( 'NONE',  ( -11.03038783319414939, -18.63467225643333336, 61.46366213062071182 ) ) ;
#20147=VERTEX_POINT ( 'NONE', #45891 ) ;
#20148=CARTESIAN_POINT ( 'NONE',  ( -24.12071508562369715, -11.54438765950021306, 63.06722961171875852 ) ) ;
#20149=CARTESIAN_POINT ( 'NONE',  ( -20.00853194199203600, -21.31477305597513094, 72.40478738567958317 ) ) ;
#20150=CARTESIAN_POINT ( 'NONE',  ( -10.42707437616525645, -14.56501420157307791, 71.55612484073525081 ) ) ;
#20152=CARTESIAN_POINT ( 'NONE',  ( -10.56492563526530581, -13.18000101695786341, 71.20828586226983248 ) ) ;
#20153=EDGE_CURVE ( 'NONE', #22320, #34081, #16352, .T. ) ;
#20156=CARTESIAN_POINT ( 'NONE',  ( -11.32173637914110742, -11.26291225165672927, 67.76297573134488061 ) ) ;
#20157=VECTOR ( 'NONE', #27265, 1000.000000000000227 ) ;
#20161=CARTESIAN_POINT ( 'NONE',  ( -10.67448150008226904, -11.65383075329928886, 74.74495363721690921 ) ) ;
#20162=CARTESIAN_POINT ( 'NONE',  ( -22.72031779163844334, -16.29245029320677673, 54.07175714974878389 ) ) ;
#20163=CYLINDRICAL_SURFACE ( 'NONE', #23293, 0.1500000000000042133 ) ;
#20165=VERTEX_POINT ( 'NONE', #19291 ) ;
#20167=CARTESIAN_POINT ( 'NONE',  ( -12.96988148894724624, -20.27865218021415572, 71.80653631827996719 ) ) ;
#20168=EDGE_CURVE ( 'NONE', #18224, #11801, #29599, .T. ) ;
#20169=CARTESIAN_POINT ( 'NONE',  ( -21.79028809537168243, -9.273590339475653366, 63.47681654923867711 ) ) ;
#20170=CARTESIAN_POINT ( 'NONE',  ( -11.08048641648777100, -18.71577166677792547, 61.47722039269356742 ) ) ;
#20172=VERTEX_POINT ( 'NONE', #17026 ) ;
#20173=CARTESIAN_POINT ( 'NONE',  ( -24.85346453946240786, -14.25412306239375049, 69.90921191474365060 ) ) ;
#20175=CARTESIAN_POINT ( 'NONE',  ( -19.24025795797341942, -7.996846695050864540, 60.24620885950562865 ) ) ;
#20176=ORIENTED_EDGE ( 'NONE', *, *, #1704, .T. ) ;
#20177=CARTESIAN_POINT ( 'NONE',  ( -18.36404507162783162, -22.19967278815455458, 68.96514700280405918 ) ) ;
#20179=CARTESIAN_POINT ( 'NONE',  ( -24.25171713147202368, -16.35308467727669068, 59.12332432120680181 ) ) ;
#20181=CARTESIAN_POINT ( 'NONE',  ( -20.31007010532247037, -7.940766544821113548, 70.37287609157104384 ) ) ;
#20185=FACE_OUTER_BOUND ( 'NONE', #29074, .T. ) ;
#20186=CARTESIAN_POINT ( 'NONE',  ( -18.60622096112062707, -22.16490860957766529, 72.47006221837980888 ) ) ;
#20187=EDGE_LOOP ( 'NONE', ( #25482, #10075, #22575, #40391, #19070 ) ) ;
#20190=ORIENTED_EDGE ( 'NONE', *, *, #14187, .T. ) ;
#20191=CARTESIAN_POINT ( 'NONE',  ( -23.34481426128875015, -18.63642081788813343, 69.29371984264746231 ) ) ;
#20193=CARTESIAN_POINT ( 'NONE',  ( -10.63534001824907449, -11.74074953021217382, 74.75851385465050214 ) ) ;
#20194=LINE ( 'NONE', #31525, #40766 ) ;
#20196=CARTESIAN_POINT ( 'NONE',  ( -16.19438353473653436, -7.918004163840022258, 60.48563071257218127 ) ) ;
#20197=CARTESIAN_POINT ( 'NONE',  ( -11.73296596577226936, -10.64774513788296240, 74.72412863062541533 ) ) ;
#20200=CARTESIAN_POINT ( 'NONE',  ( -24.68275054790482770, -16.48720572190336853, 59.23837039904986312 ) ) ;
#20202=ORIENTED_EDGE ( 'NONE', *, *, #1843, .T. ) ;
#20203=FACE_OUTER_BOUND ( 'NONE', #8898, .T. ) ;
#20205=ORIENTED_EDGE ( 'NONE', *, *, #32241, .F. ) ;
#20206=CARTESIAN_POINT ( 'NONE',  ( -15.93879930885703011, -7.917138641544859468, 67.15479422225766371 ) ) ;
#20210=EDGE_CURVE ( 'NONE', #897, #188, #17279, .T. ) ;
#20211=CARTESIAN_POINT ( 'NONE',  ( -10.98557796499954087, -17.68114198556070704, 71.86718193507100239 ) ) ;
#20212=ORIENTED_EDGE ( 'NONE', *, *, #27682, .F. ) ;
#20214=CARTESIAN_POINT ( 'NONE',  ( -13.02047698205977433, -8.799930754719115455, 64.01608198847371511 ) ) ;
#20218=( BOUNDED_CURVE ( )  B_SPLINE_CURVE ( 3, ( #11247, #8061, #18367, #22083 ),
 .UNSPECIFIED., .F., .F. ) 
 B_SPLINE_CURVE_WITH_KNOTS ( ( 4, 4 ),
 ( 1.570796326794896780, 1.780235837034216617 ),
 .UNSPECIFIED. ) 
 CURVE ( )  GEOMETRIC_REPRESENTATION_ITEM ( )  RATIONAL_B_SPLINE_CURVE ( ( 1.000000000000000000, 0.9963479302455154896, 0.9963479302455154896, 1.000000000000000000 ) ) 
 REPRESENTATION_ITEM ( '' )  );
#20219=EDGE_CURVE ( 'NONE', #44556, #17241, #36321, .T. ) ;
#20220=ORIENTED_EDGE ( 'NONE', *, *, #35174, .F. ) ;
#20222=ORIENTED_EDGE ( 'NONE', *, *, #43997, .F. ) ;
#20225=CARTESIAN_POINT ( 'NONE',  ( -24.47368665962210343, -14.70950332193510413, 62.72768537250228604 ) ) ;
#20226=FACE_OUTER_BOUND ( 'NONE', #8145, .T. ) ;
#20228=VERTEX_POINT ( 'NONE', #20023 ) ;
#20229=( BOUNDED_SURFACE ( )  B_SPLINE_SURFACE ( 3, 1, ( 
 ( #28771, #10307 ),
 ( #43804, #10059 ),
 ( #25082, #6364 ),
 ( #21396, #17670 ),
 ( #40335, #26534 ),
 ( #446, #27259 ),
 ( #23578, #33916 ) ),
 .UNSPECIFIED., .T., .F., .F. ) 
 B_SPLINE_SURFACE_WITH_KNOTS ( ( 4, 3, 4 ),
 ( 2, 2 ),
 ( 0.000000000000000000, 0.5000000000000000000, 1.000000000000000000 ),
 ( 0.000000000000000000, 1.000000000000000000 ),
 .UNSPECIFIED. ) 
 GEOMETRIC_REPRESENTATION_ITEM ( )  RATIONAL_B_SPLINE_SURFACE ( (
 ( 1.000000000000000000, 1.000000000000000000),
 ( 0.3333333333333335369, 0.3333333333333330373),
 ( 0.3333333333333335369, 0.3333333333333330373),
 ( 1.000000000000000000, 1.000000000000000000),
 ( 0.3333333333333333703, 0.3333333333333333703),
 ( 0.3333333333333333703, 0.3333333333333333703),
 ( 1.000000000000000000, 1.000000000000000000) ) ) 
 REPRESENTATION_ITEM ( '' )  SURFACE ( )  );
#20230=CARTESIAN_POINT ( 'NONE',  ( -10.81696127132008023, -11.36705524461777905, 67.81875810329987075 ) ) ;
#20232=B_SPLINE_CURVE_WITH_KNOTS ( 'NONE', 1,
 ( #12175, #46647 ),
 .UNSPECIFIED., .F., .F.,
 ( 2, 2 ),
 ( 0.000000000000000000, 1.000000000000000000 ),
 .UNSPECIFIED. ) ;
#20234=VERTEX_POINT ( 'NONE', #1544 ) ;
#20235=B_SPLINE_CURVE_WITH_KNOTS ( 'NONE', 3,
 ( #1646, #1884, #12242, #5599, #9048, #9534, #35127, #23826, #35843, #31442 ),
 .UNSPECIFIED., .F., .F.,
 ( 4, 2, 2, 2, 4 ),
 ( 0.000000000000000000, 0.2500000000000000000, 0.5000000000000000000, 0.7500000000000000000, 1.000000000000000000 ),
 .UNSPECIFIED. ) ;
#20236=CARTESIAN_POINT ( 'NONE',  ( -13.75915741662262270, -20.84105630778929097, 72.07040738930723478 ) ) ;
#20237=EDGE_CURVE ( 'NONE', #6964, #37778, #7579, .T. ) ;
#20238=CARTESIAN_POINT ( 'NONE',  ( -23.80698203817894054, -17.68407506542587271, 62.75744385471828934 ) ) ;
#20239=B_SPLINE_CURVE_WITH_KNOTS ( 'NONE', 3,
 ( #15102, #38002, #30158, #44687, #37258, #40981, #45183, #3545, #11421, #18553 ),
 .UNSPECIFIED., .F., .F.,
 ( 4, 2, 2, 2, 4 ),
 ( 0.000000000000000000, 0.2500000000000000000, 0.5000000000000000000, 0.7500000000000000000, 1.000000000000000000 ),
 .UNSPECIFIED. ) ;
#20240=ORIENTED_EDGE ( 'NONE', *, *, #30293, .T. ) ;
#20242=CARTESIAN_POINT ( 'NONE',  ( -10.12033492330167306, -13.33947326246890341, 74.83850996365745800 ) ) ;
#20243=( BOUNDED_SURFACE ( )  B_SPLINE_SURFACE ( 3, 1, ( 
 ( #24681, #5956 ),
 ( #35014, #5729 ),
 ( #1280, #20737 ),
 ( #1530, #35501 ),
 ( #12851, #35732 ),
 ( #27640, #27874 ),
 ( #42905, #39685 ) ),
 .UNSPECIFIED., .T., .F., .F. ) 
 B_SPLINE_SURFACE_WITH_KNOTS ( ( 4, 3, 4 ),
 ( 2, 2 ),
 ( 0.000000000000000000, 0.5000000000000000000, 1.000000000000000000 ),
 ( 0.000000000000000000, 1.000000000000000000 ),
 .UNSPECIFIED. ) 
 GEOMETRIC_REPRESENTATION_ITEM ( )  RATIONAL_B_SPLINE_SURFACE ( (
 ( 1.000000000000000000, 1.000000000000000000),
 ( 0.3333333333333335369, 0.3333333333333330373),
 ( 0.3333333333333335369, 0.3333333333333330373),
 ( 1.000000000000000000, 1.000000000000000000),
 ( 0.3333333333333333703, 0.3333333333333333703),
 ( 0.3333333333333333703, 0.3333333333333333703),
 ( 1.000000000000000000, 1.000000000000000000) ) ) 
 REPRESENTATION_ITEM ( '' )  SURFACE ( )  );
#20244=ORIENTED_EDGE ( 'NONE', *, *, #3951, .T. ) ;
#20245=CARTESIAN_POINT ( 'NONE',  ( -15.86712703025682103, -7.930203392541469221, 63.55522141739008646 ) ) ;
#20247=CARTESIAN_POINT ( 'NONE',  ( -10.40888626530166405, -14.10966241957602207, 60.91821293886854249 ) ) ;
#20248=VERTEX_POINT ( 'NONE', #28390 ) ;
#20249=CARTESIAN_POINT ( 'NONE',  ( -24.25563565401629162, -17.78119069831516086, 62.57337365234224080 ) ) ;
#20251=CARTESIAN_POINT ( 'NONE',  ( -19.64535672665736143, -21.50393832739607802, 62.20323457844267523 ) ) ;
#20253=CARTESIAN_POINT ( 'NONE',  ( -16.07865109465781117, -7.939724484389961034, 63.97011030347106697 ) ) ;
#20254=FACE_OUTER_BOUND ( 'NONE', #2210, .T. ) ;
#20256=ORIENTED_EDGE ( 'NONE', *, *, #13014, .T. ) ;
#20257=CARTESIAN_POINT ( 'NONE',  ( -14.99973435974856883, -8.185210394751409879, 60.61996258296040452 ) ) ;
#20261=CARTESIAN_POINT ( 'NONE',  ( -14.05658557958971855, -19.17473784764406020, 53.88362224778187226 ) ) ;
#20262=CARTESIAN_POINT ( 'NONE',  ( -10.44916060947156566, -15.83526976542894182, 64.65771589744088033 ) ) ;
#20263=FACE_OUTER_BOUND ( 'NONE', #17933, .T. ) ;
#20264=B_SPLINE_CURVE_WITH_KNOTS ( 'NONE', 3,
 ( #45516, #34887, #30972, #8092, #4375, #45988, #12733, #23829, #27748, #46224 ),
 .UNSPECIFIED., .F., .F.,
 ( 4, 2, 2, 2, 4 ),
 ( 0.000000000000000000, 0.2500000000000000000, 0.5000000000000000000, 0.7500000000000000000, 1.000000000000000000 ),
 .UNSPECIFIED. ) ;
#20265=CARTESIAN_POINT ( 'NONE',  ( -15.93879930885702656, -7.917138641544857691, 67.15479422225767792 ) ) ;
#20267=EDGE_CURVE ( 'NONE', #13276, #22004, #27535, .T. ) ;
#20272=ORIENTED_EDGE ( 'NONE', *, *, #20396, .T. ) ;
#20273=DIRECTION ( 'NONE',  ( -5.935091885548698876E-07, -2.117535313761473712E-07, 0.9999999999998014921 ) ) ;
#20275=CARTESIAN_POINT ( 'NONE',  ( -17.93986882229626190, -22.24133833173343788, 62.07547122339882151 ) ) ;
#20277=CARTESIAN_POINT ( 'NONE',  ( -12.79501450006381269, -20.06007546732424629, 68.44543540964158979 ) ) ;
#20278=CARTESIAN_POINT ( 'NONE',  ( -23.42915847708036736, -11.11517115755410146, 73.64721174900437006 ) ) ;
#20279=ORIENTED_EDGE ( 'NONE', *, *, #27552, .T. ) ;
#20281=CARTESIAN_POINT ( 'NONE',  ( -19.90432934692537614, -21.83431937171774706, 69.04987052938618319 ) ) ;
#20282=CARTESIAN_POINT ( 'NONE',  ( -10.84385027318267447, -17.33971308591566185, 64.92739379503987607 ) ) ;
#20283=CARTESIAN_POINT ( 'NONE',  ( -18.95380389027981494, -7.978394929000565128, 63.53975171141463818 ) ) ;
#20285=CARTESIAN_POINT ( 'NONE',  ( -23.93648101794248362, -17.51022725521227841, 65.95829288617392194 ) ) ;
#20288=CARTESIAN_POINT ( 'NONE',  ( -13.77492725671111806, -20.78292389580533595, 64.98628829336273327 ) ) ;
#20290=ORIENTED_EDGE ( 'NONE', *, *, #41668, .F. ) ;
#20294=AXIS2_PLACEMENT_3D ( 'NONE', #1781, #24443, #28116 ) ;
#20297=AXIS2_PLACEMENT_3D ( 'NONE', #12960, #35849, #43754 ) ;
#20298=EDGE_CURVE ( 'NONE', #35964, #32538, #30424, .T. ) ;
#20300=CARTESIAN_POINT ( 'NONE',  ( -13.97464618706818840, -20.90036148544157157, 68.74159733221011948 ) ) ;
#20301=CARTESIAN_POINT ( 'NONE',  ( -9.979672921070292801, -14.51892525773737574, 67.90154210966345261 ) ) ;
#20303=CARTESIAN_POINT ( 'NONE',  ( -24.23636277187043220, -17.82529184948975498, 62.58865552117998021 ) ) ;
#20304=VERTEX_POINT ( 'NONE', #36144 ) ;
#20307=DIRECTION ( 'NONE',  ( 0.9710973231077277834, -0.2386838684389877285, 7.431671637556432894E-08 ) ) ;
#20308=ORIENTED_EDGE ( 'NONE', *, *, #16829, .F. ) ;
#20309=CARTESIAN_POINT ( 'NONE',  ( -10.68602809008750576, -16.88409676349039046, 57.70232650191087487 ) ) ;
#20311=ORIENTED_EDGE ( 'NONE', *, *, #18264, .F. ) ;
#20314=B_SPLINE_CURVE_WITH_KNOTS ( 'NONE', 3,
 ( #47733, #21409, #9838, #20915, #13974, #21161, #43818, #36395, #17453, #32481 ),
 .UNSPECIFIED., .F., .F.,
 ( 4, 2, 2, 2, 4 ),
 ( 0.000000000000000000, 0.2500000000000000000, 0.5000000000000000000, 0.7500000000000000000, 1.000000000000000000 ),
 .UNSPECIFIED. ) ;
#20315=CARTESIAN_POINT ( 'NONE',  ( -20.04769106148205537, -8.319399502215615527, 70.47773761195011843 ) ) ;
#20316=CARTESIAN_POINT ( 'NONE',  ( -19.34682484732250884, -8.026308974676197749, 59.96652798359869507 ) ) ;
#20317=EDGE_LOOP ( 'NONE', ( #39664, #5946, #38335, #11938 ) ) ;
#20318=FACE_OUTER_BOUND ( 'NONE', #3554, .T. ) ;
#20319=DIRECTION ( 'NONE',  ( 0.9640890753730593232, -0.2655790932026004803, 6.310348465037888425E-08 ) ) ;
#20320=CARTESIAN_POINT ( 'NONE',  ( -24.55824875695236287, -12.66269769826935310, 70.02888935069151444 ) ) ;
#20321=ADVANCED_FACE ( 'NONE', ( #2667 ), #14176, .T. ) ;
#20323=ADVANCED_FACE ( 'NONE', ( #40339 ), #43123, .T. ) ;
#20325=LINE ( 'NONE', #9007, #10865 ) ;
#20326=CARTESIAN_POINT ( 'NONE',  ( -17.43006558257920346, -7.359130651351934560, 67.27685495689534889 ) ) ;
#20329=ORIENTED_EDGE ( 'NONE', *, *, #32346, .T. ) ;
#20330=DIRECTION ( 'NONE',  ( -0.2771212459065067191, 0.9608349572466770017, 4.100231986695772107E-08 ) ) ;
#20331=( BOUNDED_SURFACE ( )  B_SPLINE_SURFACE ( 3, 1, ( 
 ( #28057, #24382 ),
 ( #8385, #43082 ),
 ( #8881, #23661 ),
 ( #38403, #32002 ),
 ( #27581, #16720 ),
 ( #38901, #35200 ),
 ( #5180, #39140 ) ),
 .UNSPECIFIED., .T., .F., .F. ) 
 B_SPLINE_SURFACE_WITH_KNOTS ( ( 4, 3, 4 ),
 ( 2, 2 ),
 ( 0.000000000000000000, 0.5000000000000000000, 1.000000000000000000 ),
 ( 0.000000000000000000, 1.000000000000000000 ),
 .UNSPECIFIED. ) 
 GEOMETRIC_REPRESENTATION_ITEM ( )  RATIONAL_B_SPLINE_SURFACE ( (
 ( 1.000000000000000000, 1.000000000000000000),
 ( 0.3333333333333335369, 0.3333333333333330373),
 ( 0.3333333333333335369, 0.3333333333333330373),
 ( 1.000000000000000000, 1.000000000000000000),
 ( 0.3333333333333333703, 0.3333333333333333703),
 ( 0.3333333333333333703, 0.3333333333333333703),
 ( 1.000000000000000000, 1.000000000000000000) ) ) 
 REPRESENTATION_ITEM ( '' )  SURFACE ( )  );
#20334=CARTESIAN_POINT ( 'NONE',  ( -24.09792875595538320, -17.08130417324981565, 72.88336032035921619 ) ) ;
#20336=CARTESIAN_POINT ( 'NONE',  ( -19.86401518824997225, -21.42384811948916834, 69.22010401872219632 ) ) ;
#20337=VECTOR ( 'NONE', #42568, 1000.000000000000000 ) ;
#20338=EDGE_CURVE ( 'NONE', #15343, #28414, #19872, .T. ) ;
#20339=CARTESIAN_POINT ( 'NONE',  ( -12.68532267716109985, -9.060482739934947460, 71.03420753023118550 ) ) ;
#20340=EDGE_LOOP ( 'NONE', ( #19802, #46215 ) ) ;
#20341=VERTEX_POINT ( 'NONE', #29012 ) ;
#20343=CARTESIAN_POINT ( 'NONE',  ( -10.03016471889695183, -15.72215649304404117, 61.08143109537672188 ) ) ;
#20344=VECTOR ( 'NONE', #13915, 999.9999999999998863 ) ;
#20346=CARTESIAN_POINT ( 'NONE',  ( -10.03035368457962662, -15.72374687363213575, 61.22284448286259817 ) ) ;
#20347=CARTESIAN_POINT ( 'NONE',  ( -13.46747890590686403, -9.034676489092227314, 60.43950277890026967 ) ) ;
#20348=VERTEX_POINT ( 'NONE', #29495 ) ;
#20352=DIRECTION ( 'NONE',  ( -0.8839923186919886877, 0.4675014229855999348, -2.842058574697934120E-08 ) ) ;
#20354=CARTESIAN_POINT ( 'NONE',  ( -23.27870965407892712, -18.64632446977878999, 66.01492505208454986 ) ) ;
#20356=B_SPLINE_CURVE_WITH_KNOTS ( 'NONE', 3,
 ( #2757, #26153, #41164, #46076, #19737, #780, #1020, #26641, #532, #53 ),
 .UNSPECIFIED., .F., .F.,
 ( 4, 2, 2, 2, 4 ),
 ( 0.6272669072783091382, 0.7522669073001884144, 0.8772669073220678015, 1.002266907343947189, 1.127266907365826354 ),
 .UNSPECIFIED. ) ;
#20357=VERTEX_POINT ( 'NONE', #44527 ) ;
#20358=B_SPLINE_CURVE_WITH_KNOTS ( 'NONE', 3,
 ( #24322, #1408, #46954, #20859, #6076, #10017, #1900, #16902, #24077, #20381 ),
 .UNSPECIFIED., .F., .F.,
 ( 4, 2, 2, 2, 4 ),
 ( 0.000000000000000000, 0.2500000000000000000, 0.5000000000000000000, 0.7500000000000000000, 1.000000000000000000 ),
 .UNSPECIFIED. ) ;
#20359=CYLINDRICAL_SURFACE ( 'NONE', #40592, 0.1500000000000060452 ) ;
#20360=CARTESIAN_POINT ( 'NONE',  ( -10.37433175079900849, -14.87184048509926271, 74.79778922563521348 ) ) ;
#20365=VECTOR ( 'NONE', #40420, 1000.000000000000227 ) ;
#20367=FACE_OUTER_BOUND ( 'NONE', #14856, .T. ) ;
#20369=FACE_OUTER_BOUND ( 'NONE', #40462, .T. ) ;
#20370=ORIENTED_EDGE ( 'NONE', *, *, #34151, .T. ) ;
#20372=DIRECTION ( 'NONE',  ( 0.6043825497304157190, -0.7966942535134532433, 5.656674838975381179E-08 ) ) ;
#20373=B_SPLINE_CURVE_WITH_KNOTS ( 'NONE', 1,
 ( #43212, #5791 ),
 .UNSPECIFIED., .F., .F.,
 ( 2, 2 ),
 ( 0.000000000000000000, 1.000000000000000000 ),
 .UNSPECIFIED. ) ;
#20374=( BOUNDED_CURVE ( )  B_SPLINE_CURVE ( 3, ( #33437, #3424, #21657, #22636 ),
 .UNSPECIFIED., .F., .F. ) 
 B_SPLINE_CURVE_WITH_KNOTS ( ( 4, 4 ),
 ( 4.712388980384689674, 4.921828490624008623 ),
 .UNSPECIFIED. ) 
 CURVE ( )  GEOMETRIC_REPRESENTATION_ITEM ( )  RATIONAL_B_SPLINE_CURVE ( ( 1.000000000000000000, 0.9963479302455156006, 0.9963479302455156006, 1.000000000000000000 ) ) 
 REPRESENTATION_ITEM ( '' )  );
#20375=CARTESIAN_POINT ( 'NONE',  ( -17.36015951656348832, -7.359395083792595216, 67.20534920880687935 ) ) ;
#20377=VERTEX_POINT ( 'NONE', #10782 ) ;
#20379=ORIENTED_EDGE ( 'NONE', *, *, #38313, .F. ) ;
#20380=CARTESIAN_POINT ( 'NONE',  ( -19.23450401370881124, -7.582471044449923703, 63.53815095794843160 ) ) ;
#20381=CARTESIAN_POINT ( 'NONE',  ( -16.39888349198502127, -21.73372412438269308, 62.05568132716130236 ) ) ;
#20382=ORIENTED_EDGE ( 'NONE', *, *, #10032, .F. ) ;
#20385=CARTESIAN_POINT ( 'NONE',  ( -10.44911129250985482, -12.18941988514178121, 57.51512593431250764 ) ) ;
#20386=CARTESIAN_POINT ( 'NONE',  ( -13.24129617563109740, -8.644154241298165786, 60.69596227262822907 ) ) ;
#20390=CARTESIAN_POINT ( 'NONE',  ( -11.73260704738458671, -10.00184175524024610, 67.61401452035728710 ) ) ;
#20391=CARTESIAN_POINT ( 'NONE',  ( -20.06975372951847447, -8.274133229585533655, 73.73568642813194174 ) ) ;
#20393=CARTESIAN_POINT ( 'NONE',  ( -10.61328331460780561, -11.78972931969595273, 74.73557151665039555 ) ) ;
#20394=( BOUNDED_CURVE ( )  B_SPLINE_CURVE ( 3, ( #22490, #18792, #26428, #7734 ),
 .UNSPECIFIED., .F., .F. ) 
 B_SPLINE_CURVE_WITH_KNOTS ( ( 4, 4 ),
 ( 0.9074455897393638448, 1.000000000000000000 ),
 .UNSPECIFIED. ) 
 CURVE ( )  GEOMETRIC_REPRESENTATION_ITEM ( )  RATIONAL_B_SPLINE_CURVE ( ( 0.6983129098260933976, 0.7760317562606985353, 0.8765941196520007361, 1.000000000000000000 ) ) 
 REPRESENTATION_ITEM ( '' )  );
#20396=EDGE_CURVE ( 'NONE', #27898, #25531, #44781, .T. ) ;
#20398=ORIENTED_EDGE ( 'NONE', *, *, #12549, .F. ) ;
#20399=ORIENTED_EDGE ( 'NONE', *, *, #1147, .F. ) ;
#20400=ADVANCED_FACE ( 'NONE', ( #45266 ), #39376, .T. ) ;
#20401=CARTESIAN_POINT ( 'NONE',  ( -24.05420634179087358, -17.20676946999824608, 69.69867738674849988 ) ) ;
#20402=CARTESIAN_POINT ( 'NONE',  ( -20.09525921507954038, -21.27957844515276875, 72.47766857650304928 ) ) ;
#20404=CARTESIAN_POINT ( 'NONE',  ( -10.42496409221358178, -14.69883174549087279, 71.32782692796889989 ) ) ;
#20406=ADVANCED_FACE ( 'NONE', ( #15425 ), #7842, .T. ) ;
#20407=CARTESIAN_POINT ( 'NONE',  ( -12.32158608955787393, -9.943909642237139579, 60.57390139315987909 ) ) ;
#20409=CARTESIAN_POINT ( 'NONE',  ( -19.53727001588333323, -22.01011538462517336, 53.63095954094023909 ) ) ;
#20410=DIRECTION ( 'NONE',  ( -0.5022914217388751990, 0.8646984027090225400, 6.766381827299041184E-08 ) ) ;
#20413=CARTESIAN_POINT ( 'NONE',  ( -13.85036685459366090, -21.34611448311455106, 72.02633460110843089 ) ) ;
#20414=EDGE_LOOP ( 'NONE', ( #16999, #13441 ) ) ;
#20415=ORIENTED_EDGE ( 'NONE', *, *, #9046, .F. ) ;
#20416=CARTESIAN_POINT ( 'NONE',  ( -12.34763169630739732, -20.26208273980121533, 68.51470172492967947 ) ) ;
#20417=ADVANCED_FACE ( 'NONE', ( #30732 ), #22862, .T. ) ;
#20419=CARTESIAN_POINT ( 'NONE',  ( -23.63040034176007609, -11.57141379323375219, 66.42214533111976493 ) ) ;
#20421=CARTESIAN_POINT ( 'NONE',  ( -22.45398830698411174, -19.67764612419960457, 72.64400540998924782 ) ) ;
#20424=CARTESIAN_POINT ( 'NONE',  ( -20.23203131230217267, -21.71059417314907591, 72.51823477531823414 ) ) ;
#20428=VERTEX_POINT ( 'NONE', #30493 ) ;
#20431=AXIS2_PLACEMENT_3D ( 'NONE', #22243, #44657, #29386 ) ;
#20433=CYLINDRICAL_SURFACE ( 'NONE', #48549, 0.1499999999999992450 ) ;
#20435=EDGE_CURVE ( 'NONE', #4639, #29387, #7103, .T. ) ;
#20436=ORIENTED_EDGE ( 'NONE', *, *, #40106, .F. ) ;
#20437=CARTESIAN_POINT ( 'NONE',  ( -20.31649657898477912, -7.943510300654241796, 70.43595776394847974 ) ) ;
#20438=AXIS2_PLACEMENT_3D ( 'NONE', #8353, #11554, #12045 ) ;
#20439=VERTEX_POINT ( 'NONE', #45508 ) ;
#20440=CARTESIAN_POINT ( 'NONE',  ( -10.01583252691979986, -14.02010874201704738, 61.05787945157973695 ) ) ;
#20443=CARTESIAN_POINT ( 'NONE',  ( -10.69179989897285310, -16.90224548161295814, 57.69320343077063740 ) ) ;
#20444=EDGE_CURVE ( 'NONE', #44245, #14220, #3636, .T. ) ;
#20447=ORIENTED_EDGE ( 'NONE', *, *, #32466, .F. ) ;
#20449=CARTESIAN_POINT ( 'NONE',  ( -14.93181132608235195, -7.787654600965993268, 57.03655263075181381 ) ) ;
#20454=CARTESIAN_POINT ( 'NONE',  ( -24.59706333651279664, -12.79617740830267891, 66.48742133194130588 ) ) ;
#20455=B_SPLINE_CURVE_WITH_KNOTS ( 'NONE', 1,
 ( #28659, #47618 ),
 .UNSPECIFIED., .F., .F.,
 ( 2, 2 ),
 ( 0.000000000000000000, 1.000000000000000000 ),
 .UNSPECIFIED. ) ;
#20456=CARTESIAN_POINT ( 'NONE',  ( -20.68576094134451182, -21.00469108578126765, 62.22544513427146740 ) ) ;
#20458=ORIENTED_EDGE ( 'NONE', *, *, #13982, .T. ) ;
#20459=ORIENTED_EDGE ( 'NONE', *, *, #47125, .F. ) ;
#20460=EDGE_CURVE ( 'NONE', #27240, #20428, #2231, .T. ) ;
#20461=CARTESIAN_POINT ( 'NONE',  ( -14.66630222544869078, -8.320656262913125545, 63.80450889863892172 ) ) ;
#20462=CARTESIAN_POINT ( 'NONE',  ( -10.08052675126636721, -16.06451543208143917, 68.09272439531302723 ) ) ;
#20463=ORIENTED_EDGE ( 'NONE', *, *, #14011, .T. ) ;
#20467=EDGE_CURVE ( 'NONE', #48485, #16276, #47507, .T. ) ;
#20468=CARTESIAN_POINT ( 'NONE',  ( -12.64995474452274316, -19.99670071527213366, 68.63657438322856308 ) ) ;
#20469=CARTESIAN_POINT ( 'NONE',  ( -11.25989433568915032, -11.38792842781904469, 64.44882039367774951 ) ) ;
#20470=FACE_OUTER_BOUND ( 'NONE', #21778, .T. ) ;
#20473=CARTESIAN_POINT ( 'NONE',  ( -16.50454646563301964, -22.20232569423288282, 65.34069100801451668 ) ) ;
#20477=FACE_OUTER_BOUND ( 'NONE', #3586, .T. ) ;
#20478=LINE ( 'NONE', #21197, #5676 ) ;
#20480=EDGE_LOOP ( 'NONE', ( #7369, #36661 ) ) ;
#20481=EDGE_LOOP ( 'NONE', ( #6663, #47030, #15268, #37150, #43777 ) ) ;
#20482=B_SPLINE_CURVE_WITH_KNOTS ( 'NONE', 3,
 ( #23580, #12952, #42289, #8809, #43004, #19881, #27023, #31438, #31684, #12240 ),
 .UNSPECIFIED., .F., .F.,
 ( 4, 2, 2, 2, 4 ),
 ( 0.000000000000000000, 0.2500000000000000000, 0.5000000000000000000, 0.7500000000000000000, 1.000000000000000000 ),
 .UNSPECIFIED. ) ;
#20483=ORIENTED_EDGE ( 'NONE', *, *, #18315, .T. ) ;
#20486=CARTESIAN_POINT ( 'NONE',  ( -13.30711168077662521, -9.147894172712071281, 64.20946529582356277 ) ) ;
#20487=VECTOR ( 'NONE', #8820, 1000.000000000000227 ) ;
#20488=ORIENTED_EDGE ( 'NONE', *, *, #829, .T. ) ;
#20489=CARTESIAN_POINT ( 'NONE',  ( -10.83189492465945669, -11.33829310736856044, 67.79677371063019109 ) ) ;
#20490=CARTESIAN_POINT ( 'NONE',  ( -10.37974201859533707, -14.52605273603761660, 68.15800121751649954 ) ) ;
#20491=VERTEX_POINT ( 'NONE', #15923 ) ;
#20492=CARTESIAN_POINT ( 'NONE',  ( -20.25191534917340874, -8.350868906188830820, 70.26572394742477456 ) ) ;
#20493=ORIENTED_EDGE ( 'NONE', *, *, #231, .T. ) ;
#20494=CARTESIAN_POINT ( 'NONE',  ( -10.78748997988023639, -12.58311375253882325, 57.51960598127043767 ) ) ;
#20495=EDGE_CURVE ( 'NONE', #45387, #11424, #20482, .T. ) ;
#20496=EDGE_LOOP ( 'NONE', ( #21483, #47932 ) ) ;
#20497=CARTESIAN_POINT ( 'NONE',  ( -22.62394951084894146, -10.04809318868971424, 70.29706442286226320 ) ) ;
#20498=ORIENTED_EDGE ( 'NONE', *, *, #43738, .F. ) ;
#20500=CARTESIAN_POINT ( 'NONE',  ( -22.47397867527990201, -20.28676549996637135, 65.86568223911946518 ) ) ;
#20503=CARTESIAN_POINT ( 'NONE',  ( -24.42531087273439994, -14.77968204897741167, 62.94126267090115334 ) ) ;
#20506=CARTESIAN_POINT ( 'NONE',  ( -16.16063032598464133, -7.467038112641824377, 60.38523865926408263 ) ) ;
#20509=ORIENTED_EDGE ( 'NONE', *, *, #45969, .T. ) ;
#20510=AXIS2_PLACEMENT_3D ( 'NONE', #40283, #13905, #21085 ) ;
#20512=CARTESIAN_POINT ( 'NONE',  ( -11.79792992861738909, -18.97409303405279957, 71.98685885147807539 ) ) ;
#20513=CARTESIAN_POINT ( 'NONE',  ( -24.86242983737997747, -14.39095285025967286, 66.36788159907001727 ) ) ;
#20514=CARTESIAN_POINT ( 'NONE',  ( -15.13462684854361306, -21.89875038763135606, 68.68318760819161639 ) ) ;
#20517=ORIENTED_EDGE ( 'NONE', *, *, #46598, .T. ) ;
#20518=ADVANCED_FACE ( 'NONE', ( #24307 ), #27978, .F. ) ;
#20519=CARTESIAN_POINT ( 'NONE',  ( -22.75923480142028055, -10.27751027444597653, 66.84182257657300852 ) ) ;
#20520=CARTESIAN_POINT ( 'NONE',  ( -10.86718109655241626, -12.20887211208692413, 57.62857328228790976 ) ) ;
#20522=CARTESIAN_POINT ( 'NONE',  ( -11.45045256087476027, -18.56827314959498310, 68.36122809857093330 ) ) ;
#20523=FACE_OUTER_BOUND ( 'NONE', #32004, .T. ) ;
#20525=CARTESIAN_POINT ( 'NONE',  ( -22.75539019595755263, -10.19575032747719590, 66.82710158566565894 ) ) ;
#20526=ADVANCED_FACE ( 'NONE', ( #12480 ), #1882, .T. ) ;
#20527=CARTESIAN_POINT ( 'NONE',  ( -15.44746548810605447, -21.57648140951198812, 72.04575476862331129 ) ) ;
#20528=( BOUNDED_CURVE ( )  B_SPLINE_CURVE ( 3, ( #40863, #29539, #18441, #33449 ),
 .UNSPECIFIED., .F., .F. ) 
 B_SPLINE_CURVE_WITH_KNOTS ( ( 4, 4 ),
 ( 0.4074455897393652326, 0.5000000000000000000 ),
 .UNSPECIFIED. ) 
 CURVE ( )  GEOMETRIC_REPRESENTATION_ITEM ( )  RATIONAL_B_SPLINE_CURVE ( ( 0.6983129098260896228, 0.7760317562606828812, 0.8765941196519826395, 0.9999999999999802380 ) ) 
 REPRESENTATION_ITEM ( '' )  );
#20529=ORIENTED_EDGE ( 'NONE', *, *, #47125, .T. ) ;
#20530=CARTESIAN_POINT ( 'NONE',  ( -12.09359296509799719, -9.604326949652671530, 57.24968926044763862 ) ) ;
#20531=PLANE ( 'NONE',  #39864 ) ;
#20532=EDGE_CURVE ( 'NONE', #31415, #19901, #24586, .T. ) ;
#20535=VECTOR ( 'NONE', #23227, 1000.000000000000000 ) ;
#20537=ADVANCED_FACE ( 'NONE', ( #38826 ), #8316, .T. ) ;
#20538=CARTESIAN_POINT ( 'NONE',  ( -24.41897151118743636, -17.37347349776957017, 69.59835227440868266 ) ) ;
#20541=CARTESIAN_POINT ( 'NONE',  ( -24.11794058161805054, -12.76166764465371628, 69.77243002474142486 ) ) ;
#20542=( BOUNDED_CURVE ( )  B_SPLINE_CURVE ( 3, ( #12341, #27361, #34250, #19006 ),
 .UNSPECIFIED., .F., .F. ) 
 B_SPLINE_CURVE_WITH_KNOTS ( ( 4, 4 ),
 ( 0.000000000000000000, 0.4074455897393681747 ),
 .UNSPECIFIED. ) 
 CURVE ( )  GEOMETRIC_REPRESENTATION_ITEM ( )  RATIONAL_B_SPLINE_CURVE ( ( 1.000000000000000000, 0.4567392136813264170, 0.3561768502900282130, 0.6983129098261053880 ) ) 
 REPRESENTATION_ITEM ( '' )  );
#20543=ORIENTED_EDGE ( 'NONE', *, *, #43986, .F. ) ;
#20547=CARTESIAN_POINT ( 'NONE',  ( -13.27359419718654365, -9.172268535653204324, 64.20946477989005530 ) ) ;
#20549=FACE_OUTER_BOUND ( 'NONE', #795, .T. ) ;
#20550=ADVANCED_FACE ( 'NONE', ( #35368 ), #12727, .T. ) ;
#20551=CARTESIAN_POINT ( 'NONE',  ( -12.01932494161596487, -10.27783711031607261, 71.38381879606350822 ) ) ;
#20553=EDGE_CURVE ( 'NONE', #1779, #12574, #38077, .T. ) ;
#20554=CARTESIAN_POINT ( 'NONE',  ( -23.00381842360518547, -10.58230771189866104, 59.90203429537245228 ) ) ;
#20556=CARTESIAN_POINT ( 'NONE',  ( -11.75774202113761113, -19.00384077433692909, 71.83685884782747166 ) ) ;
#20558=CARTESIAN_POINT ( 'NONE',  ( -19.94917705995926482, -8.226604131702123013, 74.00624557436877637 ) ) ;
#20559=EDGE_CURVE ( 'NONE', #44086, #8618, #22216, .T. ) ;
#20561=CARTESIAN_POINT ( 'NONE',  ( -18.12432747636454877, -22.22630431188652977, 65.60178084401016463 ) ) ;
#20562=ORIENTED_EDGE ( 'NONE', *, *, #34654, .F. ) ;
#20563=CARTESIAN_POINT ( 'NONE',  ( -23.83080496556880945, -17.75212211224490133, 59.28906343887996400 ) ) ;
#20564=CARTESIAN_POINT ( 'NONE',  ( -11.93522140360746064, -14.45952210441258501, 53.49999999999995026 ) ) ;
#20567=CARTESIAN_POINT ( 'NONE',  ( -12.17848458102417908, -19.44617700360637613, 58.15512196582962900 ) ) ;
#20571=CARTESIAN_POINT ( 'NONE',  ( -24.40987808923448554, -15.75888385863607333, 69.83307461037107089 ) ) ;
#20573=VERTEX_POINT ( 'NONE', #925 ) ;
#20574=CARTESIAN_POINT ( 'NONE',  ( -10.33431758219403207, -12.52035302217920254, 60.98348881056122650 ) ) ;
#20576=CARTESIAN_POINT ( 'NONE',  ( -23.10841418202883446, -18.98556259803724799, 65.91569706707790033 ) ) ;
#20577=CARTESIAN_POINT ( 'NONE',  ( -12.01648241349452917, -10.28590705807702932, 67.49896869922172016 ) ) ;
#20579=CARTESIAN_POINT ( 'NONE',  ( -18.25635609959491035, -22.28132141893295071, 53.76227901944321275 ) ) ;
#20582=ORIENTED_EDGE ( 'NONE', *, *, #39631, .T. ) ;
#20585=EDGE_LOOP ( 'NONE', ( #14912, #5978, #26841, #44416, #35266 ) ) ;
#20586=CARTESIAN_POINT ( 'NONE',  ( -19.83852420082105894, -21.85790785478787868, 69.12137763959520953 ) ) ;
#20588=ORIENTED_EDGE ( 'NONE', *, *, #4173, .F. ) ;
#20589=ORIENTED_EDGE ( 'NONE', *, *, #26318, .T. ) ;
#20590=VERTEX_POINT ( 'NONE', #1153 ) ;
#20595=CARTESIAN_POINT ( 'NONE',  ( -13.43330777456016989, -9.058089930353723673, 60.43950223964813517 ) ) ;
#20596=VERTEX_POINT ( 'NONE', #25496 ) ;
#20600=CARTESIAN_POINT ( 'NONE',  ( -21.53861886228549949, -21.02004079589906027, 72.63951149839988375 ) ) ;
#20601=CARTESIAN_POINT ( 'NONE',  ( -24.87377577156081898, -14.89435671199219335, 59.38266843862005828 ) ) ;
#20602=CARTESIAN_POINT ( 'NONE',  ( -12.63240329231120995, -19.98054781565096505, 68.33657436980826105 ) ) ;
#20604=EDGE_CURVE ( 'NONE', #16043, #7957, #46939, .T. ) ;
#20606=ADVANCED_FACE ( 'NONE', ( #47910 ), #6306, .T. ) ;
#20607=EDGE_CURVE ( 'NONE', #4739, #6094, #9531, .T. ) ;
#20608=CARTESIAN_POINT ( 'NONE',  ( -12.32158608955787393, -9.943909642237139579, 60.57390139315987909 ) ) ;
#20609=EDGE_CURVE ( 'NONE', #6656, #29328, #43504, .T. ) ;
#20612=CARTESIAN_POINT ( 'NONE',  ( -11.45099342332292025, -10.35672743380498062, 74.58885046824201481 ) ) ;
#20613=ORIENTED_EDGE ( 'NONE', *, *, #5904, .T. ) ;
#20614=DIRECTION ( 'NONE',  ( -7.484513356303811700E-07, 7.898531944235430371E-07, 0.9999999999994079181 ) ) ;
#20615=DIRECTION ( 'NONE',  ( 0.5820088206811424580, -0.8131824719270214219, 7.019974882119937445E-08 ) ) ;
#20616=CARTESIAN_POINT ( 'NONE',  ( -11.29385091374517458, -19.04286921470785288, 68.33194352083310719 ) ) ;
#20617=CARTESIAN_POINT ( 'NONE',  ( -22.53655392111809164, -20.22829597721307948, 65.88917050827579658 ) ) ;
#20619=B_SPLINE_CURVE_WITH_KNOTS ( 'NONE', 3,
 ( #48687, #26285, #40330, #10304, #21623, #48199, #32922, #14196, #40560, #14428 ),
 .UNSPECIFIED., .F., .F.,
 ( 4, 2, 2, 2, 4 ),
 ( 0.6272669072877824492, 0.7522669073072968393, 0.8772669073268113404, 1.002266907346325731, 1.127266907365840121 ),
 .UNSPECIFIED. ) ;
#20620=DIRECTION ( 'NONE',  ( -0.3824554607245533866, 0.9239739285077093189, -8.917814418161381897E-09 ) ) ;
#20621=CARTESIAN_POINT ( 'NONE',  ( -22.78930279417433624, -10.31314903132836136, 63.18071954302660487 ) ) ;
#20624=CARTESIAN_POINT ( 'NONE',  ( -16.03410428664897225, -7.489899486381565552, 63.84823818164760212 ) ) ;
#20625=ORIENTED_EDGE ( 'NONE', *, *, #44212, .T. ) ;
#20627=CARTESIAN_POINT ( 'NONE',  ( -9.983021216844335299, -14.44210324501309906, 68.03612869841425947 ) ) ;
#20628=ORIENTED_EDGE ( 'NONE', *, *, #41243, .T. ) ;
#20629=CARTESIAN_POINT ( 'NONE',  ( -22.16544622181183044, -20.55585424591192378, 58.88726014294076094 ) ) ;
#20632=CARTESIAN_POINT ( 'NONE',  ( -23.98984720795339243, -17.39877237835929691, 73.02768823732557735 ) ) ;
#20633=FACE_OUTER_BOUND ( 'NONE', #27579, .T. ) ;
#20635=CARTESIAN_POINT ( 'NONE',  ( -13.43773910423563400, -20.62433115109003268, 58.33177939114180788 ) ) ;
#20636=CARTESIAN_POINT ( 'NONE',  ( -20.59780817978206002, -8.569521609192868539, 63.59504950924878131 ) ) ;
#20637=CARTESIAN_POINT ( 'NONE',  ( -15.35027142736847239, -7.653576728715946409, 74.26480947788739684 ) ) ;
#20639=CARTESIAN_POINT ( 'NONE',  ( -17.62313272718237300, -7.758403197964874209, 67.11219550178550719 ) ) ;
#20642=ORIENTED_EDGE ( 'NONE', *, *, #33045, .F. ) ;
#20643=CARTESIAN_POINT ( 'NONE',  ( -24.12000719736520438, -11.54295319193055214, 63.20864192093194589 ) ) ;
#20644=CARTESIAN_POINT ( 'NONE',  ( -13.33011785382929126, -9.069340661520646663, 63.92418669539090814 ) ) ;
#20646=DIRECTION ( 'NONE',  ( -0.3688590060343663324, 0.9294853595766526810, -1.901466464867638737E-17 ) ) ;
#20648=DIRECTION ( 'NONE',  ( -0.2771212459065067191, 0.9608349572466771127, 4.100231986695772107E-08 ) ) ;
#20649=CARTESIAN_POINT ( 'NONE',  ( -7.057530559158139205, -11.90597956881549102, 54.61912878955446615 ) ) ;
#20650=DIRECTION ( 'NONE',  ( 0.7700094066334552956, 0.6380325334150243055, -6.510647142068464459E-17 ) ) ;
#20651=CARTESIAN_POINT ( 'NONE',  ( -17.77594298899184366, -7.367433885636743618, 60.26556189360973548 ) ) ;
#20652=ORIENTED_EDGE ( 'NONE', *, *, #28829, .T. ) ;
#20654=CARTESIAN_POINT ( 'NONE',  ( -23.77487038158592014, -11.74745262826995429, 62.96690348473899235 ) ) ;
#20656=DIRECTION ( 'NONE',  ( 3.549360974554993999E-17, -6.371834667797928663E-18, -1.000000000000000000 ) ) ;
#20657=CARTESIAN_POINT ( 'NONE',  ( -19.77435985551070274, -21.87886194922281646, 65.64981515446680760 ) ) ;
#20658=CARTESIAN_POINT ( 'NONE',  ( -13.41559392277415341, -8.529421005230245711, 57.08472474434080368 ) ) ;
#20659=DIRECTION ( 'NONE',  ( -2.210955089557150869E-06, 1.097707070272558804E-06, -0.9999999999969533260 ) ) ;
#20660=VERTEX_POINT ( 'NONE', #13183 ) ;
#20661=ADVANCED_FACE ( 'NONE', ( #5831 ), #5741, .T. ) ;
#20662=EDGE_CURVE ( 'NONE', #45579, #13357, #39235, .T. ) ;
#20663=CARTESIAN_POINT ( 'NONE',  ( -20.30052658356369477, -21.25444530744949390, 72.56046004230084634 ) ) ;
#20664=CARTESIAN_POINT ( 'NONE',  ( -23.98641038275339099, -11.28202459292402082, 66.58247877162926898 ) ) ;
#20665=CARTESIAN_POINT ( 'NONE',  ( -13.18904211892903078, -11.30002761096173813, 53.49999999999995026 ) ) ;
#20666=CARTESIAN_POINT ( 'NONE',  ( -11.10470791607724550, -18.75498134223953883, 61.46206221440264983 ) ) ;
#20667=( BOUNDED_CURVE ( )  B_SPLINE_CURVE ( 3, ( #26681, #42184, #8444, #23478 ),
 .UNSPECIFIED., .F., .F. ) 
 B_SPLINE_CURVE_WITH_KNOTS ( ( 4, 4 ),
 ( 0.5000000000000000000, 0.9074455897393587378 ),
 .UNSPECIFIED. ) 
 CURVE ( )  GEOMETRIC_REPRESENTATION_ITEM ( )  RATIONAL_B_SPLINE_CURVE ( ( 1.000000000000012657, 0.4567392136813444581, 0.3561768502900259925, 0.6983129098260709711 ) ) 
 REPRESENTATION_ITEM ( '' )  );
#20668=VERTEX_POINT ( 'NONE', #9773 ) ;
#20669=CARTESIAN_POINT ( 'NONE',  ( -12.18719842096713357, -10.08886484896570934, 64.04386393395434141 ) ) ;
#20670=EDGE_CURVE ( 'NONE', #19987, #6217, #31184, .T. ) ;
#20671=EDGE_CURVE ( 'NONE', #31941, #35848, #32415, .T. ) ;
#20673=CARTESIAN_POINT ( 'NONE',  ( -18.12574864353739201, -7.786197982121914052, 60.22493603095571046 ) ) ;
#20674=ADVANCED_FACE ( 'NONE', ( #18089 ), #44236, .T. ) ;
#20675=CARTESIAN_POINT ( 'NONE',  ( -10.13783977983156248, -13.25541127610578762, 74.79322348855123437 ) ) ;
#20676=CARTESIAN_POINT ( 'NONE',  ( -16.77879762802476904, -7.785173775872046953, 74.16838186400050859 ) ) ;
#20677=CARTESIAN_POINT ( 'NONE',  ( -18.90996118681096405, -7.968724231816139536, 67.20071784163268092 ) ) ;
#20678=ORIENTED_EDGE ( 'NONE', *, *, #9747, .T. ) ;
#20679=CARTESIAN_POINT ( 'NONE',  ( -23.66599411597432834, -18.87638235353465177, 69.48710309960380016 ) ) ;
#20680=( BOUNDED_SURFACE ( )  B_SPLINE_SURFACE ( 3, 1, ( 
 ( #27068, #42093 ),
 ( #27794, #9590 ),
 ( #42823, #13489 ),
 ( #31739, #46992 ),
 ( #5882, #32227 ),
 ( #36139, #17175 ),
 ( #24606, #2173 ) ),
 .UNSPECIFIED., .T., .F., .F. ) 
 B_SPLINE_SURFACE_WITH_KNOTS ( ( 4, 3, 4 ),
 ( 2, 2 ),
 ( 0.000000000000000000, 0.5000000000000000000, 1.000000000000000000 ),
 ( 0.000000000000000000, 1.000000000000000000 ),
 .UNSPECIFIED. ) 
 GEOMETRIC_REPRESENTATION_ITEM ( )  RATIONAL_B_SPLINE_SURFACE ( (
 ( 1.000000000000000000, 1.000000000000000000),
 ( 0.3333333333333335369, 0.3333333333333330373),
 ( 0.3333333333333335369, 0.3333333333333330373),
 ( 1.000000000000000000, 1.000000000000000000),
 ( 0.3333333333333333703, 0.3333333333333333703),
 ( 0.3333333333333333703, 0.3333333333333333703),
 ( 1.000000000000000000, 1.000000000000000000) ) ) 
 REPRESENTATION_ITEM ( '' )  SURFACE ( )  );
#20681=ORIENTED_EDGE ( 'NONE', *, *, #46908, .T. ) ;
#20682=CARTESIAN_POINT ( 'NONE',  ( -11.33476867595667770, -19.10151316506851416, 68.40185013497388411 ) ) ;
#20683=CARTESIAN_POINT ( 'NONE',  ( -10.42496409221358178, -14.69883174549087279, 71.32782692796889989 ) ) ;
#20685=DIRECTION ( 'NONE',  ( -0.9999247414263406908, 0.01226831216845469807, 5.367905339378914507E-08 ) ) ;
#20686=EDGE_CURVE ( 'NONE', #47586, #4886, #32746, .T. ) ;
#20687=CARTESIAN_POINT ( 'NONE',  ( -11.42544933137708263, -10.39099551632332563, 74.56072225344634319 ) ) ;
#20688=ORIENTED_EDGE ( 'NONE', *, *, #38500, .T. ) ;
#20689=CARTESIAN_POINT ( 'NONE',  ( -13.56815751001608916, -20.71130982922042207, 61.81646292535575071 ) ) ;
#20690=CARTESIAN_POINT ( 'NONE',  ( -10.61641583932764910, -11.78277314028518319, 74.74335662173743344 ) ) ;
#20691=CARTESIAN_POINT ( 'NONE',  ( -16.05981277502693416, -21.73406819447767901, 61.90001277639490951 ) ) ;
#20692=ORIENTED_EDGE ( 'NONE', *, *, #35709, .F. ) ;
#20693=CARTESIAN_POINT ( 'NONE',  ( -23.83833616213321704, -17.61232902345998141, 62.77360984984811410 ) ) ;
#20694=CARTESIAN_POINT ( 'NONE',  ( -10.49912617938483628, -17.55847672437320028, 64.74084113084838066 ) ) ;
#20695=CARTESIAN_POINT ( 'NONE',  ( -20.57278697373333998, -8.057206101692887756, 66.89608655064280640 ) ) ;
#20696=CARTESIAN_POINT ( 'NONE',  ( -23.34092642400682038, -10.28208056094584677, 59.78698708435513254 ) ) ;
#20698=VERTEX_POINT ( 'NONE', #11697 ) ;
#20699=ORIENTED_EDGE ( 'NONE', *, *, #37931, .F. ) ;
#20701=CARTESIAN_POINT ( 'NONE',  ( -14.80056147340629380, -21.78207226143426922, 61.82095877133116346 ) ) ;
#20703=CARTESIAN_POINT ( 'NONE',  ( -19.33968306427223638, -21.54245604374635548, 62.27887115452926992 ) ) ;
#20705=CARTESIAN_POINT ( 'NONE',  ( -13.18474066807476675, -20.93551553819402855, 58.23145462665691241 ) ) ;
#20707=EDGE_LOOP ( 'NONE', ( #23380, #17786, #34884, #26896, #44671 ) ) ;
#20708=CARTESIAN_POINT ( 'NONE',  ( -22.61838138049972358, -19.58773617554900071, 69.32985287095068827 ) ) ;
#20710=CARTESIAN_POINT ( 'NONE',  ( -23.16908677366360436, -10.06487111558154801, 63.18530634343710517 ) ) ;
#20711=CARTESIAN_POINT ( 'NONE',  ( -24.87450840884172365, -14.73858704721042123, 59.35644987740099765 ) ) ;
#20715=EDGE_LOOP ( 'NONE', ( #866, #30290 ) ) ;
#20716=EDGE_CURVE ( 'NONE', #43113, #26442, #2767, .T. ) ;
#20717=CARTESIAN_POINT ( 'NONE',  ( -17.63866143434000833, -7.362211242860705163, 63.66561706598076853 ) ) ;
#20718=CARTESIAN_POINT ( 'NONE',  ( -23.63337334774834275, -11.57735749097352773, 63.14321518547134815 ) ) ;
#20719=CARTESIAN_POINT ( 'NONE',  ( -10.97170681910752421, -18.53336975224134520, 57.90740351038629541 ) ) ;
#20720=EDGE_LOOP ( 'NONE', ( #24715, #29909, #6642, #48730, #31383 ) ) ;
#20721=CARTESIAN_POINT ( 'NONE',  ( -12.40380833417894912, -19.68739609921301792, 61.39678633575574906 ) ) ;
#20723=DIRECTION ( 'NONE',  ( 0.9950649908465212246, 0.09922531930717197468, -4.894557009475175470E-08 ) ) ;
#20724=VECTOR ( 'NONE', #25877, 1000.000000000000114 ) ;
#20725=VERTEX_POINT ( 'NONE', #3830 ) ;
#20727=FACE_OUTER_BOUND ( 'NONE', #19698, .T. ) ;
#20730=ORIENTED_EDGE ( 'NONE', *, *, #18036, .F. ) ;
#20731=CARTESIAN_POINT ( 'NONE',  ( -11.73260704738458671, -10.00184175524024610, 67.61401452035728710 ) ) ;
#20732=ORIENTED_EDGE ( 'NONE', *, *, #43106, .F. ) ;
#20733=CARTESIAN_POINT ( 'NONE',  ( -10.54994933093899867, -13.24305344519376781, 71.49356453765415154 ) ) ;
#20735=CARTESIAN_POINT ( 'NONE',  ( -24.87417209744295477, -14.81009202510037959, 59.28654333241698993 ) ) ;
#20737=CARTESIAN_POINT ( 'NONE',  ( -19.37462041217285957, -21.99941596162432589, 58.56861435762115775 ) ) ;
#20739=CARTESIAN_POINT ( 'NONE',  ( -24.70006301780203017, -16.41064289384416242, 59.24519641474478959 ) ) ;
#20740=FACE_OUTER_BOUND ( 'NONE', #39778, .T. ) ;
#20741=CARTESIAN_POINT ( 'NONE',  ( -11.16720114480400383, -11.56054632708127450, 67.61864607954859707 ) ) ;
#20742=CARTESIAN_POINT ( 'NONE',  ( -23.56138462120852495, -11.33988936615837950, 70.04210750373424332 ) ) ;
#20743=DIRECTION ( 'NONE',  ( -0.3478314405900309603, -0.9375570856950864451, 9.567072274253697654E-17 ) ) ;
#20745=DIRECTION ( 'NONE',  ( 1.653275065793327654E-06, -1.135554159585744654E-05, -0.9999999999341592227 ) ) ;
#20746=CARTESIAN_POINT ( 'NONE',  ( -24.09792889798371007, -17.08130376423426000, 73.18336032035891492 ) ) ;
#20747=CARTESIAN_POINT ( 'NONE',  ( -12.18836193727821460, -19.53083876418623532, 57.94154444592973618 ) ) ;
#20754=ORIENTED_EDGE ( 'NONE', *, *, #9221, .F. ) ;
#20755=CYLINDRICAL_SURFACE ( 'NONE', #44979, 0.1499999999999962474 ) ;
#20756=CARTESIAN_POINT ( 'NONE',  ( -13.29845767883066543, -21.01266560759323809, 61.63150935275904629 ) ) ;
#20757=CARTESIAN_POINT ( 'NONE',  ( -12.68532353738824803, -9.060482037740600347, 71.03420644255490402 ) ) ;
#20759=CARTESIAN_POINT ( 'NONE',  ( -10.44911129250985482, -12.18941988514178121, 57.51512593431250764 ) ) ;
#20761=CARTESIAN_POINT ( 'NONE',  ( -24.80964181269326829, -15.78832295113944895, 69.67160939887251914 ) ) ;
#20764=CARTESIAN_POINT ( 'NONE',  ( -23.23616516995063819, -18.79948553760870666, 65.97389430042666447 ) ) ;
#20765=EDGE_LOOP ( 'NONE', ( #24627, #12456, #42147, #46351, #5951 ) ) ;
#20767=CARTESIAN_POINT ( 'NONE',  ( -16.23116076413911557, -7.455249184188991407, 60.31533086125586607 ) ) ;
#20768=CARTESIAN_POINT ( 'NONE',  ( -18.57335281209669731, -21.76520412651811043, 72.57038810541313012 ) ) ;
#20769=CARTESIAN_POINT ( 'NONE',  ( -24.40290088483126851, -17.41666877191872587, 69.61350989034804115 ) ) ;
#20770=CARTESIAN_POINT ( 'NONE',  ( -21.15336808330806662, -20.73310000539657949, 69.35450185099439580 ) ) ;
#20771=B_SPLINE_CURVE_WITH_KNOTS ( 'NONE', 1,
 ( #3744, #45130 ),
 .UNSPECIFIED., .F., .F.,
 ( 2, 2 ),
 ( 0.000000000000000000, 1.000000000000000000 ),
 .UNSPECIFIED. ) ;
#20773=CARTESIAN_POINT ( 'NONE',  ( -11.16823349194678627, -11.55205338407005122, 71.50349565124497531 ) ) ;
#20775=ORIENTED_EDGE ( 'NONE', *, *, #34557, .T. ) ;
#20776=EDGE_LOOP ( 'NONE', ( #40260, #12251, #41633, #43540, #20290 ) ) ;
#20778=CARTESIAN_POINT ( 'NONE',  ( -10.37518579106875194, -14.94145004404884602, 75.09219096253774239 ) ) ;
#20779=CARTESIAN_POINT ( 'NONE',  ( -17.79084007069931417, -7.768752218527304798, 60.38060768310334936 ) ) ;
#20782=VERTEX_POINT ( 'NONE', #33341 ) ;
#20785=CARTESIAN_POINT ( 'NONE',  ( -18.05440415122280484, -21.83127237841607027, 65.36004252941745563 ) ) ;
#20786=EDGE_CURVE ( 'NONE', #16929, #39540, #42778, .T. ) ;
#20787=ORIENTED_EDGE ( 'NONE', *, *, #17680, .F. ) ;
#20788=CYLINDRICAL_SURFACE ( 'NONE', #15490, 0.1500000000000041578 ) ;
#20789=CARTESIAN_POINT ( 'NONE',  ( -17.00708550189658652, -7.821638742870105965, 73.96018273346899718 ) ) ;
#20791=EDGE_LOOP ( 'NONE', ( #25080, #18488, #24302, #5570, #23092 ) ) ;
#20792=EDGE_CURVE ( 'NONE', #15544, #22481, #23006, .T. ) ;
#20794=CARTESIAN_POINT ( 'NONE',  ( -18.50162525266306091, -21.72577549820248421, 72.58510940979837756 ) ) ;
#20795=EDGE_LOOP ( 'NONE', ( #46018, #21923 ) ) ;
#20796=CARTESIAN_POINT ( 'NONE',  ( -10.52215041504658188, -13.37196039468857833, 74.97817647370040106 ) ) ;
#20799=EDGE_CURVE ( 'NONE', #4399, #34284, #36197, .T. ) ;
#20800=( BOUNDED_CURVE ( )  B_SPLINE_CURVE ( 3, ( #34195, #12051, #48733, #37391 ),
 .UNSPECIFIED., .F., .F. ) 
 B_SPLINE_CURVE_WITH_KNOTS ( ( 4, 4 ),
 ( 0.9074455897393668424, 1.000000000000000000 ),
 .UNSPECIFIED. ) 
 CURVE ( )  GEOMETRIC_REPRESENTATION_ITEM ( )  RATIONAL_B_SPLINE_CURVE ( ( 0.6983129098260865142, 0.7760317562606925401, 0.8765941196519970724, 1.000000000000000000 ) ) 
 REPRESENTATION_ITEM ( '' )  );
#20802=CARTESIAN_POINT ( 'NONE',  ( -11.06300712566464561, -17.73109164226346479, 71.58220677401085652 ) ) ;
#20806=ADVANCED_FACE ( 'NONE', ( #3569 ), #15781, .T. ) ;
#20808=FACE_OUTER_BOUND ( 'NONE', #5019, .T. ) ;
#20809=CARTESIAN_POINT ( 'NONE',  ( -20.25445156252866497, -7.916983464207429932, 73.90751836168473687 ) ) ;
#20810=CARTESIAN_POINT ( 'NONE',  ( -11.40127056704611519, -11.24191079892443135, 60.67885781060143557 ) ) ;
#20811=FACE_OUTER_BOUND ( 'NONE', #5634, .T. ) ;
#20812=ORIENTED_EDGE ( 'NONE', *, *, #40893, .F. ) ;
#20813=CARTESIAN_POINT ( 'NONE',  ( -24.35031885046671007, -17.55372768567562858, 66.08210759853170657 ) ) ;
#20816=ORIENTED_EDGE ( 'NONE', *, *, #24191, .F. ) ;
#20817=B_SPLINE_CURVE_WITH_KNOTS ( 'NONE', 3,
 ( #37853, #19386, #19142, #922, #41303, #41807, #11277, #11765, #45981, #27019 ),
 .UNSPECIFIED., .F., .F.,
 ( 4, 2, 2, 2, 4 ),
 ( 0.000000000000000000, 0.2500000000000000000, 0.5000000000000000000, 0.7500000000000000000, 1.000000000000000000 ),
 .UNSPECIFIED. ) ;
#20818=( BOUNDED_SURFACE ( )  B_SPLINE_SURFACE ( 3, 1, ( 
 ( #47457, #2628 ),
 ( #37073, #44257 ),
 ( #3355, #18361 ),
 ( #13925, #28971 ),
 ( #44020, #25290 ),
 ( #40305, #10513 ),
 ( #6810, #21827 ) ),
 .UNSPECIFIED., .T., .F., .F. ) 
 B_SPLINE_SURFACE_WITH_KNOTS ( ( 4, 3, 4 ),
 ( 2, 2 ),
 ( 0.000000000000000000, 0.5000000000000000000, 1.000000000000000000 ),
 ( 0.000000000000000000, 1.000000000000000000 ),
 .UNSPECIFIED. ) 
 GEOMETRIC_REPRESENTATION_ITEM ( )  RATIONAL_B_SPLINE_SURFACE ( (
 ( 1.000000000000000000, 1.000000000000000000),
 ( 0.3333333333333335369, 0.3333333333333330373),
 ( 0.3333333333333335369, 0.3333333333333330373),
 ( 1.000000000000000000, 1.000000000000000000),
 ( 0.3333333333333333703, 0.3333333333333333703),
 ( 0.3333333333333333703, 0.3333333333333333703),
 ( 1.000000000000000000, 1.000000000000000000) ) ) 
 REPRESENTATION_ITEM ( '' )  SURFACE ( )  );
#20820=ORIENTED_EDGE ( 'NONE', *, *, #20792, .F. ) ;
#20821=ORIENTED_EDGE ( 'NONE', *, *, #20947, .T. ) ;
#20822=ORIENTED_EDGE ( 'NONE', *, *, #41461, .T. ) ;
#20823=DIRECTION ( 'NONE',  ( 0.8447509909909772796, -0.5351595679979587183, 5.460905094113815840E-17 ) ) ;
#20824=DIRECTION ( 'NONE',  ( 7.404863042181874502E-06, -6.320720312887485007E-06, 0.9999999999526082428 ) ) ;
#20825=ADVANCED_FACE ( 'NONE', ( #35307 ), #31471, .T. ) ;
#20827=CARTESIAN_POINT ( 'NONE',  ( -19.84060376186859287, -21.38033729433684726, 72.48922594225743410 ) ) ;
#20828=CARTESIAN_POINT ( 'NONE',  ( -16.28340391395008169, -22.17153211024223936, 61.89534802377870193 ) ) ;
#20829=( BOUNDED_CURVE ( )  B_SPLINE_CURVE ( 3, ( #46600, #38948, #27632, #30860 ),
 .UNSPECIFIED., .F., .F. ) 
 B_SPLINE_CURVE_WITH_KNOTS ( ( 4, 4 ),
 ( 0.9074455897393733927, 1.000000000000000000 ),
 .UNSPECIFIED. ) 
 CURVE ( )  GEOMETRIC_REPRESENTATION_ITEM ( )  RATIONAL_B_SPLINE_CURVE ( ( 0.6983129098261244838, 0.7760317562607252917, 0.8765941196520171674, 1.000000000000000000 ) ) 
 REPRESENTATION_ITEM ( '' )  );
#20830=VERTEX_POINT ( 'NONE', #19322 ) ;
#20831=ORIENTED_EDGE ( 'NONE', *, *, #23521, .T. ) ;
#20835=CARTESIAN_POINT ( 'NONE',  ( -24.87396285843436772, -14.85457912869396324, 59.44311433200221018 ) ) ;
#20836=CARTESIAN_POINT ( 'NONE',  ( -24.09304468200822669, -16.93663518450954086, 73.11009419552426891 ) ) ;
#20838=ADVANCED_FACE ( 'NONE', ( #1582 ), #46410, .F. ) ;
#20840=CARTESIAN_POINT ( 'NONE',  ( -18.92057629138644970, -7.919864069981281673, 67.05071783789199458 ) ) ;
#20841=CARTESIAN_POINT ( 'NONE',  ( -9.974215857974789046, -14.86484893678357544, 74.91283499353951925 ) ) ;
#20842=CARTESIAN_POINT ( 'NONE',  ( -24.87424609913982110, -14.79435799483268177, 59.38153755231025599 ) ) ;
#20844=CARTESIAN_POINT ( 'NONE',  ( -11.75774095458083046, -19.00383931511212765, 71.68685884783835149 ) ) ;
#20845=EDGE_CURVE ( 'NONE', #6404, #23831, #28011, .T. ) ;
#20850=CARTESIAN_POINT ( 'NONE',  ( -19.37484727228654080, -7.619050864103940057, 60.14588289477547534 ) ) ;
#20851=EDGE_CURVE ( 'NONE', #47684, #25517, #19530, .T. ) ;
#20852=CARTESIAN_POINT ( 'NONE',  ( -11.75743953354532856, -10.61491319464748351, 74.73885004197741466 ) ) ;
#20853=CARTESIAN_POINT ( 'NONE',  ( -17.96469515596628597, -21.78991216099736405, 65.45605247325242715 ) ) ;
#20855=CARTESIAN_POINT ( 'NONE',  ( -22.09234551867295693, -20.09219114410425178, 62.53439162497838311 ) ) ;
#20856=EDGE_LOOP ( 'NONE', ( #45256, #21912, #33586, #6013, #15506 ) ) ;
#20857=VECTOR ( 'NONE', #9513, 1000.000000000000227 ) ;
#20858=CARTESIAN_POINT ( 'NONE',  ( -11.81178328723415660, -10.62567094834893311, 74.73885052262691886 ) ) ;
#20859=CARTESIAN_POINT ( 'NONE',  ( -16.26648990220133228, -21.71412262074107247, 61.82738493259662249 ) ) ;
#20861=CARTESIAN_POINT ( 'NONE',  ( -23.96075635701088657, -17.45014263229036899, 66.09357239682297802 ) ) ;
#20862=CARTESIAN_POINT ( 'NONE',  ( -19.86401518824997581, -21.42384811948916479, 69.22010401872219632 ) ) ;
#20864=CARTESIAN_POINT ( 'NONE',  ( -24.11881394502254849, -17.01995806294775448, 73.16863963025599560 ) ) ;
#20865=CARTESIAN_POINT ( 'NONE',  ( -22.71955324316818547, -10.22924783853478559, 70.08348758896158870 ) ) ;
#20867=FACE_OUTER_BOUND ( 'NONE', #29799, .T. ) ;
#20868=CARTESIAN_POINT ( 'NONE',  ( -16.81162750399036909, -21.83617793957379050, 65.43384172164481072 ) ) ;
#20869=CARTESIAN_POINT ( 'NONE',  ( -10.06841751317020872, -15.99566775706410482, 68.16423218926057359 ) ) ;
#20870=EDGE_CURVE ( 'NONE', #4167, #39713, #24585, .T. ) ;
#20871=B_SPLINE_CURVE_WITH_KNOTS ( 'NONE', 3,
 ( #35824, #40028, #21322, #9753, #43979, #24770, #46689, #27962, #21558, #40270 ),
 .UNSPECIFIED., .F., .F.,
 ( 4, 2, 2, 2, 4 ),
 ( 0.1272669073657797523, 0.2522669073488085223, 0.3772669073318372090, 0.5022669073148660068, 0.6272669072978946936 ),
 .UNSPECIFIED. ) ;
#20872=ORIENTED_EDGE ( 'NONE', *, *, #16103, .F. ) ;
#20873=CARTESIAN_POINT ( 'NONE',  ( -11.46028008028683942, -18.56947564720590194, 61.56238700194530367 ) ) ;
#20875=CARTESIAN_POINT ( 'NONE',  ( -11.96084906401204506, -9.743958800322932490, 60.74413413563605957 ) ) ;
#20876=ADVANCED_FACE ( 'NONE', ( #8749 ), #19249, .T. ) ;
#20877=ADVANCED_FACE ( 'NONE', ( #2309 ), #25210, .T. ) ;
#20878=VERTEX_POINT ( 'NONE', #2067 ) ;
#20879=ORIENTED_EDGE ( 'NONE', *, *, #35791, .F. ) ;
#20880=CARTESIAN_POINT ( 'NONE',  ( -14.88644031773417531, -21.33303323181352340, 58.35721170509270905 ) ) ;
#20882=CARTESIAN_POINT ( 'NONE',  ( -11.34006216982616166, -11.24017310230250111, 57.41722930122209334 ) ) ;
#20885=CARTESIAN_POINT ( 'NONE',  ( -24.12651600458584511, -12.62191667979047338, 73.25697658996379857 ) ) ;
#20886=CARTESIAN_POINT ( 'NONE',  ( -12.32149116705671332, -19.60131283701424820, 57.94184834235668546 ) ) ;
#20887=FACE_OUTER_BOUND ( 'NONE', #20585, .T. ) ;
#20888=CARTESIAN_POINT ( 'NONE',  ( -16.77581700079705485, -22.23100064957188593, 68.88834796384273318 ) ) ;
#20890=VERTEX_POINT ( 'NONE', #13617 ) ;
#20894=CARTESIAN_POINT ( 'NONE',  ( -16.03289653659843594, -7.947204529361793668, 67.25080481985611414 ) ) ;
#20895=CARTESIAN_POINT ( 'NONE',  ( -13.54792730259346456, -8.920061342218058797, 57.25495614889487683 ) ) ;
#20897=CARTESIAN_POINT ( 'NONE',  ( -20.30052658356369477, -21.25444530744949390, 72.56046004230084634 ) ) ;
#20899=ORIENTED_EDGE ( 'NONE', *, *, #41673, .F. ) ;
#20900=EDGE_CURVE ( 'NONE', #2612, #33183, #16271, .T. ) ;
#20902=CARTESIAN_POINT ( 'NONE',  ( -24.42218830102925509, -14.64588410380239480, 62.71296487252168816 ) ) ;
#20903=CARTESIAN_POINT ( 'NONE',  ( -11.17855889551124982, -18.87086522978130532, 64.86211687253867808 ) ) ;
#20905=CARTESIAN_POINT ( 'NONE',  ( -11.14016733508048240, -18.81244675540447631, 64.93362470803228348 ) ) ;
#20906=EDGE_CURVE ( 'NONE', #18272, #1731, #34627, .T. ) ;
#20907=CARTESIAN_POINT ( 'NONE',  ( -22.23733827145997566, -19.96043728507621040, 65.70421731380814379 ) ) ;
#20908=CARTESIAN_POINT ( 'NONE',  ( -17.77754172124238963, -7.367517167730140315, 60.12414849856542531 ) ) ;
#20909=EDGE_CURVE ( 'NONE', #20596, #42703, #20455, .T. ) ;
#20910=DIRECTION ( 'NONE',  ( 0.1847813031241905823, -0.9827796650397888634, 7.910442904995644076E-08 ) ) ;
#20911=CARTESIAN_POINT ( 'NONE',  ( -18.85724798917316392, -7.906108138700305155, 67.18599644112759961 ) ) ;
#20912=CARTESIAN_POINT ( 'NONE',  ( -11.10758613922248905, -10.85889423684567490, 57.31564880789826333 ) ) ;
#20913=DIRECTION ( 'NONE',  ( -8.766499794606700203E-07, -3.805972782304116817E-07, 0.9999999999995433653 ) ) ;
#20914=VERTEX_POINT ( 'NONE', #47135 ) ;
#20915=CARTESIAN_POINT ( 'NONE',  ( -23.04636716567627275, -18.97944391780718121, 58.95698644230029117 ) ) ;
#20916=ORIENTED_EDGE ( 'NONE', *, *, #9026, .F. ) ;
#20917=CARTESIAN_POINT ( 'NONE',  ( -22.27077318787935667, -19.92919612165446708, 65.99861962659834091 ) ) ;
#20919=ORIENTED_EDGE ( 'NONE', *, *, #40108, .T. ) ;
#20920=CARTESIAN_POINT ( 'NONE',  ( -13.65110067086344792, -21.23324738024127356, 68.57129742521463811 ) ) ;
#20923=CARTESIAN_POINT ( 'NONE',  ( -11.97955794321693190, -10.40884752579252037, 71.25276566430856917 ) ) ;
#20924=CARTESIAN_POINT ( 'NONE',  ( -14.86627003481517839, -7.811970263561289762, 56.96504677300865893 ) ) ;
#20925=B_SPLINE_CURVE_WITH_KNOTS ( 'NONE', 3,
 ( #4382, #41318, #23110, #18410, #18654, #22875, #41082, #7855, #37869, #4157 ),
 .UNSPECIFIED., .F., .F.,
 ( 4, 2, 2, 2, 4 ),
 ( 0.000000000000000000, 0.2500000000000000000, 0.5000000000000000000, 0.7500000000000000000, 1.000000000000000000 ),
 .UNSPECIFIED. ) ;
#20927=ORIENTED_EDGE ( 'NONE', *, *, #46819, .T. ) ;
#20928=DIRECTION ( 'NONE',  ( -0.3109111061729914471, -0.9504389954427826526, -3.354176643444200258E-08 ) ) ;
#20930=CARTESIAN_POINT ( 'NONE',  ( -10.68551981713787136, -12.73596763222149164, 64.28308208171728211 ) ) ;
#20931=VECTOR ( 'NONE', #43379, 1000.000000000000114 ) ;
#20932=CARTESIAN_POINT ( 'NONE',  ( -24.59330981698489538, -12.78255162097813447, 66.44100198564684945 ) ) ;
#20935=EDGE_CURVE ( 'NONE', #15392, #2586, #439, .T. ) ;
#20936=ORIENTED_EDGE ( 'NONE', *, *, #436, .F. ) ;
#20937=EDGE_LOOP ( 'NONE', ( #11408, #44828 ) ) ;
#20938=CARTESIAN_POINT ( 'NONE',  ( -11.77071142734671660, -18.93707127637648568, 68.40792700413676641 ) ) ;
#20939=ORIENTED_EDGE ( 'NONE', *, *, #5717, .T. ) ;
#20940=CARTESIAN_POINT ( 'NONE',  ( -23.82269675168534206, -17.76935429418745827, 59.29818642892983860 ) ) ;
#20941=CARTESIAN_POINT ( 'NONE',  ( -19.28643826901335245, -21.55824987104777790, 62.06673959588616185 ) ) ;
#20945=CARTESIAN_POINT ( 'NONE',  ( -12.41631187035346962, -9.915882575277414901, 60.74845061171743055 ) ) ;
#20946=ORIENTED_EDGE ( 'NONE', *, *, #42220, .T. ) ;
#20947=EDGE_CURVE ( 'NONE', #12237, #10231, #3379, .T. ) ;
#20949=CARTESIAN_POINT ( 'NONE',  ( -16.65185932245351808, -21.81708442718849383, 65.51092266128213737 ) ) ;
#20950=CARTESIAN_POINT ( 'NONE',  ( -10.43098718212803000, -15.70539730037032911, 61.32316937334011442 ) ) ;
#20951=CARTESIAN_POINT ( 'NONE',  ( -24.47243858273885664, -15.17772250287404567, 59.38732937676161328 ) ) ;
#20952=DIRECTION ( 'NONE',  ( 0.2843796944294933460, 0.9587117342539337450, 5.205739956168972140E-08 ) ) ;
#20953=( BOUNDED_SURFACE ( )  B_SPLINE_SURFACE ( 3, 1, ( 
 ( #21098, #31934 ),
 ( #32185, #13444 ),
 ( #28490, #24565 ),
 ( #40295, #36095 ),
 ( #21584, #28961 ),
 ( #13194, #36562 ),
 ( #43515, #10503 ) ),
 .UNSPECIFIED., .T., .F., .F. ) 
 B_SPLINE_SURFACE_WITH_KNOTS ( ( 4, 3, 4 ),
 ( 2, 2 ),
 ( 0.000000000000000000, 0.5000000000000000000, 1.000000000000000000 ),
 ( 0.000000000000000000, 1.000000000000000000 ),
 .UNSPECIFIED. ) 
 GEOMETRIC_REPRESENTATION_ITEM ( )  RATIONAL_B_SPLINE_SURFACE ( (
 ( 1.000000000000000000, 1.000000000000000000),
 ( 0.3333333333333335369, 0.3333333333333330373),
 ( 0.3333333333333335369, 0.3333333333333330373),
 ( 1.000000000000000000, 1.000000000000000000),
 ( 0.3333333333333333703, 0.3333333333333333703),
 ( 0.3333333333333333703, 0.3333333333333333703),
 ( 1.000000000000000000, 1.000000000000000000) ) ) 
 REPRESENTATION_ITEM ( '' )  SURFACE ( )  );
#20954=ORIENTED_EDGE ( 'NONE', *, *, #27294, .T. ) ;
#20957=CARTESIAN_POINT ( 'NONE',  ( -24.07704370891654122, -17.14264987453632827, 72.89808101046213551 ) ) ;
#20958=CARTESIAN_POINT ( 'NONE',  ( -23.34715393241125980, -19.32824242744487719, 59.00597867367864779 ) ) ;
#20959=EDGE_LOOP ( 'NONE', ( #40987, #6488, #37612, #30312, #45080 ) ) ;
#20960=B_SPLINE_CURVE_WITH_KNOTS ( 'NONE', 1,
 ( #20930, #46564 ),
 .UNSPECIFIED., .F., .F.,
 ( 2, 2 ),
 ( 0.000000000000000000, 1.000000000000000000 ),
 .UNSPECIFIED. ) ;
#20961=( BOUNDED_CURVE ( )  B_SPLINE_CURVE ( 3, ( #42597, #23147, #38375, #19434 ),
 .UNSPECIFIED., .F., .F. ) 
 B_SPLINE_CURVE_WITH_KNOTS ( ( 4, 4 ),
 ( 0.4074455897393639559, 0.5000000000000000000 ),
 .UNSPECIFIED. ) 
 CURVE ( )  GEOMETRIC_REPRESENTATION_ITEM ( )  RATIONAL_B_SPLINE_CURVE ( ( 0.6983129098260814072, 0.7760317562606796615, 0.8765941196519831946, 0.9999999999999863443 ) ) 
 REPRESENTATION_ITEM ( '' )  );
#20964=VECTOR ( 'NONE', #13241, 1000.000000000000114 ) ;
#20966=CARTESIAN_POINT ( 'NONE',  ( -20.13271805750754950, -8.299978134201072777, 70.53628287813307907 ) ) ;
#20967=CARTESIAN_POINT ( 'NONE',  ( -17.87922833762628017, -21.79450501533915840, 62.17535931805394256 ) ) ;
#20969=CARTESIAN_POINT ( 'NONE',  ( -21.93498049285785001, -8.880082814678040393, 66.86161196829021947 ) ) ;
#20971=CARTESIAN_POINT ( 'NONE',  ( -10.59617215550872693, -13.26637052363490810, 71.49363181683084179 ) ) ;
#20973=CARTESIAN_POINT ( 'NONE',  ( -11.95665483952126351, -19.86987859786184885, 58.11956535282013192 ) ) ;
#20978=FACE_OUTER_BOUND ( 'NONE', #15259, .T. ) ;
#20980=CARTESIAN_POINT ( 'NONE',  ( -13.75553758628831424, -8.845634084518218643, 57.08040952457714923 ) ) ;
#20982=CARTESIAN_POINT ( 'NONE',  ( -15.39536932222403287, -19.92137602241599836, 53.49999999999995026 ) ) ;
#20985=CARTESIAN_POINT ( 'NONE',  ( -24.66730449611544529, -13.06573935865489844, 62.94768786448354092 ) ) ;
#20986=CARTESIAN_POINT ( 'NONE',  ( -16.15373903644572451, -7.468189973811639959, 60.32215689887271992 ) ) ;
#20987=B_SPLINE_CURVE_WITH_KNOTS ( 'NONE', 1,
 ( #22397, #7886 ),
 .UNSPECIFIED., .F., .F.,
 ( 2, 2 ),
 ( 0.000000000000000000, 1.000000000000000000 ),
 .UNSPECIFIED. ) ;
#20988=CARTESIAN_POINT ( 'NONE',  ( -13.37636250268599092, -20.58507941322447365, 61.93135214938352107 ) ) ;
#20989=CARTESIAN_POINT ( 'NONE',  ( -14.07761608144266674, -20.95746532167037302, 71.92607703845176559 ) ) ;
#20991=ADVANCED_FACE ( 'NONE', ( #31868 ), #46886, .T. ) ;
#20992=ORIENTED_EDGE ( 'NONE', *, *, #977, .F. ) ;
#20995=ORIENTED_EDGE ( 'NONE', *, *, #16142, .F. ) ;
#20996=CARTESIAN_POINT ( 'NONE',  ( -10.37394849890712401, -14.76283852923608464, 71.61310637325181006 ) ) ;
#20997=DIRECTION ( 'NONE',  ( -0.8201047403141396019, 0.5722134347551370848, 7.883065731424289661E-08 ) ) ;
#20998=FACE_OUTER_BOUND ( 'NONE', #2138, .T. ) ;
#20999=CARTESIAN_POINT ( 'NONE',  ( -16.22163365158137793, -21.75594374583092616, 58.58585541130567975 ) ) ;
#21000=ORIENTED_EDGE ( 'NONE', *, *, #9829, .F. ) ;
#21001=CARTESIAN_POINT ( 'NONE',  ( -23.91439695282944200, -17.43141281116713515, 66.24357239631997629 ) ) ;
#21003=CARTESIAN_POINT ( 'NONE',  ( -23.65624089557865872, -11.51332380282628343, 66.57214514605458078 ) ) ;
#21004=VECTOR ( 'NONE', #8725, 1000.000000000000114 ) ;
#21005=ADVANCED_FACE ( 'NONE', ( #44908 ), #85, .F. ) ;
#21007=CARTESIAN_POINT ( 'NONE',  ( -21.94239013569476171, -20.22099906679998327, 58.76442899523448204 ) ) ;
#21008=ORIENTED_EDGE ( 'NONE', *, *, #33907, .F. ) ;
#21011=EDGE_CURVE ( 'NONE', #20172, #16663, #36734, .T. ) ;
#21013=ADVANCED_FACE ( 'NONE', ( #37230 ), #21410, .T. ) ;
#21014=LINE ( 'NONE', #18015, #39767 ) ;
#21015=CARTESIAN_POINT ( 'NONE',  ( -24.15317529415027309, -18.00651073652558054, 59.11104256832918935 ) ) ;
#21016=CARTESIAN_POINT ( 'NONE',  ( -24.20884359724224311, -11.73171579724705005, 59.59740298356196320 ) ) ;
#21017=CARTESIAN_POINT ( 'NONE',  ( -16.59344707466788549, -21.75974795715521282, 65.52564390620075585 ) ) ;
#21018=VERTEX_POINT ( 'NONE', #3024 ) ;
#21019=ORIENTED_EDGE ( 'NONE', *, *, #27011, .T. ) ;
#21021=EDGE_CURVE ( 'NONE', #30787, #37220, #28059, .T. ) ;
#21025=VERTEX_POINT ( 'NONE', #3767 ) ;
#21026=CARTESIAN_POINT ( 'NONE',  ( -21.02147767800124356, -20.81425002204343500, 65.88453904403851880 ) ) ;
#21029=CARTESIAN_POINT ( 'NONE',  ( -24.42256168835771746, -14.59956871858401684, 66.29365741613838736 ) ) ;
#21030=CARTESIAN_POINT ( 'NONE',  ( -24.47432067347917695, -14.77756146504815327, 59.52828185648635184 ) ) ;
#21032=VECTOR ( 'NONE', #26355, 1000.000000000000227 ) ;
#21033=EDGE_LOOP ( 'NONE', ( #14463, #40543, #23105, #10517, #6862 ) ) ;
#21035=CARTESIAN_POINT ( 'NONE',  ( -12.24245737956772473, -19.51581737952565376, 57.92682380653661056 ) ) ;
#21036=EDGE_LOOP ( 'NONE', ( #42192, #33266 ) ) ;
#21038=CARTESIAN_POINT ( 'NONE',  ( -24.41160895735743352, -13.85031893932584701, 73.00782755091154286 ) ) ;
#21041=CARTESIAN_POINT ( 'NONE',  ( -16.72764935575746748, -21.77453510730240183, 65.29852372421919426 ) ) ;
#21043=EDGE_LOOP ( 'NONE', ( #32993, #4668, #24083, #48291 ) ) ;
#21044=CARTESIAN_POINT ( 'NONE',  ( -22.17374636168253943, -9.068608547125135644, 63.37809084343794552 ) ) ;
#21045=FACE_OUTER_BOUND ( 'NONE', #20480, .T. ) ;
#21046=CARTESIAN_POINT ( 'NONE',  ( -24.30112618867181240, -13.25578303422174997, 59.64795780745660636 ) ) ;
#21047=FACE_OUTER_BOUND ( 'NONE', #196, .T. ) ;
#21050=EDGE_CURVE ( 'NONE', #39081, #22354, #18687, .T. ) ;
#21051=CARTESIAN_POINT ( 'NONE',  ( -17.11809369177854379, -21.86054179209348192, 68.85127668957714775 ) ) ;
#21053=ORIENTED_EDGE ( 'NONE', *, *, #48071, .T. ) ;
#21054=PLANE ( 'NONE',  #19810 ) ;
#21056=CARTESIAN_POINT ( 'NONE',  ( -20.47136568995129480, -10.23054578351413468, 54.07175714974879099 ) ) ;
#21057=ORIENTED_EDGE ( 'NONE', *, *, #34313, .T. ) ;
#21062=EDGE_CURVE ( 'NONE', #1905, #20878, #22763, .T. ) ;
#21063=CARTESIAN_POINT ( 'NONE',  ( -14.00884730389179822, -20.92003478889483858, 72.20991175584978805 ) ) ;
#21064=AXIS2_PLACEMENT_3D ( 'NONE', #38399, #8153, #23166 ) ;
#21065=ADVANCED_FACE ( 'NONE', ( #38707 ), #33028, .T. ) ;
#21066=CARTESIAN_POINT ( 'NONE',  ( -23.72077351878440510, -11.75113111449199721, 59.67339008053482274 ) ) ;
#21067=CARTESIAN_POINT ( 'NONE',  ( -15.94604045176571283, -7.966968909199487747, 63.89684263511286133 ) ) ;
#21068=CARTESIAN_POINT ( 'NONE',  ( -19.85909425162068942, -21.37257694502213567, 72.64634926892956912 ) ) ;
#21069=CARTESIAN_POINT ( 'NONE',  ( -22.88850900265194355, -15.54278860761184866, 53.88362224778186516 ) ) ;
#21070=AXIS2_PLACEMENT_3D ( 'NONE', #19191, #4411, #15473 ) ;
#21071=AXIS2_PLACEMENT_3D ( 'NONE', #13192, #43514, #24794 ) ;
#21072=ORIENTED_EDGE ( 'NONE', *, *, #8484, .F. ) ;
#21073=ORIENTED_EDGE ( 'NONE', *, *, #27493, .F. ) ;
#21074=EDGE_CURVE ( 'NONE', #18139, #3011, #38073, .T. ) ;
#21076=B_SPLINE_CURVE_WITH_KNOTS ( 'NONE', 3,
 ( #23810, #16138, #24048, #27727, #5327, #46204, #23314, #31671, #4356, #34374 ),
 .UNSPECIFIED., .F., .F.,
 ( 4, 2, 2, 2, 4 ),
 ( 0.000000000000000000, 0.2500000000000000000, 0.5000000000000000000, 0.7500000000000000000, 1.000000000000000000 ),
 .UNSPECIFIED. ) ;
#21079=DIRECTION ( 'NONE',  ( 0.3374354101627465297, 0.9413486835218388693, 1.423378189492272923E-08 ) ) ;
#21080=EDGE_CURVE ( 'NONE', #32817, #35558, #36483, .T. ) ;
#21083=ORIENTED_EDGE ( 'NONE', *, *, #13802, .F. ) ;
#21084=CARTESIAN_POINT ( 'NONE',  ( -15.55648817577099585, -8.010769314271311003, 74.09457776258329886 ) ) ;
#21085=DIRECTION ( 'NONE',  ( -2.430360958779124298E-06, -9.751098539734333949E-07, 0.9999999999965712982 ) ) ;
#21086=( BOUNDED_CURVE ( )  B_SPLINE_CURVE ( 3, ( #40079, #20882, #32449, #17158 ),
 .UNSPECIFIED., .F., .F. ) 
 B_SPLINE_CURVE_WITH_KNOTS ( ( 4, 4 ),
 ( 0.000000000000000000, 0.4074455897393671200 ),
 .UNSPECIFIED. ) 
 CURVE ( )  GEOMETRIC_REPRESENTATION_ITEM ( )  RATIONAL_B_SPLINE_CURVE ( ( 1.000000000000000000, 0.4567392136813310244, 0.3561768502900299338, 0.6983129098260968393 ) ) 
 REPRESENTATION_ITEM ( '' )  );
#21087=ORIENTED_EDGE ( 'NONE', *, *, #5334, .T. ) ;
#21089=ORIENTED_EDGE ( 'NONE', *, *, #1147, .T. ) ;
#21090=FACE_OUTER_BOUND ( 'NONE', #7292, .T. ) ;
#21091=CARTESIAN_POINT ( 'NONE',  ( -10.40888601095206134, -14.10966482229656194, 61.21821293885882653 ) ) ;
#21092=CARTESIAN_POINT ( 'NONE',  ( -14.43571338001569870, -7.984821196993008741, 63.88955222746418627 ) ) ;
#21093=ORIENTED_EDGE ( 'NONE', *, *, #8608, .F. ) ;
#21095=DIRECTION ( 'NONE',  ( 7.652304183832323392E-06, 2.165757503891338892E-06, 0.9999999999683758523 ) ) ;
#21097=EDGE_CURVE ( 'NONE', #11018, #22946, #20829, .T. ) ;
#21098=CARTESIAN_POINT ( 'NONE',  ( -22.75539019595755263, -10.19575032747719590, 66.82710158566565894 ) ) ;
#21099=FACE_OUTER_BOUND ( 'NONE', #26262, .T. ) ;
#21100=ORIENTED_EDGE ( 'NONE', *, *, #32711, .F. ) ;
#21101=CARTESIAN_POINT ( 'NONE',  ( -20.77672337442954031, -20.95411300689461953, 58.83578372821326496 ) ) ;
#21103=AXIS2_PLACEMENT_3D ( 'NONE', #46953, #2857, #24570 ) ;
#21104=EDGE_LOOP ( 'NONE', ( #28113, #12305 ) ) ;
#21105=DIRECTION ( 'NONE',  ( 0.9904243694481097426, 0.1380563957348939774, 6.973877024228147881E-08 ) ) ;
#21106=DIRECTION ( 'NONE',  ( 0.3111098983483954750, 0.8385765505603235415, 0.4472135954999582608 ) ) ;
#21108=DIRECTION ( 'NONE',  ( 0.9271861211590526342, 0.3746009833543293421, -1.005599061620490611E-08 ) ) ;
#21110=CARTESIAN_POINT ( 'NONE',  ( -17.20949509180255887, -7.759470163990226155, 74.37506982372057962 ) ) ;
#21111=DIRECTION ( 'NONE',  ( 0.9372362738803845517, 0.3486949482324239735, -5.386914174890155429E-09 ) ) ;
#21112=ORIENTED_EDGE ( 'NONE', *, *, #16613, .T. ) ;
#21115=CARTESIAN_POINT ( 'NONE',  ( -15.09544287645192640, -21.46351977604527761, 65.10596681500476279 ) ) ;
#21116=FACE_OUTER_BOUND ( 'NONE', #7533, .T. ) ;
#21118=CARTESIAN_POINT ( 'NONE',  ( -10.38974003836240634, -14.29666208179129150, 68.27288787427933414 ) ) ;
#21119=( BOUNDED_CURVE ( )  B_SPLINE_CURVE ( 3, ( #36490, #2771, #32098, #28158 ),
 .UNSPECIFIED., .F., .F. ) 
 B_SPLINE_CURVE_WITH_KNOTS ( ( 4, 4 ),
 ( 0.000000000000000000, 0.4074455897393701176 ),
 .UNSPECIFIED. ) 
 CURVE ( )  GEOMETRIC_REPRESENTATION_ITEM ( )  RATIONAL_B_SPLINE_CURVE ( ( 1.000000000000000000, 0.4567392136813304138, 0.3561768502900297118, 0.6983129098260978385 ) ) 
 REPRESENTATION_ITEM ( '' )  );
#21120=CARTESIAN_POINT ( 'NONE',  ( -12.50648677543191134, -9.746390325112967545, 60.70350793514798937 ) ) ;
#21121=EDGE_LOOP ( 'NONE', ( #5382, #23893, #47865, #46684, #24178 ) ) ;
#21122=ORIENTED_EDGE ( 'NONE', *, *, #5429, .T. ) ;
#21123=LINE ( 'NONE', #36120, #40882 ) ;
#21126=CARTESIAN_POINT ( 'NONE',  ( -19.92736525831631766, -21.34646298403863085, 72.70478735915031621 ) ) ;
#21128=CARTESIAN_POINT ( 'NONE',  ( -10.12326218194131044, -13.32541594658350448, 74.86312942357149325 ) ) ;
#21129=CARTESIAN_POINT ( 'NONE',  ( -23.85760449859744625, -11.05106826658364838, 70.00555402674318373 ) ) ;
#21130=CARTESIAN_POINT ( 'NONE',  ( -12.37644175686812709, -19.65923236128709561, 61.39678630681033411 ) ) ;
#21131=CARTESIAN_POINT ( 'NONE',  ( -12.89671927708317689, -20.22380232670898081, 68.49224713894388117 ) ) ;
#21133=ORIENTED_EDGE ( 'NONE', *, *, #3796, .F. ) ;
#21134=EDGE_LOOP ( 'NONE', ( #87, #9659, #44325, #11722, #15219 ) ) ;
#21135=EDGE_CURVE ( 'NONE', #25681, #37096, #25853, .T. ) ;
#21136=CARTESIAN_POINT ( 'NONE',  ( -10.45033584411928551, -15.86823462405053853, 61.03788874849474411 ) ) ;
#21137=CARTESIAN_POINT ( 'NONE',  ( -23.11114181986270566, -9.996704532105994190, 66.64208010989614195 ) ) ;
#21139=CARTESIAN_POINT ( 'NONE',  ( -11.39216336840796373, -18.45920852072106300, 61.29182966166492719 ) ) ;
#21140=CARTESIAN_POINT ( 'NONE',  ( -10.53786819255349805, -17.65216208274645382, 68.24721944767701132 ) ) ;
#21141=EDGE_CURVE ( 'NONE', #18208, #2492, #5763, .T. ) ;
#21142=CARTESIAN_POINT ( 'NONE',  ( -11.12358220677134035, -11.75903396576748605, 71.08860871065073184 ) ) ;
#21146=ORIENTED_EDGE ( 'NONE', *, *, #34780, .T. ) ;
#21147=CARTESIAN_POINT ( 'NONE',  ( -22.92319923916556235, -10.39759239192951235, 63.07185995337424345 ) ) ;
#21150=CARTESIAN_POINT ( 'NONE',  ( -10.38377074815290868, -15.30802594933397920, 61.18222038349547631 ) ) ;
#21152=EDGE_CURVE ( 'NONE', #19754, #47755, #16331, .T. ) ;
#21153=ORIENTED_EDGE ( 'NONE', *, *, #43993, .F. ) ;
#21154=EDGE_CURVE ( 'NONE', #21258, #22071, #25156, .T. ) ;
#21159=DIRECTION ( 'NONE',  ( 1.205044182495138397E-05, 2.694341358818416019E-06, 0.9999999999237635384 ) ) ;
#21161=CARTESIAN_POINT ( 'NONE',  ( -23.05544494128708521, -18.96707680103153493, 59.07513778477354549 ) ) ;
#21162=ORIENTED_EDGE ( 'NONE', *, *, #25735, .T. ) ;
#21163=CARTESIAN_POINT ( 'NONE',  ( -23.59327504554355315, -11.39630409041826020, 69.90682860766239060 ) ) ;
#21164=CARTESIAN_POINT ( 'NONE',  ( -10.21764033814386963, -12.91954908504599331, 67.92327745040803677 ) ) ;
#21166=CARTESIAN_POINT ( 'NONE',  ( -13.72534930678190079, -21.27637739626202062, 68.61658465623135328 ) ) ;
#21167=CARTESIAN_POINT ( 'NONE',  ( -12.54422445394979135, -19.90840678475983694, 71.95086485943772914 ) ) ;
#21172=CARTESIAN_POINT ( 'NONE',  ( -17.59331746331979929, -7.761237803891376963, 63.55057029381061540 ) ) ;
#21173=CARTESIAN_POINT ( 'NONE',  ( -10.88209246082447912, -17.29963176008448400, 64.92739380462948873 ) ) ;
#21174=ORIENTED_EDGE ( 'NONE', *, *, #15675, .F. ) ;
#21176=VECTOR ( 'NONE', #22441, 1000.000000000000000 ) ;
#21178=CARTESIAN_POINT ( 'NONE',  ( -17.26457240846633567, -7.760713630915982542, 70.50507891880883449 ) ) ;
#21179=DIRECTION ( 'NONE',  ( 0.9660698163281071782, 0.2582810677919975539, -5.363434502754611677E-08 ) ) ;
#21180=CARTESIAN_POINT ( 'NONE',  ( -23.00454255336054743, -10.50046069577333263, 59.88731295783226471 ) ) ;
#21181=ORIENTED_EDGE ( 'NONE', *, *, #8727, .T. ) ;
#21183=FACE_OUTER_BOUND ( 'NONE', #17974, .T. ) ;
#21184=CARTESIAN_POINT ( 'NONE',  ( -24.31717724401442027, -16.02832029180493478, 62.66616618629565494 ) ) ;
#21185=EDGE_LOOP ( 'NONE', ( #702, #1557, #16244, #33681, #9857, #22833, #14502, #26419, #44463, #25685, #16140, #21947, #44860, #27087, #1485, #44631, #32304, #48104, #26884, #7873, #47857, #25643, #9416, #18599, #1929, #38607, #19912, #2450, #42719, #40486, #38465, #21181, #3034 ) ) ;
#21186=CARTESIAN_POINT ( 'NONE',  ( -10.56492483649129710, -13.18000429128331596, 71.50828586225091499 ) ) ;
#21189=CARTESIAN_POINT ( 'NONE',  ( -15.83093346616859876, -7.941424302753512521, 67.43447455194694840 ) ) ;
#21191=CARTESIAN_POINT ( 'NONE',  ( -20.58562488885964825, -8.063118024066820766, 66.94250577013032455 ) ) ;
#21194=CARTESIAN_POINT ( 'NONE',  ( -11.10681587527927938, -11.67891925637714401, 71.10332952723315714 ) ) ;
#21195=CARTESIAN_POINT ( 'NONE',  ( -14.86706299937602793, -21.37930449507021180, 61.64160199363316650 ) ) ;
#21196=DIRECTION ( 'NONE',  ( 0.5510797171261918592, -0.8280216580999281151, 0.1033986416233892563 ) ) ;
#21197=CARTESIAN_POINT ( 'NONE',  ( -11.42622260759249286, -18.51434353338492400, 61.57710833179551457 ) ) ;
#21198=EDGE_LOOP ( 'NONE', ( #5748, #1259, #11003, #10990, #11281 ) ) ;
#21199=VERTEX_POINT ( 'NONE', #24672 ) ;
#21200=CARTESIAN_POINT ( 'NONE',  ( -24.87289997924709439, -14.67112824012948202, 62.82801159608117558 ) ) ;
#21201=CARTESIAN_POINT ( 'NONE',  ( -14.07810500574514556, -21.01869930352526694, 68.66444892306193992 ) ) ;
#21202=AXIS2_PLACEMENT_3D ( 'NONE', #18162, #33174, #14440 ) ;
#21203=CARTESIAN_POINT ( 'NONE',  ( -24.09792889798371007, -17.08130376423426000, 73.18336032035891492 ) ) ;
#21204=VERTEX_POINT ( 'NONE', #39916 ) ;
#21206=EDGE_CURVE ( 'NONE', #25341, #14217, #39662, .T. ) ;
#21207=CARTESIAN_POINT ( 'NONE',  ( -20.75918756122348441, -8.147305293919229641, 63.42626095967343502 ) ) ;
#21208=B_SPLINE_CURVE_WITH_KNOTS ( 'NONE', 3,
 ( #46844, #38966, #32544, #35265, #13805, #39694, #13570, #17272, #35984, #5494 ),
 .UNSPECIFIED., .F., .F.,
 ( 4, 2, 2, 2, 4 ),
 ( 0.000000000000000000, 0.2500000000000000000, 0.5000000000000000000, 0.7500000000000000000, 1.000000000000000000 ),
 .UNSPECIFIED. ) ;
#21210=EDGE_CURVE ( 'NONE', #41834, #14119, #987, .T. ) ;
#21211=ADVANCED_FACE ( 'NONE', ( #20727 ), #44419, .T. ) ;
#21212=VERTEX_POINT ( 'NONE', #20492 ) ;
#21213=DIRECTION ( 'NONE',  ( -0.8244078399817417191, -0.5659962132175737626, -7.627400653636452305E-08 ) ) ;
#21215=CARTESIAN_POINT ( 'NONE',  ( -12.51352073908361184, -20.41184545669705130, 71.91379515285952095 ) ) ;
#21216=CARTESIAN_POINT ( 'NONE',  ( -16.82968708298378857, -21.83425273348639806, 68.99000854178609643 ) ) ;
#21217=ORIENTED_EDGE ( 'NONE', *, *, #41730, .T. ) ;
#21219=VERTEX_POINT ( 'NONE', #5719 ) ;
#21220=CARTESIAN_POINT ( 'NONE',  ( -14.19282086353638661, -8.542981675383003903, 71.01485553001869278 ) ) ;
#21221=PLANE ( 'NONE',  #22047 ) ;
#21222=CARTESIAN_POINT ( 'NONE',  ( -10.76763519559319882, -17.13171766695033327, 61.15743118826002700 ) ) ;
#21224=CARTESIAN_POINT ( 'NONE',  ( -21.36930209557634086, -21.12890771240575916, 69.16176048667763610 ) ) ;
#21225=CARTESIAN_POINT ( 'NONE',  ( -24.47354813883760016, -12.39902559715248032, 73.42720875634239519 ) ) ;
#21226=CARTESIAN_POINT ( 'NONE',  ( -24.10584550580110985, -12.56049697540380095, 73.54225570139644219 ) ) ;
#21230=VERTEX_POINT ( 'NONE', #13073 ) ;
#21232=CARTESIAN_POINT ( 'NONE',  ( -11.79792781917550570, -18.97409009807959279, 71.68685885149984927 ) ) ;
#21233=CARTESIAN_POINT ( 'NONE',  ( -24.69063629745726374, -16.45233172012289558, 59.27332428859715918 ) ) ;
#21236=CARTESIAN_POINT ( 'NONE',  ( -24.26335596148664564, -16.30820463372698725, 62.78255861953126526 ) ) ;
#21237=EDGE_CURVE ( 'NONE', #10202, #18022, #43132, .T. ) ;
#21241=CARTESIAN_POINT ( 'NONE',  ( -21.24416713127566325, -21.20535426119284139, 65.62808000370414163 ) ) ;
#21242=CARTESIAN_POINT ( 'NONE',  ( -11.53247254227971830, -18.68106628708273931, 65.04707076447483871 ) ) ;
#21243=VERTEX_POINT ( 'NONE', #43626 ) ;
#21244=CARTESIAN_POINT ( 'NONE',  ( -11.83425018566923370, -19.11833757169930692, 68.37256453262955347 ) ) ;
#21245=CARTESIAN_POINT ( 'NONE',  ( -17.98657259272421172, -21.83703102787368167, 62.16063850355641307 ) ) ;
#21246=CARTESIAN_POINT ( 'NONE',  ( -10.50429924535250414, -16.15944446069506668, 71.46222527016213633 ) ) ;
#21247=CARTESIAN_POINT ( 'NONE',  ( -12.91576191806997542, -9.388722997169708151, 71.13453240065665284 ) ) ;
#21249=FACE_OUTER_BOUND ( 'NONE', #33886, .T. ) ;
#21250=CARTESIAN_POINT ( 'NONE',  ( -9.939267784769082681, -14.33236412611010913, 47.99999999999994316 ) ) ;
#21251=( BOUNDED_CURVE ( )  B_SPLINE_CURVE ( 3, ( #25944, #14573, #40962, #29634 ),
 .UNSPECIFIED., .F., .F. ) 
 B_SPLINE_CURVE_WITH_KNOTS ( ( 4, 4 ),
 ( 0.000000000000000000, 0.4074455897393683412 ),
 .UNSPECIFIED. ) 
 CURVE ( )  GEOMETRIC_REPRESENTATION_ITEM ( )  RATIONAL_B_SPLINE_CURVE ( ( 1.000000000000000000, 0.4567392136813350767, 0.3561768502900314326, 0.6983129098260890677 ) ) 
 REPRESENTATION_ITEM ( '' )  );
#21253=CARTESIAN_POINT ( 'NONE',  ( -12.72102574358543059, -9.031338699541656467, 71.04936556502208589 ) ) ;
#21254=FACE_OUTER_BOUND ( 'NONE', #35064, .T. ) ;
#21256=CARTESIAN_POINT ( 'NONE',  ( -16.94458744105653381, -7.374567917109038362, 74.14513580114275726 ) ) ;
#21257=CARTESIAN_POINT ( 'NONE',  ( -14.87973245694827718, -7.806975737088362344, 56.98966612870860615 ) ) ;
#21258=VERTEX_POINT ( 'NONE', #20966 ) ;
#21260=CARTESIAN_POINT ( 'NONE',  ( -11.46875891826176819, -18.48806303968299858, 61.27710833525312495 ) ) ;
#21261=ADVANCED_FACE ( 'NONE', ( #24905 ), #6185, .T. ) ;
#21262=CARTESIAN_POINT ( 'NONE',  ( -24.41050200104759682, -17.39623818674726863, 69.61328578849980886 ) ) ;
#21263=CARTESIAN_POINT ( 'NONE',  ( -20.80666424517567492, -21.44721877540349908, 58.80621670974001347 ) ) ;
#21266=( BOUNDED_SURFACE ( )  B_SPLINE_SURFACE ( 3, 1, ( 
 ( #37169, #26609 ),
 ( #749, #41627 ),
 ( #37413, #3710 ),
 ( #4435, #3455 ),
 ( #12074, #19215 ),
 ( #8376, #18712 ),
 ( #38154, #33725 ) ),
 .UNSPECIFIED., .T., .F., .F. ) 
 B_SPLINE_SURFACE_WITH_KNOTS ( ( 4, 3, 4 ),
 ( 2, 2 ),
 ( 0.000000000000000000, 0.5000000000000000000, 1.000000000000000000 ),
 ( 0.000000000000000000, 1.000000000000000000 ),
 .UNSPECIFIED. ) 
 GEOMETRIC_REPRESENTATION_ITEM ( )  RATIONAL_B_SPLINE_SURFACE ( (
 ( 1.000000000000000000, 1.000000000000000000),
 ( 0.3333333333333335369, 0.3333333333333330373),
 ( 0.3333333333333335369, 0.3333333333333330373),
 ( 1.000000000000000000, 1.000000000000000000),
 ( 0.3333333333333333703, 0.3333333333333333703),
 ( 0.3333333333333333703, 0.3333333333333333703),
 ( 1.000000000000000000, 1.000000000000000000) ) ) 
 REPRESENTATION_ITEM ( '' )  SURFACE ( )  );
#21267=EDGE_LOOP ( 'NONE', ( #46399, #12022, #12539, #1262, #46101 ) ) ;
#21275=EDGE_CURVE ( 'NONE', #26071, #2695, #43342, .T. ) ;
#21277=ORIENTED_EDGE ( 'NONE', *, *, #28283, .T. ) ;
#21279=CARTESIAN_POINT ( 'NONE',  ( -11.02112013093993426, -11.00071374030268778, 60.77911540634885768 ) ) ;
#21280=DIRECTION ( 'NONE',  ( 3.549360974554993999E-17, -6.371834667797928663E-18, -1.000000000000000000 ) ) ;
#21281=ORIENTED_EDGE ( 'NONE', *, *, #31918, .T. ) ;
#21282=CARTESIAN_POINT ( 'NONE',  ( -17.96252028288565228, -22.23973478741342902, 61.97512300109620043 ) ) ;
#21287=EDGE_CURVE ( 'NONE', #9616, #30534, #24290, .T. ) ;
#21288=CARTESIAN_POINT ( 'NONE',  ( -10.40860991809309155, -15.50898095412354571, 57.85320721669017985 ) ) ;
#21289=ORIENTED_EDGE ( 'NONE', *, *, #19393, .F. ) ;
#21290=CARTESIAN_POINT ( 'NONE',  ( -10.76458884141051975, -11.46785096862322995, 71.27516169247240896 ) ) ;
#21292=CARTESIAN_POINT ( 'NONE',  ( -24.45563843384471880, -14.25946414430215903, 73.53760260359439371 ) ) ;
#21296=CARTESIAN_POINT ( 'NONE',  ( -24.69519500507366061, -13.18560008479083123, 59.52301243476822634 ) ) ;
#21298=CARTESIAN_POINT ( 'NONE',  ( -13.33011785382929304, -9.069340661520646663, 63.92418669539090814 ) ) ;
#21299=CARTESIAN_POINT ( 'NONE',  ( -11.24165692237015968, -11.41328057087977044, 60.67885513026408262 ) ) ;
#21300=DIRECTION ( 'NONE',  ( 0.3163880819683242973, 0.8528035521334695890, -0.4154812667942338611 ) ) ;
#21308=CARTESIAN_POINT ( 'NONE',  ( -23.49605051889219709, -11.22618518380361152, 73.37665428612797314 ) ) ;
#21310=CARTESIAN_POINT ( 'NONE',  ( -9.999902751509219812, -15.43079746462003854, 57.72939317863753672 ) ) ;
#21311=B_SPLINE_CURVE_WITH_KNOTS ( 'NONE', 3,
 ( #36463, #14286, #32778, #36688, #18237, #29092, #40649, #6928, #33244, #36945 ),
 .UNSPECIFIED., .F., .F.,
 ( 4, 2, 2, 2, 4 ),
 ( 0.6272669072878210850, 0.7522669073073205981, 0.8772669073268200002, 1.002266907346319513, 1.127266907365819026 ),
 .UNSPECIFIED. ) ;
#21313=B_SPLINE_CURVE_WITH_KNOTS ( 'NONE', 3,
 ( #15302, #37969, #34268, #23216, #37470, #46100, #19265, #30369, #34770, #41921 ),
 .UNSPECIFIED., .F., .F.,
 ( 4, 2, 2, 2, 4 ),
 ( 0.6272669072877787855, 0.7522669073072940638, 0.8772669073268094531, 1.002266907346324842, 1.127266907365840121 ),
 .UNSPECIFIED. ) ;
#21315=B_SPLINE_CURVE_WITH_KNOTS ( 'NONE', 1,
 ( #1725, #35440 ),
 .UNSPECIFIED., .F., .F.,
 ( 2, 2 ),
 ( 0.000000000000000000, 1.000000000000000000 ),
 .UNSPECIFIED. ) ;
#21317=ORIENTED_EDGE ( 'NONE', *, *, #36915, .F. ) ;
#21319=ORIENTED_EDGE ( 'NONE', *, *, #43765, .F. ) ;
#21320=VECTOR ( 'NONE', #34412, 1000.000000000000000 ) ;
#21321=DIRECTION ( 'NONE',  ( -5.731567514496413899E-31, -1.020425574103664789E-16, -1.000000000000000000 ) ) ;
#21322=CARTESIAN_POINT ( 'NONE',  ( -12.91491141960329792, -8.878583893719202536, 67.51909449892792736 ) ) ;
#21324=CARTESIAN_POINT ( 'NONE',  ( -12.70616753690738143, -9.559812705026583757, 71.00492334522255078 ) ) ;
#21329=CARTESIAN_POINT ( 'NONE',  ( -11.42622172434740158, -18.51434208396348069, 61.42710833180511543 ) ) ;
#21330=EDGE_CURVE ( 'NONE', #39625, #47942, #9846, .T. ) ;
#21334=CARTESIAN_POINT ( 'NONE',  ( -10.99373011207215356, -17.70814896605071809, 68.30541983026010655 ) ) ;
#21335=CARTESIAN_POINT ( 'NONE',  ( -24.87387917185663966, -14.87237230681592948, 59.35026067257155802 ) ) ;
#21336=( BOUNDED_CURVE ( )  B_SPLINE_CURVE ( 3, ( #22901, #4184, #14979, #19679 ),
 .UNSPECIFIED., .F., .F. ) 
 B_SPLINE_CURVE_WITH_KNOTS ( ( 4, 4 ),
 ( 0.000000000000000000, 0.4074455897393624015 ),
 .UNSPECIFIED. ) 
 CURVE ( )  GEOMETRIC_REPRESENTATION_ITEM ( )  RATIONAL_B_SPLINE_CURVE ( ( 1.000000000000000000, 0.4567392136813315240, 0.3561768502900301003, 0.6983129098260958401 ) ) 
 REPRESENTATION_ITEM ( '' )  );
#21337=ORIENTED_EDGE ( 'NONE', *, *, #48209, .T. ) ;
#21339=EDGE_LOOP ( 'NONE', ( #33532, #39445 ) ) ;
#21341=CARTESIAN_POINT ( 'NONE',  ( -10.52215064345839757, -13.37195933026064232, 74.82817647370434599 ) ) ;
#21342=CARTESIAN_POINT ( 'NONE',  ( -16.28288173181390874, -21.71561457058961153, 58.30087945820258000 ) ) ;
#21343=CARTESIAN_POINT ( 'NONE',  ( -18.59285626271963210, -7.848678033734123538, 67.05638626395584367 ) ) ;
#21344=ADVANCED_FACE ( 'NONE', ( #7412 ), #29305, .T. ) ;
#21347=FACE_OUTER_BOUND ( 'NONE', #2497, .T. ) ;
#21348=EDGE_CURVE ( 'NONE', #25, #10344, #37162, .T. ) ;
#21349=CARTESIAN_POINT ( 'NONE',  ( -18.46410521509267610, -21.78222384695268588, 72.29070755221093236 ) ) ;
#21354=CARTESIAN_POINT ( 'NONE',  ( -10.68602809008750576, -16.88409676349039046, 57.70232650191087487 ) ) ;
#21355=ORIENTED_EDGE ( 'NONE', *, *, #43624, .F. ) ;
#21356=CARTESIAN_POINT ( 'NONE',  ( -14.93108437845038594, -21.82978844404615160, 65.36242591972883531 ) ) ;
#21357=CARTESIAN_POINT ( 'NONE',  ( -9.982716954774490503, -14.44908413001617298, 67.97304700561097945 ) ) ;
#21358=ORIENTED_EDGE ( 'NONE', *, *, #6947, .T. ) ;
#21359=CARTESIAN_POINT ( 'NONE',  ( -12.69763806180496601, -20.04058448603118592, 68.62185382311069759 ) ) ;
#21360=CARTESIAN_POINT ( 'NONE',  ( -24.66206412712445939, -13.04441865846056103, 62.93289937805066359 ) ) ;
#21361=CARTESIAN_POINT ( 'NONE',  ( -13.24261710015883864, -8.643249176123326549, 60.55454998173587455 ) ) ;
#21362=CARTESIAN_POINT ( 'NONE',  ( -22.73036010286993047, -10.24127059135640039, 70.12251572578897196 ) ) ;
#21363=EDGE_LOOP ( 'NONE', ( #31022, #15012, #11255, #31259, #25042 ) ) ;
#21364=CARTESIAN_POINT ( 'NONE',  ( -22.01903099019451560, -9.527854123353398208, 60.00554641628053076 ) ) ;
#21365=VECTOR ( 'NONE', #16522, 1000.000000000000000 ) ;
#21367=CARTESIAN_POINT ( 'NONE',  ( -16.58751095051766455, -21.80939428823196025, 65.22564390318969174 ) ) ;
#21368=CARTESIAN_POINT ( 'NONE',  ( -21.55883939963115026, -8.611815437115641458, 73.78624134823098757 ) ) ;
#21369=VERTEX_POINT ( 'NONE', #22666 ) ;
#21371=CARTESIAN_POINT ( 'NONE',  ( -12.32158608955787393, -9.943909642237139579, 60.57390139315987909 ) ) ;
#21373=VERTEX_POINT ( 'NONE', #10606 ) ;
#21375=CARTESIAN_POINT ( 'NONE',  ( -14.62110356098912511, -21.71197821782932991, 58.32651279851500448 ) ) ;
#21377=CARTESIAN_POINT ( 'NONE',  ( -13.21599742097365038, -20.46930908964682416, 58.46138952334620598 ) ) ;
#21378=CARTESIAN_POINT ( 'NONE',  ( -23.83043773139750243, -11.86620498678314561, 59.78235732590890450 ) ) ;
#21379=CARTESIAN_POINT ( 'NONE',  ( -19.41926759185595586, -7.631331631424885131, 60.16104200576716465 ) ) ;
#21380=CARTESIAN_POINT ( 'NONE',  ( -21.20288680779426116, -21.22975277188588805, 65.68479702206012405 ) ) ;
#21381=CARTESIAN_POINT ( 'NONE',  ( -12.45682740369385044, -20.36257741321750103, 68.45002181329043367 ) ) ;
#21382=CARTESIAN_POINT ( 'NONE',  ( -20.31413516131974362, -8.378470924821744603, 67.06632013881642251 ) ) ;
#21383=EDGE_LOOP ( 'NONE', ( #19729, #13705 ) ) ;
#21384=ORIENTED_EDGE ( 'NONE', *, *, #43580, .F. ) ;
#21386=CARTESIAN_POINT ( 'NONE',  ( -24.81704557732260952, -15.73545128243976521, 73.18959105933400622 ) ) ;
#21387=VECTOR ( 'NONE', #44698, 1000.000000000000114 ) ;
#21389=CARTESIAN_POINT ( 'NONE',  ( -10.63632956816940300, -16.72782611610072934, 57.98760696268571024 ) ) ;
#21390=CARTESIAN_POINT ( 'NONE',  ( -12.20309422964675150, -20.12380354524033521, 64.98179449731530610 ) ) ;
#21391=CARTESIAN_POINT ( 'NONE',  ( -10.18401502636761968, -13.05277926903019470, 71.32333192088977114 ) ) ;
#21392=( BOUNDED_CURVE ( )  B_SPLINE_CURVE ( 3, ( #46284, #16211, #43062, #35179 ),
 .UNSPECIFIED., .F., .F. ) 
 B_SPLINE_CURVE_WITH_KNOTS ( ( 4, 4 ),
 ( 0.000000000000000000, 0.4074455897393596260 ),
 .UNSPECIFIED. ) 
 CURVE ( )  GEOMETRIC_REPRESENTATION_ITEM ( )  RATIONAL_B_SPLINE_CURVE ( ( 1.000000000000000000, 0.4567392136813429593, 0.3561768502900343747, 0.6983129098260744128 ) ) 
 REPRESENTATION_ITEM ( '' )  );
#21393=EDGE_CURVE ( 'NONE', #4575, #28527, #6668, .T. ) ;
#21395=VERTEX_POINT ( 'NONE', #47786 ) ;
#21396=CARTESIAN_POINT ( 'NONE',  ( -14.84927081153347039, -21.37251255130113137, 61.65072491673618771 ) ) ;
#21397=CARTESIAN_POINT ( 'NONE',  ( -23.98985609448851264, -11.28854004645977582, 66.54401757043002874 ) ) ;
#21398=CARTESIAN_POINT ( 'NONE',  ( -10.46944733747312917, -15.96661384539355133, 67.99239968927004441 ) ) ;
#21399=ORIENTED_EDGE ( 'NONE', *, *, #26052, .T. ) ;
#21400=( BOUNDED_SURFACE ( )  B_SPLINE_SURFACE ( 3, 1, ( 
 ( #18611, #33623 ),
 ( #14908, #13103 ),
 ( #43168, #31841 ),
 ( #24935, #31603 ),
 ( #10161, #32334 ),
 ( #47590, #46862 ),
 ( #21247, #20757 ) ),
 .UNSPECIFIED., .T., .F., .F. ) 
 B_SPLINE_SURFACE_WITH_KNOTS ( ( 4, 3, 4 ),
 ( 2, 2 ),
 ( 0.000000000000000000, 0.5000000000000000000, 1.000000000000000000 ),
 ( 0.000000000000000000, 1.000000000000000000 ),
 .UNSPECIFIED. ) 
 GEOMETRIC_REPRESENTATION_ITEM ( )  RATIONAL_B_SPLINE_SURFACE ( (
 ( 1.000000000000000000, 1.000000000000000000),
 ( 0.3333333333333335369, 0.3333333333333330373),
 ( 0.3333333333333335369, 0.3333333333333330373),
 ( 1.000000000000000000, 1.000000000000000000),
 ( 0.3333333333333333703, 0.3333333333333333703),
 ( 0.3333333333333333703, 0.3333333333333333703),
 ( 1.000000000000000000, 1.000000000000000000) ) ) 
 REPRESENTATION_ITEM ( '' )  SURFACE ( )  );
#21401=B_SPLINE_CURVE_WITH_KNOTS ( 'NONE', 3,
 ( #26677, #37737, #41435, #8698, #16051, #7732, #22747, #31090, #8212, #811 ),
 .UNSPECIFIED., .F., .F.,
 ( 4, 2, 2, 2, 4 ),
 ( 0.1272669073658901084, 0.2522669073439965937, 0.3772669073221031066, 0.5022669073002096196, 0.6272669072783161326 ),
 .UNSPECIFIED. ) ;
#21405=FACE_OUTER_BOUND ( 'NONE', #5365, .T. ) ;
#21406=EDGE_CURVE ( 'NONE', #33162, #15971, #34466, .T. ) ;
#21407=CARTESIAN_POINT ( 'NONE',  ( -20.72573862760241070, -8.580110178657996300, 60.14125250079694496 ) ) ;
#21409=CARTESIAN_POINT ( 'NONE',  ( -22.99015624685222292, -19.05428196339609315, 58.88410607238818528 ) ) ;
#21410=( BOUNDED_SURFACE ( )  B_SPLINE_SURFACE ( 3, 1, ( 
 ( #18279, #6735 ),
 ( #21749, #15069 ),
 ( #29382, #45382 ),
 ( #44414, #26180 ),
 ( #33285, #11634 ),
 ( #22738, #40457 ),
 ( #18034, #10669 ) ),
 .UNSPECIFIED., .T., .F., .F. ) 
 B_SPLINE_SURFACE_WITH_KNOTS ( ( 4, 3, 4 ),
 ( 2, 2 ),
 ( 0.000000000000000000, 0.5000000000000000000, 1.000000000000000000 ),
 ( 0.000000000000000000, 1.000000000000000000 ),
 .UNSPECIFIED. ) 
 GEOMETRIC_REPRESENTATION_ITEM ( )  RATIONAL_B_SPLINE_SURFACE ( (
 ( 1.000000000000000000, 1.000000000000000000),
 ( 0.3333333333333335369, 0.3333333333333330373),
 ( 0.3333333333333335369, 0.3333333333333330373),
 ( 1.000000000000000000, 1.000000000000000000),
 ( 0.3333333333333333703, 0.3333333333333333703),
 ( 0.3333333333333333703, 0.3333333333333333703),
 ( 1.000000000000000000, 1.000000000000000000) ) ) 
 REPRESENTATION_ITEM ( '' )  SURFACE ( )  );
#21411=ORIENTED_EDGE ( 'NONE', *, *, #4389, .T. ) ;
#21412=CARTESIAN_POINT ( 'NONE',  ( -16.06904265174829405, -7.890656434512189676, 63.82011029958098192 ) ) ;
#21414=ADVANCED_FACE ( 'NONE', ( #29555 ), #37786, .T. ) ;
#21418=VECTOR ( 'NONE', #37277, 1000.000000000000114 ) ;
#21420=CARTESIAN_POINT ( 'NONE',  ( -18.75616561686623740, -7.937006977771949856, 70.37068081711387890 ) ) ;
#21421=ADVANCED_FACE ( 'NONE', ( #20367 ), #24310, .T. ) ;
#21422=EDGE_CURVE ( 'NONE', #34511, #26563, #16159, .T. ) ;
#21426=DIRECTION ( 'NONE',  ( 0.9997277805376393323, -0.02333162706040292980, -9.101776391673710038E-09 ) ) ;
#21428=CARTESIAN_POINT ( 'NONE',  ( -10.64854695470030599, -12.86019059820356780, 64.55364013863997741 ) ) ;
#21429=DIRECTION ( 'NONE',  ( 7.357566626357555830E-06, 1.068273751274826037E-05, -0.9999999999158726283 ) ) ;
#21430=EDGE_LOOP ( 'NONE', ( #586, #16862, #20681, #7567, #11083 ) ) ;
#21432=CARTESIAN_POINT ( 'NONE',  ( -24.17067115178138081, -16.86763775777920316, 73.09156006070151079 ) ) ;
#21433=CARTESIAN_POINT ( 'NONE',  ( -24.22652117640109992, -16.69121458274543102, 59.26765574801870429 ) ) ;
#21434=VERTEX_POINT ( 'NONE', #9537 ) ;
#21435=CARTESIAN_POINT ( 'NONE',  ( -10.44250057104172669, -15.78999660075996836, 64.51331401163844248 ) ) ;
#21437=DIRECTION ( 'NONE',  ( 0.4639960340712823705, -0.8858372764600287441, 1.924356585498154222E-16 ) ) ;
#21438=CARTESIAN_POINT ( 'NONE',  ( -16.92322068952146807, -21.79132391646259848, 68.76848671744031094 ) ) ;
#21441=VERTEX_POINT ( 'NONE', #34886 ) ;
#21442=B_SPLINE_CURVE_WITH_KNOTS ( 'NONE', 1,
 ( #36075, #2356 ),
 .UNSPECIFIED., .F., .F.,
 ( 2, 2 ),
 ( 0.000000000000000000, 1.000000000000000000 ),
 .UNSPECIFIED. ) ;
#21443=CARTESIAN_POINT ( 'NONE',  ( -11.89203589379550685, -19.18525226774134396, 71.89505619424038230 ) ) ;
#21444=FACE_OUTER_BOUND ( 'NONE', #40473, .T. ) ;
#21445=CARTESIAN_POINT ( 'NONE',  ( -10.79572390357762046, -11.40795830647630282, 67.80360014157953685 ) ) ;
#21446=ADVANCED_FACE ( 'NONE', ( #31202 ), #41240, .T. ) ;
#21447=ORIENTED_EDGE ( 'NONE', *, *, #40709, .F. ) ;
#21448=VERTEX_POINT ( 'NONE', #27747 ) ;
#21449=CARTESIAN_POINT ( 'NONE',  ( -20.66570527118851786, -8.604879590079393736, 60.14125219010794154 ) ) ;
#21450=CARTESIAN_POINT ( 'NONE',  ( -10.00661911024752726, -14.11250400273905470, 61.04008521068034554 ) ) ;
#21453=ADVANCED_FACE ( 'NONE', ( #42777 ), #699, .T. ) ;
#21454=CARTESIAN_POINT ( 'NONE',  ( -16.24510065014822047, -7.452919174226901866, 60.36175022640202315 ) ) ;
#21455=CARTESIAN_POINT ( 'NONE',  ( -23.77560840941285036, -17.75199072401120404, 59.00378408732571955 ) ) ;
#21456=VERTEX_POINT ( 'NONE', #41621 ) ;
#21458=CARTESIAN_POINT ( 'NONE',  ( -12.56172001024846452, -20.45377019276184427, 71.99149100736865137 ) ) ;
#21462=CARTESIAN_POINT ( 'NONE',  ( -24.34502386579654498, -17.56683345968398768, 66.12852568699506151 ) ) ;
#21463=FACE_OUTER_BOUND ( 'NONE', #16744, .T. ) ;
#21465=CARTESIAN_POINT ( 'NONE',  ( -19.49109506855409180, -21.54969648977046148, 62.28031529404344013 ) ) ;
#21466=ORIENTED_EDGE ( 'NONE', *, *, #30189, .F. ) ;
#21467=CARTESIAN_POINT ( 'NONE',  ( -21.41609786863869758, -21.09944828077204804, 69.16111856145751347 ) ) ;
#21468=LINE ( 'NONE', #43886, #37567 ) ;
#21470=CARTESIAN_POINT ( 'NONE',  ( -15.16142571637111303, -21.90729309775286282, 68.72592917306566562 ) ) ;
#21471=ADVANCED_FACE ( 'NONE', ( #21090 ), #47195, .F. ) ;
#21472=B_SPLINE_CURVE_WITH_KNOTS ( 'NONE', 1,
 ( #13149, #43470 ),
 .UNSPECIFIED., .F., .F.,
 ( 2, 2 ),
 ( 0.000000000000000000, 1.000000000000000000 ),
 .UNSPECIFIED. ) ;
#21473=CARTESIAN_POINT ( 'NONE',  ( -24.86601949095794239, -14.46076817688473071, 66.43938638393159124 ) ) ;
#21475=CARTESIAN_POINT ( 'NONE',  ( -16.58751391467172098, -21.80939466075598077, 65.52564390317479592 ) ) ;
#21476=EDGE_LOOP ( 'NONE', ( #5820, #40011, #19992, #7421, #2874 ) ) ;
#21477=CARTESIAN_POINT ( 'NONE',  ( -23.80321465417087978, -17.81075909821204917, 59.15378417737379380 ) ) ;
#21478=CARTESIAN_POINT ( 'NONE',  ( -16.84865286310842336, -21.83598151670433296, 68.98088545748413480 ) ) ;
#21479=CARTESIAN_POINT ( 'NONE',  ( -22.68646480449111635, -20.08284195570847430, 69.35913425646373298 ) ) ;
#21480=CARTESIAN_POINT ( 'NONE',  ( -13.60236376389480384, -20.73382277062339085, 61.80174179654961364 ) ) ;
#21481=FACE_OUTER_BOUND ( 'NONE', #32258, .T. ) ;
#21483=ORIENTED_EDGE ( 'NONE', *, *, #30646, .T. ) ;
#21486=LINE ( 'NONE', #27897, #1385 ) ;
#21487=ORIENTED_EDGE ( 'NONE', *, *, #12834, .F. ) ;
#21489=CARTESIAN_POINT ( 'NONE',  ( -10.13258914451759019, -16.33817228489381179, 71.63245656337019796 ) ) ;
#21491=CARTESIAN_POINT ( 'NONE',  ( -24.19351282280050341, -13.02564333272532515, 66.58630226542909725 ) ) ;
#21492=CARTESIAN_POINT ( 'NONE',  ( -19.37484727228654080, -7.619050864103940057, 60.14588289477547534 ) ) ;
#21493=LINE ( 'NONE', #3485, #28960 ) ;
#21494=CARTESIAN_POINT ( 'NONE',  ( -12.41315146567208139, -9.850077947585075933, 57.08935532239181754 ) ) ;
#21495=EDGE_CURVE ( 'NONE', #32931, #11764, #42834, .T. ) ;
#21496=CARTESIAN_POINT ( 'NONE',  ( -12.32278866559117780, -19.67576434477648917, 61.41150688479135766 ) ) ;
#21500=CARTESIAN_POINT ( 'NONE',  ( -14.82200063897825970, -7.828394103733741005, 57.04988785029721754 ) ) ;
#21502=EDGE_CURVE ( 'NONE', #34949, #28014, #6313, .T. ) ;
#21503=ORIENTED_EDGE ( 'NONE', *, *, #7793, .T. ) ;
#21505=DIRECTION ( 'NONE',  ( -5.731567514496413899E-31, -1.020425574103664789E-16, -1.000000000000000000 ) ) ;
#21507=CARTESIAN_POINT ( 'NONE',  ( -21.02642564228531441, -20.81301427019056760, 69.16523372085018195 ) ) ;
#21509=DIRECTION ( 'NONE',  ( 0.2664710960620865765, -0.9638429098994649724, 4.833213314675752896E-08 ) ) ;
#21510=ORIENTED_EDGE ( 'NONE', *, *, #2472, .F. ) ;
#21511=ORIENTED_EDGE ( 'NONE', *, *, #23888, .F. ) ;
#21513=ORIENTED_EDGE ( 'NONE', *, *, #36711, .T. ) ;
#21514=CARTESIAN_POINT ( 'NONE',  ( -14.92898057683877155, -8.215345490092026637, 57.14440235176596161 ) ) ;
#21515=VECTOR ( 'NONE', #10390, 1000.000000000000114 ) ;
#21516=CARTESIAN_POINT ( 'NONE',  ( -11.64187585391237612, -10.11031112578646152, 67.61241562450165077 ) ) ;
#21517=B_SPLINE_CURVE_WITH_KNOTS ( 'NONE', 1,
 ( #10608, #37919 ),
 .UNSPECIFIED., .F., .F.,
 ( 2, 2 ),
 ( 0.000000000000000000, 1.000000000000000000 ),
 .UNSPECIFIED. ) ;
#21521=ORIENTED_EDGE ( 'NONE', *, *, #21741, .T. ) ;
#21522=CARTESIAN_POINT ( 'NONE',  ( -20.12289122552838094, -7.865124802246414859, 73.90591932823114973 ) ) ;
#21524=( BOUNDED_CURVE ( )  B_SPLINE_CURVE ( 3, ( #46916, #4290, #48602, #45415 ),
 .UNSPECIFIED., .F., .F. ) 
 B_SPLINE_CURVE_WITH_KNOTS ( ( 4, 4 ),
 ( 0.000000000000000000, 0.4074455897393559622 ),
 .UNSPECIFIED. ) 
 CURVE ( )  GEOMETRIC_REPRESENTATION_ITEM ( )  RATIONAL_B_SPLINE_CURVE ( ( 1.000000000000000000, 0.4567392136813420711, 0.3561768502900340416, 0.6983129098260760781 ) ) 
 REPRESENTATION_ITEM ( '' )  );
#21525=ORIENTED_EDGE ( 'NONE', *, *, #45324, .F. ) ;
#21526=DIRECTION ( 'NONE',  ( -0.3037135924646502394, 0.9527633776296274837, 2.170275161112374562E-08 ) ) ;
#21529=CARTESIAN_POINT ( 'NONE',  ( -19.64401462542318200, -21.92156298671864434, 62.10848288909245696 ) ) ;
#21530=CARTESIAN_POINT ( 'NONE',  ( -16.74780546227259848, -22.22844731805369278, 68.84560649934257981 ) ) ;
#21536=CARTESIAN_POINT ( 'NONE',  ( -24.70317136920038337, -13.22248578388119000, 59.46244285080189940 ) ) ;
#21537=VERTEX_POINT ( 'NONE', #28485 ) ;
#21538=( BOUNDED_CURVE ( )  B_SPLINE_CURVE ( 3, ( #22130, #18649, #45041, #18913 ),
 .UNSPECIFIED., .F., .F. ) 
 B_SPLINE_CURVE_WITH_KNOTS ( ( 4, 4 ),
 ( 0.9074455897393695070, 1.000000000000000000 ),
 .UNSPECIFIED. ) 
 CURVE ( )  GEOMETRIC_REPRESENTATION_ITEM ( )  RATIONAL_B_SPLINE_CURVE ( ( 0.6983129098261253720, 0.7760317562607260689, 0.8765941196520176115, 1.000000000000000000 ) ) 
 REPRESENTATION_ITEM ( '' )  );
#21539=FACE_OUTER_BOUND ( 'NONE', #41277, .T. ) ;
#21540=CARTESIAN_POINT ( 'NONE',  ( -12.00532783130394776, -19.33158900886926546, 58.07115174146640157 ) ) ;
#21541=CARTESIAN_POINT ( 'NONE',  ( -10.78898398081525301, -17.19290454168847404, 61.44271037915215317 ) ) ;
#21543=DIRECTION ( 'NONE',  ( 0.9959323210854038599, -0.09010444948746666738, -2.601165157765165743E-08 ) ) ;
#21544=CARTESIAN_POINT ( 'NONE',  ( -24.68345461824787890, -13.13130818398968103, 59.47612521039077649 ) ) ;
#21546=CARTESIAN_POINT ( 'NONE',  ( -18.48325495428488807, -7.889676674725549788, 73.84064351486135536 ) ) ;
#21548=B_SPLINE_CURVE_WITH_KNOTS ( 'NONE', 1,
 ( #13386, #42729 ),
 .UNSPECIFIED., .F., .F.,
 ( 2, 2 ),
 ( 0.000000000000000000, 1.000000000000000000 ),
 .UNSPECIFIED. ) ;
#21549=EDGE_LOOP ( 'NONE', ( #47565, #27723, #8623, #11625, #40407 ) ) ;
#21551=( BOUNDED_CURVE ( )  B_SPLINE_CURVE ( 3, ( #21475, #7428, #14761, #40183 ),
 .UNSPECIFIED., .F., .F. ) 
 B_SPLINE_CURVE_WITH_KNOTS ( ( 4, 4 ),
 ( 0.9074455897393642889, 1.000000000000000000 ),
 .UNSPECIFIED. ) 
 CURVE ( )  GEOMETRIC_REPRESENTATION_ITEM ( )  RATIONAL_B_SPLINE_CURVE ( ( 0.6983129098260967282, 0.7760317562607014219, 0.8765941196520025125, 1.000000000000000000 ) ) 
 REPRESENTATION_ITEM ( '' )  );
#21552=ORIENTED_EDGE ( 'NONE', *, *, #43261, .F. ) ;
#21553=EDGE_CURVE ( 'NONE', #20596, #15704, #34324, .T. ) ;
#21554=ADVANCED_FACE ( 'NONE', ( #13671 ), #44003, .T. ) ;
#21555=VERTEX_POINT ( 'NONE', #44242 ) ;
#21556=ORIENTED_EDGE ( 'NONE', *, *, #24334, .F. ) ;
#21557=CARTESIAN_POINT ( 'NONE',  ( -18.89230742602834923, -7.910091329180813702, 63.63909002588712127 ) ) ;
#21558=CARTESIAN_POINT ( 'NONE',  ( -12.85294938858001501, -8.926356163590522641, 67.57216919348684314 ) ) ;
#21559=DIRECTION ( 'NONE',  ( 0.7971031148784507581, -0.6038432116460916710, 6.916509187980650173E-08 ) ) ;
#21560=CARTESIAN_POINT ( 'NONE',  ( -11.89178972046640936, -10.43929686452144878, 71.11893105542935700 ) ) ;
#21561=VERTEX_POINT ( 'NONE', #25273 ) ;
#21566=B_SPLINE_CURVE_WITH_KNOTS ( 'NONE', 3,
 ( #26874, #19720, #12319, #31044, #19463, #37684, #12085, #1002, #11847, #15266 ),
 .UNSPECIFIED., .F., .F.,
 ( 4, 2, 2, 2, 4 ),
 ( 0.6272669072964546233, 0.7522669073137989715, 0.8772669073311434307, 1.002266907348487779, 1.127266907365832127 ),
 .UNSPECIFIED. ) ;
#21568=CARTESIAN_POINT ( 'NONE',  ( -12.60227155074094441, -19.95281705956671559, 68.35129494334645983 ) ) ;
#21570=ORIENTED_EDGE ( 'NONE', *, *, #24890, .T. ) ;
#21571=ADVANCED_FACE ( 'NONE', ( #13910 ), #21579, .T. ) ;
#21573=VECTOR ( 'NONE', #21426, 999.9999999999998863 ) ;
#21574=CARTESIAN_POINT ( 'NONE',  ( -24.79803955827340545, -15.87155823828966561, 69.78953433284350183 ) ) ;
#21577=B_SPLINE_CURVE_WITH_KNOTS ( 'NONE', 1,
 ( #47282, #32495 ),
 .UNSPECIFIED., .F., .F.,
 ( 2, 2 ),
 ( 0.000000000000000000, 1.000000000000000000 ),
 .UNSPECIFIED. ) ;
#21578=VERTEX_POINT ( 'NONE', #34097 ) ;
#21579=PLANE ( 'NONE',  #12699 ) ;
#21580=CARTESIAN_POINT ( 'NONE',  ( -18.17450532280264142, -21.77015438960330229, 69.04344613823298005 ) ) ;
#21581=CARTESIAN_POINT ( 'NONE',  ( -21.53227841957539113, -21.02428511524863097, 72.64729568458159292 ) ) ;
#21584=CARTESIAN_POINT ( 'NONE',  ( -23.01445215836851688, -10.50074233538543211, 66.68615203886294296 ) ) ;
#21585=CARTESIAN_POINT ( 'NONE',  ( -12.05483428091225129, -10.31798718066989551, 67.49896870046983111 ) ) ;
#21586=VERTEX_POINT ( 'NONE', #18342 ) ;
#21587=CARTESIAN_POINT ( 'NONE',  ( -20.76359895218475060, -20.96132515946565888, 58.87148521899143816 ) ) ;
#21588=CARTESIAN_POINT ( 'NONE',  ( -21.55884032038934350, -8.611816057827914150, 73.78624026056009200 ) ) ;
#21589=CARTESIAN_POINT ( 'NONE',  ( -17.42409385541300892, -14.80920654474439679, 56.49999999999994316 ) ) ;
#21590=EDGE_LOOP ( 'NONE', ( #36535, #14605, #19359, #28681 ) ) ;
#21591=CARTESIAN_POINT ( 'NONE',  ( -13.35818949714929360, -21.05197827947291955, 61.70141596610112344 ) ) ;
#21592=ORIENTED_EDGE ( 'NONE', *, *, #14205, .F. ) ;
#21593=CYLINDRICAL_SURFACE ( 'NONE', #34443, 0.1500000000000084044 ) ;
#21594=CARTESIAN_POINT ( 'NONE',  ( -24.82750195234013191, -13.97654432178796569, 73.30766915316792165 ) ) ;
#21595=CARTESIAN_POINT ( 'NONE',  ( -19.80301194551662647, -21.44571530912114099, 68.93482476707502826 ) ) ;
#21596=B_SPLINE_CURVE_WITH_KNOTS ( 'NONE', 1,
 ( #11872, #11619 ),
 .UNSPECIFIED., .F., .F.,
 ( 2, 2 ),
 ( 0.000000000000000000, 1.000000000000000000 ),
 .UNSPECIFIED. ) ;
#21597=DIRECTION ( 'NONE',  ( -0.3478314405900309603, -0.9375570856950864451, 9.567072274253697654E-17 ) ) ;
#21599=CARTESIAN_POINT ( 'NONE',  ( -10.47352321885900928, -13.96536482376412458, 61.02894424119286754 ) ) ;
#21600=CARTESIAN_POINT ( 'NONE',  ( -10.85887813628090015, -11.28619579020030628, 64.26226673522833721 ) ) ;
#21601=DIRECTION ( 'NONE',  ( -1.389773828427094234E-07, -3.718553705696926905E-07, 0.9999999999999211742 ) ) ;
#21602=ORIENTED_EDGE ( 'NONE', *, *, #47467, .F. ) ;
#21603=CARTESIAN_POINT ( 'NONE',  ( -23.80338573481879294, -11.80731802715296297, 59.76763678108634537 ) ) ;
#21604=AXIS2_PLACEMENT_3D ( 'NONE', #14641, #28735, #37308 ) ;
#21605=CARTESIAN_POINT ( 'NONE',  ( -24.77839546667076931, -16.00024531626065283, 66.18512132471579434 ) ) ;
#21606=ADVANCED_FACE ( 'NONE', ( #48636 ), #30907, .T. ) ;
#21607=EDGE_LOOP ( 'NONE', ( #17589, #42787 ) ) ;
#21608=ORIENTED_EDGE ( 'NONE', *, *, #13811, .T. ) ;
#21609=CARTESIAN_POINT ( 'NONE',  ( -14.99706723701585354, -21.85287888328288375, 65.29092001793476641 ) ) ;
#21611=FACE_OUTER_BOUND ( 'NONE', #30054, .T. ) ;
#21612=CARTESIAN_POINT ( 'NONE',  ( -21.25211362912655488, -21.20065753679924114, 65.76170813790885461 ) ) ;
#21613=CARTESIAN_POINT ( 'NONE',  ( -22.82985190038863621, -19.93574988146554006, 72.68754644230530459 ) ) ;
#21614=VERTEX_POINT ( 'NONE', #22298 ) ;
#21615=VERTEX_POINT ( 'NONE', #22803 ) ;
#21616=EDGE_CURVE ( 'NONE', #9195, #21614, #3968, .T. ) ;
#21618=ADVANCED_FACE ( 'NONE', ( #14876 ), #29938, .T. ) ;
#21619=CARTESIAN_POINT ( 'NONE',  ( -19.95259202802825271, -8.281694549620906898, 73.72096610892648982 ) ) ;
#21620=CYLINDRICAL_SURFACE ( 'NONE', #39380, 0.1499999999999994948 ) ;
#21622=( BOUNDED_SURFACE ( )  B_SPLINE_SURFACE ( 3, 1, ( 
 ( #13150, #23941 ),
 ( #46349, #4486 ),
 ( #38945, #16526 ),
 ( #31561, #9404 ),
 ( #28104, #31804 ),
 ( #46596, #16765 ),
 ( #1767, #27379 ) ),
 .UNSPECIFIED., .T., .F., .F. ) 
 B_SPLINE_SURFACE_WITH_KNOTS ( ( 4, 3, 4 ),
 ( 2, 2 ),
 ( 0.000000000000000000, 0.5000000000000000000, 1.000000000000000000 ),
 ( 0.000000000000000000, 1.000000000000000000 ),
 .UNSPECIFIED. ) 
 GEOMETRIC_REPRESENTATION_ITEM ( )  RATIONAL_B_SPLINE_SURFACE ( (
 ( 1.000000000000000000, 1.000000000000000000),
 ( 0.3333333333333335369, 0.3333333333333330373),
 ( 0.3333333333333335369, 0.3333333333333330373),
 ( 1.000000000000000000, 1.000000000000000000),
 ( 0.3333333333333333703, 0.3333333333333333703),
 ( 0.3333333333333333703, 0.3333333333333333703),
 ( 1.000000000000000000, 1.000000000000000000) ) ) 
 REPRESENTATION_ITEM ( '' )  SURFACE ( )  );
#21623=CARTESIAN_POINT ( 'NONE',  ( -18.55266926790839221, -7.445060760019332591, 73.96251610088971518 ) ) ;
#21625=VERTEX_POINT ( 'NONE', #153 ) ;
#21628=CARTESIAN_POINT ( 'NONE',  ( -24.35164181862008803, -15.81450316290537650, 69.53307533821916309 ) ) ;
#21629=CARTESIAN_POINT ( 'NONE',  ( -23.98651520682892624, -11.28222280472095029, 66.56068001652479893 ) ) ;
#21632=VECTOR ( 'NONE', #30714, 1000.000000000000114 ) ;
#21633=CARTESIAN_POINT ( 'NONE',  ( -10.57458500277835434, -16.25348641136583083, 71.44750329828485746 ) ) ;
#21634=CARTESIAN_POINT ( 'NONE',  ( -10.76785811675247118, -12.48515291162924434, 57.61385273545094066 ) ) ;
#21635=AXIS2_PLACEMENT_3D ( 'NONE', #34736, #27347, #39152 ) ;
#21637=CARTESIAN_POINT ( 'NONE',  ( -20.92788686586858660, -8.687255892883298358, 60.14125422863671844 ) ) ;
#21639=PLANE ( 'NONE',  #13374 ) ;
#21640=ORIENTED_EDGE ( 'NONE', *, *, #26514, .F. ) ;
#21642=CARTESIAN_POINT ( 'NONE',  ( -17.61324970268224277, -7.361601100360097405, 63.75068226507995917 ) ) ;
#21643=ORIENTED_EDGE ( 'NONE', *, *, #10028, .F. ) ;
#21645=CARTESIAN_POINT ( 'NONE',  ( -12.50776718604994109, -20.40684089597385764, 71.92158360616595303 ) ) ;
#21647=CARTESIAN_POINT ( 'NONE',  ( -21.36489517220793743, -8.963474395264050543, 73.75128753236120360 ) ) ;
#21649=CARTESIAN_POINT ( 'NONE',  ( -19.93475561761363934, -21.40553454266635569, 65.62053285436006433 ) ) ;
#21650=CARTESIAN_POINT ( 'NONE',  ( -23.96159466281891071, -11.23502865522796768, 70.07866094266108803 ) ) ;
#21653=PLANE ( 'NONE',  #32217 ) ;
#21656=VERTEX_POINT ( 'NONE', #30191 ) ;
#21657=CARTESIAN_POINT ( 'NONE',  ( -22.92161870814259217, -14.39064228688693170, 53.88362224778187226 ) ) ;
#21658=CARTESIAN_POINT ( 'NONE',  ( -23.00442008925061899, -19.11762375203660724, 59.18410642057862248 ) ) ;
#21659=ORIENTED_EDGE ( 'NONE', *, *, #37931, .T. ) ;
#21662=CARTESIAN_POINT ( 'NONE',  ( -22.96375064570672819, -10.44813988596692411, 63.08658113699938497 ) ) ;
#21663=( BOUNDED_CURVE ( )  B_SPLINE_CURVE ( 3, ( #45686, #45918, #4538, #26958 ),
 .UNSPECIFIED., .F., .F. ) 
 B_SPLINE_CURVE_WITH_KNOTS ( ( 4, 4 ),
 ( 0.9074455897393651771, 1.000000000000000000 ),
 .UNSPECIFIED. ) 
 CURVE ( )  GEOMETRIC_REPRESENTATION_ITEM ( )  RATIONAL_B_SPLINE_CURVE ( ( 0.6983129098260874024, 0.7760317562606933173, 0.8765941196519975165, 1.000000000000000000 ) ) 
 REPRESENTATION_ITEM ( '' )  );
#21664=CARTESIAN_POINT ( 'NONE',  ( -13.99679447977218061, -20.97040113148658591, 71.94079819673058296 ) ) ;
#21665=B_SPLINE_CURVE_WITH_KNOTS ( 'NONE', 3,
 ( #4764, #7746, #41706, #345, #19532, #11914, #11659, #41448, #33810, #26439 ),
 .UNSPECIFIED., .F., .F.,
 ( 4, 2, 2, 2, 4 ),
 ( 0.1272669073657870520, 0.2522669073463000844, 0.3772669073268131168, 0.5022669073073261492, 0.6272669072878391816 ),
 .UNSPECIFIED. ) ;
#21666=CARTESIAN_POINT ( 'NONE',  ( -23.69549191163005020, -18.83074896771919526, 69.40033652239984008 ) ) ;
#21667=CARTESIAN_POINT ( 'NONE',  ( -14.74956223559871482, -8.338905777109427930, 64.01808618867474365 ) ) ;
#21668=VECTOR ( 'NONE', #38750, 1000.000000000000114 ) ;
#21669=VERTEX_POINT ( 'NONE', #26235 ) ;
#21670=CARTESIAN_POINT ( 'NONE',  ( -10.57110082969170683, -13.38215148069720861, 74.67817647591368768 ) ) ;
#21671=FACE_OUTER_BOUND ( 'NONE', #40184, .T. ) ;
#21672=ADVANCED_FACE ( 'NONE', ( #25999 ), #47859, .T. ) ;
#21673=DIRECTION ( 'NONE',  ( -0.03181436478788691319, -0.9994937949748079475, -6.982004198809111150E-09 ) ) ;
#21674=DIRECTION ( 'NONE',  ( 0.8967515337576290602, -0.4425343904188011046, 9.546469656967254525E-09 ) ) ;
#21675=ADVANCED_FACE ( 'NONE', ( #46419 ), #870, .F. ) ;
#21676=( BOUNDED_SURFACE ( )  B_SPLINE_SURFACE ( 3, 1, ( 
 ( #14890, #37550 ),
 ( #10989, #7057 ),
 ( #22555, #25514 ),
 ( #48403, #41509 ),
 ( #18355, #33360 ),
 ( #21820, #47929 ),
 ( #18860, #29953 ) ),
 .UNSPECIFIED., .T., .F., .F. ) 
 B_SPLINE_SURFACE_WITH_KNOTS ( ( 4, 3, 4 ),
 ( 2, 2 ),
 ( 0.000000000000000000, 0.5000000000000000000, 1.000000000000000000 ),
 ( 0.000000000000000000, 1.000000000000000000 ),
 .UNSPECIFIED. ) 
 GEOMETRIC_REPRESENTATION_ITEM ( )  RATIONAL_B_SPLINE_SURFACE ( (
 ( 1.000000000000000000, 1.000000000000000000),
 ( 0.3333333333333335369, 0.3333333333333330373),
 ( 0.3333333333333335369, 0.3333333333333330373),
 ( 1.000000000000000000, 1.000000000000000000),
 ( 0.3333333333333333703, 0.3333333333333333703),
 ( 0.3333333333333333703, 0.3333333333333333703),
 ( 1.000000000000000000, 1.000000000000000000) ) ) 
 REPRESENTATION_ITEM ( '' )  SURFACE ( )  );
#21677=ORIENTED_EDGE ( 'NONE', *, *, #23518, .T. ) ;
#21678=EDGE_CURVE ( 'NONE', #43576, #35243, #30408, .T. ) ;
#21679=EDGE_LOOP ( 'NONE', ( #21748, #23972, #45062, #45384, #8785 ) ) ;
#21680=DIRECTION ( 'NONE',  ( -1.389773828427094234E-07, -3.718553705696926905E-07, 0.9999999999999211742 ) ) ;
#21681=CARTESIAN_POINT ( 'NONE',  ( -23.34754611528896362, -19.32773447048098348, 59.06127517204052424 ) ) ;
#21682=DIRECTION ( 'NONE',  ( -0.9640890753730593232, 0.2655790932026005358, -6.310348464816974292E-08 ) ) ;
#21683=ADVANCED_FACE ( 'NONE', ( #23527 ), #38527, .T. ) ;
#21685=CARTESIAN_POINT ( 'NONE',  ( -12.64995486802317082, -19.99670083032576429, 68.33657438322859434 ) ) ;
#21686=CARTESIAN_POINT ( 'NONE',  ( -11.22844613476422460, -11.44458948612160043, 64.43409918096024569 ) ) ;
#21687=VERTEX_POINT ( 'NONE', #38265 ) ;
#21688=CARTESIAN_POINT ( 'NONE',  ( -13.64505908608012064, -21.22973791158431922, 68.63437918312371266 ) ) ;
#21689=CARTESIAN_POINT ( 'NONE',  ( -19.71455631245729379, -21.89842510487585869, 65.65824520983085222 ) ) ;
#21690=CARTESIAN_POINT ( 'NONE',  ( -23.33670675297031849, -10.27651039223464657, 59.72390641345293716 ) ) ;
#21691=VERTEX_POINT ( 'NONE', #13136 ) ;
#21694=ORIENTED_EDGE ( 'NONE', *, *, #21011, .T. ) ;
#21695=CARTESIAN_POINT ( 'NONE',  ( -10.44881481234349252, -17.42631575494719698, 64.74243950200344955 ) ) ;
#21696=CARTESIAN_POINT ( 'NONE',  ( -19.35593647574418341, -21.53741737806316792, 58.59795352067202145 ) ) ;
#21697=EDGE_LOOP ( 'NONE', ( #1760, #3407, #1341, #33593, #25023 ) ) ;
#21698=CARTESIAN_POINT ( 'NONE',  ( -24.43416774132473890, -14.02670544446237422, 69.86095212020217105 ) ) ;
#21699=CARTESIAN_POINT ( 'NONE',  ( -23.41616298382994898, -18.52428493080399008, 72.77840375779385340 ) ) ;
#21701=CARTESIAN_POINT ( 'NONE',  ( -10.80042129562301589, -17.07348610811987299, 57.87863715479691251 ) ) ;
#21703=CARTESIAN_POINT ( 'NONE',  ( -24.16575310113231367, -12.74704012323608104, 70.07243002239954421 ) ) ;
#21705=CARTESIAN_POINT ( 'NONE',  ( -10.06050713658121154, -13.29172449529390398, 53.76227901944321985 ) ) ;
#21707=CARTESIAN_POINT ( 'NONE',  ( -22.93618324136711450, -9.797101482063153455, 70.13365771114293068 ) ) ;
#21708=CARTESIAN_POINT ( 'NONE',  ( -13.14412777716299274, -20.90712260751159590, 58.14675838192486879 ) ) ;
#21712=VERTEX_POINT ( 'NONE', #35559 ) ;
#21713=CARTESIAN_POINT ( 'NONE',  ( -23.49945856589985027, -11.21686614839013885, 66.57781614479455357 ) ) ;
#21715=ORIENTED_EDGE ( 'NONE', *, *, #40332, .T. ) ;
#21716=CARTESIAN_POINT ( 'NONE',  ( -15.41904748403203484, -7.634001509309876532, 74.19490257054667381 ) ) ;
#21719=CARTESIAN_POINT ( 'NONE',  ( -15.69021238316472022, -21.64649376854531226, 72.04575306413649116 ) ) ;
#21720=CARTESIAN_POINT ( 'NONE',  ( -22.17046091269999764, -9.065891900838490614, 59.83515915777798710 ) ) ;
#21721=CARTESIAN_POINT ( 'NONE',  ( -24.71344798646422802, -16.35160113208834431, 62.77984073303771595 ) ) ;
#21723=CARTESIAN_POINT ( 'NONE',  ( -11.13733870171179596, -11.61806121328042174, 67.90392505421056057 ) ) ;
#21724=CYLINDRICAL_SURFACE ( 'NONE', #418, 0.1500000000000045464 ) ;
#21725=( BOUNDED_CURVE ( )  B_SPLINE_CURVE ( 3, ( #37361, #44130, #8097, #33664 ),
 .UNSPECIFIED., .F., .F. ) 
 B_SPLINE_CURVE_WITH_KNOTS ( ( 4, 4 ),
 ( 0.5000000000000000000, 0.9074455897393660653 ),
 .UNSPECIFIED. ) 
 CURVE ( )  GEOMETRIC_REPRESENTATION_ITEM ( )  RATIONAL_B_SPLINE_CURVE ( ( 1.000000000000010214, 0.4567392136813359649, 0.3561768502900245492, 0.6983129098260869583 ) ) 
 REPRESENTATION_ITEM ( '' )  );
#21726=CARTESIAN_POINT ( 'NONE',  ( -11.68335768792166185, -18.81469630946190819, 68.51689631952916670 ) ) ;
#21728=CARTESIAN_POINT ( 'NONE',  ( -10.78031428196279329, -11.32923628920978310, 54.27966884056655061 ) ) ;
#21729=CARTESIAN_POINT ( 'NONE',  ( -11.60882265867669538, -10.15221075964790742, 71.13039628648064649 ) ) ;
#21730=EDGE_CURVE ( 'NONE', #48127, #44738, #15108, .T. ) ;
#21731=CARTESIAN_POINT ( 'NONE',  ( -11.16720068213728467, -11.56054720508597455, 67.76864607954532005 ) ) ;
#21732=CARTESIAN_POINT ( 'NONE',  ( -24.57849813159777597, -12.72878314728456850, 66.41591366067137869 ) ) ;
#21733=CARTESIAN_POINT ( 'NONE',  ( -10.73412848974934874, -11.53077067998621175, 71.20365450754333381 ) ) ;
#21734=DIRECTION ( 'NONE',  ( 0.8547111024021490921, 0.5191039697695417621, 7.472447835916433805E-08 ) ) ;
#21735=ORIENTED_EDGE ( 'NONE', *, *, #27398, .T. ) ;
#21736=VECTOR ( 'NONE', #11568, 1000.000000000000000 ) ;
#21737=EDGE_LOOP ( 'NONE', ( #32882, #30417, #5672, #34936 ) ) ;
#21738=VECTOR ( 'NONE', #12006, 999.9999999999998863 ) ;
#21740=B_SPLINE_CURVE_WITH_KNOTS ( 'NONE', 3,
 ( #4780, #9205, #42455, #26945, #16077, #41965, #24226, #8470, #8726, #31119 ),
 .UNSPECIFIED., .F., .F.,
 ( 4, 2, 2, 2, 4 ),
 ( 0.1272669073658330707, 0.2522669073463126299, 0.3772669073267921336, 0.5022669073072716373, 0.6272669072877512519 ),
 .UNSPECIFIED. ) ;
#21741=EDGE_CURVE ( 'NONE', #25935, #38842, #29257, .T. ) ;
#21743=CARTESIAN_POINT ( 'NONE',  ( -17.40971054907340942, -7.359207646686905413, 67.12065337040019131 ) ) ;
#21744=FACE_OUTER_BOUND ( 'NONE', #36876, .T. ) ;
#21746=CARTESIAN_POINT ( 'NONE',  ( -15.42638489646220279, -7.631913115121209401, 74.20268781468831776 ) ) ;
#21747=CARTESIAN_POINT ( 'NONE',  ( -9.975073501874963000, -14.93475060744560245, 74.84132960708070925 ) ) ;
#21748=ORIENTED_EDGE ( 'NONE', *, *, #29922, .T. ) ;
#21749=CARTESIAN_POINT ( 'NONE',  ( -13.99854101903132531, -20.98015058628177698, 65.14195714266269022 ) ) ;
#21750=CARTESIAN_POINT ( 'NONE',  ( -20.94265863490610258, -21.37680627582274795, 62.30126734817043399 ) ) ;
#21751=ORIENTED_EDGE ( 'NONE', *, *, #12269, .F. ) ;
#21752=LINE ( 'NONE', #39742, #44635 ) ;
#21753=EDGE_CURVE ( 'NONE', #3004, #37170, #43929, .T. ) ;
#21754=CARTESIAN_POINT ( 'NONE',  ( -12.73047692465080338, -11.91646811004319062, 53.88362224778186516 ) ) ;
#21755=EDGE_CURVE ( 'NONE', #21199, #18877, #4158, .T. ) ;
#21756=EDGE_LOOP ( 'NONE', ( #38523, #36831, #36196, #32397, #44490 ) ) ;
#21757=CARTESIAN_POINT ( 'NONE',  ( -23.32045150837215175, -18.68837265512984303, 62.50973769122266788 ) ) ;
#21759=CARTESIAN_POINT ( 'NONE',  ( -23.34189317711797429, -10.28335673940103590, 59.64557479084083269 ) ) ;
#21760=EDGE_CURVE ( 'NONE', #44791, #8067, #39797, .T. ) ;
#21762=CARTESIAN_POINT ( 'NONE',  ( -10.73412800634210029, -11.53077167852495677, 71.20365559628196195 ) ) ;
#21763=CARTESIAN_POINT ( 'NONE',  ( -12.05615918852498680, -19.97535170061420828, 61.51183199568394144 ) ) ;
#21764=CARTESIAN_POINT ( 'NONE',  ( -24.32852063849251323, -13.38246526728995001, 59.37740068604990995 ) ) ;
#21768=CARTESIAN_POINT ( 'NONE',  ( -15.34011657121100924, -21.49348207936204247, 72.23502552990838410 ) ) ;
#21769=AXIS2_PLACEMENT_3D ( 'NONE', #6161, #48236, #43603 ) ;
#21771=CARTESIAN_POINT ( 'NONE',  ( -11.73296596577226936, -10.64774513788296240, 74.72412863062541533 ) ) ;
#21772=CARTESIAN_POINT ( 'NONE',  ( -16.98902004117856990, -21.84877635801032270, 68.58071880800348197 ) ) ;
#21773=CARTESIAN_POINT ( 'NONE',  ( -24.30112618867181240, -13.25578303422174997, 59.64795780745660636 ) ) ;
#21774=ORIENTED_EDGE ( 'NONE', *, *, #6369, .F. ) ;
#21775=CARTESIAN_POINT ( 'NONE',  ( -10.67361454459859260, -12.95690279139224188, 64.45939287679182428 ) ) ;
#21777=LINE ( 'NONE', #36763, #7042 ) ;
#21778=EDGE_LOOP ( 'NONE', ( #46017, #45874, #44421, #26448, #3722 ) ) ;
#21781=EDGE_LOOP ( 'NONE', ( #45819, #13160 ) ) ;
#21782=ORIENTED_EDGE ( 'NONE', *, *, #43370, .T. ) ;
#21783=FACE_OUTER_BOUND ( 'NONE', #3396, .T. ) ;
#21785=CARTESIAN_POINT ( 'NONE',  ( -12.68532353738824803, -9.060482037740600347, 71.03420644255490402 ) ) ;
#21786=EDGE_LOOP ( 'NONE', ( #443, #3101, #24872, #23932, #36380 ) ) ;
#21787=ORIENTED_EDGE ( 'NONE', *, *, #26409, .F. ) ;
#21789=ADVANCED_FACE ( 'NONE', ( #8498 ), #11336, .T. ) ;
#21791=CARTESIAN_POINT ( 'NONE',  ( -23.44879792247470007, -11.14072156699261207, 69.89210571255328830 ) ) ;
#21792=( BOUNDED_SURFACE ( )  B_SPLINE_SURFACE ( 3, 1, ( 
 ( #23755, #23256 ),
 ( #46639, #27910 ),
 ( #12166, #9208 ),
 ( #1810, #24231 ),
 ( #16081, #27185 ),
 ( #39234, #35537 ),
 ( #31121, #13112 ) ),
 .UNSPECIFIED., .T., .F., .F. ) 
 B_SPLINE_SURFACE_WITH_KNOTS ( ( 4, 3, 4 ),
 ( 2, 2 ),
 ( 0.000000000000000000, 0.5000000000000000000, 1.000000000000000000 ),
 ( 0.000000000000000000, 1.000000000000000000 ),
 .UNSPECIFIED. ) 
 GEOMETRIC_REPRESENTATION_ITEM ( )  RATIONAL_B_SPLINE_SURFACE ( (
 ( 1.000000000000000000, 1.000000000000000000),
 ( 0.3333333333333335369, 0.3333333333333330373),
 ( 0.3333333333333335369, 0.3333333333333330373),
 ( 1.000000000000000000, 1.000000000000000000),
 ( 0.3333333333333333703, 0.3333333333333333703),
 ( 0.3333333333333333703, 0.3333333333333333703),
 ( 1.000000000000000000, 1.000000000000000000) ) ) 
 REPRESENTATION_ITEM ( '' )  SURFACE ( )  );
#21796=VERTEX_POINT ( 'NONE', #6508 ) ;
#21797=CARTESIAN_POINT ( 'NONE',  ( -24.37451731887211892, -15.64135521309706967, 69.75980740431705840 ) ) ;
#21798=CARTESIAN_POINT ( 'NONE',  ( -24.45288365649568618, -15.45035942066159862, 69.68874360283344060 ) ) ;
#21799=AXIS2_PLACEMENT_3D ( 'NONE', #14564, #22742, #4026 ) ;
#21800=CARTESIAN_POINT ( 'NONE',  ( -21.32695110138281791, -8.937895085234787373, 73.89568928637402223 ) ) ;
#21802=( BOUNDED_CURVE ( )  B_SPLINE_CURVE ( 3, ( #15033, #44157, #30095, #40909 ),
 .UNSPECIFIED., .F., .F. ) 
 B_SPLINE_CURVE_WITH_KNOTS ( ( 4, 4 ),
 ( 0.000000000000000000, 0.4074455897393631787 ),
 .UNSPECIFIED. ) 
 CURVE ( )  GEOMETRIC_REPRESENTATION_ITEM ( )  RATIONAL_B_SPLINE_CURVE ( ( 1.000000000000000000, 0.4567392136813362979, 0.3561768502900319322, 0.6983129098260868473 ) ) 
 REPRESENTATION_ITEM ( '' )  );
#21803=DIRECTION ( 'NONE',  ( 1.896855589267346620E-06, 2.136244919385519396E-06, 0.9999999999959191532 ) ) ;
#21804=( BOUNDED_CURVE ( )  B_SPLINE_CURVE ( 3, ( #47261, #32704, #17193, #31993 ),
 .UNSPECIFIED., .F., .F. ) 
 B_SPLINE_CURVE_WITH_KNOTS ( ( 4, 4 ),
 ( 0.9074455897393587378, 1.000000000000000000 ),
 .UNSPECIFIED. ) 
 CURVE ( )  GEOMETRIC_REPRESENTATION_ITEM ( )  RATIONAL_B_SPLINE_CURVE ( ( 0.6983129098260755230, 0.7760317562606831032, 0.8765941196519912992, 1.000000000000000000 ) ) 
 REPRESENTATION_ITEM ( '' )  );
#21806=ORIENTED_EDGE ( 'NONE', *, *, #38120, .F. ) ;
#21808=CARTESIAN_POINT ( 'NONE',  ( -10.11684863658992839, -16.26127201416540302, 71.62563171993747346 ) ) ;
#21809=EDGE_CURVE ( 'NONE', #39260, #8618, #9286, .T. ) ;
#21812=CARTESIAN_POINT ( 'NONE',  ( -21.52668677937081299, -21.02802818395438322, 72.66413103959850162 ) ) ;
#21813=ORIENTED_EDGE ( 'NONE', *, *, #8380, .T. ) ;
#21814=CARTESIAN_POINT ( 'NONE',  ( -22.82568502052561499, -19.94010355682323166, 72.83674718307834439 ) ) ;
#21815=DIRECTION ( 'NONE',  ( 5.517078692044801135E-07, 1.257343604232908019E-06, 0.9999999999990574207 ) ) ;
#21816=CARTESIAN_POINT ( 'NONE',  ( -21.52726120556258849, -9.076273861542912158, 70.28132538914752558 ) ) ;
#21818=CARTESIAN_POINT ( 'NONE',  ( -20.71231197388234690, -20.98888764657868578, 58.65977609787367442 ) ) ;
#21820=CARTESIAN_POINT ( 'NONE',  ( -18.92901792560347829, -7.918630368440815026, 70.78556921992733919 ) ) ;
#21821=( BOUNDED_CURVE ( )  B_SPLINE_CURVE ( 3, ( #47504, #29022, #10074, #24854 ),
 .UNSPECIFIED., .F., .F. ) 
 B_SPLINE_CURVE_WITH_KNOTS ( ( 4, 4 ),
 ( 0.000000000000000000, 0.4074455897393606252 ),
 .UNSPECIFIED. ) 
 CURVE ( )  GEOMETRIC_REPRESENTATION_ITEM ( )  RATIONAL_B_SPLINE_CURVE ( ( 1.000000000000000000, 0.4567392136813354653, 0.3561768502900315991, 0.6983129098260884016 ) ) 
 REPRESENTATION_ITEM ( '' )  );
#21822=VERTEX_POINT ( 'NONE', #48102 ) ;
#21823=CARTESIAN_POINT ( 'NONE',  ( -11.72322480355222396, -10.74717599656355027, 74.62988016596645480 ) ) ;
#21824=B_SPLINE_CURVE_WITH_KNOTS ( 'NONE', 3,
 ( #10636, #25644, #40658, #19732, #45607, #34240, #5196, #4229, #8896, #45352 ),
 .UNSPECIFIED., .F., .F.,
 ( 4, 2, 2, 2, 4 ),
 ( 0.1272669073657614613, 0.2522669073462631140, 0.3772669073267648221, 0.5022669073072665302, 0.6272669072877681273 ),
 .UNSPECIFIED. ) ;
#21827=CARTESIAN_POINT ( 'NONE',  ( -13.71293330176565384, -21.26916511146244915, 68.64120417180296840 ) ) ;
#21829=CARTESIAN_POINT ( 'NONE',  ( -22.65633676998887935, -10.15891879009521581, 70.31178531762441253 ) ) ;
#21831=CARTESIAN_POINT ( 'NONE',  ( -10.46640864507116753, -14.03671221754458109, 60.93437953636007620 ) ) ;
#21832=VERTEX_POINT ( 'NONE', #43208 ) ;
#21833=CARTESIAN_POINT ( 'NONE',  ( -24.20817551436923765, -11.73026151181330512, 59.73881638530829008 ) ) ;
#21835=ORIENTED_EDGE ( 'NONE', *, *, #6461, .F. ) ;
#21838=DIRECTION ( 'NONE',  ( -0.9132646967824439299, 0.4073666574609056124, -8.344532079829881716E-09 ) ) ;
#21840=ORIENTED_EDGE ( 'NONE', *, *, #16694, .T. ) ;
#21842=CARTESIAN_POINT ( 'NONE',  ( -14.77890319739905145, -21.35274797201484276, 65.25029445929627059 ) ) ;
#21844=CARTESIAN_POINT ( 'NONE',  ( -10.15209110106313695, -13.18697342404853146, 74.86472985364514443 ) ) ;
#21845=CARTESIAN_POINT ( 'NONE',  ( -10.04084212758499994, -13.81292206000487433, 57.60971574196104683 ) ) ;
#21846=CARTESIAN_POINT ( 'NONE',  ( -14.80624607021532135, -8.317144234858641738, 60.31996281969095719 ) ) ;
#21847=CARTESIAN_POINT ( 'NONE',  ( -24.30048588269890075, -16.36411231998813065, 59.12332431758468942 ) ) ;
#21848=CARTESIAN_POINT ( 'NONE',  ( -20.18610667881221232, -8.319513185189903126, 66.66615430743608783 ) ) ;
#21850=ORIENTED_EDGE ( 'NONE', *, *, #41450, .T. ) ;
#21851=EDGE_LOOP ( 'NONE', ( #42098, #7054, #29263, #30196, #39580 ) ) ;
#21852=CARTESIAN_POINT ( 'NONE',  ( -13.38575581802539993, -9.030060914960570173, 60.72478133471773276 ) ) ;
#21854=CARTESIAN_POINT ( 'NONE',  ( -21.07302329935935958, -21.30456606900342464, 62.29188282781374397 ) ) ;
#21855=CARTESIAN_POINT ( 'NONE',  ( -24.03160971261424805, -17.26750559640275640, 69.71339792588547368 ) ) ;
#21856=LINE ( 'NONE', #23091, #18152 ) ;
#21857=VERTEX_POINT ( 'NONE', #6743 ) ;
#21859=ORIENTED_EDGE ( 'NONE', *, *, #8908, .T. ) ;
#21864=CARTESIAN_POINT ( 'NONE',  ( -10.39906353449755372, -15.43672942677450521, 61.45277822496478848 ) ) ;
#21866=EDGE_LOOP ( 'NONE', ( #4097, #2551, #43077, #19942, #34391 ) ) ;
#21867=CARTESIAN_POINT ( 'NONE',  ( -14.73482268938652417, -8.346338953448071862, 60.33498763304578461 ) ) ;
#21868=EDGE_CURVE ( 'NONE', #35725, #37402, #25218, .T. ) ;
#21869=ORIENTED_EDGE ( 'NONE', *, *, #13811, .F. ) ;
#21870=CARTESIAN_POINT ( 'NONE',  ( -15.57524973202195184, -7.592253851314364255, 70.80978608612899450 ) ) ;
#21871=DIRECTION ( 'NONE',  ( 0.2122660683108583690, -0.9772119095896469876, 7.504255179194988334E-08 ) ) ;
#21872=ORIENTED_EDGE ( 'NONE', *, *, #15125, .F. ) ;
#21874=ORIENTED_EDGE ( 'NONE', *, *, #25705, .T. ) ;
#21878=CARTESIAN_POINT ( 'NONE',  ( -24.87323499971020624, -14.68548341078430575, 62.85263093027649006 ) ) ;
#21879=ORIENTED_EDGE ( 'NONE', *, *, #32110, .T. ) ;
#21880=CARTESIAN_POINT ( 'NONE',  ( -22.41240261796999178, -19.79131148728009393, 69.46858230278321855 ) ) ;
#21882=CARTESIAN_POINT ( 'NONE',  ( -11.47236213698566054, -10.32806074475630886, 74.55389686390628867 ) ) ;
#21883=ORIENTED_EDGE ( 'NONE', *, *, #43703, .T. ) ;
#21885=ADVANCED_FACE ( 'NONE', ( #47390 ), #36035, .T. ) ;
#21886=B_SPLINE_CURVE_WITH_KNOTS ( 'NONE', 3,
 ( #3994, #16017, #26642, #23686, #26388, #41403, #19004, #34009, #306, #41657 ),
 .UNSPECIFIED., .F., .F.,
 ( 4, 2, 2, 2, 4 ),
 ( 0.6272669072877865570, 0.7522669073073026125, 0.8772669073268186679, 1.002266907346334612, 1.127266907365850779 ),
 .UNSPECIFIED. ) ;
#21888=CARTESIAN_POINT ( 'NONE',  ( -24.86170408668008847, -14.37683769452534222, 66.32146239653503983 ) ) ;
#21889=ORIENTED_EDGE ( 'NONE', *, *, #2845, .T. ) ;
#21890=CARTESIAN_POINT ( 'NONE',  ( -11.73296596577226936, -10.64774513788296417, 74.72412863062541533 ) ) ;
#21891=EDGE_CURVE ( 'NONE', #45956, #15007, #48608, .T. ) ;
#21892=ORIENTED_EDGE ( 'NONE', *, *, #39882, .F. ) ;
#21893=ORIENTED_EDGE ( 'NONE', *, *, #9769, .T. ) ;
#21894=FACE_OUTER_BOUND ( 'NONE', #21198, .T. ) ;
#21895=CARTESIAN_POINT ( 'NONE',  ( -17.39742520082695165, -7.759256980592265762, 67.17039592192074338 ) ) ;
#21897=CARTESIAN_POINT ( 'NONE',  ( -10.44916039635137039, -15.83526825291551177, 64.50771589744864798 ) ) ;
#21898=( BOUNDED_SURFACE ( )  B_SPLINE_SURFACE ( 3, 1, ( 
 ( #11422, #40263 ),
 ( #36531, #32844 ),
 ( #47883, #3054 ),
 ( #18066, #33076 ),
 ( #14355, #29412 ),
 ( #19541, #11925 ),
 ( #4291, #38741 ) ),
 .UNSPECIFIED., .T., .F., .F. ) 
 B_SPLINE_SURFACE_WITH_KNOTS ( ( 4, 3, 4 ),
 ( 2, 2 ),
 ( 0.000000000000000000, 0.5000000000000000000, 1.000000000000000000 ),
 ( 0.000000000000000000, 1.000000000000000000 ),
 .UNSPECIFIED. ) 
 GEOMETRIC_REPRESENTATION_ITEM ( )  RATIONAL_B_SPLINE_SURFACE ( (
 ( 1.000000000000000000, 1.000000000000000000),
 ( 0.3333333333333335369, 0.3333333333333330373),
 ( 0.3333333333333335369, 0.3333333333333330373),
 ( 1.000000000000000000, 1.000000000000000000),
 ( 0.3333333333333333703, 0.3333333333333333703),
 ( 0.3333333333333333703, 0.3333333333333333703),
 ( 1.000000000000000000, 1.000000000000000000) ) ) 
 REPRESENTATION_ITEM ( '' )  SURFACE ( )  );
#21900=CARTESIAN_POINT ( 'NONE',  ( -8.039996143071578061, -9.893874759132541996, 53.49999999999995026 ) ) ;
#21901=MECHANICAL_DESIGN_GEOMETRIC_PRESENTATION_REPRESENTATION('',(#41558),#48644);
#21902=CARTESIAN_POINT ( 'NONE',  ( -15.48396703021662546, -7.615489166865526904, 70.72334449499163611 ) ) ;
#21906=VERTEX_POINT ( 'NONE', #13856 ) ;
#21907=CARTESIAN_POINT ( 'NONE',  ( -11.16720021946830244, -11.56054808309503557, 67.91864607954204303 ) ) ;
#21909=VECTOR ( 'NONE', #41760, 999.9999999999998863 ) ;
#21911=CARTESIAN_POINT ( 'NONE',  ( -17.72419722990865054, -21.80277058550420577, 58.40553378253839156 ) ) ;
#21912=ORIENTED_EDGE ( 'NONE', *, *, #30299, .T. ) ;
#21916=CYLINDRICAL_SURFACE ( 'NONE', #1670, 0.1500000000000071554 ) ;
#21917=PLANE ( 'NONE',  #4436 ) ;
#21918=EDGE_CURVE ( 'NONE', #14949, #9880, #38051, .T. ) ;
#21923=ORIENTED_EDGE ( 'NONE', *, *, #1140, .T. ) ;
#21924=CARTESIAN_POINT ( 'NONE',  ( -13.67308226471031141, -21.24601619275060571, 68.65636342939112069 ) ) ;
#21926=CARTESIAN_POINT ( 'NONE',  ( -12.56747607676768830, -20.45877693976744638, 71.98370581712723038 ) ) ;
#21927=CARTESIAN_POINT ( 'NONE',  ( -10.83447764080151643, -17.17455424171161482, 64.85569185657212188 ) ) ;
#21929=CARTESIAN_POINT ( 'NONE',  ( -24.84449963183508459, -13.71944596863515464, 47.99999999999994316 ) ) ;
#21931=AXIS2_PLACEMENT_3D ( 'NONE', #1063, #16061, #31102 ) ;
#21932=ORIENTED_EDGE ( 'NONE', *, *, #5408, .T. ) ;
#21933=DIRECTION ( 'NONE',  ( 0.8356905716187448263, -0.5492005722024783099, -7.728900804118361606E-08 ) ) ;
#21934=CARTESIAN_POINT ( 'NONE',  ( -24.39025819466740685, -14.12117216163392186, 69.72563349076150985 ) ) ;
#21943=( BOUNDED_SURFACE ( )  B_SPLINE_SURFACE ( 3, 1, ( 
 ( #24944, #39963 ),
 ( #6231, #2045 ),
 ( #47110, #6479 ),
 ( #40208, #17771 ),
 ( #17295, #6711 ),
 ( #36253, #43917 ),
 ( #36484, #46868 ) ),
 .UNSPECIFIED., .T., .F., .F. ) 
 B_SPLINE_SURFACE_WITH_KNOTS ( ( 4, 3, 4 ),
 ( 2, 2 ),
 ( 0.000000000000000000, 0.5000000000000000000, 1.000000000000000000 ),
 ( 0.000000000000000000, 1.000000000000000000 ),
 .UNSPECIFIED. ) 
 GEOMETRIC_REPRESENTATION_ITEM ( )  RATIONAL_B_SPLINE_SURFACE ( (
 ( 1.000000000000000000, 1.000000000000000000),
 ( 0.3333333333333335369, 0.3333333333333330373),
 ( 0.3333333333333335369, 0.3333333333333330373),
 ( 1.000000000000000000, 1.000000000000000000),
 ( 0.3333333333333333703, 0.3333333333333333703),
 ( 0.3333333333333333703, 0.3333333333333333703),
 ( 1.000000000000000000, 1.000000000000000000) ) ) 
 REPRESENTATION_ITEM ( '' )  SURFACE ( )  );
#21944=CARTESIAN_POINT ( 'NONE',  ( -24.23636321612255173, -17.82529083293033167, 62.58865660992282898 ) ) ;
#21945=CARTESIAN_POINT ( 'NONE',  ( -22.86460234468921016, -19.29871796126476013, 59.18410835798781022 ) ) ;
#21946=CARTESIAN_POINT ( 'NONE',  ( -24.23267513707162379, -12.96582210470760543, 70.07243177896738473 ) ) ;
#21947=ORIENTED_EDGE ( 'NONE', *, *, #38791, .T. ) ;
#21948=CARTESIAN_POINT ( 'NONE',  ( -9.939267784769082681, -14.33236412611010913, 54.27966884056655061 ) ) ;
#21949=FACE_OUTER_BOUND ( 'NONE', #16305, .T. ) ;
#21951=CARTESIAN_POINT ( 'NONE',  ( -10.44916060947156566, -15.83526976542894182, 64.65771589744088033 ) ) ;
#21952=ADVANCED_FACE ( 'NONE', ( #17565 ), #46587, .T. ) ;
#21953=CARTESIAN_POINT ( 'NONE',  ( -16.23263389423368963, -22.16407464444966280, 58.39930168947970657 ) ) ;
#21955=VERTEX_POINT ( 'NONE', #26189 ) ;
#21956=ORIENTED_EDGE ( 'NONE', *, *, #30513, .F. ) ;
#21957=CARTESIAN_POINT ( 'NONE',  ( -11.39216336840796373, -18.45920852072106300, 61.29182966166492719 ) ) ;
#21958=ORIENTED_EDGE ( 'NONE', *, *, #45028, .F. ) ;
#21961=CARTESIAN_POINT ( 'NONE',  ( -11.30083338927175873, -18.20384847608787027, 57.87884914278906479 ) ) ;
#21962=CARTESIAN_POINT ( 'NONE',  ( -11.57425704488359841, -18.65360627554439077, 65.04707076833931012 ) ) ;
#21963=CARTESIAN_POINT ( 'NONE',  ( -14.47717485532954029, -21.65240259781455023, 58.35273132940589136 ) ) ;
#21965=B_SPLINE_CURVE_WITH_KNOTS ( 'NONE', 3,
 ( #6763, #43717, #25472, #20813, #17094, #9971, #40481, #32617, #6525, #2811 ),
 .UNSPECIFIED., .F., .F.,
 ( 4, 2, 2, 2, 4 ),
 ( 0.6272669072782678379, 0.7522669073001559958, 0.8772669073220440428, 1.002266907343932090, 1.127266907365820359 ),
 .UNSPECIFIED. ) ;
#21966=FACE_BOUND ( 'NONE', #28281, .T. ) ;
#21968=( BOUNDED_CURVE ( )  B_SPLINE_CURVE ( 3, ( #34880, #923, #38824, #30492 ),
 .UNSPECIFIED., .F., .F. ) 
 B_SPLINE_CURVE_WITH_KNOTS ( ( 4, 4 ),
 ( 0.9074455897393660653, 1.000000000000000000 ),
 .UNSPECIFIED. ) 
 CURVE ( )  GEOMETRIC_REPRESENTATION_ITEM ( )  RATIONAL_B_SPLINE_CURVE ( ( 0.6983129098260907330, 0.7760317562606962039, 0.8765941196519992928, 1.000000000000000000 ) ) 
 REPRESENTATION_ITEM ( '' )  );
#21969=CARTESIAN_POINT ( 'NONE',  ( -23.41616298382994898, -18.52428493080399008, 72.77840375779385340 ) ) ;
#21970=CARTESIAN_POINT ( 'NONE',  ( -16.74954815124876006, -21.77674055613599080, 68.99560679921106043 ) ) ;
#21971=ORIENTED_EDGE ( 'NONE', *, *, #46580, .F. ) ;
#21974=VECTOR ( 'NONE', #33194, 1000.000000000000000 ) ;
#21975=CARTESIAN_POINT ( 'NONE',  ( -16.84878425383806189, -22.23771130781744532, 72.35198525528087998 ) ) ;
#21976=CARTESIAN_POINT ( 'NONE',  ( -11.06177494515391757, -11.76359664285707574, 67.61864456584771688 ) ) ;
#21977=CARTESIAN_POINT ( 'NONE',  ( -24.21572389103915413, -12.90431785807809639, 62.83263897504365048 ) ) ;
#21978=CARTESIAN_POINT ( 'NONE',  ( -14.06084784944548716, -21.00867483325099982, 68.34136283933983691 ) ) ;
#21983=ORIENTED_EDGE ( 'NONE', *, *, #8079, .T. ) ;
#21985=ORIENTED_EDGE ( 'NONE', *, *, #46915, .F. ) ;
#21986=CARTESIAN_POINT ( 'NONE',  ( -17.13206997002025389, -21.80311261865791295, 72.27429256327307883 ) ) ;
#21987=B_SPLINE_CURVE_WITH_KNOTS ( 'NONE', 1,
 ( #10971, #26966 ),
 .UNSPECIFIED., .F., .F.,
 ( 2, 2 ),
 ( 0.000000000000000000, 1.000000000000000000 ),
 .UNSPECIFIED. ) ;
#21994=ORIENTED_EDGE ( 'NONE', *, *, #39390, .T. ) ;
#21995=DIRECTION ( 'NONE',  ( -0.6105870317843966610, -0.7919491628991827126, 6.540688078712155195E-08 ) ) ;
#21997=ORIENTED_EDGE ( 'NONE', *, *, #5265, .T. ) ;
#21998=CARTESIAN_POINT ( 'NONE',  ( -21.49815937814055999, -9.116931945208399668, 70.43132539264750847 ) ) ;
#22000=ORIENTED_EDGE ( 'NONE', *, *, #47856, .F. ) ;
#22001=CARTESIAN_POINT ( 'NONE',  ( -10.55090139406780558, -17.68373120125836806, 68.14076041135473361 ) ) ;
#22003=CARTESIAN_POINT ( 'NONE',  ( -23.00454255336054743, -10.50046069577333263, 59.88731295783226471 ) ) ;
#22004=VERTEX_POINT ( 'NONE', #34042 ) ;
#22005=CARTESIAN_POINT ( 'NONE',  ( -11.22470860480879118, -11.43539691024457206, 71.23293728648457090 ) ) ;
#22006=EDGE_CURVE ( 'NONE', #5056, #18999, #36802, .T. ) ;
#22007=CARTESIAN_POINT ( 'NONE',  ( -23.36642234765754367, -18.50986368505970958, 72.77984929533243985 ) ) ;
#22008=VECTOR ( 'NONE', #44914, 1000.000000000000000 ) ;
#22009=EDGE_CURVE ( 'NONE', #33660, #44249, #46270, .T. ) ;
#22010=CARTESIAN_POINT ( 'NONE',  ( -10.76763519559319882, -17.13171766695033327, 61.15743118826002700 ) ) ;
#22011=CARTESIAN_POINT ( 'NONE',  ( -21.99213670719075253, -20.17946569659695655, 59.04970794435396897 ) ) ;
#22012=ORIENTED_EDGE ( 'NONE', *, *, #44965, .T. ) ;
#22014=CARTESIAN_POINT ( 'NONE',  ( -15.48424252676649182, -21.53505049348036948, 72.34575460973682937 ) ) ;
#22015=CARTESIAN_POINT ( 'NONE',  ( -21.92674792687542862, -8.873837487361237564, 66.81149990064047017 ) ) ;
#22016=ADVANCED_FACE ( 'NONE', ( #14568 ), #19275, .T. ) ;
#22018=ORIENTED_EDGE ( 'NONE', *, *, #12128, .F. ) ;
#22019=CARTESIAN_POINT ( 'NONE',  ( -24.66730423131801331, -13.06573828131289616, 62.94768895321241331 ) ) ;
#22021=EDGE_LOOP ( 'NONE', ( #26279, #15496, #33617, #34657, #10283 ) ) ;
#22022=CARTESIAN_POINT ( 'NONE',  ( -17.91839958824308709, -21.79173199888728263, 61.87535923606637311 ) ) ;
#22023=AXIS2_PLACEMENT_3D ( 'NONE', #33683, #48732, #45064 ) ;
#22025=CARTESIAN_POINT ( 'NONE',  ( -24.43362360091611052, -14.05489060867666673, 73.42271507725003232 ) ) ;
#22026=CARTESIAN_POINT ( 'NONE',  ( -11.70231104532641631, -10.03806069876099727, 67.69885649244250203 ) ) ;
#22027=EDGE_LOOP ( 'NONE', ( #36407, #8677, #8195, #12654, #69 ) ) ;
#22029=ORIENTED_EDGE ( 'NONE', *, *, #14781, .T. ) ;
#22030=VERTEX_POINT ( 'NONE', #3777 ) ;
#22031=ORIENTED_EDGE ( 'NONE', *, *, #48438, .T. ) ;
#22036=CARTESIAN_POINT ( 'NONE',  ( -14.05958695725781915, -8.162196217632502027, 70.82934004658783067 ) ) ;
#22037=ADVANCED_FACE ( 'NONE', ( #41434 ), #44662, .F. ) ;
#22038=CARTESIAN_POINT ( 'NONE',  ( -13.18494979104506015, -8.682762004662409439, 60.48304321394137162 ) ) ;
#22039=B_SPLINE_CURVE_WITH_KNOTS ( 'NONE', 3,
 ( #44779, #21628, #3387, #44292, #14203, #18397, #33402, #14433, #3634, #48443 ),
 .UNSPECIFIED., .F., .F.,
 ( 4, 2, 2, 2, 4 ),
 ( 0.000000000000000000, 0.2500000000000000000, 0.5000000000000000000, 0.7500000000000000000, 1.000000000000000000 ),
 .UNSPECIFIED. ) ;
#22040=EDGE_CURVE ( 'NONE', #39442, #32446, #37236, .T. ) ;
#22042=ORIENTED_EDGE ( 'NONE', *, *, #12402, .T. ) ;
#22045=CARTESIAN_POINT ( 'NONE',  ( -11.47653751526730304, -10.32245935128858427, 74.61697868304008807 ) ) ;
#22046=CYLINDRICAL_SURFACE ( 'NONE', #8007, 0.1500000000000003553 ) ;
#22047=AXIS2_PLACEMENT_3D ( 'NONE', #9897, #39924, #47563 ) ;
#22050=ORIENTED_EDGE ( 'NONE', *, *, #32515, .F. ) ;
#22051=CARTESIAN_POINT ( 'NONE',  ( -16.71957921250844592, -21.82421608262117729, 68.71032757591046902 ) ) ;
#22056=EDGE_LOOP ( 'NONE', ( #29186, #9143 ) ) ;
#22057=CARTESIAN_POINT ( 'NONE',  ( -13.07136565370527315, -8.762923774744256988, 64.02451247989536398 ) ) ;
#22058=CARTESIAN_POINT ( 'NONE',  ( -20.28184570768963013, -8.419050735858720103, 66.79606545271752793 ) ) ;
#22059=CARTESIAN_POINT ( 'NONE',  ( -18.56294508348570460, -7.902357773425570997, 73.84064450189322315 ) ) ;
#22060=CARTESIAN_POINT ( 'NONE',  ( -10.39641337496300544, -12.33600653425179416, 57.48890720123886666 ) ) ;
#22062=CARTESIAN_POINT ( 'NONE',  ( -11.09546941031917378, -10.87811254196722111, 57.34756656758956694 ) ) ;
#22063=CARTESIAN_POINT ( 'NONE',  ( -24.42531086868747892, -14.77968181448406426, 62.78466667327232642 ) ) ;
#22064=B_SPLINE_CURVE_WITH_KNOTS ( 'NONE', 1,
 ( #21699, #47086 ),
 .UNSPECIFIED., .F., .F.,
 ( 2, 2 ),
 ( 0.000000000000000000, 1.000000000000000000 ),
 .UNSPECIFIED. ) ;
#22066=CARTESIAN_POINT ( 'NONE',  ( -19.28352822169459202, -22.07505156356299381, 47.99999999999994316 ) ) ;
#22067=ORIENTED_EDGE ( 'NONE', *, *, #18454, .F. ) ;
#22068=CARTESIAN_POINT ( 'NONE',  ( -16.26183769579148475, -7.855670737815882099, 60.50028478907628937 ) ) ;
#22070=DIRECTION ( 'NONE',  ( -0.003782665018460030538, -0.9999928456970870183, -9.532993539451315208E-09 ) ) ;
#22071=VERTEX_POINT ( 'NONE', #19037 ) ;
#22072=FACE_BOUND ( 'NONE', #47254, .T. ) ;
#22077=ADVANCED_FACE ( 'NONE', ( #38714 ), #9185, .T. ) ;
#22080=ORIENTED_EDGE ( 'NONE', *, *, #31742, .F. ) ;
#22081=LINE ( 'NONE', #48413, #32359 ) ;
#22082=ORIENTED_EDGE ( 'NONE', *, *, #20662, .F. ) ;
#22083=CARTESIAN_POINT ( 'NONE',  ( -21.57946453887431204, -8.565578233975859490, 54.27966884056655061 ) ) ;
#22085=VERTEX_POINT ( 'NONE', #27392 ) ;
#22086=CARTESIAN_POINT ( 'NONE',  ( -9.979603264230430426, -14.52052340097724148, 68.04295441848455539 ) ) ;
#22087=AXIS2_PLACEMENT_3D ( 'NONE', #20612, #35605, #1389 ) ;
#22088=CARTESIAN_POINT ( 'NONE',  ( -18.39951368268757648, -22.19516171751901368, 69.00010101991060196 ) ) ;
#22091=CYLINDRICAL_SURFACE ( 'NONE', #10773, 0.1500000000000054345 ) ;
#22092=DIRECTION ( 'NONE',  ( 1.590464103011092396E-07, -3.579926632912963412E-07, 0.9999999999999231726 ) ) ;
#22093=AXIS2_PLACEMENT_3D ( 'NONE', #29987, #37341, #47960 ) ;
#22094=CARTESIAN_POINT ( 'NONE',  ( -23.45365590349393869, -19.18493892615664365, 62.45383243984888111 ) ) ;
#22095=CARTESIAN_POINT ( 'NONE',  ( -10.02995815481606634, -13.89786978184575794, 57.63320425522585566 ) ) ;
#22096=( BOUNDED_CURVE ( )  B_SPLINE_CURVE ( 3, ( #28761, #29484, #2654, #44284 ),
 .UNSPECIFIED., .F., .F. ) 
 B_SPLINE_CURVE_WITH_KNOTS ( ( 4, 4 ),
 ( 0.000000000000000000, 0.4074455897393662318 ),
 .UNSPECIFIED. ) 
 CURVE ( )  GEOMETRIC_REPRESENTATION_ITEM ( )  RATIONAL_B_SPLINE_CURVE ( ( 1.000000000000000000, 0.4567392136813306358, 0.3561768502900297673, 0.6983129098260973944 ) ) 
 REPRESENTATION_ITEM ( '' )  );
#22097=CARTESIAN_POINT ( 'NONE',  ( -11.67943375510494874, -18.89645239624664796, 68.50217487844219022 ) ) ;
#22098=CARTESIAN_POINT ( 'NONE',  ( -13.95122194917832914, -8.664767797030865637, 70.88524802578001527 ) ) ;
#22099=CARTESIAN_POINT ( 'NONE',  ( -22.87929373774275632, -19.88409160966729772, 72.75745300618787326 ) ) ;
#22100=EDGE_CURVE ( 'NONE', #18877, #22777, #40954, .T. ) ;
#22101=ORIENTED_EDGE ( 'NONE', *, *, #34512, .F. ) ;
#22103=DIRECTION ( 'NONE',  ( -0.3636930986378154040, -0.9315188296557533887, 1.850371887917986020E-09 ) ) ;
#22104=EDGE_CURVE ( 'NONE', #6106, #20133, #28030, .T. ) ;
#22109=DIRECTION ( 'NONE',  ( -1.487365705136564946E-06, 6.376425429333053644E-07, 0.9999999999986904919 ) ) ;
#22112=EDGE_LOOP ( 'NONE', ( #39386, #22661, #22889, #21510, #14628 ) ) ;
#22113=( BOUNDED_SURFACE ( )  B_SPLINE_SURFACE ( 3, 1, ( 
 ( #3785, #11407 ),
 ( #33065, #44670 ),
 ( #10929, #40966 ),
 ( #29894, #44925 ),
 ( #31337, #12376 ),
 ( #20017, #26682 ),
 ( #340, #27400 ) ),
 .UNSPECIFIED., .T., .F., .F. ) 
 B_SPLINE_SURFACE_WITH_KNOTS ( ( 4, 3, 4 ),
 ( 2, 2 ),
 ( 0.000000000000000000, 0.5000000000000000000, 1.000000000000000000 ),
 ( 0.000000000000000000, 1.000000000000000000 ),
 .UNSPECIFIED. ) 
 GEOMETRIC_REPRESENTATION_ITEM ( )  RATIONAL_B_SPLINE_SURFACE ( (
 ( 1.000000000000000000, 1.000000000000000000),
 ( 0.3333333333333335369, 0.3333333333333330373),
 ( 0.3333333333333335369, 0.3333333333333330373),
 ( 1.000000000000000000, 1.000000000000000000),
 ( 0.3333333333333333703, 0.3333333333333333703),
 ( 0.3333333333333333703, 0.3333333333333333703),
 ( 1.000000000000000000, 1.000000000000000000) ) ) 
 REPRESENTATION_ITEM ( '' )  SURFACE ( )  );
#22115=( BOUNDED_CURVE ( )  B_SPLINE_CURVE ( 3, ( #41600, #19188, #4910, #46751 ),
 .UNSPECIFIED., .F., .F. ) 
 B_SPLINE_CURVE_WITH_KNOTS ( ( 4, 4 ),
 ( 0.9074455897393582937, 1.000000000000000000 ),
 .UNSPECIFIED. ) 
 CURVE ( )  GEOMETRIC_REPRESENTATION_ITEM ( )  RATIONAL_B_SPLINE_CURVE ( ( 0.6983129098260780765, 0.7760317562606853237, 0.8765941196519926315, 1.000000000000000000 ) ) 
 REPRESENTATION_ITEM ( '' )  );
#22118=CARTESIAN_POINT ( 'NONE',  ( -16.91478550490786859, -21.84108428878278119, 72.18015306840750611 ) ) ;
#22119=CARTESIAN_POINT ( 'NONE',  ( -12.00910550946480093, -19.92697606054074910, 58.04027092519303466 ) ) ;
#22121=CARTESIAN_POINT ( 'NONE',  ( -10.52422430310768320, -17.61911375464911700, 68.21226508126260057 ) ) ;
#22123=AXIS2_PLACEMENT_3D ( 'NONE', #40758, #14148, #25026 ) ;
#22124=( BOUNDED_CURVE ( )  B_SPLINE_CURVE ( 3, ( #44131, #29082, #6195, #2501 ),
 .UNSPECIFIED., .F., .F. ) 
 B_SPLINE_CURVE_WITH_KNOTS ( ( 4, 4 ),
 ( 0.4074455897393659543, 0.5000000000000000000 ),
 .UNSPECIFIED. ) 
 CURVE ( )  GEOMETRIC_REPRESENTATION_ITEM ( )  RATIONAL_B_SPLINE_CURVE ( ( 0.6983129098260879575, 0.7760317562606924291, 0.8765941196519958512, 0.9999999999999976685 ) ) 
 REPRESENTATION_ITEM ( '' )  );
#22125=CARTESIAN_POINT ( 'NONE',  ( -15.47038646904106507, -21.58309222549749506, 72.34575460768671462 ) ) ;
#22126=DIRECTION ( 'NONE',  ( -0.9840843158728899143, 0.1445225939548007710, 0.1033986416233888955 ) ) ;
#22128=ORIENTED_EDGE ( 'NONE', *, *, #10177, .T. ) ;
#22130=CARTESIAN_POINT ( 'NONE',  ( -18.72680718162379065, -7.880610904852765053, 70.67068030199192208 ) ) ;
#22131=CARTESIAN_POINT ( 'NONE',  ( -10.43972881942000086, -15.77115500203794873, 64.52243715390834211 ) ) ;
#22132=ORIENTED_EDGE ( 'NONE', *, *, #23533, .F. ) ;
#22133=CARTESIAN_POINT ( 'NONE',  ( -21.99178500617274779, -9.439039195359631762, 59.72171213140594404 ) ) ;
#22135=CARTESIAN_POINT ( 'NONE',  ( -15.35953700001868683, -21.96742592204022770, 72.19575459128920158 ) ) ;
#22136=CARTESIAN_POINT ( 'NONE',  ( -11.53125565324743107, -18.58817318659712114, 65.03090579962859863 ) ) ;
#22138=CARTESIAN_POINT ( 'NONE',  ( -13.17078218117215549, -9.186392337449538203, 67.39414915108072535 ) ) ;
#22140=CARTESIAN_POINT ( 'NONE',  ( -18.62018691191416764, -22.16273284384092079, 72.42364395285933654 ) ) ;
#22141=EDGE_CURVE ( 'NONE', #39613, #22485, #46880, .T. ) ;
#22142=ORIENTED_EDGE ( 'NONE', *, *, #33234, .F. ) ;
#22143=CARTESIAN_POINT ( 'NONE',  ( -12.00971705810820467, -9.691755786776280246, 60.67422651510300113 ) ) ;
#22145=CARTESIAN_POINT ( 'NONE',  ( -21.61813339613238227, -8.651787399021619862, 73.71633365192373333 ) ) ;
#22147=CARTESIAN_POINT ( 'NONE',  ( -12.53474317923432224, -20.43030517998690954, 71.95653676292567980 ) ) ;
#22148=CARTESIAN_POINT ( 'NONE',  ( -11.33335366867738259, -11.35902659219953748, 60.90559029689631387 ) ) ;
#22151=ORIENTED_EDGE ( 'NONE', *, *, #14607, .F. ) ;
#22153=CARTESIAN_POINT ( 'NONE',  ( -22.79960313759534074, -9.650943445293346912, 73.66656413195866548 ) ) ;
#22154=CARTESIAN_POINT ( 'NONE',  ( -18.05440415122280839, -21.83127237841607027, 65.36004252941745563 ) ) ;
#22157=LINE ( 'NONE', #44819, #8520 ) ;
#22158=CARTESIAN_POINT ( 'NONE',  ( -12.84691039585993444, -8.931012183600500975, 67.56438067310742213 ) ) ;
#22159=CARTESIAN_POINT ( 'NONE',  ( -19.17247849636888901, -7.567181371456696226, 63.61584626116109575 ) ) ;
#22161=ORIENTED_EDGE ( 'NONE', *, *, #1768, .T. ) ;
#22162=CARTESIAN_POINT ( 'NONE',  ( -24.45201639769885205, -14.25170802724723451, 69.80275273439818307 ) ) ;
#22163=EDGE_CURVE ( 'NONE', #35531, #11465, #37184, .T. ) ;
#22164=EDGE_CURVE ( 'NONE', #18995, #42817, #25671, .T. ) ;
#22168=ORIENTED_EDGE ( 'NONE', *, *, #26234, .F. ) ;
#22169=EDGE_CURVE ( 'NONE', #46048, #30823, #32058, .T. ) ;
#22170=EDGE_CURVE ( 'NONE', #28666, #32577, #42263, .T. ) ;
#22171=ORIENTED_EDGE ( 'NONE', *, *, #26217, .F. ) ;
#22172=CARTESIAN_POINT ( 'NONE',  ( -20.70232472158584969, -8.624289250480600799, 59.84125250310036392 ) ) ;
#22173=CYLINDRICAL_SURFACE ( 'NONE', #25272, 0.1500000000000020484 ) ;
#22174=CARTESIAN_POINT ( 'NONE',  ( -13.35819042472069107, -21.05197888995676436, 61.70141705377209007 ) ) ;
#22175=CARTESIAN_POINT ( 'NONE',  ( -11.55573855159262386, -10.21941529800896653, 71.15388400389697665 ) ) ;
#22176=EDGE_LOOP ( 'NONE', ( #1155, #24076 ) ) ;
#22177=DIRECTION ( 'NONE',  ( -0.9660698163281070672, -0.2582810677919976095, 5.363434502754640132E-08 ) ) ;
#22178=CARTESIAN_POINT ( 'NONE',  ( -11.42264205816738176, -11.09470156419723708, 64.29315101522172426 ) ) ;
#22180=EDGE_LOOP ( 'NONE', ( #21994, #6002 ) ) ;
#22181=CARTESIAN_POINT ( 'NONE',  ( -22.27803375191225399, -20.46189896727856095, 62.42094464928214848 ) ) ;
#22183=LINE ( 'NONE', #26121, #588 ) ;
#22184=EDGE_LOOP ( 'NONE', ( #7153, #31699, #6311, #18857, #15205 ) ) ;
#22186=ORIENTED_EDGE ( 'NONE', *, *, #36273, .T. ) ;
#22187=CARTESIAN_POINT ( 'NONE',  ( -10.45186911607087943, -17.43433898691305473, 64.82077674941292855 ) ) ;
#22189=VERTEX_POINT ( 'NONE', #9666 ) ;
#22190=CARTESIAN_POINT ( 'NONE',  ( -23.71751471349159601, -11.63122711669449494, 63.23746208799618529 ) ) ;
#22193=FACE_OUTER_BOUND ( 'NONE', #48454, .T. ) ;
#22194=CARTESIAN_POINT ( 'NONE',  ( -24.48201381491371009, -14.78211897600973934, 66.32725479646262556 ) ) ;
#22196=CYLINDRICAL_SURFACE ( 'NONE', #42368, 0.1499999999999988287 ) ;
#22197=ORIENTED_EDGE ( 'NONE', *, *, #2049, .F. ) ;
#22198=CARTESIAN_POINT ( 'NONE',  ( -10.41614636368765900, -13.97037319380632248, 64.53236772669211518 ) ) ;
#22200=CARTESIAN_POINT ( 'NONE',  ( -11.92015382652974154, -10.40338788426078587, 70.97452903744414243 ) ) ;
#22201=CARTESIAN_POINT ( 'NONE',  ( -10.79744568551467587, -12.55229167313659921, 60.81470185434422859 ) ) ;
#22202=CARTESIAN_POINT ( 'NONE',  ( -17.06612543921954028, -7.818304145033148522, 70.71709262193978418 ) ) ;
#22203=ORIENTED_EDGE ( 'NONE', *, *, #20716, .F. ) ;
#22204=EDGE_LOOP ( 'NONE', ( #23024, #29743, #13715, #30686, #37997 ) ) ;
#22205=CARTESIAN_POINT ( 'NONE',  ( -11.06712688165958269, -18.69414528815109477, 61.39215548186584215 ) ) ;
#22207=ORIENTED_EDGE ( 'NONE', *, *, #48001, .T. ) ;
#22208=B_SPLINE_CURVE_WITH_KNOTS ( 'NONE', 1,
 ( #13226, #43549 ),
 .UNSPECIFIED., .F., .F.,
 ( 2, 2 ),
 ( 0.000000000000000000, 1.000000000000000000 ),
 .UNSPECIFIED. ) ;
#22210=CARTESIAN_POINT ( 'NONE',  ( -10.71495554099518088, -12.81234323494808436, 64.56836111193433680 ) ) ;
#22211=CARTESIAN_POINT ( 'NONE',  ( -20.68242297322939649, -8.109334927485972955, 63.44975001546675486 ) ) ;
#22212=CARTESIAN_POINT ( 'NONE',  ( -12.60165769527841384, -19.96275654529059906, 61.55245915020547898 ) ) ;
#22213=FACE_BOUND ( 'NONE', #37518, .T. ) ;
#22215=DIRECTION ( 'NONE',  ( 0.9918916210775228226, 0.1270866320121812332, -6.503929235867083869E-08 ) ) ;
#22216=B_SPLINE_CURVE_WITH_KNOTS ( 'NONE', 3,
 ( #38323, #31198, #45983, #9045, #4612, #19635, #24062, #5105, #16653, #46709 ),
 .UNSPECIFIED., .F., .F.,
 ( 4, 2, 2, 2, 4 ),
 ( 0.1272669073658303229, 0.2522669073463129630, 0.3772669073267956863, 0.5022669073072782986, 0.6272669072877610219 ),
 .UNSPECIFIED. ) ;
#22217=CYLINDRICAL_SURFACE ( 'NONE', #9454, 0.1500000000000013267 ) ;
#22219=VERTEX_POINT ( 'NONE', #5728 ) ;
#22221=CARTESIAN_POINT ( 'NONE',  ( -11.60479079619936371, -10.15731510490028100, 71.09176221476478474 ) ) ;
#22222=CARTESIAN_POINT ( 'NONE',  ( -19.83021750621371737, -21.38439240218873039, 72.58761523121964387 ) ) ;
#22224=CARTESIAN_POINT ( 'NONE',  ( -15.43182990062313564, -8.046249867383863830, 74.36513541778452918 ) ) ;
#22225=CARTESIAN_POINT ( 'NONE',  ( -10.42496409799848323, -14.69883155267435626, 71.62782692796884021 ) ) ;
#22227=ORIENTED_EDGE ( 'NONE', *, *, #4641, .F. ) ;
#22230=VERTEX_POINT ( 'NONE', #17505 ) ;
#22233=CARTESIAN_POINT ( 'NONE',  ( -20.13067905174874639, -8.351893152775456741, 73.83169569948991295 ) ) ;
#22234=ADVANCED_FACE ( 'NONE', ( #32536 ), #14035, .T. ) ;
#22238=CARTESIAN_POINT ( 'NONE',  ( -24.38143503755601316, -15.58083059521001168, 73.30303748419844112 ) ) ;
#22239=PLANE ( 'NONE',  #13935 ) ;
#22241=( BOUNDED_CURVE ( )  B_SPLINE_CURVE ( 3, ( #31836, #13098, #43163, #24462 ),
 .UNSPECIFIED., .F., .F. ) 
 B_SPLINE_CURVE_WITH_KNOTS ( ( 4, 4 ),
 ( 0.5000000000000000000, 0.9074455897393643999 ),
 .UNSPECIFIED. ) 
 CURVE ( )  GEOMETRIC_REPRESENTATION_ITEM ( )  RATIONAL_B_SPLINE_CURVE ( ( 1.000000000000017542, 0.4567392136813297476, 0.3561768502900171107, 0.6983129098260985046 ) ) 
 REPRESENTATION_ITEM ( '' )  );
#22243=CARTESIAN_POINT ( 'NONE',  ( -11.53247150430815715, -18.68106468654471541, 64.89707076448696910 ) ) ;
#22245=CARTESIAN_POINT ( 'NONE',  ( -17.76182844141538553, -7.366698643885237985, 60.21914265551018275 ) ) ;
#22246=CARTESIAN_POINT ( 'NONE',  ( -21.36284888653444725, -21.13297021396988384, 69.16954901539321554 ) ) ;
#22248=ORIENTED_EDGE ( 'NONE', *, *, #13877, .F. ) ;
#22249=CARTESIAN_POINT ( 'NONE',  ( -10.70297003644833644, -11.59513240183115279, 71.27356180636090244 ) ) ;
#22250=DIRECTION ( 'NONE',  ( 0.9584484254710482487, 0.2852658684667118694, -3.516456353195806577E-08 ) ) ;
#22251=CARTESIAN_POINT ( 'NONE',  ( -15.11195812866605692, -21.41632606413040918, 65.10596681519622564 ) ) ;
#22252=CARTESIAN_POINT ( 'NONE',  ( -22.22496508270376481, -20.50616197626463233, 58.80796965402809917 ) ) ;
#22254=CARTESIAN_POINT ( 'NONE',  ( -24.68275079258767235, -16.48720463981601370, 59.23837148777906236 ) ) ;
#22256=CARTESIAN_POINT ( 'NONE',  ( -20.16691314815865255, -21.73601827195274794, 72.58974169946205279 ) ) ;
#22257=( BOUNDED_CURVE ( )  B_SPLINE_CURVE ( 3, ( #6179, #21201, #35957, #47312 ),
 .UNSPECIFIED., .F., .F. ) 
 B_SPLINE_CURVE_WITH_KNOTS ( ( 4, 4 ),
 ( 0.000000000000000000, 0.4074455897393615689 ),
 .UNSPECIFIED. ) 
 CURVE ( )  GEOMETRIC_REPRESENTATION_ITEM ( )  RATIONAL_B_SPLINE_CURVE ( ( 1.000000000000000000, 0.4567392136813364090, 0.3561768502900319322, 0.6983129098260865142 ) ) 
 REPRESENTATION_ITEM ( '' )  );
#22258=CARTESIAN_POINT ( 'NONE',  ( -16.45566506110110438, -21.79267588865899086, 62.04095995016087528 ) ) ;
#22260=ORIENTED_EDGE ( 'NONE', *, *, #5099, .F. ) ;
#22261=CARTESIAN_POINT ( 'NONE',  ( -20.72573962529263625, -8.580110715261016097, 59.99125250080121674 ) ) ;
#22262=CARTESIAN_POINT ( 'NONE',  ( -24.32852063849251323, -13.38246526728995001, 59.37740068604990995 ) ) ;
#22263=VERTEX_POINT ( 'NONE', #28115 ) ;
#22264=CARTESIAN_POINT ( 'NONE',  ( -16.98991614605047218, -22.24663000551990777, 72.35038637723081933 ) ) ;
#22265=LINE ( 'NONE', #29652, #3020 ) ;
#22267=ADVANCED_FACE ( 'NONE', ( #21463 ), #21221, .T. ) ;
#22268=ORIENTED_EDGE ( 'NONE', *, *, #35505, .T. ) ;
#22270=DIRECTION ( 'NONE',  ( -5.731567514496413899E-31, -1.020425574103664789E-16, -1.000000000000000000 ) ) ;
#22272=VERTEX_POINT ( 'NONE', #46834 ) ;
#22275=DIRECTION ( 'NONE',  ( -0.5420872618288282707, -0.8403222004463035688, 7.592316861452269267E-08 ) ) ;
#22277=CARTESIAN_POINT ( 'NONE',  ( -10.72552546848295485, -12.61109793159036485, 61.09853568372136579 ) ) ;
#22279=ORIENTED_EDGE ( 'NONE', *, *, #15124, .F. ) ;
#22280=VERTEX_POINT ( 'NONE', #28839 ) ;
#22282=EDGE_CURVE ( 'NONE', #30016, #20100, #22124, .T. ) ;
#22284=CARTESIAN_POINT ( 'NONE',  ( -12.96596342764269316, -9.347744029417796696, 71.14925352873375175 ) ) ;
#22291=CARTESIAN_POINT ( 'NONE',  ( -16.16379449968008331, -22.15191876840708929, 58.47080954035841671 ) ) ;
#22292=ADVANCED_FACE ( 'NONE', ( #10135 ), #29014, .T. ) ;
#22294=CARTESIAN_POINT ( 'NONE',  ( -24.41897151118743636, -17.37347349776957017, 69.59835227440868266 ) ) ;
#22296=B_SPLINE_CURVE_WITH_KNOTS ( 'NONE', 1,
 ( #17778, #21733 ),
 .UNSPECIFIED., .F., .F.,
 ( 2, 2 ),
 ( 0.000000000000000000, 1.000000000000000000 ),
 .UNSPECIFIED. ) ;
#22298=CARTESIAN_POINT ( 'NONE',  ( -12.52591642561268515, -9.195683996340104471, 74.50418400381258266 ) ) ;
#22299=CARTESIAN_POINT ( 'NONE',  ( -24.30048628764226137, -16.36411057843138650, 59.27332431757403697 ) ) ;
#22300=FACE_OUTER_BOUND ( 'NONE', #42492, .T. ) ;
#22301=CARTESIAN_POINT ( 'NONE',  ( -9.990123186454296089, -14.31889395325652714, 64.50991104586785241 ) ) ;
#22305=CARTESIAN_POINT ( 'NONE',  ( -24.19823205308740910, -11.70861652093786454, 59.68246929106484799 ) ) ;
#22306=DIRECTION ( 'NONE',  ( -0.7437128929774847741, 0.6684991644116393683, -1.736198598217016398E-08 ) ) ;
#22307=DIRECTION ( 'NONE',  ( 2.671295499615842957E-06, 1.272698189891367967E-05, 0.9999999999154439712 ) ) ;
#22308=ORIENTED_EDGE ( 'NONE', *, *, #12879, .F. ) ;
#22312=FACE_BOUND ( 'NONE', #25395, .T. ) ;
#22315=CARTESIAN_POINT ( 'NONE',  ( -13.61033894779295395, -20.67921429907312003, 61.81646270068954152 ) ) ;
#22318=ORIENTED_EDGE ( 'NONE', *, *, #23198, .T. ) ;
#22319=CARTESIAN_POINT ( 'NONE',  ( -10.45160180800373873, -14.17496150716750769, 64.45974129894086957 ) ) ;
#22320=VERTEX_POINT ( 'NONE', #48036 ) ;
#22321=PLANE ( 'NONE',  #46313 ) ;
#22322=CARTESIAN_POINT ( 'NONE',  ( -10.97344478688443914, -18.53636807463781722, 58.00725798456583959 ) ) ;
#22323=EDGE_CURVE ( 'NONE', #8916, #36242, #39095, .T. ) ;
#22324=CARTESIAN_POINT ( 'NONE',  ( -10.61330328728660533, -12.98831903967553814, 67.73832347272892207 ) ) ;
#22326=CARTESIAN_POINT ( 'NONE',  ( -13.47643240338711124, -20.58993545956319338, 58.33184665923734968 ) ) ;
#22327=VERTEX_POINT ( 'NONE', #11583 ) ;
#22330=FACE_OUTER_BOUND ( 'NONE', #42285, .T. ) ;
#22331=CARTESIAN_POINT ( 'NONE',  ( -21.93774155219031385, -8.882177397035567523, 66.76175749538603554 ) ) ;
#22332=CARTESIAN_POINT ( 'NONE',  ( -20.69509252757554307, -8.115601716887088202, 63.49616818922779515 ) ) ;
#22333=DIRECTION ( 'NONE',  ( 0.2664710960620865210, -0.9638429098994647504, 4.833213314675751572E-08 ) ) ;
#22334=CARTESIAN_POINT ( 'NONE',  ( -14.23114477490021379, -8.578028806345869839, 74.38881623979730762 ) ) ;
#22335=EDGE_CURVE ( 'NONE', #23362, #27190, #22725, .T. ) ;
#22336=CARTESIAN_POINT ( 'NONE',  ( -17.85497298213014261, -7.371550647135725498, 60.20343865544412409 ) ) ;
#22337=ORIENTED_EDGE ( 'NONE', *, *, #30293, .F. ) ;
#22338=ORIENTED_EDGE ( 'NONE', *, *, #24628, .F. ) ;
#22340=CARTESIAN_POINT ( 'NONE',  ( -12.15423770757536026, -10.20156791825057496, 64.32914322081802538 ) ) ;
#22341=AXIS2_PLACEMENT_3D ( 'NONE', #22498, #33303, #33807 ) ;
#22342=CARTESIAN_POINT ( 'NONE',  ( -22.53028194631272640, -20.23415643105539274, 65.81083435350976174 ) ) ;
#22343=FACE_OUTER_BOUND ( 'NONE', #7294, .T. ) ;
#22345=EDGE_LOOP ( 'NONE', ( #15147, #23243, #44616, #47145, #32487, #30035, #36173 ) ) ;
#22348=ADVANCED_FACE ( 'NONE', ( #37417 ), #11102, .T. ) ;
#22349=FACE_OUTER_BOUND ( 'NONE', #33563, .T. ) ;
#22350=CARTESIAN_POINT ( 'NONE',  ( -23.98474789688958353, -17.25007084823549874, 69.71339792561613535 ) ) ;
#22352=CARTESIAN_POINT ( 'NONE',  ( -10.03016176022630646, -13.89628074529801438, 57.49179087295118507 ) ) ;
#22353=ADVANCED_FACE ( 'NONE', ( #10612 ), #26, .T. ) ;
#22354=VERTEX_POINT ( 'NONE', #40888 ) ;
#22356=CARTESIAN_POINT ( 'NONE',  ( -24.18470913683765389, -12.80901137141652768, 69.78715111652664405 ) ) ;
#22358=CARTESIAN_POINT ( 'NONE',  ( -15.25439996314754509, -21.46446225238890904, 65.29699935524728005 ) ) ;
#22359=ADVANCED_FACE ( 'NONE', ( #3966 ), #40379, .T. ) ;
#22360=FACE_OUTER_BOUND ( 'NONE', #16987, .T. ) ;
#22362=ORIENTED_EDGE ( 'NONE', *, *, #1459, .T. ) ;
#22363=B_SPLINE_CURVE_WITH_KNOTS ( 'NONE', 3,
 ( #24195, #39452, #39202, #30683, #30441, #45708, #38961, #1784, #2018, #41997 ),
 .UNSPECIFIED., .F., .F.,
 ( 4, 2, 2, 2, 4 ),
 ( 0.1272669073658251604, 0.2522669073463064682, 0.3772669073267878037, 0.5022669073072690837, 0.6272669072877503638 ),
 .UNSPECIFIED. ) ;
#22364=CARTESIAN_POINT ( 'NONE',  ( -24.69852204723760281, -16.41745771733451775, 59.30827817708741634 ) ) ;
#22366=ORIENTED_EDGE ( 'NONE', *, *, #41940, .F. ) ;
#22368=CARTESIAN_POINT ( 'NONE',  ( -10.31133302210429470, -17.02573883484783579, 57.81043661216028084 ) ) ;
#22369=CARTESIAN_POINT ( 'NONE',  ( -11.57425704488359841, -18.65360627554439077, 65.04707076833931012 ) ) ;
#22372=ADVANCED_FACE ( 'NONE', ( #15989 ), #8381, .F. ) ;
#22373=PLANE ( 'NONE',  #13198 ) ;
#22375=CARTESIAN_POINT ( 'NONE',  ( -18.59773863799375349, -22.16623006980740129, 72.39172614962501484 ) ) ;
#22377=CARTESIAN_POINT ( 'NONE',  ( -22.92319923916556235, -10.39759239192951590, 63.07185995337423634 ) ) ;
#22378=( BOUNDED_SURFACE ( )  B_SPLINE_SURFACE ( 3, 1, ( 
 ( #20094, #46450 ),
 ( #34618, #35100 ),
 ( #23561, #20343 ),
 ( #31419, #5085 ),
 ( #42755, #24045 ),
 ( #904, #1366 ),
 ( #15902, #42268 ) ),
 .UNSPECIFIED., .T., .F., .F. ) 
 B_SPLINE_SURFACE_WITH_KNOTS ( ( 4, 3, 4 ),
 ( 2, 2 ),
 ( 0.000000000000000000, 0.5000000000000000000, 1.000000000000000000 ),
 ( 0.000000000000000000, 1.000000000000000000 ),
 .UNSPECIFIED. ) 
 GEOMETRIC_REPRESENTATION_ITEM ( )  RATIONAL_B_SPLINE_SURFACE ( (
 ( 1.000000000000000000, 1.000000000000000000),
 ( 0.3333333333333335369, 0.3333333333333330373),
 ( 0.3333333333333335369, 0.3333333333333330373),
 ( 1.000000000000000000, 1.000000000000000000),
 ( 0.3333333333333333703, 0.3333333333333333703),
 ( 0.3333333333333333703, 0.3333333333333333703),
 ( 1.000000000000000000, 1.000000000000000000) ) ) 
 REPRESENTATION_ITEM ( '' )  SURFACE ( )  );
#22379=CARTESIAN_POINT ( 'NONE',  ( -16.00544582274271477, -7.903112417841744453, 63.95538887075813506 ) ) ;
#22380=CARTESIAN_POINT ( 'NONE',  ( -24.41485939984550058, -14.44976655980182834, 66.48292729254383460 ) ) ;
#22381=ORIENTED_EDGE ( 'NONE', *, *, #26179, .T. ) ;
#22382=CARTESIAN_POINT ( 'NONE',  ( -19.17551372071283922, -8.031400147991478278, 63.44705914822644388 ) ) ;
#22385=ORIENTED_EDGE ( 'NONE', *, *, #16524, .F. ) ;
#22391=CARTESIAN_POINT ( 'NONE',  ( -19.88388893082392528, -8.193741602349351894, 70.40667630031393287 ) ) ;
#22392=CARTESIAN_POINT ( 'NONE',  ( -12.40538917401127961, -20.31523793222865493, 68.52152763170285255 ) ) ;
#22393=CARTESIAN_POINT ( 'NONE',  ( -24.31823774515246939, -17.63313259158020685, 66.05861911469568781 ) ) ;
#22394=( BOUNDED_CURVE ( )  B_SPLINE_CURVE ( 3, ( #41904, #42146, #8182, #8410 ),
 .UNSPECIFIED., .F., .F. ) 
 B_SPLINE_CURVE_WITH_KNOTS ( ( 4, 4 ),
 ( 0.4074455897393676751, 0.5000000000000000000 ),
 .UNSPECIFIED. ) 
 CURVE ( )  GEOMETRIC_REPRESENTATION_ITEM ( )  RATIONAL_B_SPLINE_CURVE ( ( 0.6983129098260865142, 0.7760317562606877662, 0.8765941196519909662, 0.9999999999999924505 ) ) 
 REPRESENTATION_ITEM ( '' )  );
#22396=ORIENTED_EDGE ( 'NONE', *, *, #16694, .F. ) ;
#22397=CARTESIAN_POINT ( 'NONE',  ( -12.76547314785493192, -9.517330534081262172, 74.60450883341005124 ) ) ;
#22398=ADVANCED_FACE ( 'NONE', ( #41879 ), #34720, .T. ) ;
#22399=DIRECTION ( 'NONE',  ( 0.2122660683108583690, -0.9772119095896469876, 7.504255179194988334E-08 ) ) ;
#22400=DIRECTION ( 'NONE',  ( 7.404863042181874502E-06, -6.320720312887485007E-06, 0.9999999999526082428 ) ) ;
#22402=( BOUNDED_CURVE ( )  B_SPLINE_CURVE ( 3, ( #6901, #25608, #44347, #10599 ),
 .UNSPECIFIED., .F., .F. ) 
 B_SPLINE_CURVE_WITH_KNOTS ( ( 4, 4 ),
 ( 0.9074455897393601811, 1.000000000000000000 ),
 .UNSPECIFIED. ) 
 CURVE ( )  GEOMETRIC_REPRESENTATION_ITEM ( )  RATIONAL_B_SPLINE_CURVE ( ( 0.6983129098260714152, 0.7760317562606795505, 0.8765941196519890788, 1.000000000000000000 ) ) 
 REPRESENTATION_ITEM ( '' )  );
#22404=EDGE_LOOP ( 'NONE', ( #36146, #44483 ) ) ;
#22405=ADVANCED_FACE ( 'NONE', ( #20185 ), #1221, .T. ) ;
#22408=CARTESIAN_POINT ( 'NONE',  ( -10.61357140615669792, -13.19155887971477448, 71.50828586566468914 ) ) ;
#22409=CARTESIAN_POINT ( 'NONE',  ( -15.33251096848727002, -21.95963115018486533, 72.15301311573767862 ) ) ;
#22410=LINE ( 'NONE', #4197, #21736 ) ;
#22411=B_SPLINE_CURVE_WITH_KNOTS ( 'NONE', 3,
 ( #30287, #30044, #45550, #965, #19680, #15467, #22903, #26830, #41850, #37641 ),
 .UNSPECIFIED., .F., .F.,
 ( 4, 2, 2, 2, 4 ),
 ( 0.1272669073658187489, 0.2522669073463080780, 0.3772669073267974627, 0.5022669073072867363, 0.6272669072877761209 ),
 .UNSPECIFIED. ) ;
#22412=ORIENTED_EDGE ( 'NONE', *, *, #10241, .F. ) ;
#22415=CARTESIAN_POINT ( 'NONE',  ( -22.14090652532222236, -20.04928072148792495, 62.51967078134249078 ) ) ;
#22417=CARTESIAN_POINT ( 'NONE',  ( -24.41089624436030547, -15.77327213725850719, 65.94836039739031719 ) ) ;
#22418=ORIENTED_EDGE ( 'NONE', *, *, #43731, .T. ) ;
#22420=ADVANCED_FACE ( 'NONE', ( #31037 ), #46051, .T. ) ;
#22421=ORIENTED_EDGE ( 'NONE', *, *, #8427, .F. ) ;
#22422=CARTESIAN_POINT ( 'NONE',  ( -23.77946760588002562, -10.92150643066187143, 73.50046759018312059 ) ) ;
#22424=ORIENTED_EDGE ( 'NONE', *, *, #35235, .F. ) ;
#22425=CARTESIAN_POINT ( 'NONE',  ( -13.54792730259346456, -8.920061342218058797, 57.25495614889487683 ) ) ;
#22426=EDGE_CURVE ( 'NONE', #19220, #34107, #10328, .T. ) ;
#22428=CARTESIAN_POINT ( 'NONE',  ( -24.40658474706614101, -15.78251040532600769, 69.68307488409816131 ) ) ;
#22430=CARTESIAN_POINT ( 'NONE',  ( -21.42336380182764088, -21.09487415076890215, 69.23945570945444672 ) ) ;
#22432=DIRECTION ( 'NONE',  ( -0.6621635203543606574, -0.7493593746073508033, -2.316976118889527729E-08 ) ) ;
#22433=ORIENTED_EDGE ( 'NONE', *, *, #9889, .F. ) ;
#22434=CARTESIAN_POINT ( 'NONE',  ( -12.16006207029921171, -10.11953296189675733, 64.02914329232321222 ) ) ;
#22435=DIRECTION ( 'NONE',  ( -0.8743548079231422410, -0.4852872034802500067, 5.778319183281968808E-08 ) ) ;
#22436=CARTESIAN_POINT ( 'NONE',  ( -18.26342096751342581, -21.75870509638779993, 65.53635344041087762 ) ) ;
#22440=PLANE ( 'NONE',  #13209 ) ;
#22441=DIRECTION ( 'NONE',  ( -5.731567514496413899E-31, -1.020425574103664789E-16, -1.000000000000000000 ) ) ;
#22444=EDGE_LOOP ( 'NONE', ( #22698, #3351, #33346, #26202 ) ) ;
#22445=ORIENTED_EDGE ( 'NONE', *, *, #31345, .T. ) ;
#22446=CARTESIAN_POINT ( 'NONE',  ( -23.96044199021409327, -11.23292130238350772, 66.53559200982742539 ) ) ;
#22448=ORIENTED_EDGE ( 'NONE', *, *, #32541, .F. ) ;
#22449=B_SPLINE_CURVE_WITH_KNOTS ( 'NONE', 3,
 ( #2052, #25198, #32805, #21263, #2546, #44175, #10424, #17051, #24950, #36013 ),
 .UNSPECIFIED., .F., .F.,
 ( 4, 2, 2, 2, 4 ),
 ( 0.1272669073658731220, 0.2522669073439754439, 0.3772669073220777936, 0.5022669073001800877, 0.6272669072782823818 ),
 .UNSPECIFIED. ) ;
#22450=CARTESIAN_POINT ( 'NONE',  ( -15.35027035934970918, -7.653577032698213323, 74.26481056556292515 ) ) ;
#22451=CARTESIAN_POINT ( 'NONE',  ( -18.01624426275133217, -7.780493777692311319, 60.17240823276083006 ) ) ;
#22453=CARTESIAN_POINT ( 'NONE',  ( -21.82220603157065497, -9.299244845878236632, 63.49153740581677141 ) ) ;
#22454=CARTESIAN_POINT ( 'NONE',  ( -14.54324430907851173, -21.67975036377454501, 58.42263788831355953 ) ) ;
#22455=FACE_BOUND ( 'NONE', #4268, .T. ) ;
#22456=CARTESIAN_POINT ( 'NONE',  ( -19.56876505180931147, -21.94388403446443903, 62.10165325708241113 ) ) ;
#22457=CARTESIAN_POINT ( 'NONE',  ( -23.33263663379104713, -18.66181210963279469, 72.85548507352433489 ) ) ;
#22460=ADVANCED_FACE ( 'NONE', ( #22935 ), #42361, .T. ) ;
#22461=ORIENTED_EDGE ( 'NONE', *, *, #30013, .F. ) ;
#22463=CARTESIAN_POINT ( 'NONE',  ( -15.54561766592941119, -8.065849124998859310, 74.07985694182616498 ) ) ;
#22465=FACE_OUTER_BOUND ( 'NONE', #34808, .T. ) ;
#22467=CARTESIAN_POINT ( 'NONE',  ( -23.63568631841604883, -11.45792465866591137, 73.50626392806049125 ) ) ;
#22469=ORIENTED_EDGE ( 'NONE', *, *, #7382, .T. ) ;
#22471=VERTEX_POINT ( 'NONE', #4439 ) ;
#22473=CARTESIAN_POINT ( 'NONE',  ( -23.56007973304975422, -19.03440283107118347, 66.02400637107398040 ) ) ;
#22475=VECTOR ( 'NONE', #21196, 1000.000000000000000 ) ;
#22476=CARTESIAN_POINT ( 'NONE',  ( -10.81484411697162962, -17.11524594140972155, 61.15743118925659161 ) ) ;
#22477=CARTESIAN_POINT ( 'NONE',  ( -15.86788899160417721, -21.69347836327019863, 58.43018749706013182 ) ) ;
#22478=ORIENTED_EDGE ( 'NONE', *, *, #19034, .T. ) ;
#22480=CARTESIAN_POINT ( 'NONE',  ( -21.87646569334848579, -9.342856855644162906, 63.19713549603849145 ) ) ;
#22481=VERTEX_POINT ( 'NONE', #15497 ) ;
#22482=B_SPLINE_CURVE_WITH_KNOTS ( 'NONE', 3,
 ( #3811, #14601, #4301, #26460, #41228, #18826, #15599, #22781, #11682, #367 ),
 .UNSPECIFIED., .F., .F.,
 ( 4, 2, 2, 2, 4 ),
 ( 0.1272669073658803385, 0.2522669073463614797, 0.3772669073268426487, 0.5022669073073238177, 0.6272669072878049867 ),
 .UNSPECIFIED. ) ;
#22483=CARTESIAN_POINT ( 'NONE',  ( -15.12068013687281187, -21.47611964231171200, 61.84420477127756044 ) ) ;
#22484=CARTESIAN_POINT ( 'NONE',  ( -23.93244371613987553, -17.39065613319298009, 69.52412788448918946 ) ) ;
#22485=VERTEX_POINT ( 'NONE', #34464 ) ;
#22486=FACE_OUTER_BOUND ( 'NONE', #47450, .T. ) ;
#22488=CARTESIAN_POINT ( 'NONE',  ( -16.65185932245351452, -21.81708442718849383, 65.51092266128213737 ) ) ;
#22490=CARTESIAN_POINT ( 'NONE',  ( -10.61330258792943226, -12.98832159324075874, 68.03832347271723791 ) ) ;
#22492=CARTESIAN_POINT ( 'NONE',  ( -24.45201643071094111, -14.25170847814747255, 69.65275273439885950 ) ) ;
#22493=CARTESIAN_POINT ( 'NONE',  ( -11.77169535943213319, -10.59578862612641714, 74.73885051658085388 ) ) ;
#22494=CARTESIAN_POINT ( 'NONE',  ( -23.92991418586306906, -17.39300562425996333, 65.94357246486060831 ) ) ;
#22496=CARTESIAN_POINT ( 'NONE',  ( -10.61707248396235315, -11.78131495581930999, 74.60194320761131337 ) ) ;
#22498=CARTESIAN_POINT ( 'NONE',  ( -18.50932031946840439, -21.77517977232111690, 72.43510940650374152 ) ) ;
#22499=EDGE_CURVE ( 'NONE', #6775, #2848, #5175, .T. ) ;
#22502=EDGE_LOOP ( 'NONE', ( #12266, #41573, #40835, #22881, #1144 ) ) ;
#22503=EDGE_CURVE ( 'NONE', #45493, #17650, #6232, .T. ) ;
#22504=CARTESIAN_POINT ( 'NONE',  ( -17.56236230286711475, -7.756850561809762290, 60.08060705895821485 ) ) ;
#22507=CARTESIAN_POINT ( 'NONE',  ( -11.34298429649192386, -19.11328791028677898, 68.37722950534919164 ) ) ;
#22509=CARTESIAN_POINT ( 'NONE',  ( -22.57893663749957369, -9.999394138389961384, 73.49633153340955971 ) ) ;
#22511=EDGE_LOOP ( 'NONE', ( #2652, #334, #8054, #29621, #20459 ) ) ;
#22512=DIRECTION ( 'NONE',  ( -0.2696806815386156297, 0.9629498065864429135, 3.780696488502153947E-18 ) ) ;
#22513=AXIS2_PLACEMENT_3D ( 'NONE', #11333, #33461, #497 ) ;
#22515=CARTESIAN_POINT ( 'NONE',  ( -10.70034868013728691, -12.85632356314325264, 67.84905489101299736 ) ) ;
#22516=EDGE_CURVE ( 'NONE', #14163, #32753, #34997, .T. ) ;
#22519=CARTESIAN_POINT ( 'NONE',  ( -18.84997077804804988, -7.496759192315632703, 70.51034705133518798 ) ) ;
#22520=PLANE ( 'NONE',  #28480 ) ;
#22521=CARTESIAN_POINT ( 'NONE',  ( -24.85359113602694237, -14.25571898851532460, 69.76779851910008290 ) ) ;
#22522=CARTESIAN_POINT ( 'NONE',  ( -19.61601503992405071, -21.50980213996393786, 65.76486213821362981 ) ) ;
#22526=CARTESIAN_POINT ( 'NONE',  ( -23.00442008925062254, -19.11762375203660724, 59.18410642057862248 ) ) ;
#22527=CARTESIAN_POINT ( 'NONE',  ( -19.30272045617997634, -8.014115550771091279, 59.96092997145631642 ) ) ;
#22528=( BOUNDED_CURVE ( )  B_SPLINE_CURVE ( 3, ( #101, #29637, #11406, #22493 ),
 .UNSPECIFIED., .F., .F. ) 
 B_SPLINE_CURVE_WITH_KNOTS ( ( 4, 4 ),
 ( 0.5000000000000000000, 0.9074455897393649551 ),
 .UNSPECIFIED. ) 
 CURVE ( )  GEOMETRIC_REPRESENTATION_ITEM ( )  RATIONAL_B_SPLINE_CURVE ( ( 1.000000000000030198, 0.4567392136813385184, 0.3561768502900115041, 0.6983129098260819623 ) ) 
 REPRESENTATION_ITEM ( '' )  );
#22531=CARTESIAN_POINT ( 'NONE',  ( -16.71219879347879100, -22.22520166962337740, 68.81065243885818461 ) ) ;
#22532=CARTESIAN_POINT ( 'NONE',  ( -15.55171133418867235, -7.598245370416885969, 70.79485226425863686 ) ) ;
#22533=FACE_OUTER_BOUND ( 'NONE', #34411, .T. ) ;
#22534=ADVANCED_FACE ( 'NONE', ( #43078 ), #32000, .T. ) ;
#22536=CARTESIAN_POINT ( 'NONE',  ( -14.83274962301728195, -7.824406256316001951, 56.99999999999994316 ) ) ;
#22537=( BOUNDED_CURVE ( )  B_SPLINE_CURVE ( 3, ( #40196, #6469, #28629, #13583 ),
 .UNSPECIFIED., .F., .F. ) 
 B_SPLINE_CURVE_WITH_KNOTS ( ( 4, 4 ),
 ( 0.4074455897393632342, 0.5000000000000000000 ),
 .UNSPECIFIED. ) 
 CURVE ( )  GEOMETRIC_REPRESENTATION_ITEM ( )  RATIONAL_B_SPLINE_CURVE ( ( 0.6983129098260907330, 0.7760317562606838804, 0.8765941196519834167, 0.9999999999999804601 ) ) 
 REPRESENTATION_ITEM ( '' )  );
#22539=AXIS2_PLACEMENT_3D ( 'NONE', #736, #37908, #4194 ) ;
#22540=ORIENTED_EDGE ( 'NONE', *, *, #41920, .T. ) ;
#22541=CARTESIAN_POINT ( 'NONE',  ( -12.59071586039360113, -9.139687517221355861, 74.48069540779324882 ) ) ;
#22542=CARTESIAN_POINT ( 'NONE',  ( -18.30726797983150789, -21.75326897020822514, 68.81514702557041119 ) ) ;
#22543=CARTESIAN_POINT ( 'NONE',  ( -24.42397805733578409, -17.36001670251561890, 69.57373184374615960 ) ) ;
#22545=EDGE_CURVE ( 'NONE', #25448, #38352, #9206, .T. ) ;
#22546=ORIENTED_EDGE ( 'NONE', *, *, #42961, .F. ) ;
#22547=CARTESIAN_POINT ( 'NONE',  ( -10.37871274698333046, -17.23124524545501046, 61.41389037703014964 ) ) ;
#22548=CARTESIAN_POINT ( 'NONE',  ( -15.34960817952164192, -21.96456228242026754, 72.24586663247542617 ) ) ;
#22550=CARTESIAN_POINT ( 'NONE',  ( -12.20124559944014564, -19.54486383628789170, 57.93242146526704062 ) ) ;
#22551=CARTESIAN_POINT ( 'NONE',  ( -10.08493034298069269, -16.08955231886988813, 68.17779037433831490 ) ) ;
#22554=DIRECTION ( 'NONE',  ( -0.9243256318339804212, 0.3816046728418208134, -8.614662759602032238E-09 ) ) ;
#22555=CARTESIAN_POINT ( 'NONE',  ( -18.52460027084869765, -7.842592186127370191, 70.25579138408188840 ) ) ;
#22556=DIRECTION ( 'NONE',  ( -0.6562885720885137664, 0.7545099801500437797, 1.193821363054684963E-08 ) ) ;
#22557=VERTEX_POINT ( 'NONE', #2198 ) ;
#22558=CARTESIAN_POINT ( 'NONE',  ( -13.11988144144721780, -20.89017172700268787, 58.16933213661681634 ) ) ;
#22565=EDGE_CURVE ( 'NONE', #32730, #31348, #1511, .T. ) ;
#22566=ORIENTED_EDGE ( 'NONE', *, *, #33248, .T. ) ;
#22567=CARTESIAN_POINT ( 'NONE',  ( -20.21038821853196055, -19.56678358210140800, 53.69233794759168887 ) ) ;
#22568=CARTESIAN_POINT ( 'NONE',  ( -14.93677222777187197, -21.83177888374075692, 65.21322516587865437 ) ) ;
#22570=DIRECTION ( 'NONE',  ( -0.8743548079231423520, -0.4852872034802501178, 5.778319183281970132E-08 ) ) ;
#22571=EDGE_CURVE ( 'NONE', #13964, #2446, #47402, .T. ) ;
#22572=CARTESIAN_POINT ( 'NONE',  ( -13.53742098904418079, -20.63104252237469538, 58.23753158413811803 ) ) ;
#22573=ORIENTED_EDGE ( 'NONE', *, *, #35108, .F. ) ;
#22575=ORIENTED_EDGE ( 'NONE', *, *, #42706, .T. ) ;
#22577=CARTESIAN_POINT ( 'NONE',  ( -20.31413516131974362, -8.378470924821744603, 67.06632013881642251 ) ) ;
#22579=FACE_OUTER_BOUND ( 'NONE', #15130, .T. ) ;
#22580=ADVANCED_FACE ( 'NONE', ( #44076 ), #33669, .T. ) ;
#22581=CARTESIAN_POINT ( 'NONE',  ( -21.89264518680100835, -20.26253109894388160, 58.77915004610761684 ) ) ;
#22583=CARTESIAN_POINT ( 'NONE',  ( -12.55596561939055000, -20.44876490328156393, 71.99927837297406086 ) ) ;
#22585=AXIS2_PLACEMENT_3D ( 'NONE', #3082, #29198, #44237 ) ;
#22586=ORIENTED_EDGE ( 'NONE', *, *, #25817, .T. ) ;
#22587=ORIENTED_EDGE ( 'NONE', *, *, #47945, .T. ) ;
#22588=CARTESIAN_POINT ( 'NONE',  ( -12.18170095131842068, -10.17053037870675780, 64.02914326641410980 ) ) ;
#22589=CARTESIAN_POINT ( 'NONE',  ( -11.82099675438171005, -9.899106633794131582, 64.21409753874590365 ) ) ;
#22590=DIRECTION ( 'NONE',  ( -6.885933442982639089E-06, 1.077603661691792080E-05, -0.9999999999182304089 ) ) ;
#22596=PLANE ( 'NONE',  #15421 ) ;
#22597=DIRECTION ( 'NONE',  ( -0.5540494244615012942, 0.8324837747691419265, -8.494877338007846103E-17 ) ) ;
#22598=CARTESIAN_POINT ( 'NONE',  ( -10.42302287260171312, -13.97751933429587012, 57.73352905910142852 ) ) ;
#22599=B_SPLINE_CURVE_WITH_KNOTS ( 'NONE', 3,
 ( #18005, #48065, #30099, #15281, #36960, #30347, #37444, #33259, #15038, #18496 ),
 .UNSPECIFIED., .F., .F.,
 ( 4, 2, 2, 2, 4 ),
 ( 0.000000000000000000, 0.2500000000000000000, 0.5000000000000000000, 0.7500000000000000000, 1.000000000000000000 ),
 .UNSPECIFIED. ) ;
#22600=EDGE_CURVE ( 'NONE', #23164, #8867, #37366, .T. ) ;
#22601=ORIENTED_EDGE ( 'NONE', *, *, #8216, .F. ) ;
#22603=CARTESIAN_POINT ( 'NONE',  ( -10.39215589072981416, -14.30487699944780289, 64.68803863382906627 ) ) ;
#22604=CARTESIAN_POINT ( 'NONE',  ( -21.53338499259908545, -20.54219595513480101, 72.73266144511720199 ) ) ;
#22606=CARTESIAN_POINT ( 'NONE',  ( -24.22092373047179237, -12.93688097883364208, 66.30246741375938768 ) ) ;
#22607=B_SPLINE_CURVE_WITH_KNOTS ( 'NONE', 3,
 ( #13284, #35221, #28338, #9383, #1496, #43364, #24403, #5450, #9636, #24651 ),
 .UNSPECIFIED., .F., .F.,
 ( 4, 2, 2, 2, 4 ),
 ( 0.1272669073658181105, 0.2522669073463079670, 0.3772669073267977957, 0.5022669073072876245, 0.6272669072877774532 ),
 .UNSPECIFIED. ) ;
#22609=DIRECTION ( 'NONE',  ( -0.05957303659011965041, -0.9982239494779875377, 2.515684304538401650E-08 ) ) ;
#22610=ORIENTED_EDGE ( 'NONE', *, *, #41940, .T. ) ;
#22612=VECTOR ( 'NONE', #30535, 999.9999999999998863 ) ;
#22613=AXIS2_PLACEMENT_3D ( 'NONE', #11287, #41078, #26299 ) ;
#22615=CARTESIAN_POINT ( 'NONE',  ( -10.31624708743292018, -17.04119049769829886, 57.88098858207660413 ) ) ;
#22616=CARTESIAN_POINT ( 'NONE',  ( -19.17247849636888901, -7.567181371456696226, 63.61584626116109575 ) ) ;
#22617=B_SPLINE_CURVE_WITH_KNOTS ( 'NONE', 3,
 ( #5655, #19696, #16706, #4928, #23644, #24610, #20170, #27801, #8864, #20666 ),
 .UNSPECIFIED., .F., .F.,
 ( 4, 2, 2, 2, 4 ),
 ( 0.1272669073658166949, 0.2522669073463078560, 0.3772669073267990725, 0.5022669073072902890, 0.6272669072877814500 ),
 .UNSPECIFIED. ) ;
#22620=CARTESIAN_POINT ( 'NONE',  ( -24.53826898343381302, -12.59737971884151975, 69.81597065678789704 ) ) ;
#22621=CARTESIAN_POINT ( 'NONE',  ( -20.54979551517892489, -8.489990701729437816, 63.31121512946744190 ) ) ;
#22622=EDGE_CURVE ( 'NONE', #44379, #14, #5453, .T. ) ;
#22623=ORIENTED_EDGE ( 'NONE', *, *, #43989, .T. ) ;
#22624=CARTESIAN_POINT ( 'NONE',  ( -17.89813664734472098, -21.84329158499116375, 61.87535928523301720 ) ) ;
#22625=SHAPE_REPRESENTATION ( 'Pin Studded Brass Music Cylinder', ( #29031 ), #47881 ) ;
#22626=CARTESIAN_POINT ( 'NONE',  ( -10.67159949484657488, -12.77026894434614590, 67.83012539855924672 ) ) ;
#22627=DIRECTION ( 'NONE',  ( -7.404863043337546774E-06, 6.320720317253164815E-06, -0.9999999999526082428 ) ) ;
#22628=ORIENTED_EDGE ( 'NONE', *, *, #27547, .T. ) ;
#22629=CARTESIAN_POINT ( 'NONE',  ( -19.13761704877036962, -8.022058368695287101, 63.73089277027707311 ) ) ;
#22632=CARTESIAN_POINT ( 'NONE',  ( -21.78215779604922275, -8.766813257424896477, 70.32470860997653972 ) ) ;
#22634=VERTEX_POINT ( 'NONE', #6864 ) ;
#22635=ORIENTED_EDGE ( 'NONE', *, *, #538, .F. ) ;
#22636=CARTESIAN_POINT ( 'NONE',  ( -22.86572475812252847, -14.01004878893095196, 54.07175714974878389 ) ) ;
#22637=CARTESIAN_POINT ( 'NONE',  ( -10.72456167543150229, -11.55053214535348616, 71.18886621469862064 ) ) ;
#22638=CARTESIAN_POINT ( 'NONE',  ( -23.16117746674104438, -18.90708040007733359, 62.63934749780565880 ) ) ;
#22639=EDGE_CURVE ( 'NONE', #16518, #31075, #28554, .T. ) ;
#22641=CARTESIAN_POINT ( 'NONE',  ( -20.31649760022732565, -7.943510736669368910, 70.43595667626200907 ) ) ;
#22642=CARTESIAN_POINT ( 'NONE',  ( -11.85162103594838001, -10.49015045520576983, 71.25420998615621215 ) ) ;
#22644=CARTESIAN_POINT ( 'NONE',  ( -17.19980212172655953, -7.762775302065858085, 70.79035839668003405 ) ) ;
#22648=CARTESIAN_POINT ( 'NONE',  ( -17.00410561000564513, -7.771727611841389383, 74.26018273220857679 ) ) ;
#22649=CARTESIAN_POINT ( 'NONE',  ( -12.77013062424865630, -8.927826924028671840, 53.49999999999994316 ) ) ;
#22650=EDGE_CURVE ( 'NONE', #2641, #41338, #42702, .T. ) ;
#22651=AXIS2_PLACEMENT_3D ( 'NONE', #6075, #21105, #3352 ) ;
#22652=EDGE_LOOP ( 'NONE', ( #14524, #31533, #43482, #3504, #30243 ) ) ;
#22655=EDGE_CURVE ( 'NONE', #21712, #4554, #7472, .T. ) ;
#22657=LINE ( 'NONE', #10, #46522 ) ;
#22658=CARTESIAN_POINT ( 'NONE',  ( -11.67765893934995169, -10.06753235597849461, 67.63750359946666890 ) ) ;
#22659=CARTESIAN_POINT ( 'NONE',  ( -13.81847227395522992, -21.32875440241131670, 72.06574357974443501 ) ) ;
#22661=ORIENTED_EDGE ( 'NONE', *, *, #7182, .T. ) ;
#22662=AXIS2_PLACEMENT_3D ( 'NONE', #48150, #47194, #21803 ) ;
#22663=CARTESIAN_POINT ( 'NONE',  ( -13.76849323099554567, -20.83774554052356009, 65.27156739751333703 ) ) ;
#22664=CARTESIAN_POINT ( 'NONE',  ( -14.12328906776938631, -8.570644558479624919, 67.41542347112275024 ) ) ;
#22666=CARTESIAN_POINT ( 'NONE',  ( -20.57278697373333998, -8.057206101692887756, 66.89608655064280640 ) ) ;
#22668=( BOUNDED_SURFACE ( )  B_SPLINE_SURFACE ( 3, 1, ( 
 ( #11412, #41447 ),
 ( #344, #15331 ),
 ( #30390, #25466 ),
 ( #40476, #36757 ),
 ( #18058, #48113 ),
 ( #14344, #44437 ),
 ( #6995, #10686 ) ),
 .UNSPECIFIED., .T., .F., .F. ) 
 B_SPLINE_SURFACE_WITH_KNOTS ( ( 4, 3, 4 ),
 ( 2, 2 ),
 ( 0.000000000000000000, 0.5000000000000000000, 1.000000000000000000 ),
 ( 0.000000000000000000, 1.000000000000000000 ),
 .UNSPECIFIED. ) 
 GEOMETRIC_REPRESENTATION_ITEM ( )  RATIONAL_B_SPLINE_SURFACE ( (
 ( 1.000000000000000000, 1.000000000000000000),
 ( 0.3333333333333335369, 0.3333333333333330373),
 ( 0.3333333333333335369, 0.3333333333333330373),
 ( 1.000000000000000000, 1.000000000000000000),
 ( 0.3333333333333333703, 0.3333333333333333703),
 ( 0.3333333333333333703, 0.3333333333333333703),
 ( 1.000000000000000000, 1.000000000000000000) ) ) 
 REPRESENTATION_ITEM ( '' )  SURFACE ( )  );
#22669=CARTESIAN_POINT ( 'NONE',  ( -14.75738004989435481, -8.279008875931440414, 56.85000000000044196 ) ) ;
#22671=CARTESIAN_POINT ( 'NONE',  ( -17.47591198265878631, -7.808960448257721509, 67.30422983416791283 ) ) ;
#22672=ORIENTED_EDGE ( 'NONE', *, *, #14731, .F. ) ;
#22673=CARTESIAN_POINT ( 'NONE',  ( -22.83095763869631512, -19.93459457198476770, 72.82895875648904394 ) ) ;
#22674=CARTESIAN_POINT ( 'NONE',  ( -11.28158159523816728, -11.33292898549803240, 57.36470039992773451 ) ) ;
#22676=FACE_OUTER_BOUND ( 'NONE', #474, .T. ) ;
#22677=CARTESIAN_POINT ( 'NONE',  ( -20.10030204730919223, -21.76202525863913451, 72.51983304728076973 ) ) ;
#22680=CARTESIAN_POINT ( 'NONE',  ( -10.56492523587830235, -13.18000265412059058, 71.35828586226037373 ) ) ;
#22682=B_SPLINE_CURVE_WITH_KNOTS ( 'NONE', 1,
 ( #8701, #5237 ),
 .UNSPECIFIED., .F., .F.,
 ( 2, 2 ),
 ( 0.000000000000000000, 1.000000000000000000 ),
 .UNSPECIFIED. ) ;
#22683=FACE_OUTER_BOUND ( 'NONE', #17395, .T. ) ;
#22685=CARTESIAN_POINT ( 'NONE',  ( -21.72145186077268519, -9.220171914992313589, 66.66709799741713027 ) ) ;
#22686=ORIENTED_EDGE ( 'NONE', *, *, #4988, .T. ) ;
#22687=CARTESIAN_POINT ( 'NONE',  ( -10.43358824505211224, -14.44357141193983374, 64.61477203541403469 ) ) ;
#22688=( BOUNDED_CURVE ( )  B_SPLINE_CURVE ( 3, ( #8394, #45599, #26877, #19723 ),
 .UNSPECIFIED., .F., .F. ) 
 B_SPLINE_CURVE_WITH_KNOTS ( ( 4, 4 ),
 ( 0.5000000000000000000, 0.9074455897393621795 ),
 .UNSPECIFIED. ) 
 CURVE ( )  GEOMETRIC_REPRESENTATION_ITEM ( )  RATIONAL_B_SPLINE_CURVE ( ( 0.9999999999999794609, 0.4567392136813308579, 0.3561768502900442002, 0.6983129098260970613 ) ) 
 REPRESENTATION_ITEM ( '' )  );
#22691=LINE ( 'NONE', #25406, #42375 ) ;
#22693=CARTESIAN_POINT ( 'NONE',  ( -22.38971998310932676, -20.36320860488637763, 62.41156058973809451 ) ) ;
#22694=EDGE_CURVE ( 'NONE', #43000, #43727, #45996, .T. ) ;
#22695=CARTESIAN_POINT ( 'NONE',  ( -12.01648201532752935, -10.28590752825076926, 67.64896869922044687 ) ) ;
#22696=B_SPLINE_CURVE_WITH_KNOTS ( 'NONE', 1,
 ( #45856, #8669 ),
 .UNSPECIFIED., .F., .F.,
 ( 2, 2 ),
 ( 0.000000000000000000, 1.000000000000000000 ),
 .UNSPECIFIED. ) ;
#22697=CARTESIAN_POINT ( 'NONE',  ( -16.00544582274271477, -7.903112417841744453, 63.95538887075813506 ) ) ;
#22698=ORIENTED_EDGE ( 'NONE', *, *, #18715, .F. ) ;
#22699=ORIENTED_EDGE ( 'NONE', *, *, #46810, .F. ) ;
#22700=B_SPLINE_CURVE_WITH_KNOTS ( 'NONE', 3,
 ( #15833, #30882, #45895, #12155, #27173, #42195, #38485, #4770, #31109, #34798 ),
 .UNSPECIFIED., .F., .F.,
 ( 4, 2, 2, 2, 4 ),
 ( 0.6272669072877545826, 0.7522669073072720813, 0.8772669073267895801, 1.002266907346307079, 1.127266907365824578 ),
 .UNSPECIFIED. ) ;
#22701=ADVANCED_FACE ( 'NONE', ( #29276 ), #10479, .T. ) ;
#22702=CARTESIAN_POINT ( 'NONE',  ( -11.60247201135026884, -18.79965542285971836, 61.43277710409636683 ) ) ;
#22703=CARTESIAN_POINT ( 'NONE',  ( -14.91737466579130711, -8.273365706877857662, 56.86467890717403861 ) ) ;
#22705=CARTESIAN_POINT ( 'NONE',  ( -20.99124470470196968, -21.34988281449478364, 62.25438046261486136 ) ) ;
#22708=CARTESIAN_POINT ( 'NONE',  ( -11.86732220369407997, -9.846751984446582284, 64.28560238571537866 ) ) ;
#22709=CARTESIAN_POINT ( 'NONE',  ( -10.45629970556533905, -15.48118908973361485, 57.56792791464064152 ) ) ;
#22710=CARTESIAN_POINT ( 'NONE',  ( -12.10599200002982556, -20.02663609087960239, 61.58174067880212021 ) ) ;
#22712=( BOUNDED_CURVE ( )  B_SPLINE_CURVE ( 3, ( #26168, #34696, #40932, #38631 ),
 .UNSPECIFIED., .F., .F. ) 
 B_SPLINE_CURVE_WITH_KNOTS ( ( 4, 4 ),
 ( 0.5000000000000000000, 0.9074455897393589598 ),
 .UNSPECIFIED. ) 
 CURVE ( )  GEOMETRIC_REPRESENTATION_ITEM ( )  RATIONAL_B_SPLINE_CURVE ( ( 0.9999999999999746869, 0.4567392136813389625, 0.3561768502900504729, 0.6983129098260817402 ) ) 
 REPRESENTATION_ITEM ( '' )  );
#22713=LINE ( 'NONE', #37206, #25961 ) ;
#22714=CARTESIAN_POINT ( 'NONE',  ( -10.02281612969872349, -15.66031113496680049, 61.14514897868617282 ) ) ;
#22715=CARTESIAN_POINT ( 'NONE',  ( -24.12409162043482524, -11.55122986829102238, 63.07501371131629497 ) ) ;
#22717=CARTESIAN_POINT ( 'NONE',  ( -17.74207408223254845, -7.814823900609349394, 63.73984019819800295 ) ) ;
#22719=CARTESIAN_POINT ( 'NONE',  ( -23.78676244964941233, -10.93361294341921131, 73.54688584860882372 ) ) ;
#22721=VERTEX_POINT ( 'NONE', #8573 ) ;
#22722=ORIENTED_EDGE ( 'NONE', *, *, #48107, .T. ) ;
#22724=ORIENTED_EDGE ( 'NONE', *, *, #8186, .F. ) ;
#22725=B_SPLINE_CURVE_WITH_KNOTS ( 'NONE', 3,
 ( #36934, #3218, #26611, #22422, #3457, #14504, #29563, #44594, #29326, #7668 ),
 .UNSPECIFIED., .F., .F.,
 ( 4, 2, 2, 2, 4 ),
 ( 0.6272669072877775642, 0.7522669073072877355, 0.8772669073267977957, 1.002266907346307967, 1.127266907365818138 ),
 .UNSPECIFIED. ) ;
#22731=CARTESIAN_POINT ( 'NONE',  ( -17.52853272358826686, -7.759682304905023642, 63.83584969886392457 ) ) ;
#22732=VECTOR ( 'NONE', #44173, 1000.000000000000000 ) ;
#22733=VECTOR ( 'NONE', #39151, 999.9999999999998863 ) ;
#22735=CARTESIAN_POINT ( 'NONE',  ( -11.28351140919878759, -11.44840856261519768, 64.14882000273821916 ) ) ;
#22736=CARTESIAN_POINT ( 'NONE',  ( -16.08586241947643458, -22.13815726599775857, 58.40868711133772706 ) ) ;
#22737=ORIENTED_EDGE ( 'NONE', *, *, #30824, .T. ) ;
#22738=CARTESIAN_POINT ( 'NONE',  ( -13.53844544295976249, -20.69534049476535031, 65.40117765236396963 ) ) ;
#22739=CARTESIAN_POINT ( 'NONE',  ( -17.59054788464097996, -7.361056023586105113, 63.65033409075859794 ) ) ;
#22740=B_SPLINE_CURVE_WITH_KNOTS ( 'NONE', 3,
 ( #47007, #18100, #48157, #13254, #43333, #9604, #24618, #39621, #13503, #32246 ),
 .UNSPECIFIED., .F., .F.,
 ( 4, 2, 2, 2, 4 ),
 ( 0.6272669072877842256, 0.7522669073072956181, 0.8772669073268071216, 1.002266907346318625, 1.127266907365829907 ),
 .UNSPECIFIED. ) ;
#22742=DIRECTION ( 'NONE',  ( 0.4780674886490096642, -0.8783231047267436864, -5.292596398047473452E-08 ) ) ;
#22743=CARTESIAN_POINT ( 'NONE',  ( -12.25434508901797770, -20.17367074759813406, 65.05170324716399932 ) ) ;
#22744=ORIENTED_EDGE ( 'NONE', *, *, #36988, .F. ) ;
#22746=CARTESIAN_POINT ( 'NONE',  ( -11.04141237841800560, -11.93494539390495568, 74.85840195306853673 ) ) ;
#22747=CARTESIAN_POINT ( 'NONE',  ( -17.19740490131689015, -7.362649021479085398, 70.69047035906775989 ) ) ;
#22748=ORIENTED_EDGE ( 'NONE', *, *, #26947, .T. ) ;
#22749=CARTESIAN_POINT ( 'NONE',  ( -12.79725838692604434, -20.12850099319811292, 71.80653676770127447 ) ) ;
#22750=EDGE_CURVE ( 'NONE', #27898, #23048, #16776, .T. ) ;
#22752=CARTESIAN_POINT ( 'NONE',  ( -24.30112618867181240, -13.25578303422174997, 59.64795780745660636 ) ) ;
#22754=VERTEX_POINT ( 'NONE', #4385 ) ;
#22755=CARTESIAN_POINT ( 'NONE',  ( -24.68310392741195258, -16.48564297948346891, 59.37978378043003147 ) ) ;
#22756=FACE_OUTER_BOUND ( 'NONE', #2884, .T. ) ;
#22757=CARTESIAN_POINT ( 'NONE',  ( -10.43098718212803000, -15.70539730037032911, 61.32316937334011442 ) ) ;
#22758=CARTESIAN_POINT ( 'NONE',  ( -10.38360249164154325, -14.43747963625415309, 67.87272197508832505 ) ) ;
#22760=CARTESIAN_POINT ( 'NONE',  ( -21.06702863216100496, -20.84540773593990792, 65.86981821684420879 ) ) ;
#22762=ORIENTED_EDGE ( 'NONE', *, *, #44562, .F. ) ;
#22763=B_SPLINE_CURVE_WITH_KNOTS ( 'NONE', 3,
 ( #14809, #34035, #324, #12362, #30615, #1272, #23459, #4744, #15551, #7970 ),
 .UNSPECIFIED., .F., .F.,
 ( 4, 2, 2, 2, 4 ),
 ( 0.6272669072877556928, 0.7522669073072749679, 0.8772669073267943540, 1.002266907346313740, 1.127266907365833015 ),
 .UNSPECIFIED. ) ;
#22764=EDGE_CURVE ( 'NONE', #14369, #35176, #2268, .T. ) ;
#22767=DIRECTION ( 'NONE',  ( -8.262539633966638414E-06, 9.998826072665628149E-07, 0.9999999999653652605 ) ) ;
#22769=DIRECTION ( 'NONE',  ( -5.731567514496413899E-31, -1.020425574103664789E-16, -1.000000000000000000 ) ) ;
#22771=CARTESIAN_POINT ( 'NONE',  ( -19.28939461086542906, -8.062307027802660286, 60.26092997386343342 ) ) ;
#22772=ORIENTED_EDGE ( 'NONE', *, *, #12824, .F. ) ;
#22774=VECTOR ( 'NONE', #28923, 1000.000000000000000 ) ;
#22775=CARTESIAN_POINT ( 'NONE',  ( -10.47910621644337326, -16.03883162486972935, 64.39282756246913664 ) ) ;
#22777=VERTEX_POINT ( 'NONE', #26806 ) ;
#22780=CARTESIAN_POINT ( 'NONE',  ( -10.99668346656864060, -11.04197136062318307, 60.72239829427679325 ) ) ;
#22781=CARTESIAN_POINT ( 'NONE',  ( -24.80433737800517591, -15.82637729575692553, 69.73296257493650785 ) ) ;
#22784=EDGE_LOOP ( 'NONE', ( #39289, #24666, #41640, #23776, #35886 ) ) ;
#22787=ADVANCED_FACE ( 'NONE', ( #41828 ), #30333, .T. ) ;
#22789=CARTESIAN_POINT ( 'NONE',  ( -23.48344415125163565, -18.41350569598871090, 73.04896097104848707 ) ) ;
#22793=EDGE_CURVE ( 'NONE', #6378, #4829, #20358, .T. ) ;
#22794=CARTESIAN_POINT ( 'NONE',  ( -16.06904075904983031, -7.890656793283918446, 63.97011029956862416 ) ) ;
#22795=CARTESIAN_POINT ( 'NONE',  ( -10.23610939720467528, -12.85046776639672039, 67.85337053980535416 ) ) ;
#22796=ADVANCED_FACE ( 'NONE', ( #46492 ), #27996, .T. ) ;
#22798=CARTESIAN_POINT ( 'NONE',  ( -11.46043946983621709, -11.04924301243271678, 57.35903212150709152 ) ) ;
#22800=DIRECTION ( 'NONE',  ( -0.9997277805376393323, 0.02333162706040292633, 9.101776391673754705E-09 ) ) ;
#22802=VERTEX_POINT ( 'NONE', #12969 ) ;
#22803=CARTESIAN_POINT ( 'NONE',  ( -14.44809130310161471, -8.473323905341505480, 67.25975083863336579 ) ) ;
#22804=CARTESIAN_POINT ( 'NONE',  ( -13.62243047842596866, -8.871999776185514719, 56.96967785305174203 ) ) ;
#22807=ADVANCED_FACE ( 'NONE', ( #2384 ), #1661, .F. ) ;
#22809=CARTESIAN_POINT ( 'NONE',  ( -17.98584054083101691, -22.23808389992613499, 62.06031238270200845 ) ) ;
#22811=CARTESIAN_POINT ( 'NONE',  ( -22.79909142865265537, -19.96788931561671276, 72.84411743013269813 ) ) ;
#22812=CARTESIAN_POINT ( 'NONE',  ( -13.06813783877040791, -9.265530354883376063, 67.66470656304637998 ) ) ;
#22813=FACE_OUTER_BOUND ( 'NONE', #11435, .T. ) ;
#22815=CARTESIAN_POINT ( 'NONE',  ( -23.12302852889638061, -18.95946475466559633, 62.65406880579606508 ) ) ;
#22816=CARTESIAN_POINT ( 'NONE',  ( -18.57335281209669375, -21.76520412651811043, 72.57038810541313012 ) ) ;
#22818=FACE_BOUND ( 'NONE', #31512, .T. ) ;
#22820=ORIENTED_EDGE ( 'NONE', *, *, #41809, .F. ) ;
#22823=CARTESIAN_POINT ( 'NONE',  ( -10.55151208239364635, -17.68521041179895548, 68.28217381303441869 ) ) ;
#22825=EDGE_LOOP ( 'NONE', ( #9547, #44011, #22834, #37858, #34799 ) ) ;
#22826=CARTESIAN_POINT ( 'NONE',  ( -10.44202790750644461, -14.30845231023897846, 64.38803863533676974 ) ) ;
#22828=CARTESIAN_POINT ( 'NONE',  ( -12.28110106126006507, -10.05819346760517341, 64.13987352327488622 ) ) ;
#22829=CARTESIAN_POINT ( 'NONE',  ( -17.40545348791034286, -7.756229321676927135, 70.90524440011041918 ) ) ;
#22832=CARTESIAN_POINT ( 'NONE',  ( -10.98345768875619832, -17.55129762975471408, 68.38256636668904775 ) ) ;
#22833=ORIENTED_EDGE ( 'NONE', *, *, #20870, .T. ) ;
#22834=ORIENTED_EDGE ( 'NONE', *, *, #21080, .F. ) ;
#22836=CARTESIAN_POINT ( 'NONE',  ( -15.46105799208929454, -21.99670631207736449, 72.15920124769014876 ) ) ;
#22839=CARTESIAN_POINT ( 'NONE',  ( -24.82750195234013191, -13.97654432178796569, 73.30766915316792165 ) ) ;
#22840=CARTESIAN_POINT ( 'NONE',  ( -10.03092739215081686, -13.89030502949973567, 57.64099168746837165 ) ) ;
#22841=EDGE_CURVE ( 'NONE', #7586, #10306, #19757, .T. ) ;
#22842=( BOUNDED_CURVE ( )  B_SPLINE_CURVE ( 3, ( #46565, #31280, #42629, #38909 ),
 .UNSPECIFIED., .F., .F. ) 
 B_SPLINE_CURVE_WITH_KNOTS ( ( 4, 4 ),
 ( 0.000000000000000000, 0.4074455897393638448 ),
 .UNSPECIFIED. ) 
 CURVE ( )  GEOMETRIC_REPRESENTATION_ITEM ( )  RATIONAL_B_SPLINE_CURVE ( ( 1.000000000000000000, 0.4567392136813312464, 0.3561768502900300448, 0.6983129098260963952 ) ) 
 REPRESENTATION_ITEM ( '' )  );
#22845=CARTESIAN_POINT ( 'NONE',  ( -12.50201028167747275, -20.40183342018594814, 71.92936770876625019 ) ) ;
#22849=CARTESIAN_POINT ( 'NONE',  ( -24.82492784865917201, -15.66438054851105832, 73.25949685721523963 ) ) ;
#22850=ADVANCED_FACE ( 'NONE', ( #9302 ), #47301, .T. ) ;
#22851=DIRECTION ( 'NONE',  ( -5.255974128148611414E-06, 1.684062796621483993E-06, 0.9999999999847694054 ) ) ;
#22853=CARTESIAN_POINT ( 'NONE',  ( -19.60046790782316251, -21.46228069541063732, 65.46486213989528835 ) ) ;
#22854=EDGE_LOOP ( 'NONE', ( #3572, #894 ) ) ;
#22856=( BOUNDED_CURVE ( )  B_SPLINE_CURVE ( 3, ( #13427, #36076, #24300, #9525 ),
 .UNSPECIFIED., .F., .F. ) 
 B_SPLINE_CURVE_WITH_KNOTS ( ( 4, 4 ),
 ( 0.9074455897393604031, 1.000000000000000000 ),
 .UNSPECIFIED. ) 
 CURVE ( )  GEOMETRIC_REPRESENTATION_ITEM ( )  RATIONAL_B_SPLINE_CURVE ( ( 0.6983129098260820733, 0.7760317562606887654, 0.8765941196519947409, 1.000000000000000000 ) ) 
 REPRESENTATION_ITEM ( '' )  );
#22859=DIRECTION ( 'NONE',  ( 0.9974380310868018462, 0.07153582418399356824, -3.008056593457534435E-08 ) ) ;
#22860=CARTESIAN_POINT ( 'NONE',  ( -15.42710743425593733, -21.51837058719337037, 68.64880986307761646 ) ) ;
#22862=PLANE ( 'NONE',  #45688 ) ;
#22863=EDGE_CURVE ( 'NONE', #1260, #48343, #43824, .T. ) ;
#22864=VERTEX_POINT ( 'NONE', #14578 ) ;
#22865=CARTESIAN_POINT ( 'NONE',  ( -20.32351072818673288, -7.946504961695468161, 70.44374510728370353 ) ) ;
#22875=CARTESIAN_POINT ( 'NONE',  ( -10.52210740440793124, -15.97650391503338874, 64.69874700433834391 ) ) ;
#22877=ORIENTED_EDGE ( 'NONE', *, *, #2986, .F. ) ;
#22881=ORIENTED_EDGE ( 'NONE', *, *, #4853, .F. ) ;
#22883=PLANE ( 'NONE',  #25528 ) ;
#22884=CARTESIAN_POINT ( 'NONE',  ( -18.61375994297531378, -22.16373410720964543, 72.46227804786110482 ) ) ;
#22885=ORIENTED_EDGE ( 'NONE', *, *, #429, .T. ) ;
#22886=CARTESIAN_POINT ( 'NONE',  ( -21.38163477318978423, -20.58317637574389991, 72.80981012061528190 ) ) ;
#22888=CARTESIAN_POINT ( 'NONE',  ( -11.43178109911094431, -11.19077805147660065, 57.28191156135590489 ) ) ;
#22889=ORIENTED_EDGE ( 'NONE', *, *, #41035, .T. ) ;
#22890=CARTESIAN_POINT ( 'NONE',  ( -19.09949158415725634, -8.012660229328147921, 63.43089235425713923 ) ) ;
#22894=ORIENTED_EDGE ( 'NONE', *, *, #33030, .T. ) ;
#22895=CARTESIAN_POINT ( 'NONE',  ( -22.75923595801102550, -10.27751167601812909, 66.54182257657851096 ) ) ;
#22897=B_SPLINE_CURVE_WITH_KNOTS ( 'NONE', 1,
 ( #37348, #3635 ),
 .UNSPECIFIED., .F., .F.,
 ( 2, 2 ),
 ( 0.000000000000000000, 1.000000000000000000 ),
 .UNSPECIFIED. ) ;
#22899=FACE_OUTER_BOUND ( 'NONE', #14294, .T. ) ;
#22901=CARTESIAN_POINT ( 'NONE',  ( -10.42302287260171312, -13.97751933429587012, 57.73352905910142852 ) ) ;
#22902=ADVANCED_FACE ( 'NONE', ( #4275 ), #30621, .T. ) ;
#22903=CARTESIAN_POINT ( 'NONE',  ( -12.13611197186221524, -9.561363708614054602, 57.28946728381664855 ) ) ;
#22904=CARTESIAN_POINT ( 'NONE',  ( -16.99405130501816075, -7.371615963843898278, 74.06044024557584748 ) ) ;
#22906=ORIENTED_EDGE ( 'NONE', *, *, #27691, .T. ) ;
#22908=LINE ( 'NONE', #11558, #22612 ) ;
#22909=VECTOR ( 'NONE', #34120, 1000.000000000000000 ) ;
#22910=CARTESIAN_POINT ( 'NONE',  ( -10.02813348864759035, -13.91211103331672483, 57.60858365818264559 ) ) ;
#22911=CARTESIAN_POINT ( 'NONE',  ( -23.88415222675040184, -17.63235122089636775, 62.47360984996718258 ) ) ;
#22912=AXIS2_PLACEMENT_3D ( 'NONE', #12420, #16591, #23768 ) ;
#22913=EDGE_LOOP ( 'NONE', ( #36399, #34993, #2382, #32509, #7782 ) ) ;
#22915=CARTESIAN_POINT ( 'NONE',  ( -19.89647106316203562, -21.35805615853005435, 69.18000941309762197 ) ) ;
#22916=ADVANCED_FACE ( 'NONE', ( #17629 ), #3560, .T. ) ;
#22917=CARTESIAN_POINT ( 'NONE',  ( -22.83095840648717711, -19.93459376977450859, 72.82895984417613988 ) ) ;
#22918=PLANE ( 'NONE',  #506 ) ;
#22919=EDGE_CURVE ( 'NONE', #7972, #35214, #7989, .T. ) ;
#22921=CARTESIAN_POINT ( 'NONE',  ( -23.54764978442466727, -11.41761097281034409, 66.64887858452939895 ) ) ;
#22922=ADVANCED_FACE ( 'NONE', ( #33804 ), #8615, .T. ) ;
#22923=CARTESIAN_POINT ( 'NONE',  ( -22.97645422746545663, -19.15384556476019995, 58.88970445631586159 ) ) ;
#22924=VECTOR ( 'NONE', #6070, 1000.000000000000114 ) ;
#22925=ORIENTED_EDGE ( 'NONE', *, *, #44676, .F. ) ;
#22926=CARTESIAN_POINT ( 'NONE',  ( -10.37818569806566948, -17.22973468411262132, 61.27247807055057649 ) ) ;
#22927=CARTESIAN_POINT ( 'NONE',  ( -17.66159697976433307, -21.85550285805611637, 58.42025434932890704 ) ) ;
#22928=EDGE_CURVE ( 'NONE', #47072, #34499, #22402, .T. ) ;
#22929=CARTESIAN_POINT ( 'NONE',  ( -14.97188219925329378, -8.199429090594037461, 56.84999999999995168 ) ) ;
#22930=ORIENTED_EDGE ( 'NONE', *, *, #32405, .T. ) ;
#22934=B_SPLINE_CURVE_WITH_KNOTS ( 'NONE', 3,
 ( #21846, #25311, #40322, #36129, #28524, #17657, #47479, #25538, #14419, #28755 ),
 .UNSPECIFIED., .F., .F.,
 ( 4, 2, 2, 2, 4 ),
 ( 0.000000000000000000, 0.2500000000000000000, 0.5000000000000000000, 0.7500000000000000000, 1.000000000000000000 ),
 .UNSPECIFIED. ) ;
#22935=FACE_OUTER_BOUND ( 'NONE', #4441, .T. ) ;
#22936=CARTESIAN_POINT ( 'NONE',  ( -11.35070632453979478, -11.22329048540824559, 57.09414325051740491 ) ) ;
#22938=CARTESIAN_POINT ( 'NONE',  ( -16.52316554273587101, -21.80170452179945073, 65.24036514508233608 ) ) ;
#22941=AXIS2_PLACEMENT_3D ( 'NONE', #44937, #22769, #3304 ) ;
#22942=CARTESIAN_POINT ( 'NONE',  ( -11.35825037048775066, -11.21643016533577075, 60.67885780704619947 ) ) ;
#22944=CARTESIAN_POINT ( 'NONE',  ( -10.55151208239364635, -17.68521041179895548, 68.28217381303441869 ) ) ;
#22945=CARTESIAN_POINT ( 'NONE',  ( -13.37591485149932602, -8.555017749724795451, 57.16956523174690119 ) ) ;
#22946=VERTEX_POINT ( 'NONE', #37156 ) ;
#22949=CARTESIAN_POINT ( 'NONE',  ( -13.41327670018355001, -20.54622194888242603, 58.34650078082590596 ) ) ;
#22950=CARTESIAN_POINT ( 'NONE',  ( -18.71756812234623979, -7.929749856837892352, 70.67068030594712980 ) ) ;
#22951=CARTESIAN_POINT ( 'NONE',  ( -24.21188451782586881, -13.09817894282342898, 63.13264126965447076 ) ) ;
#22952=ORIENTED_EDGE ( 'NONE', *, *, #27239, .T. ) ;
#22954=PLANE ( 'NONE',  #26705 ) ;
#22955=CARTESIAN_POINT ( 'NONE',  ( -10.34189029804177906, -12.49727573565278504, 60.99842349757105353 ) ) ;
#22956=VERTEX_POINT ( 'NONE', #29549 ) ;
#22958=AXIS2_PLACEMENT_3D ( 'NONE', #36143, #10547, #9825 ) ;
#22959=DIRECTION ( 'NONE',  ( -7.130145686836404013E-06, 1.088473443322539125E-05, 0.9999999999153418306 ) ) ;
#22960=CARTESIAN_POINT ( 'NONE',  ( -23.00454255336054743, -10.50046069577333441, 59.88731295783226471 ) ) ;
#22961=CARTESIAN_POINT ( 'NONE',  ( -13.38462805196022565, -20.58720062598995426, 58.34650077712429095 ) ) ;
#22962=ADVANCED_FACE ( 'NONE', ( #6662 ), #21917, .T. ) ;
#22963=CARTESIAN_POINT ( 'NONE',  ( -23.55811799921815819, -19.03726020201580837, 65.92415190940894831 ) ) ;
#22964=CARTESIAN_POINT ( 'NONE',  ( -22.37985683132060188, -19.82347751554591753, 69.47417989525709459 ) ) ;
#22969=CARTESIAN_POINT ( 'NONE',  ( -21.59804182614902146, -20.98026282434625500, 72.70941811628220819 ) ) ;
#22972=ORIENTED_EDGE ( 'NONE', *, *, #48322, .T. ) ;
#22976=ORIENTED_EDGE ( 'NONE', *, *, #10858, .F. ) ;
#22977=CARTESIAN_POINT ( 'NONE',  ( -14.72778360411233045, -21.32322305517535099, 58.31617885012778402 ) ) ;
#22979=CARTESIAN_POINT ( 'NONE',  ( -10.03884236986523604, -13.82852981289494210, 57.70470977341523167 ) ) ;
#22980=( BOUNDED_CURVE ( )  B_SPLINE_CURVE ( 3, ( #29250, #44286, #25546, #6838 ),
 .UNSPECIFIED., .F., .F. ) 
 B_SPLINE_CURVE_WITH_KNOTS ( ( 4, 4 ),
 ( 0.5000000000000000000, 0.9074455897393668424 ),
 .UNSPECIFIED. ) 
 CURVE ( )  GEOMETRIC_REPRESENTATION_ITEM ( )  RATIONAL_B_SPLINE_CURVE ( ( 1.000000000000035083, 0.4567392136813309134, 0.3561768502900051203, 0.6983129098260960621 ) ) 
 REPRESENTATION_ITEM ( '' )  );
#22981=ADVANCED_FACE ( 'NONE', ( #12895 ), #7158, .F. ) ;
#22983=CARTESIAN_POINT ( 'NONE',  ( -17.05968203966123298, -22.25103879409192231, 72.27887915399999486 ) ) ;
#22984=VERTEX_POINT ( 'NONE', #18212 ) ;
#22985=EDGE_CURVE ( 'NONE', #20660, #40480, #27151, .T. ) ;
#22986=CARTESIAN_POINT ( 'NONE',  ( -13.99679447977218061, -20.97040113148658591, 71.94079819673058296 ) ) ;
#22987=CARTESIAN_POINT ( 'NONE',  ( -9.990608257894338706, -8.638304610707185915, 54.49999999999995026 ) ) ;
#22988=ORIENTED_EDGE ( 'NONE', *, *, #5735, .F. ) ;
#22989=CARTESIAN_POINT ( 'NONE',  ( -22.33041777183100507, -20.41561037748852669, 62.34943743628787161 ) ) ;
#22990=AXIS2_PLACEMENT_3D ( 'NONE', #46250, #4894, #40010 ) ;
#22991=( BOUNDED_SURFACE ( )  B_SPLINE_SURFACE ( 3, 1, ( 
 ( #36358, #22086 ),
 ( #36585, #2637 ),
 ( #37083, #43775 ),
 ( #47943, #47220 ),
 ( #17643, #2869 ),
 ( #21118, #29229 ),
 ( #44268, #10522 ) ),
 .UNSPECIFIED., .T., .F., .F. ) 
 B_SPLINE_SURFACE_WITH_KNOTS ( ( 4, 3, 4 ),
 ( 2, 2 ),
 ( 0.000000000000000000, 0.5000000000000000000, 1.000000000000000000 ),
 ( 0.000000000000000000, 1.000000000000000000 ),
 .UNSPECIFIED. ) 
 GEOMETRIC_REPRESENTATION_ITEM ( )  RATIONAL_B_SPLINE_SURFACE ( (
 ( 1.000000000000000000, 1.000000000000000000),
 ( 0.3333333333333335369, 0.3333333333333330373),
 ( 0.3333333333333335369, 0.3333333333333330373),
 ( 1.000000000000000000, 1.000000000000000000),
 ( 0.3333333333333333703, 0.3333333333333333703),
 ( 0.3333333333333333703, 0.3333333333333333703),
 ( 1.000000000000000000, 1.000000000000000000) ) ) 
 REPRESENTATION_ITEM ( '' )  SURFACE ( )  );
#22992=CARTESIAN_POINT ( 'NONE',  ( -23.98474799315784978, -17.25007060033011896, 69.41339792561625188 ) ) ;
#22995=CARTESIAN_POINT ( 'NONE',  ( -15.12990733413706046, -8.194132228790286021, 56.96073009183007940 ) ) ;
#22996=ORIENTED_EDGE ( 'NONE', *, *, #20532, .F. ) ;
#22997=CARTESIAN_POINT ( 'NONE',  ( -10.93436299408032752, -11.15019271687858726, 64.31028572978402735 ) ) ;
#22999=ADVANCED_FACE ( 'NONE', ( #33218 ), #35549, .T. ) ;
#23000=CARTESIAN_POINT ( 'NONE',  ( -11.57022994764690260, -10.20106918018851339, 71.06869474401152331 ) ) ;
#23002=CARTESIAN_POINT ( 'NONE',  ( -24.31477923169101629, -16.30090137217950641, 59.40860294853779777 ) ) ;
#23004=CARTESIAN_POINT ( 'NONE',  ( -20.25191534917340874, -8.350868906188830820, 70.26572394742477456 ) ) ;
#23005=ADVANCED_FACE ( 'NONE', ( #43197 ), #40650, .T. ) ;
#23006=( BOUNDED_CURVE ( )  B_SPLINE_CURVE ( 3, ( #23040, #10968, #15363, #29434 ),
 .UNSPECIFIED., .F., .F. ) 
 B_SPLINE_CURVE_WITH_KNOTS ( ( 4, 4 ),
 ( 0.5000000000000000000, 0.9074455897393631787 ),
 .UNSPECIFIED. ) 
 CURVE ( )  GEOMETRIC_REPRESENTATION_ITEM ( )  RATIONAL_B_SPLINE_CURVE ( ( 0.9999999999999653610, 0.4567392136813298587, 0.3561768502900535815, 0.6983129098260990597 ) ) 
 REPRESENTATION_ITEM ( '' )  );
#23007=CARTESIAN_POINT ( 'NONE',  ( -13.06813783877040791, -9.265530354883376063, 67.66470656304637998 ) ) ;
#23008=DIRECTION ( 'NONE',  ( -0.3478314405900310713, -0.9375570856950864451, 0.000000000000000000 ) ) ;
#23009=CARTESIAN_POINT ( 'NONE',  ( -10.49862840407593367, -15.82799419795606966, 64.80771590052736997 ) ) ;
#23011=ADVANCED_FACE ( 'NONE', ( #30306 ), #41125, .T. ) ;
#23015=CARTESIAN_POINT ( 'NONE',  ( -11.03951130610352749, -10.96966301366620478, 60.84032324715965245 ) ) ;
#23017=CARTESIAN_POINT ( 'NONE',  ( -18.37611662992575390, -7.874247802443992583, 73.94950313365406203 ) ) ;
#23019=CARTESIAN_POINT ( 'NONE',  ( -10.42546172544805039, -12.25520447285018122, 57.44362008841285672 ) ) ;
#23020=VERTEX_POINT ( 'NONE', #12062 ) ;
#23021=CARTESIAN_POINT ( 'NONE',  ( -17.98089531606498781, -21.84518143609853524, 68.95947724711012938 ) ) ;
#23022=CARTESIAN_POINT ( 'NONE',  ( -16.94458744105653381, -7.374567917109038362, 74.14513580114275726 ) ) ;
#23023=CARTESIAN_POINT ( 'NONE',  ( -10.67174875255963329, -12.96329817365894321, 68.03832382196286233 ) ) ;
#23024=ORIENTED_EDGE ( 'NONE', *, *, #22622, .T. ) ;
#23027=CARTESIAN_POINT ( 'NONE',  ( -24.54825887019308794, -12.63003870855543553, 69.92243000373970574 ) ) ;
#23029=CARTESIAN_POINT ( 'NONE',  ( -13.59466166437493762, -8.949414174231923980, 57.26967704109966917 ) ) ;
#23033=EDGE_CURVE ( 'NONE', #41432, #1105, #45432, .T. ) ;
#23034=CARTESIAN_POINT ( 'NONE',  ( -14.01837044221388417, -8.636059239884620098, 74.48482605064899076 ) ) ;
#23036=DIRECTION ( 'NONE',  ( 0.3109111061729913916, 0.9504389954427825415, 3.354176643444177759E-08 ) ) ;
#23039=CARTESIAN_POINT ( 'NONE',  ( -10.21764062494887781, -12.91954801228597915, 67.92327636273336111 ) ) ;
#23040=CARTESIAN_POINT ( 'NONE',  ( -18.44528782684011858, -21.78515541812411982, 72.29983070759432451 ) ) ;
#23041=EDGE_LOOP ( 'NONE', ( #31553, #20463, #32646, #18244, #39839 ) ) ;
#23044=CARTESIAN_POINT ( 'NONE',  ( -22.04114742393716142, -9.481025248639415537, 59.73643293354757589 ) ) ;
#23045=CARTESIAN_POINT ( 'NONE',  ( -20.22893085845381123, -8.395648538660806182, 66.85392180442863719 ) ) ;
#23046=CARTESIAN_POINT ( 'NONE',  ( -12.51522269766590512, -9.204924993125867871, 74.45776466667307147 ) ) ;
#23047=DIRECTION ( 'NONE',  ( 3.549360974554993999E-17, -6.371834667797928663E-18, -1.000000000000000000 ) ) ;
#23048=VERTEX_POINT ( 'NONE', #38144 ) ;
#23049=CARTESIAN_POINT ( 'NONE',  ( -10.87811525140410929, -17.44835992831754368, 61.31310265544169624 ) ) ;
#23050=CARTESIAN_POINT ( 'NONE',  ( -24.69336539026762267, -16.44026253781551361, 59.22308793767378177 ) ) ;
#23051=CARTESIAN_POINT ( 'NONE',  ( -15.69736699998981422, -8.025519224215527103, 70.60989840319118116 ) ) ;
#23052=CARTESIAN_POINT ( 'NONE',  ( -24.31456807776294227, -16.04512561575171503, 66.34708430620283082 ) ) ;
#23053=ORIENTED_EDGE ( 'NONE', *, *, #35383, .T. ) ;
#23054=CARTESIAN_POINT ( 'NONE',  ( -22.69786088827318338, -10.13032044058513748, 70.01738298352940149 ) ) ;
#23055=CARTESIAN_POINT ( 'NONE',  ( -17.77921064978749044, -22.25082400685520057, 58.59048811498988840 ) ) ;
#23056=CARTESIAN_POINT ( 'NONE',  ( -10.92750425249182022, -11.16255029878774252, 64.26386639478288032 ) ) ;
#23057=FACE_BOUND ( 'NONE', #9031, .T. ) ;
#23059=EDGE_CURVE ( 'NONE', #9176, #29117, #7023, .T. ) ;
#23060=EDGE_CURVE ( 'NONE', #46952, #38508, #22410, .T. ) ;
#23062=CARTESIAN_POINT ( 'NONE',  ( -10.82687744661835971, -17.29512782721398523, 64.62739381397786076 ) ) ;
#23064=CARTESIAN_POINT ( 'NONE',  ( -15.12736045941317897, -21.89643407171298151, 68.69097498501147925 ) ) ;
#23065=CARTESIAN_POINT ( 'NONE',  ( -24.83515304063678286, -14.04764234229505959, 73.23776096988058271 ) ) ;
#23066=EDGE_LOOP ( 'NONE', ( #39889, #39309, #19385, #20816, #21806 ) ) ;
#23067=CARTESIAN_POINT ( 'NONE',  ( -10.45275820844018355, -14.15883753957306546, 64.57730928593822739 ) ) ;
#23068=EDGE_LOOP ( 'NONE', ( #29370, #2046, #4864, #22906, #48537 ) ) ;
#23069=CARTESIAN_POINT ( 'NONE',  ( -14.05371385056185574, -21.00138210837564401, 72.07607703579976999 ) ) ;
#23070=CARTESIAN_POINT ( 'NONE',  ( -12.10131192688100299, -10.18592936015514816, 64.31442259820508411 ) ) ;
#23073=EDGE_CURVE ( 'NONE', #11801, #48136, #32038, .T. ) ;
#23074=CARTESIAN_POINT ( 'NONE',  ( -21.73662441638723308, -9.231682010981758779, 66.67622112302015580 ) ) ;
#23075=VERTEX_POINT ( 'NONE', #18453 ) ;
#23076=ORIENTED_EDGE ( 'NONE', *, *, #5072, .T. ) ;
#23078=CARTESIAN_POINT ( 'NONE',  ( -15.15660932275500095, -21.48492473237050859, 65.39124617759186719 ) ) ;
#23079=PLANE ( 'NONE',  #23389 ) ;
#23080=CARTESIAN_POINT ( 'NONE',  ( -15.62101046192594289, -7.580605815997546237, 70.72494447658496597 ) ) ;
#23081=CARTESIAN_POINT ( 'NONE',  ( -12.01648161716052954, -10.28590799842451098, 67.79896869921918778 ) ) ;
#23082=CARTESIAN_POINT ( 'NONE',  ( -19.30271816048872324, -8.014114901043837946, 60.26092997144682784 ) ) ;
#23083=CARTESIAN_POINT ( 'NONE',  ( -10.64854695470030599, -12.86019059820356958, 64.55364013863997741 ) ) ;
#23084=CARTESIAN_POINT ( 'NONE',  ( -10.51729421260818498, -16.22293138110306998, 71.44750383217574097 ) ) ;
#23085=ORIENTED_EDGE ( 'NONE', *, *, #12809, .F. ) ;
#23086=EDGE_LOOP ( 'NONE', ( #11790, #8841, #45093, #19270, #7001 ) ) ;
#23087=CARTESIAN_POINT ( 'NONE',  ( -24.40844971322602319, -15.79084262311724629, 73.41792560911460441 ) ) ;
#23088=ADVANCED_FACE ( 'NONE', ( #264 ), #22918, .F. ) ;
#23089=CARTESIAN_POINT ( 'NONE',  ( -11.87774890630698899, -9.834968260482170876, 64.19060820317955063 ) ) ;
#23090=CARTESIAN_POINT ( 'NONE',  ( -19.61601425152793254, -21.50980239257335569, 65.61486213821591207 ) ) ;
#23091=CARTESIAN_POINT ( 'NONE',  ( -13.54822921233619226, -20.69819393533649077, 61.51646323540209949 ) ) ;
#23092=ORIENTED_EDGE ( 'NONE', *, *, #33153, .F. ) ;
#23094=EDGE_LOOP ( 'NONE', ( #2774, #2938, #48565, #42017, #45698 ) ) ;
#23095=B_SPLINE_CURVE_WITH_KNOTS ( 'NONE', 3,
 ( #9652, #8920, #38943, #31314, #34999, #1264, #9400, #20719, #19998, #16272 ),
 .UNSPECIFIED., .F., .F.,
 ( 4, 2, 2, 2, 4 ),
 ( 0.6272669072877873342, 0.7522669073072947299, 0.8772669073268022366, 1.002266907346309743, 1.127266907365817028 ),
 .UNSPECIFIED. ) ;
#23098=AXIS2_PLACEMENT_3D ( 'NONE', #45717, #35079, #31400 ) ;
#23099=CARTESIAN_POINT ( 'NONE',  ( -15.15518245968824651, -21.43299258235331450, 68.76519962665837227 ) ) ;
#23102=CARTESIAN_POINT ( 'NONE',  ( -22.08174701096107384, -8.994662730349551438, 63.29130125984253397 ) ) ;
#23103=CARTESIAN_POINT ( 'NONE',  ( -22.78678841951795420, -19.98074385893927740, 72.75126376599935440 ) ) ;
#23105=ORIENTED_EDGE ( 'NONE', *, *, #20686, .T. ) ;
#23106=( BOUNDED_CURVE ( )  B_SPLINE_CURVE ( 3, ( #43047, #20409, #1925, #1688 ),
 .UNSPECIFIED., .F., .F. ) 
 B_SPLINE_CURVE_WITH_KNOTS ( ( 4, 4 ),
 ( 1.570796326794896558, 1.675516081914546707 ),
 .UNSPECIFIED. ) 
 CURVE ( )  GEOMETRIC_REPRESENTATION_ITEM ( )  RATIONAL_B_SPLINE_CURVE ( ( 1.000000000000000000, 0.9990863565030494442, 0.9990863565030494442, 1.000000000000000000 ) ) 
 REPRESENTATION_ITEM ( '' )  );
#23108=CARTESIAN_POINT ( 'NONE',  ( -20.14464072020449237, -7.873698051035776579, 73.82072983659610088 ) ) ;
#23109=ORIENTED_EDGE ( 'NONE', *, *, #39342, .T. ) ;
#23110=CARTESIAN_POINT ( 'NONE',  ( -10.51021933215485227, -15.90427549348945035, 64.52273984823442277 ) ) ;
#23115=EDGE_CURVE ( 'NONE', #828, #21857, #33765, .T. ) ;
#23117=CARTESIAN_POINT ( 'NONE',  ( -17.92193097897699872, -21.84160713959417421, 62.17535923543130139 ) ) ;
#23118=CARTESIAN_POINT ( 'NONE',  ( -14.26926634389775828, -8.060150775150390245, 67.36000830278645424 ) ) ;
#23121=CARTESIAN_POINT ( 'NONE',  ( -22.23346828763840222, -19.89562310515971078, 65.70421727878456863 ) ) ;
#23122=( BOUNDED_CURVE ( )  B_SPLINE_CURVE ( 3, ( #10916, #44417, #7482, #40951 ),
 .UNSPECIFIED., .F., .F. ) 
 B_SPLINE_CURVE_WITH_KNOTS ( ( 4, 4 ),
 ( 0.5000000000000000000, 0.9074455897393700621 ),
 .UNSPECIFIED. ) 
 CURVE ( )  GEOMETRIC_REPRESENTATION_ITEM ( )  RATIONAL_B_SPLINE_CURVE ( ( 1.000000000000003997, 0.4567392136813233083, 0.3561768502900242162, 0.6983129098261110501 ) ) 
 REPRESENTATION_ITEM ( '' )  );
#23123=CARTESIAN_POINT ( 'NONE',  ( -10.38078069312423679, -14.50222183502507356, 68.00800126083242958 ) ) ;
#23125=CARTESIAN_POINT ( 'NONE',  ( -12.20316607747752613, -9.493609027659992705, 57.27590782196710251 ) ) ;
#23126=ADVANCED_FACE ( 'NONE', ( #26846 ), #30059, .F. ) ;
#23127=CARTESIAN_POINT ( 'NONE',  ( -13.19711905255361195, -20.45611100226741641, 58.34650356412061001 ) ) ;
#23128=VECTOR ( 'NONE', #2514, 1000.000000000000227 ) ;
#23130=EDGE_LOOP ( 'NONE', ( #32903, #20582, #36540, #33465, #22433 ) ) ;
#23131=B_SPLINE_CURVE_WITH_KNOTS ( 'NONE', 3,
 ( #2312, #9720, #47387, #28429, #32369, #36736, #21282, #36280, #32592, #6738 ),
 .UNSPECIFIED., .F., .F.,
 ( 4, 2, 2, 2, 4 ),
 ( 0.6272669072877743446, 0.7522669073072896229, 0.8772669073268047901, 1.002266907346319957, 1.127266907365835236 ),
 .UNSPECIFIED. ) ;
#23132=EDGE_CURVE ( 'NONE', #19831, #26003, #42608, .T. ) ;
#23133=DIRECTION ( 'NONE',  ( 0.8244078399817417191, 0.5659962132175737626, 7.627400655798535667E-08 ) ) ;
#23134=CARTESIAN_POINT ( 'NONE',  ( -10.18401476999287425, -13.05278034840643286, 71.32333300961973066 ) ) ;
#23135=CARTESIAN_POINT ( 'NONE',  ( -10.72552559342236833, -12.61109755851567549, 60.94853568372188590 ) ) ;
#23137=EDGE_CURVE ( 'NONE', #31902, #5757, #2639, .T. ) ;
#23138=CARTESIAN_POINT ( 'NONE',  ( -10.61330328728660533, -12.98831903967553814, 67.73832347272892207 ) ) ;
#23139=CARTESIAN_POINT ( 'NONE',  ( -12.40421236734144728, -20.31415489762336435, 68.38011531907731921 ) ) ;
#23141=( BOUNDED_CURVE ( )  B_SPLINE_CURVE ( 3, ( #4698, #30084, #18987, #4951 ),
 .UNSPECIFIED., .F., .F. ) 
 B_SPLINE_CURVE_WITH_KNOTS ( ( 4, 4 ),
 ( 0.000000000000000000, 0.4074455897393651771 ),
 .UNSPECIFIED. ) 
 CURVE ( )  GEOMETRIC_REPRESENTATION_ITEM ( )  RATIONAL_B_SPLINE_CURVE ( ( 1.000000000000000000, 0.4567392136813308023, 0.3561768502900298783, 0.6983129098260971723 ) ) 
 REPRESENTATION_ITEM ( '' )  );
#23142=CARTESIAN_POINT ( 'NONE',  ( -10.76351158211370240, -11.46999907741044034, 67.73209273364366823 ) ) ;
#23147=CARTESIAN_POINT ( 'NONE',  ( -12.49057014363319773, -19.84541670790808965, 64.86674882886633497 ) ) ;
#23149=ORIENTED_EDGE ( 'NONE', *, *, #7241, .F. ) ;
#23150=CARTESIAN_POINT ( 'NONE',  ( -19.90352600502131963, -21.35538510417552516, 69.16997613342608986 ) ) ;
#23152=CARTESIAN_POINT ( 'NONE',  ( -15.40768640085200047, -21.98131303373579115, 72.20608812448921299 ) ) ;
#23153=CARTESIAN_POINT ( 'NONE',  ( -11.49688049385020960, -18.62690763749001732, 64.76179218520603342 ) ) ;
#23157=CARTESIAN_POINT ( 'NONE',  ( -14.61306878872958137, -8.340592061241681066, 67.67463703838096478 ) ) ;
#23158=VECTOR ( 'NONE', #20031, 1000.000000000000227 ) ;
#23159=ORIENTED_EDGE ( 'NONE', *, *, #12542, .T. ) ;
#23160=CARTESIAN_POINT ( 'NONE',  ( -24.45304548397136202, -14.21871265238332604, 66.18292724403113425 ) ) ;
#23161=CARTESIAN_POINT ( 'NONE',  ( -23.62594491300536959, -11.45603751788689451, 66.70742424642772050 ) ) ;
#23163=EDGE_LOOP ( 'NONE', ( #33243, #4749 ) ) ;
#23164=VERTEX_POINT ( 'NONE', #8622 ) ;
#23166=DIRECTION ( 'NONE',  ( 2.331190576225089612E-06, -8.511884079520847478E-06, 0.9999999999610567070 ) ) ;
#23172=CARTESIAN_POINT ( 'NONE',  ( -24.47217469780903798, -14.64471797168181233, 63.01296487297644688 ) ) ;
#23173=CARTESIAN_POINT ( 'NONE',  ( -24.20884359724224311, -11.73171579724705005, 59.59740298356196320 ) ) ;
#23174=CARTESIAN_POINT ( 'NONE',  ( -21.95939004544374740, -9.477125498926222136, 59.72171213236985921 ) ) ;
#23176=FACE_OUTER_BOUND ( 'NONE', #19892, .T. ) ;
#23179=B_SPLINE_CURVE_WITH_KNOTS ( 'NONE', 3,
 ( #24834, #4730, #39843, #28763, #20894, #12110, #9588, #8417, #32224, #45858 ),
 .UNSPECIFIED., .F., .F.,
 ( 4, 2, 2, 2, 4 ),
 ( 0.000000000000000000, 0.2500000000000000000, 0.5000000000000000000, 0.7500000000000000000, 1.000000000000000000 ),
 .UNSPECIFIED. ) ;
#23180=CARTESIAN_POINT ( 'NONE',  ( -18.58429415988738143, -7.905961439831743931, 70.59741261408042590 ) ) ;
#23182=VERTEX_POINT ( 'NONE', #9595 ) ;
#23183=ORIENTED_EDGE ( 'NONE', *, *, #26850, .T. ) ;
#23185=CARTESIAN_POINT ( 'NONE',  ( -21.46132405888245032, -9.088780516485673644, 73.71201958758717865 ) ) ;
#23186=CARTESIAN_POINT ( 'NONE',  ( -10.35661267713556022, -12.45241038966069347, 60.91358145539074798 ) ) ;
#23188=CARTESIAN_POINT ( 'NONE',  ( -18.01931865558045942, -7.780653922786444632, 60.38060830724960937 ) ) ;
#23189=PLANE ( 'NONE',  #24004 ) ;
#23191=EDGE_CURVE ( 'NONE', #38842, #15214, #22617, .T. ) ;
#23192=CARTESIAN_POINT ( 'NONE',  ( -17.35131669183886061, -7.807977842693357040, 70.60108831583485767 ) ) ;
#23193=CARTESIAN_POINT ( 'NONE',  ( -24.39823041255490921, -14.19330756662983362, 73.19441791716994317 ) ) ;
#23194=CARTESIAN_POINT ( 'NONE',  ( -19.58430998839561354, -21.93927299186879765, 62.17220519270452428 ) ) ;
#23196=VECTOR ( 'NONE', #17140, 1000.000000000000114 ) ;
#23198=EDGE_CURVE ( 'NONE', #508, #28688, #13010, .T. ) ;
#23199=CARTESIAN_POINT ( 'NONE',  ( -24.38143469521110518, -15.58083332675401067, 73.00303748421107741 ) ) ;
#23202=ADVANCED_BREP_SHAPE_REPRESENTATION ( '', ( #48318, #29031 ), #47881 ) ;
#23203=CARTESIAN_POINT ( 'NONE',  ( -24.10584550580110630, -12.56049697540380095, 73.54225570139644219 ) ) ;
#23204=CARTESIAN_POINT ( 'NONE',  ( -17.72591277258568709, -7.814435863198863075, 63.62227229162045461 ) ) ;
#23206=ADVANCED_FACE ( 'NONE', ( #13244 ), #6728, .T. ) ;
#23207=CARTESIAN_POINT ( 'NONE',  ( -23.42915847708036381, -11.11517115755410146, 73.64721174900437006 ) ) ;
#23208=ORIENTED_EDGE ( 'NONE', *, *, #9347, .F. ) ;
#23209=EDGE_LOOP ( 'NONE', ( #19190, #17530, #31411, #14842 ) ) ;
#23210=CARTESIAN_POINT ( 'NONE',  ( -20.10030308072983374, -21.76202485516048668, 72.51983413602351902 ) ) ;
#23211=ORIENTED_EDGE ( 'NONE', *, *, #37603, .T. ) ;
#23212=DIRECTION ( 'NONE',  ( 5.625773296287788022E-06, 7.100530152274343103E-06, 0.9999999999589664901 ) ) ;
#23213=CARTESIAN_POINT ( 'NONE',  ( -16.53298114947924802, -21.75231650153539675, 61.98241377463749302 ) ) ;
#23214=( BOUNDED_SURFACE ( )  B_SPLINE_SURFACE ( 3, 1, ( 
 ( #17088, #6025 ),
 ( #9247, #32137 ),
 ( #24987, #5800 ),
 ( #40005, #28197 ),
 ( #43473, #20809 ),
 ( #28451, #13397 ),
 ( #9735, #6274 ) ),
 .UNSPECIFIED., .T., .F., .F. ) 
 B_SPLINE_SURFACE_WITH_KNOTS ( ( 4, 3, 4 ),
 ( 2, 2 ),
 ( 0.000000000000000000, 0.5000000000000000000, 1.000000000000000000 ),
 ( 0.000000000000000000, 1.000000000000000000 ),
 .UNSPECIFIED. ) 
 GEOMETRIC_REPRESENTATION_ITEM ( )  RATIONAL_B_SPLINE_SURFACE ( (
 ( 1.000000000000000000, 1.000000000000000000),
 ( 0.3333333333333335369, 0.3333333333333330373),
 ( 0.3333333333333335369, 0.3333333333333330373),
 ( 1.000000000000000000, 1.000000000000000000),
 ( 0.3333333333333333703, 0.3333333333333333703),
 ( 0.3333333333333333703, 0.3333333333333333703),
 ( 1.000000000000000000, 1.000000000000000000) ) ) 
 REPRESENTATION_ITEM ( '' )  SURFACE ( )  );
#23215=B_SPLINE_CURVE_WITH_KNOTS ( 'NONE', 3,
 ( #26628, #22693, #37690, #3980, #18992, #33995, #15271, #7929, #19233, #9128 ),
 .UNSPECIFIED., .F., .F.,
 ( 4, 2, 2, 2, 4 ),
 ( 0.6272669072877684604, 0.7522669073072830725, 0.8772669073267977957, 1.002266907346312408, 1.127266907365827020 ),
 .UNSPECIFIED. ) ;
#23216=CARTESIAN_POINT ( 'NONE',  ( -13.34362782723684049, -8.575845938274239799, 57.10821201658431789 ) ) ;
#23217=LINE ( 'NONE', #82, #34033 ) ;
#23219=CARTESIAN_POINT ( 'NONE',  ( -14.23443154292173674, -21.09974595518388440, 71.81118900415394535 ) ) ;
#23220=CARTESIAN_POINT ( 'NONE',  ( -17.55954837273607438, -7.360311716977308905, 63.72773943437917410 ) ) ;
#23222=CARTESIAN_POINT ( 'NONE',  ( -10.83683317046381234, -12.44108562964681219, 57.62857332099802932 ) ) ;
#23224=DIRECTION ( 'NONE',  ( -8.560949394918188676E-06, 2.380493831898821895E-06, -0.9999999999605216905 ) ) ;
#23225=AXIS2_PLACEMENT_3D ( 'NONE', #19483, #46330, #28754 ) ;
#23226=ORIENTED_EDGE ( 'NONE', *, *, #493, .F. ) ;
#23227=DIRECTION ( 'NONE',  ( 3.549360974554993999E-17, -6.371834667797928663E-18, -1.000000000000000000 ) ) ;
#23228=CARTESIAN_POINT ( 'NONE',  ( -16.71379370341422543, -22.22534705626145879, 68.95206582789661809 ) ) ;
#23230=EDGE_LOOP ( 'NONE', ( #23770, #26948 ) ) ;
#23235=B_SPLINE_CURVE_WITH_KNOTS ( 'NONE', 3,
 ( #46978, #27302, #35163, #12519, #42328, #27544, #46515, #12768, #38868, #9576 ),
 .UNSPECIFIED., .F., .F.,
 ( 4, 2, 2, 2, 4 ),
 ( 0.000000000000000000, 0.2500000000000000000, 0.5000000000000000000, 0.7500000000000000000, 1.000000000000000000 ),
 .UNSPECIFIED. ) ;
#23237=EDGE_CURVE ( 'NONE', #48136, #2367, #46697, .T. ) ;
#23239=CARTESIAN_POINT ( 'NONE',  ( -11.07752443122393693, -17.88727437471119330, 71.77538231106770183 ) ) ;
#23240=FACE_OUTER_BOUND ( 'NONE', #11095, .T. ) ;
#23243=ORIENTED_EDGE ( 'NONE', *, *, #41061, .T. ) ;
#23246=CARTESIAN_POINT ( 'NONE',  ( -10.99975357571800849, -11.03678792477782622, 60.87159911480458874 ) ) ;
#23248=CARTESIAN_POINT ( 'NONE',  ( -15.66191361000415583, -7.982949215278682509, 70.90989811847559565 ) ) ;
#23251=CARTESIAN_POINT ( 'NONE',  ( -14.76542504939979139, -8.279692840553558142, 60.61996284471974406 ) ) ;
#23252=CARTESIAN_POINT ( 'NONE',  ( -16.94618458872839994, -7.374472604449730184, 74.00372349603880195 ) ) ;
#23254=CARTESIAN_POINT ( 'NONE',  ( -18.96774969734608618, -7.981470143064878897, 63.65762499020824805 ) ) ;
#23256=CARTESIAN_POINT ( 'NONE',  ( -17.15134141312287852, -7.364115244199362920, 70.67531166753866501 ) ) ;
#23257=EDGE_CURVE ( 'NONE', #46413, #44873, #32189, .T. ) ;
#23259=CARTESIAN_POINT ( 'NONE',  ( -10.41531639268335496, -14.04517892474411589, 60.93293405735092705 ) ) ;
#23260=( BOUNDED_SURFACE ( )  B_SPLINE_SURFACE ( 3, 1, ( 
 ( #26600, #37405 ),
 ( #22664, #269 ),
 ( #4200, #19205 ),
 ( #37915, #34211 ),
 ( #18706, #33972 ),
 ( #23157, #41128 ),
 ( #3702, #33714 ) ),
 .UNSPECIFIED., .T., .F., .F. ) 
 B_SPLINE_SURFACE_WITH_KNOTS ( ( 4, 3, 4 ),
 ( 2, 2 ),
 ( 0.000000000000000000, 0.5000000000000000000, 1.000000000000000000 ),
 ( 0.000000000000000000, 1.000000000000000000 ),
 .UNSPECIFIED. ) 
 GEOMETRIC_REPRESENTATION_ITEM ( )  RATIONAL_B_SPLINE_SURFACE ( (
 ( 1.000000000000000000, 1.000000000000000000),
 ( 0.3333333333333335369, 0.3333333333333330373),
 ( 0.3333333333333335369, 0.3333333333333330373),
 ( 1.000000000000000000, 1.000000000000000000),
 ( 0.3333333333333333703, 0.3333333333333333703),
 ( 0.3333333333333333703, 0.3333333333333333703),
 ( 1.000000000000000000, 1.000000000000000000) ) ) 
 REPRESENTATION_ITEM ( '' )  SURFACE ( )  );
#23262=CARTESIAN_POINT ( 'NONE',  ( -23.16981202414103080, -18.80754655606318693, 62.54509979339044179 ) ) ;
#23263=ORIENTED_EDGE ( 'NONE', *, *, #2601, .T. ) ;
#23265=AXIS2_PLACEMENT_3D ( 'NONE', #30841, #23699, #4244 ) ;
#23268=CARTESIAN_POINT ( 'NONE',  ( -20.25220558506708102, -7.916061535415647832, 70.36445088532752834 ) ) ;
#23270=EDGE_CURVE ( 'NONE', #1137, #35822, #8487, .T. ) ;
#23271=( BOUNDED_CURVE ( )  B_SPLINE_CURVE ( 3, ( #28925, #10229, #34554, #41223 ),
 .UNSPECIFIED., .F., .F. ) 
 B_SPLINE_CURVE_WITH_KNOTS ( ( 4, 4 ),
 ( 0.4074455897393626236, 0.5000000000000000000 ),
 .UNSPECIFIED. ) 
 CURVE ( )  GEOMETRIC_REPRESENTATION_ITEM ( )  RATIONAL_B_SPLINE_CURVE ( ( 0.6983129098260891787, 0.7760317562606902086, 0.8765941196519926315, 0.9999999999999927836 ) ) 
 REPRESENTATION_ITEM ( '' )  );
#23272=EDGE_CURVE ( 'NONE', #46893, #9283, #24368, .T. ) ;
#23273=B_SPLINE_CURVE_WITH_KNOTS ( 'NONE', 1,
 ( #2876, #47474 ),
 .UNSPECIFIED., .F., .F.,
 ( 2, 2 ),
 ( 0.000000000000000000, 1.000000000000000000 ),
 .UNSPECIFIED. ) ;
#23276=CARTESIAN_POINT ( 'NONE',  ( -20.88147674714181079, -8.209942860146695054, 60.02620543942160225 ) ) ;
#23277=DIRECTION ( 'NONE',  ( 0.000000000000000000, 0.000000000000000000, 1.000000000000000000 ) ) ;
#23278=EDGE_LOOP ( 'NONE', ( #36638, #4896 ) ) ;
#23279=CARTESIAN_POINT ( 'NONE',  ( -14.01118748589248320, -10.49619482288619920, 53.49999999999995026 ) ) ;
#23281=DIRECTION ( 'NONE',  ( -0.1675476790616363121, 0.9858639740050647582, -1.222863418168487711E-17 ) ) ;
#23282=CARTESIAN_POINT ( 'NONE',  ( -20.98899269145036328, -20.89566229441305723, 69.14630445674248449 ) ) ;
#23284=CARTESIAN_POINT ( 'NONE',  ( -11.69468685320639345, -19.67737422254949919, 54.02312124697527906 ) ) ;
#23286=CARTESIAN_POINT ( 'NONE',  ( -20.22231478687352890, -8.334269993598422133, 74.02096540213653952 ) ) ;
#23287=CARTESIAN_POINT ( 'NONE',  ( -10.35661267713556022, -12.45241038966069347, 60.91358145539074798 ) ) ;
#23288=CARTESIAN_POINT ( 'NONE',  ( -24.46690853180149361, -14.41907004423223171, 62.92116527710209084 ) ) ;
#23290=CARTESIAN_POINT ( 'NONE',  ( -18.17795515447646792, -21.82680332084924046, 72.42944048533317414 ) ) ;
#23291=CARTESIAN_POINT ( 'NONE',  ( -17.71538801587749035, -22.25356272040728101, 58.51279210549326848 ) ) ;
#23293=AXIS2_PLACEMENT_3D ( 'NONE', #24108, #19928, #9095 ) ;
#23294=CARTESIAN_POINT ( 'NONE',  ( -21.15981645306944259, -20.78812328065465920, 69.05450213015602401 ) ) ;
#23296=DIRECTION ( 'NONE',  ( -0.5420872618288283817, -0.8403222004463036798, 7.592316861452270591E-08 ) ) ;
#23298=CARTESIAN_POINT ( 'NONE',  ( -15.19549097431359463, -21.91815212410659086, 68.76088336006283441 ) ) ;
#23299=LINE ( 'NONE', #16617, #32183 ) ;
#23300=VERTEX_POINT ( 'NONE', #18163 ) ;
#23302=EDGE_LOOP ( 'NONE', ( #13648, #4372, #9058, #24389, #23956 ) ) ;
#23304=ORIENTED_EDGE ( 'NONE', *, *, #37976, .F. ) ;
#23305=FACE_BOUND ( 'NONE', #10925, .T. ) ;
#23306=EDGE_CURVE ( 'NONE', #21625, #44542, #7327, .T. ) ;
#23307=ORIENTED_EDGE ( 'NONE', *, *, #23060, .T. ) ;
#23308=ORIENTED_EDGE ( 'NONE', *, *, #31431, .T. ) ;
#23310=CARTESIAN_POINT ( 'NONE',  ( -17.58740562021222686, -21.86528886929834670, 62.01968736857112674 ) ) ;
#23314=CARTESIAN_POINT ( 'NONE',  ( -12.58533685989522333, -19.86927988795931554, 68.56487230657450027 ) ) ;
#23316=ORIENTED_EDGE ( 'NONE', *, *, #40247, .F. ) ;
#23317=VERTEX_POINT ( 'NONE', #3642 ) ;
#23319=FACE_OUTER_BOUND ( 'NONE', #36657, .T. ) ;
#23320=CARTESIAN_POINT ( 'NONE',  ( -11.35825037048775066, -11.21643016533576898, 60.67885780704619947 ) ) ;
#23321=CARTESIAN_POINT ( 'NONE',  ( -21.56183257638102901, -9.162504018457454436, 70.14749226153745099 ) ) ;
#23322=ORIENTED_EDGE ( 'NONE', *, *, #27212, .F. ) ;
#23327=ORIENTED_EDGE ( 'NONE', *, *, #12075, .T. ) ;
#23328=EDGE_CURVE ( 'NONE', #48564, #38209, #14683, .T. ) ;
#23329=EDGE_CURVE ( 'NONE', #1270, #8865, #6744, .T. ) ;
#23332=CARTESIAN_POINT ( 'NONE',  ( -12.23220189640646538, -19.57856266540686718, 58.07682373937821296 ) ) ;
#23333=VERTEX_POINT ( 'NONE', #18405 ) ;
#23335=CARTESIAN_POINT ( 'NONE',  ( -11.76008542200333018, -19.01204350050032232, 68.10200740694565980 ) ) ;
#23336=CARTESIAN_POINT ( 'NONE',  ( -24.18875248430348179, -11.68798133371211279, 59.58212113430876400 ) ) ;
#23337=VERTEX_POINT ( 'NONE', #33659 ) ;
#23339=DIRECTION ( 'NONE',  ( -0.1666496227699850730, 0.9805797387979519053, 0.1033986416233890343 ) ) ;
#23340=CARTESIAN_POINT ( 'NONE',  ( -20.49170831689750472, -8.461258797198503601, 63.59649424907593129 ) ) ;
#23341=ORIENTED_EDGE ( 'NONE', *, *, #23820, .T. ) ;
#23344=B_SPLINE_CURVE_WITH_KNOTS ( 'NONE', 1,
 ( #45258, #45019 ),
 .UNSPECIFIED., .F., .F.,
 ( 2, 2 ),
 ( 0.000000000000000000, 1.000000000000000000 ),
 .UNSPECIFIED. ) ;
#23345=CARTESIAN_POINT ( 'NONE',  ( -19.15853812393435618, -7.563744986369119516, 63.59122566566123425 ) ) ;
#23347=ORIENTED_EDGE ( 'NONE', *, *, #27337, .T. ) ;
#23349=CARTESIAN_POINT ( 'NONE',  ( -11.08976439687648075, -11.70580308251566315, 74.85839985167115174 ) ) ;
#23350=ADVANCED_FACE ( 'NONE', ( #14943 ), #17061, .T. ) ;
#23351=DIRECTION ( 'NONE',  ( -1.274157596560980788E-05, -2.329884826735012561E-06, 0.9999999999161118813 ) ) ;
#23352=EDGE_LOOP ( 'NONE', ( #24236, #10329, #23159, #3581, #8906 ) ) ;
#23353=CYLINDRICAL_SURFACE ( 'NONE', #27596, 0.1500000000000050182 ) ;
#23356=CARTESIAN_POINT ( 'NONE',  ( -11.95103603871087650, -9.754441519819101458, 60.71951479555669096 ) ) ;
#23357=ORIENTED_EDGE ( 'NONE', *, *, #45220, .T. ) ;
#23358=CARTESIAN_POINT ( 'NONE',  ( -12.45873566688478107, -9.804017486950373339, 57.10407583662104258 ) ) ;
#23359=VECTOR ( 'NONE', #47226, 1000.000000000000000 ) ;
#23360=AXIS2_PLACEMENT_3D ( 'NONE', #40458, #39739, #10670 ) ;
#23361=DIRECTION ( 'NONE',  ( 0.3126464228004117163, 0.3197690014840504635, 0.8944271909999156334 ) ) ;
#23362=VERTEX_POINT ( 'NONE', #12487 ) ;
#23364=CARTESIAN_POINT ( 'NONE',  ( -10.47787889545108087, -15.67627839034492787, 61.03789014633728272 ) ) ;
#23365=LINE ( 'NONE', #30281, #19493 ) ;
#23366=EDGE_CURVE ( 'NONE', #43494, #7495, #20264, .T. ) ;
#23367=CARTESIAN_POINT ( 'NONE',  ( -10.40277084706750621, -15.44444119821074679, 57.86792809062919218 ) ) ;
#23369=CARTESIAN_POINT ( 'NONE',  ( -12.50974054546264469, -19.79409688107175924, 61.58781908136975147 ) ) ;
#23370=CARTESIAN_POINT ( 'NONE',  ( -12.89671927708317689, -20.22380232670898081, 68.49224713894388117 ) ) ;
#23371=CARTESIAN_POINT ( 'NONE',  ( -23.23017095593700532, -18.72167141714702510, 69.52201958683488670 ) ) ;
#23372=LINE ( 'NONE', #8355, #4868 ) ;
#23376=CARTESIAN_POINT ( 'NONE',  ( -14.17292126938155761, -21.07377676424729884, 68.61192020317307083 ) ) ;
#23377=CARTESIAN_POINT ( 'NONE',  ( -17.23248763171904230, -7.758097994416163878, 74.26018367925263419 ) ) ;
#23378=CARTESIAN_POINT ( 'NONE',  ( -18.66311988809301425, -7.868636481342422329, 70.65595886192740238 ) ) ;
#23379=ORIENTED_EDGE ( 'NONE', *, *, #4783, .F. ) ;
#23380=ORIENTED_EDGE ( 'NONE', *, *, #27011, .F. ) ;
#23382=CARTESIAN_POINT ( 'NONE',  ( -19.85889901765038346, -21.37233916515964438, 69.21353063550283480 ) ) ;
#23384=CARTESIAN_POINT ( 'NONE',  ( -14.99706828511980916, -21.85287925006270626, 65.29092110561946072 ) ) ;
#23386=( BOUNDED_SURFACE ( )  B_SPLINE_SURFACE ( 3, 1, ( 
 ( #11543, #26569 ),
 ( #41588, #19175 ),
 ( #473, #15455 ),
 ( #30523, #35400 ),
 ( #34916, #15952 ),
 ( #24090, #35154 ),
 ( #19911, #4643 ) ),
 .UNSPECIFIED., .T., .F., .F. ) 
 B_SPLINE_SURFACE_WITH_KNOTS ( ( 4, 3, 4 ),
 ( 2, 2 ),
 ( 0.000000000000000000, 0.5000000000000000000, 1.000000000000000000 ),
 ( 0.000000000000000000, 1.000000000000000000 ),
 .UNSPECIFIED. ) 
 GEOMETRIC_REPRESENTATION_ITEM ( )  RATIONAL_B_SPLINE_SURFACE ( (
 ( 1.000000000000000000, 1.000000000000000000),
 ( 0.3333333333333335369, 0.3333333333333330373),
 ( 0.3333333333333335369, 0.3333333333333330373),
 ( 1.000000000000000000, 1.000000000000000000),
 ( 0.3333333333333333703, 0.3333333333333333703),
 ( 0.3333333333333333703, 0.3333333333333333703),
 ( 1.000000000000000000, 1.000000000000000000) ) ) 
 REPRESENTATION_ITEM ( '' )  SURFACE ( )  );
#23387=ORIENTED_EDGE ( 'NONE', *, *, #41868, .T. ) ;
#23388=CARTESIAN_POINT ( 'NONE',  ( -24.84793648988037518, -14.18443574041886457, 69.83770584630335065 ) ) ;
#23389=AXIS2_PLACEMENT_3D ( 'NONE', #15167, #14415, #48425 ) ;
#23391=EDGE_CURVE ( 'NONE', #38482, #26173, #14374, .T. ) ;
#23392=ADVANCED_FACE ( 'NONE', ( #12245 ), #34393, .T. ) ;
#23393=CARTESIAN_POINT ( 'NONE',  ( -19.55442184481404766, -21.52995072282663358, 65.47958309245051112 ) ) ;
#23396=VECTOR ( 'NONE', #29279, 1000.000000000000000 ) ;
#23397=CARTESIAN_POINT ( 'NONE',  ( -12.86134249074305913, -20.11797452945269882, 72.10653668688858886 ) ) ;
#23398=EDGE_CURVE ( 'NONE', #5898, #10296, #9050, .T. ) ;
#23399=CARTESIAN_POINT ( 'NONE',  ( -13.97837889017616320, -8.203094814523453238, 74.38609903144701718 ) ) ;
#23400=( BOUNDED_CURVE ( )  B_SPLINE_CURVE ( 3, ( #31287, #15771, #31054, #46071 ),
 .UNSPECIFIED., .F., .F. ) 
 B_SPLINE_CURVE_WITH_KNOTS ( ( 4, 4 ),
 ( 0.5000000000000000000, 0.9074455897393672865 ),
 .UNSPECIFIED. ) 
 CURVE ( )  GEOMETRIC_REPRESENTATION_ITEM ( )  RATIONAL_B_SPLINE_CURVE ( ( 0.9999999999999759082, 0.4567392136813248626, 0.3561768502900444222, 0.6983129098261084966 ) ) 
 REPRESENTATION_ITEM ( '' )  );
#23401=ORIENTED_EDGE ( 'NONE', *, *, #8722, .T. ) ;
#23402=( BOUNDED_CURVE ( )  B_SPLINE_CURVE ( 3, ( #4431, #37918, #23160, #33225 ),
 .UNSPECIFIED., .F., .F. ) 
 B_SPLINE_CURVE_WITH_KNOTS ( ( 4, 4 ),
 ( 0.000000000000000000, 0.4074455897393657322 ),
 .UNSPECIFIED. ) 
 CURVE ( )  GEOMETRIC_REPRESENTATION_ITEM ( )  RATIONAL_B_SPLINE_CURVE ( ( 1.000000000000000000, 0.4567392136813294146, 0.3561768502900293787, 0.6983129098260999479 ) ) 
 REPRESENTATION_ITEM ( '' )  );
#23408=CARTESIAN_POINT ( 'NONE',  ( -13.88419686192642111, -8.703135698866935499, 57.11400917758039952 ) ) ;
#23409=CARTESIAN_POINT ( 'NONE',  ( -10.29140437080923220, -12.65793278909525377, 64.46174418839692066 ) ) ;
#23410=EDGE_CURVE ( 'NONE', #26632, #28414, #29062, .T. ) ;
#23412=CARTESIAN_POINT ( 'NONE',  ( -21.37011387998928669, -21.12839667555923029, 69.24788507571554419 ) ) ;
#23416=CARTESIAN_POINT ( 'NONE',  ( -15.28291064399146215, -21.52618758091310980, 68.57592918174772478 ) ) ;
#23417=( BOUNDED_SURFACE ( )  B_SPLINE_SURFACE ( 3, 1, ( 
 ( #5753, #17034 ),
 ( #47103, #43906 ),
 ( #43663, #13343 ),
 ( #42925, #25180 ),
 ( #39951, #9918 ),
 ( #36244, #2526 ),
 ( #27900, #21489 ) ),
 .UNSPECIFIED., .T., .F., .F. ) 
 B_SPLINE_SURFACE_WITH_KNOTS ( ( 4, 3, 4 ),
 ( 2, 2 ),
 ( 0.000000000000000000, 0.5000000000000000000, 1.000000000000000000 ),
 ( 0.000000000000000000, 1.000000000000000000 ),
 .UNSPECIFIED. ) 
 GEOMETRIC_REPRESENTATION_ITEM ( )  RATIONAL_B_SPLINE_SURFACE ( (
 ( 1.000000000000000000, 1.000000000000000000),
 ( 0.3333333333333335369, 0.3333333333333330373),
 ( 0.3333333333333335369, 0.3333333333333330373),
 ( 1.000000000000000000, 1.000000000000000000),
 ( 0.3333333333333333703, 0.3333333333333333703),
 ( 0.3333333333333333703, 0.3333333333333333703),
 ( 1.000000000000000000, 1.000000000000000000) ) ) 
 REPRESENTATION_ITEM ( '' )  SURFACE ( )  );
#23418=CARTESIAN_POINT ( 'NONE',  ( -13.65948078749761585, -20.77935321253323053, 58.20216925893738846 ) ) ;
#23421=CARTESIAN_POINT ( 'NONE',  ( -20.74847686076342157, -20.96993771475205293, 62.13088051185322769 ) ) ;
#23422=ORIENTED_EDGE ( 'NONE', *, *, #40052, .F. ) ;
#23424=CARTESIAN_POINT ( 'NONE',  ( -18.59601872632196873, -7.856991649524070809, 73.85536540707786912 ) ) ;
#23425=CARTESIAN_POINT ( 'NONE',  ( -14.72744631621160494, -8.295007313424175521, 60.60524229057013201 ) ) ;
#23428=FACE_OUTER_BOUND ( 'NONE', #42751, .T. ) ;
#23429=CARTESIAN_POINT ( 'NONE',  ( -15.06075745000970834, -21.87520294740874149, 68.76248218113177302 ) ) ;
#23430=CARTESIAN_POINT ( 'NONE',  ( -10.45630165105249532, -15.48121050910559937, 57.86792791455135188 ) ) ;
#23431=LINE ( 'NONE', #4717, #26699 ) ;
#23432=CARTESIAN_POINT ( 'NONE',  ( -11.30174378650323064, -18.30512181131203064, 57.81274399976084766 ) ) ;
#23433=VECTOR ( 'NONE', #6703, 1000.000000000000114 ) ;
#23438=CARTESIAN_POINT ( 'NONE',  ( -11.06712629860931152, -18.69414434431124761, 61.39215439313597500 ) ) ;
#23440=CARTESIAN_POINT ( 'NONE',  ( -11.67943375510494874, -18.89645239624664796, 68.50217487844219022 ) ) ;
#23441=CARTESIAN_POINT ( 'NONE',  ( -21.43520510711937277, -9.072323815021505311, 70.14634923480093676 ) ) ;
#23442=EDGE_CURVE ( 'NONE', #20668, #25586, #45734, .T. ) ;
#23443=CARTESIAN_POINT ( 'NONE',  ( -14.78750802578769452, -21.29541614796527682, 61.82527411501091308 ) ) ;
#23444=VECTOR ( 'NONE', #45544, 1000.000000000000000 ) ;
#23446=ORIENTED_EDGE ( 'NONE', *, *, #31060, .T. ) ;
#23447=B_SPLINE_CURVE_WITH_KNOTS ( 'NONE', 3,
 ( #41548, #915, #440, #23089, #18628, #30958, #34143, #27012, #45973, #22589 ),
 .UNSPECIFIED., .F., .F.,
 ( 4, 2, 2, 2, 4 ),
 ( 0.1272669073658179995, 0.2522669073439466336, 0.3772669073220752400, 0.5022669073002039575, 0.6272669072783325639 ),
 .UNSPECIFIED. ) ;
#23451=CARTESIAN_POINT ( 'NONE',  ( -17.52853272358826686, -7.759682304905023642, 63.83584969886392457 ) ) ;
#23453=ORIENTED_EDGE ( 'NONE', *, *, #23306, .T. ) ;
#23455=CARTESIAN_POINT ( 'NONE',  ( -17.85555652284939043, -7.772123375420258107, 60.09532845646905486 ) ) ;
#23456=DIRECTION ( 'NONE',  ( -0.9950649908465211135, -0.09922531930717196080, 4.894557008102618136E-08 ) ) ;
#23457=ORIENTED_EDGE ( 'NONE', *, *, #25091, .F. ) ;
#23458=ADVANCED_FACE ( 'NONE', ( #688 ), #13892, .T. ) ;
#23459=CARTESIAN_POINT ( 'NONE',  ( -15.98001679475065373, -7.500493000024420098, 63.76987390602237582 ) ) ;
#23461=CARTESIAN_POINT ( 'NONE',  ( -10.47558912380517882, -13.96067967406488464, 57.44824990916067975 ) ) ;
#23462=EDGE_CURVE ( 'NONE', #34358, #35817, #12056, .T. ) ;
#23464=EDGE_LOOP ( 'NONE', ( #34165, #47784, #30224, #36306, #30220 ) ) ;
#23466=CARTESIAN_POINT ( 'NONE',  ( -10.37136279787074500, -14.92680326906059740, 71.32782707526337163 ) ) ;
#23469=ORIENTED_EDGE ( 'NONE', *, *, #34052, .F. ) ;
#23470=CARTESIAN_POINT ( 'NONE',  ( -23.42532394183187705, -19.22384306421519184, 62.46911594462533657 ) ) ;
#23471=CARTESIAN_POINT ( 'NONE',  ( -22.51880736180295983, -20.24487813920610790, 65.90410515226939481 ) ) ;
#23472=CARTESIAN_POINT ( 'NONE',  ( -22.27608729174900049, -12.19078426442220930, 53.88362224778187226 ) ) ;
#23473=ORIENTED_EDGE ( 'NONE', *, *, #13422, .T. ) ;
#23475=CARTESIAN_POINT ( 'NONE',  ( -24.08569470166255400, -11.47342236436628404, 63.12935185382383452 ) ) ;
#23478=CARTESIAN_POINT ( 'NONE',  ( -15.47038646904106507, -21.58309222549749506, 72.34575460768671462 ) ) ;
#23479=CARTESIAN_POINT ( 'NONE',  ( -21.18836735823073525, -20.77369112572868914, 65.46965119999302374 ) ) ;
#23482=LINE ( 'NONE', #16060, #29751 ) ;
#23483=CARTESIAN_POINT ( 'NONE',  ( -17.42409385541300892, -14.80920654474439502, 75.49999999999994316 ) ) ;
#23486=ORIENTED_EDGE ( 'NONE', *, *, #39300, .F. ) ;
#23488=CARTESIAN_POINT ( 'NONE',  ( -24.25171713147202368, -16.35308467727669068, 59.12332432120680181 ) ) ;
#23490=CYLINDRICAL_SURFACE ( 'NONE', #24525, 0.1499999999999993838 ) ;
#23491=CARTESIAN_POINT ( 'NONE',  ( -16.17067486245293040, -22.15313371995832625, 58.40772777080032796 ) ) ;
#23493=CARTESIAN_POINT ( 'NONE',  ( -14.74690617566109019, -21.27702427001963414, 58.46617884968173229 ) ) ;
#23494=ORIENTED_EDGE ( 'NONE', *, *, #9945, .F. ) ;
#23495=CARTESIAN_POINT ( 'NONE',  ( -10.37497031247464463, -14.69804315800203121, 71.62782692816419683 ) ) ;
#23496=CARTESIAN_POINT ( 'NONE',  ( -20.72573862760241070, -8.580110178657996300, 60.14125250079693785 ) ) ;
#23497=CARTESIAN_POINT ( 'NONE',  ( -10.09412421677371796, -16.14182453506428061, 68.09955039505892671 ) ) ;
#23498=VERTEX_POINT ( 'NONE', #39798 ) ;
#23499=CARTESIAN_POINT ( 'NONE',  ( -23.87505191747562705, -17.66227225522637667, 66.24357201825841912 ) ) ;
#23500=AXIS2_PLACEMENT_3D ( 'NONE', #20018, #30388, #26929 ) ;
#23501=( BOUNDED_CURVE ( )  B_SPLINE_CURVE ( 3, ( #25760, #29701, #33612, #41770 ),
 .UNSPECIFIED., .F., .F. ) 
 B_SPLINE_CURVE_WITH_KNOTS ( ( 4, 4 ),
 ( 0.000000000000000000, 0.4074455897393618464 ),
 .UNSPECIFIED. ) 
 CURVE ( )  GEOMETRIC_REPRESENTATION_ITEM ( )  RATIONAL_B_SPLINE_CURVE ( ( 1.000000000000000000, 0.4567392136813374082, 0.3561768502900323208, 0.6983129098260847378 ) ) 
 REPRESENTATION_ITEM ( '' )  );
#23503=CARTESIAN_POINT ( 'NONE',  ( -10.00747133761319141, -14.10395761772617362, 60.96175355949325336 ) ) ;
#23505=CARTESIAN_POINT ( 'NONE',  ( -10.21764033814386963, -12.91954908504599331, 67.92327745040803677 ) ) ;
#23506=CARTESIAN_POINT ( 'NONE',  ( -17.59331746331979929, -7.761237803891376075, 63.55057029381062961 ) ) ;
#23508=ORIENTED_EDGE ( 'NONE', *, *, #11329, .T. ) ;
#23511=LINE ( 'NONE', #4793, #27983 ) ;
#23513=AXIS2_PLACEMENT_3D ( 'NONE', #48645, #29948, #11231 ) ;
#23515=B_SPLINE_CURVE_WITH_KNOTS ( 'NONE', 3,
 ( #40582, #17458, #21166, #39869, #29278, #5902, #17689, #32714, #39630, #20920 ),
 .UNSPECIFIED., .F., .F.,
 ( 4, 2, 2, 2, 4 ),
 ( 0.6272669072782607325, 0.7522669073001474471, 0.8772669073220342728, 1.002266907343920987, 1.127266907365807702 ),
 .UNSPECIFIED. ) ;
#23516=CARTESIAN_POINT ( 'NONE',  ( -17.63792724537347212, -22.25688666393347859, 58.59208636575791473 ) ) ;
#23517=CARTESIAN_POINT ( 'NONE',  ( -20.42320262601612413, -8.483743935243163392, 66.79720689127475453 ) ) ;
#23518=EDGE_CURVE ( 'NONE', #41967, #7285, #33143, .T. ) ;
#23519=CARTESIAN_POINT ( 'NONE',  ( -10.41586258189964376, -15.60891902706924306, 64.80771822714827124 ) ) ;
#23521=EDGE_CURVE ( 'NONE', #5461, #1862, #35372, .T. ) ;
#23522=VERTEX_POINT ( 'NONE', #5602 ) ;
#23523=CARTESIAN_POINT ( 'NONE',  ( -21.68499379980493558, -9.192514338196573931, 66.96149992326067490 ) ) ;
#23525=EDGE_LOOP ( 'NONE', ( #36214, #5376, #42618, #13681, #26483 ) ) ;
#23527=FACE_OUTER_BOUND ( 'NONE', #25457, .T. ) ;
#23529=ORIENTED_EDGE ( 'NONE', *, *, #48001, .F. ) ;
#23530=CARTESIAN_POINT ( 'NONE',  ( -18.18630483459547165, -22.22016634624343467, 65.53806309781653283 ) ) ;
#23533=EDGE_CURVE ( 'NONE', #46821, #2243, #43851, .T. ) ;
#23535=CARTESIAN_POINT ( 'NONE',  ( -10.32991051753928780, -12.53378322482101126, 60.93707066162556885 ) ) ;
#23536=CARTESIAN_POINT ( 'NONE',  ( -24.32102835452959866, -16.00663571048927381, 66.36324977196242969 ) ) ;
#23537=ORIENTED_EDGE ( 'NONE', *, *, #33662, .T. ) ;
#23538=CARTESIAN_POINT ( 'NONE',  ( -22.06477193427564387, -8.981018767459000074, 63.23507824025425350 ) ) ;
#23539=CARTESIAN_POINT ( 'NONE',  ( -20.89525781030762630, -21.40132374626120182, 58.78328657048043482 ) ) ;
#23543=FACE_BOUND ( 'NONE', #34200, .T. ) ;
#23544=CARTESIAN_POINT ( 'NONE',  ( -11.36795091080559850, -18.31963851737709348, 58.10714594516144871 ) ) ;
#23548=CYLINDRICAL_SURFACE ( 'NONE', #42547, 0.1499999999999973577 ) ;
#23550=CARTESIAN_POINT ( 'NONE',  ( -11.17634552511236734, -11.65223367170475655, 67.63367030445587602 ) ) ;
#23551=CARTESIAN_POINT ( 'NONE',  ( -24.29232374648589854, -16.16102685949518403, 62.89328677060923667 ) ) ;
#23552=( BOUNDED_CURVE ( )  B_SPLINE_CURVE ( 3, ( #46693, #2824, #44453, #25006 ),
 .UNSPECIFIED., .F., .F. ) 
 B_SPLINE_CURVE_WITH_KNOTS ( ( 4, 4 ),
 ( 0.9074455897393639559, 1.000000000000000000 ),
 .UNSPECIFIED. ) 
 CURVE ( )  GEOMETRIC_REPRESENTATION_ITEM ( )  RATIONAL_B_SPLINE_CURVE ( ( 0.6983129098260923984, 0.7760317562606976471, 0.8765941196520001810, 1.000000000000000000 ) ) 
 REPRESENTATION_ITEM ( '' )  );
#23553=EDGE_CURVE ( 'NONE', #31463, #18208, #2029, .T. ) ;
#23554=VERTEX_POINT ( 'NONE', #43010 ) ;
#23557=FACE_BOUND ( 'NONE', #30889, .T. ) ;
#23558=VERTEX_POINT ( 'NONE', #17618 ) ;
#23560=ORIENTED_EDGE ( 'NONE', *, *, #12476, .F. ) ;
#23561=CARTESIAN_POINT ( 'NONE',  ( -10.44761804341386124, -15.84536169652562343, 60.92300268024614240 ) ) ;
#23562=CARTESIAN_POINT ( 'NONE',  ( -16.25451963475149952, -21.76959929332391397, 65.36997467570328979 ) ) ;
#23563=EDGE_CURVE ( 'NONE', #33660, #44249, #28473, .T. ) ;
#23564=CARTESIAN_POINT ( 'NONE',  ( -17.40624601077856681, -7.359220752920395903, 67.22050788099178931 ) ) ;
#23565=CARTESIAN_POINT ( 'NONE',  ( -13.79463883769849097, -8.760909077082668972, 57.26968041321134706 ) ) ;
#23566=CARTESIAN_POINT ( 'NONE',  ( -12.54339362283315396, -20.43782951766612044, 72.00642459070172663 ) ) ;
#23567=( BOUNDED_CURVE ( )  B_SPLINE_CURVE ( 3, ( #19529, #7991, #1288, #11411 ),
 .UNSPECIFIED., .F., .F. ) 
 B_SPLINE_CURVE_WITH_KNOTS ( ( 4, 4 ),
 ( 0.9074455897393722825, 1.000000000000000000 ),
 .UNSPECIFIED. ) 
 CURVE ( )  GEOMETRIC_REPRESENTATION_ITEM ( )  RATIONAL_B_SPLINE_CURVE ( ( 0.6983129098261009471, 0.7760317562607050856, 0.8765941196520047329, 1.000000000000000000 ) ) 
 REPRESENTATION_ITEM ( '' )  );
#23569=ORIENTED_EDGE ( 'NONE', *, *, #2101, .F. ) ;
#23571=AXIS2_PLACEMENT_3D ( 'NONE', #32763, #13791, #3216 ) ;
#23572=DIRECTION ( 'NONE',  ( 1.070267892916910012E-05, 6.715522048394477486E-06, -0.9999999999201771850 ) ) ;
#23573=CARTESIAN_POINT ( 'NONE',  ( -19.74286224202880291, -21.41400126446427166, 65.65589394489410324 ) ) ;
#23574=ORIENTED_EDGE ( 'NONE', *, *, #32860, .F. ) ;
#23577=ORIENTED_EDGE ( 'NONE', *, *, #8305, .F. ) ;
#23578=CARTESIAN_POINT ( 'NONE',  ( -14.97035482569482312, -21.41873484682592377, 61.92128389535452015 ) ) ;
#23580=CARTESIAN_POINT ( 'NONE',  ( -17.39761409878557785, -7.809256622337199971, 67.02039592144427615 ) ) ;
#23581=VECTOR ( 'NONE', #27350, 1000.000000000000114 ) ;
#23583=CARTESIAN_POINT ( 'NONE',  ( -17.79084007069931417, -7.768752218527305686, 60.38060768310334225 ) ) ;
#23585=CARTESIAN_POINT ( 'NONE',  ( -22.05807764791711278, -8.975638133202819446, 63.31340990608051555 ) ) ;
#23587=EDGE_CURVE ( 'NONE', #23075, #5574, #36117, .T. ) ;
#23588=ORIENTED_EDGE ( 'NONE', *, *, #5232, .T. ) ;
#23589=B_SPLINE_CURVE_WITH_KNOTS ( 'NONE', 1,
 ( #19076, #11440 ),
 .UNSPECIFIED., .F., .F.,
 ( 2, 2 ),
 ( 0.000000000000000000, 1.000000000000000000 ),
 .UNSPECIFIED. ) ;
#23590=LINE ( 'NONE', #12017, #19446 ) ;
#23591=CARTESIAN_POINT ( 'NONE',  ( -24.82475127085388422, -15.66597259679895693, 73.11808347143848152 ) ) ;
#23594=CARTESIAN_POINT ( 'NONE',  ( -15.98090817348981751, -7.500318407754576810, 63.86999797141741908 ) ) ;
#23595=EDGE_LOOP ( 'NONE', ( #26478, #41858, #6077, #23825, #19141 ) ) ;
#23599=CARTESIAN_POINT ( 'NONE',  ( -16.45566506110110083, -21.79267588865899086, 62.04095995016087528 ) ) ;
#23600=CARTESIAN_POINT ( 'NONE',  ( -24.14679772577363437, -12.68507108172156883, 70.05770892828130059 ) ) ;
#23601=CARTESIAN_POINT ( 'NONE',  ( -15.39536932222403287, -19.92137602241599836, 53.49999999999995026 ) ) ;
#23604=CARTESIAN_POINT ( 'NONE',  ( -10.57723003925373106, -17.74759380694297306, 71.75373442408677249 ) ) ;
#23606=CARTESIAN_POINT ( 'NONE',  ( -15.15158015243114953, -21.90415461596747448, 68.77604118143560186 ) ) ;
#23611=B_SPLINE_CURVE_WITH_KNOTS ( 'NONE', 1,
 ( #44302, #6129 ),
 .UNSPECIFIED., .F., .F.,
 ( 2, 2 ),
 ( 0.000000000000000000, 1.000000000000000000 ),
 .UNSPECIFIED. ) ;
#23612=CARTESIAN_POINT ( 'NONE',  ( -10.64577744754535082, -11.71757184301072563, 74.67344733366148546 ) ) ;
#23614=EDGE_CURVE ( 'NONE', #596, #19379, #45575, .T. ) ;
#23615=LINE ( 'NONE', #16437, #19628 ) ;
#23616=ADVANCED_FACE ( 'NONE', ( #48637 ), #14877, .T. ) ;
#23618=EDGE_CURVE ( 'NONE', #31116, #8437, #5631, .T. ) ;
#23621=CARTESIAN_POINT ( 'NONE',  ( -22.85634303820408064, -10.39183521286026490, 66.73109339323789868 ) ) ;
#23622=CARTESIAN_POINT ( 'NONE',  ( -11.16720021946830421, -11.56054808309503379, 67.91864607954204303 ) ) ;
#23623=CARTESIAN_POINT ( 'NONE',  ( -10.42732927881409388, -14.54885027197008185, 71.51709673969678249 ) ) ;
#23626=DIRECTION ( 'NONE',  ( -0.9729319276368275649, -0.2310918955413239495, 6.827553174175006206E-08 ) ) ;
#23628=CARTESIAN_POINT ( 'NONE',  ( -23.22139472215082279, -18.73524832941601304, 69.48299170654385648 ) ) ;
#23629=CARTESIAN_POINT ( 'NONE',  ( -11.03230881600246427, -10.98182333549695322, 60.79390388117851529 ) ) ;
#23630=EDGE_LOOP ( 'NONE', ( #7077, #36264, #6801, #13498, #4429 ) ) ;
#23631=ORIENTED_EDGE ( 'NONE', *, *, #19563, .F. ) ;
#23632=CARTESIAN_POINT ( 'NONE',  ( -12.37147782024668707, -20.28402873453449828, 68.53668635025047706 ) ) ;
#23634=B_SPLINE_CURVE_WITH_KNOTS ( 'NONE', 3,
 ( #26376, #44866, #3982, #18994, #15273, #33997, #26882, #37940, #29839, #7196 ),
 .UNSPECIFIED., .F., .F.,
 ( 4, 2, 2, 2, 4 ),
 ( 0.1272669073658881933, 0.2522669073463699174, 0.3772669073268516970, 0.5022669073073334767, 0.6272669072878152008 ),
 .UNSPECIFIED. ) ;
#23635=FACE_OUTER_BOUND ( 'NONE', #42358, .T. ) ;
#23639=EDGE_CURVE ( 'NONE', #7665, #39283, #47810, .T. ) ;
#23640=FACE_OUTER_BOUND ( 'NONE', #19626, .T. ) ;
#23641=CARTESIAN_POINT ( 'NONE',  ( -10.34343347544818847, -12.28147837111555774, 54.02312124697528617 ) ) ;
#23643=CARTESIAN_POINT ( 'NONE',  ( -18.68070144837527735, -7.415226739706411330, 54.27966884056654351 ) ) ;
#23644=CARTESIAN_POINT ( 'NONE',  ( -11.06345430940418417, -18.68820014949154640, 61.45523615231426362 ) ) ;
#23647=CARTESIAN_POINT ( 'NONE',  ( -24.85359104829803911, -14.25571788259268402, 69.76779960783916579 ) ) ;
#23648=CARTESIAN_POINT ( 'NONE',  ( -17.42409385541300892, -14.80920654474439502, 77.49999999999994316 ) ) ;
#23650=EDGE_CURVE ( 'NONE', #47561, #32087, #4924, .T. ) ;
#23651=CARTESIAN_POINT ( 'NONE',  ( -14.98249323814573941, -9.880861343182303358, 53.49999999999995026 ) ) ;
#23652=B_SPLINE_CURVE_WITH_KNOTS ( 'NONE', 3,
 ( #28746, #43776, #10034, #40073, #21605, #25057, #6340, #17878, #32902, #14177 ),
 .UNSPECIFIED., .F., .F.,
 ( 4, 2, 2, 2, 4 ),
 ( 0.6272669072877726792, 0.7522669073072767443, 0.8772669073267809203, 1.002266907346284874, 1.127266907365789050 ),
 .UNSPECIFIED. ) ;
#23653=CARTESIAN_POINT ( 'NONE',  ( -23.65624057141237202, -11.51332318074561911, 66.72214514605295221 ) ) ;
#23654=ORIENTED_EDGE ( 'NONE', *, *, #31718, .T. ) ;
#23655=DIRECTION ( 'NONE',  ( 0.9375570856950864451, -0.3478314405900309603, 3.549360974553817487E-17 ) ) ;
#23658=CYLINDRICAL_SURFACE ( 'NONE', #25801, 0.1499999999999949984 ) ;
#23659=EDGE_LOOP ( 'NONE', ( #4851, #33493, #47415, #21000, #28366 ) ) ;
#23660=CARTESIAN_POINT ( 'NONE',  ( -24.20836943865575464, -17.88934756284849215, 62.66016244028183024 ) ) ;
#23661=CARTESIAN_POINT ( 'NONE',  ( -18.39792479006713677, -22.19536379348757293, 68.85868763382491409 ) ) ;
#23663=CARTESIAN_POINT ( 'NONE',  ( -15.12736151640637416, -21.89643440865206614, 68.69097607374993686 ) ) ;
#23665=B_SPLINE_CURVE_WITH_KNOTS ( 'NONE', 3,
 ( #29834, #11117, #17991, #17747, #37183, #32546, #14515, #10146, #26138, #3469 ),
 .UNSPECIFIED., .F., .F.,
 ( 4, 2, 2, 2, 4 ),
 ( 0.1272669073658366790, 0.2522669073463276179, 0.3772669073268185014, 0.5022669073073093848, 0.6272669072878003238 ),
 .UNSPECIFIED. ) ;
#23666=CARTESIAN_POINT ( 'NONE',  ( -14.79906637807316550, -21.78150152883456059, 61.67954536979805624 ) ) ;
#23671=CARTESIAN_POINT ( 'NONE',  ( -20.55284450191522083, -8.048022495885772898, 66.88129830338009185 ) ) ;
#23673=CARTESIAN_POINT ( 'NONE',  ( -13.17078218117215549, -9.186392337449538203, 67.39414915108072535 ) ) ;
#23674=ADVANCED_FACE ( 'NONE', ( #47918 ), #48153, .F. ) ;
#23675=EDGE_CURVE ( 'NONE', #5852, #486, #39004, .T. ) ;
#23676=ORIENTED_EDGE ( 'NONE', *, *, #31436, .F. ) ;
#23677=ORIENTED_EDGE ( 'NONE', *, *, #35548, .F. ) ;
#23679=CARTESIAN_POINT ( 'NONE',  ( -18.55957040452605611, -7.446158924837727788, 74.02559677774105751 ) ) ;
#23680=CARTESIAN_POINT ( 'NONE',  ( -10.33431723597471930, -12.52035407725662886, 60.98348989824278732 ) ) ;
#23681=ORIENTED_EDGE ( 'NONE', *, *, #5733, .F. ) ;
#23682=CARTESIAN_POINT ( 'NONE',  ( -22.48430662296557614, -20.27711519517875516, 65.81926411519917508 ) ) ;
#23683=CARTESIAN_POINT ( 'NONE',  ( -16.30515107485298998, -22.17475187132452064, 61.86293996623023617 ) ) ;
#23685=LINE ( 'NONE', #22961, #19512 ) ;
#23686=CARTESIAN_POINT ( 'NONE',  ( -21.60978650687268754, -20.97240088203421493, 72.66299873415312049 ) ) ;
#23687=CARTESIAN_POINT ( 'NONE',  ( -11.32469144785209103, -18.34471071427194389, 57.80714594245691273 ) ) ;
#23689=CARTESIAN_POINT ( 'NONE',  ( -23.59327504554355315, -11.39630409041826198, 69.90682860766239060 ) ) ;
#23691=EDGE_CURVE ( 'NONE', #12198, #26955, #12342, .T. ) ;
#23693=EDGE_CURVE ( 'NONE', #42299, #42753, #11772, .T. ) ;
#23694=B_SPLINE_CURVE_WITH_KNOTS ( 'NONE', 3,
 ( #34288, #38964, #41941, #818, #12622, #15568, #573, #42677, #37988, #8942 ),
 .UNSPECIFIED., .F., .F.,
 ( 4, 2, 2, 2, 4 ),
 ( 0.1272669073658150296, 0.2522669073463081890, 0.3772669073268013484, 0.5022669073072945078, 0.6272669072877876673 ),
 .UNSPECIFIED. ) ;
#23695=CARTESIAN_POINT ( 'NONE',  ( -20.42942694929465119, -8.423054519096806914, 59.99692253513481432 ) ) ;
#23698=CARTESIAN_POINT ( 'NONE',  ( -22.88264614489240856, -10.34704276773305764, 63.35713876973677827 ) ) ;
#23699=DIRECTION ( 'NONE',  ( -0.4846961512978548714, -0.8746825943832684525, -4.196010045124609427E-08 ) ) ;
#23701=( BOUNDED_SURFACE ( )  B_SPLINE_SURFACE ( 3, 1, ( 
 ( #40201, #5755 ),
 ( #47360, #43909 ),
 ( #24469, #47105 ),
 ( #1803, #39473 ),
 ( #13824, #16802 ),
 ( #29108, #10162 ),
 ( #24936, #21492 ) ),
 .UNSPECIFIED., .T., .F., .F. ) 
 B_SPLINE_SURFACE_WITH_KNOTS ( ( 4, 3, 4 ),
 ( 2, 2 ),
 ( 0.000000000000000000, 0.5000000000000000000, 1.000000000000000000 ),
 ( 0.000000000000000000, 1.000000000000000000 ),
 .UNSPECIFIED. ) 
 GEOMETRIC_REPRESENTATION_ITEM ( )  RATIONAL_B_SPLINE_SURFACE ( (
 ( 1.000000000000000000, 1.000000000000000000),
 ( 0.3333333333333335369, 0.3333333333333330373),
 ( 0.3333333333333335369, 0.3333333333333330373),
 ( 1.000000000000000000, 1.000000000000000000),
 ( 0.3333333333333333703, 0.3333333333333333703),
 ( 0.3333333333333333703, 0.3333333333333333703),
 ( 1.000000000000000000, 1.000000000000000000) ) ) 
 REPRESENTATION_ITEM ( '' )  SURFACE ( )  );
#23702=ORIENTED_EDGE ( 'NONE', *, *, #17958, .F. ) ;
#23703=ORIENTED_EDGE ( 'NONE', *, *, #43918, .T. ) ;
#23705=ORIENTED_EDGE ( 'NONE', *, *, #12278, .F. ) ;
#23706=EDGE_CURVE ( 'NONE', #575, #34661, #1409, .T. ) ;
#23708=VECTOR ( 'NONE', #36811, 1000.000000000000000 ) ;
#23709=CYLINDRICAL_SURFACE ( 'NONE', #35470, 0.1500000000000015488 ) ;
#23710=ORIENTED_EDGE ( 'NONE', *, *, #2653, .T. ) ;
#23711=( BOUNDED_CURVE ( )  B_SPLINE_CURVE ( 3, ( #34093, #4086, #45694, #15614 ),
 .UNSPECIFIED., .F., .F. ) 
 B_SPLINE_CURVE_WITH_KNOTS ( ( 4, 4 ),
 ( 0.000000000000000000, 0.4074455897393659543 ),
 .UNSPECIFIED. ) 
 CURVE ( )  GEOMETRIC_REPRESENTATION_ITEM ( )  RATIONAL_B_SPLINE_CURVE ( ( 1.000000000000000000, 0.4567392136813356873, 0.3561768502900316546, 0.6983129098260879575 ) ) 
 REPRESENTATION_ITEM ( '' )  );
#23712=CARTESIAN_POINT ( 'NONE',  ( -10.83529129721023487, -11.33175171474136533, 67.75831252372202584 ) ) ;
#23714=ORIENTED_EDGE ( 'NONE', *, *, #20670, .T. ) ;
#23716=CARTESIAN_POINT ( 'NONE',  ( -20.92219709818629170, -8.231526085280929550, 60.04136453195106782 ) ) ;
#23717=FACE_OUTER_BOUND ( 'NONE', #45606, .T. ) ;
#23718=ORIENTED_EDGE ( 'NONE', *, *, #33650, .F. ) ;
#23720=AXIS2_PLACEMENT_3D ( 'NONE', #8263, #1591, #23281 ) ;
#23721=CARTESIAN_POINT ( 'NONE',  ( -10.12326195556307695, -13.32541703369907893, 74.86313051124790263 ) ) ;
#23722=( BOUNDED_CURVE ( )  B_SPLINE_CURVE ( 3, ( #4809, #15621, #11959, #12673 ),
 .UNSPECIFIED., .F., .T. ) 
 B_SPLINE_CURVE_WITH_KNOTS ( ( 4, 4 ),
 ( 0.4074455897393560178, 0.5000000000000000000 ),
 .UNSPECIFIED. ) 
 CURVE ( )  GEOMETRIC_REPRESENTATION_ITEM ( )  RATIONAL_B_SPLINE_CURVE ( ( 0.6983129098260760781, 0.7760317562606792174, 0.8765941196519858591, 0.9999999999999930056 ) ) 
 REPRESENTATION_ITEM ( '' )  );
#23723=VERTEX_POINT ( 'NONE', #26733 ) ;
#23724=CARTESIAN_POINT ( 'NONE',  ( -10.38078070663892660, -14.50222156296673148, 67.85800126083267969 ) ) ;
#23725=CARTESIAN_POINT ( 'NONE',  ( -12.41310947992116098, -19.76871611099698001, 61.68206578716802113 ) ) ;
#23726=CARTESIAN_POINT ( 'NONE',  ( -18.75796263175485734, -7.882761566875607251, 74.14064681633755072 ) ) ;
#23727=ORIENTED_EDGE ( 'NONE', *, *, #14735, .F. ) ;
#23729=CARTESIAN_POINT ( 'NONE',  ( -21.99213670719075253, -20.17946569659695655, 59.04970794435396897 ) ) ;
#23730=AXIS2_PLACEMENT_3D ( 'NONE', #47377, #36270, #25445 ) ;
#23732=CARTESIAN_POINT ( 'NONE',  ( -24.37533454541335232, -13.98391229038511163, 73.40806141292473797 ) ) ;
#23733=DIRECTION ( 'NONE',  ( -0.7971031148784508691, 0.6038432116460915600, -6.916509187980531058E-08 ) ) ;
#23737=ADVANCED_FACE ( 'NONE', ( #4557 ), #34586, .F. ) ;
#23739=ORIENTED_EDGE ( 'NONE', *, *, #27796, .T. ) ;
#23740=FACE_OUTER_BOUND ( 'NONE', #33696, .T. ) ;
#23742=ORIENTED_EDGE ( 'NONE', *, *, #23693, .T. ) ;
#23743=CARTESIAN_POINT ( 'NONE',  ( -20.60942684424193416, -21.09890871138989965, 58.65947248567252359 ) ) ;
#23744=CARTESIAN_POINT ( 'NONE',  ( -14.54749350918765671, -8.372447261038937327, 64.07506791522041567 ) ) ;
#23745=LINE ( 'NONE', #38738, #23158 ) ;
#23746=CARTESIAN_POINT ( 'NONE',  ( -12.71429358501400131, -19.98796095756949143, 68.33657440636297054 ) ) ;
#23747=FACE_OUTER_BOUND ( 'NONE', #28528, .T. ) ;
#23748=VERTEX_POINT ( 'NONE', #11704 ) ;
#23749=CARTESIAN_POINT ( 'NONE',  ( -24.79887126163464828, -15.86559147609933618, 69.64033351364996349 ) ) ;
#23750=CARTESIAN_POINT ( 'NONE',  ( -17.22364295584634775, -7.762016434835315337, 70.49035836927656362 ) ) ;
#23751=EDGE_CURVE ( 'NONE', #30534, #24642, #45448, .T. ) ;
#23753=CARTESIAN_POINT ( 'NONE',  ( -10.09142662841313332, -16.12648724910785702, 68.08429501313727883 ) ) ;
#23754=EDGE_LOOP ( 'NONE', ( #41646, #28857, #19403, #13044, #42883 ) ) ;
#23755=CARTESIAN_POINT ( 'NONE',  ( -17.13503149044196405, -7.764836982087095052, 70.77563787455143540 ) ) ;
#23759=CARTESIAN_POINT ( 'NONE',  ( -23.91632973644556159, -12.05317525496800357, 59.89724340139424896 ) ) ;
#23761=CARTESIAN_POINT ( 'NONE',  ( -11.08846142298070880, -18.82290330472913098, 53.49999999999994316 ) ) ;
#23762=EDGE_LOOP ( 'NONE', ( #44644, #25526 ) ) ;
#23763=ORIENTED_EDGE ( 'NONE', *, *, #2089, .T. ) ;
#23767=CARTESIAN_POINT ( 'NONE',  ( -21.02205230129062485, -8.737166911425223503, 59.98558246646761916 ) ) ;
#23768=DIRECTION ( 'NONE',  ( 0.8603613874411334406, -0.3191920208248665292, 0.3973597071195140162 ) ) ;
#23769=CARTESIAN_POINT ( 'NONE',  ( -24.46356860818091405, -14.42337734487177947, 66.48292728742831059 ) ) ;
#23770=ORIENTED_EDGE ( 'NONE', *, *, #92, .F. ) ;
#23771=CARTESIAN_POINT ( 'NONE',  ( -24.17969144601942233, -17.95015662838525117, 59.04732501252154009 ) ) ;
#23773=EDGE_LOOP ( 'NONE', ( #21869, #28064, #10755, #39523, #41233 ) ) ;
#23774=CARTESIAN_POINT ( 'NONE',  ( -10.33531692083374587, -17.10115316349580894, 57.87255846826901262 ) ) ;
#23775=DIRECTION ( 'NONE',  ( -0.1675476790616295397, 0.9858639740050658684, -1.006000811662239041E-16 ) ) ;
#23776=ORIENTED_EDGE ( 'NONE', *, *, #17576, .T. ) ;
#23777=CARTESIAN_POINT ( 'NONE',  ( -10.34546495671637700, -12.48638223296730487, 60.94853567734574540 ) ) ;
#23779=EDGE_CURVE ( 'NONE', #47586, #19229, #46420, .T. ) ;
#23780=CARTESIAN_POINT ( 'NONE',  ( -10.00117625416208433, -15.44487358686203571, 57.68297391752145842 ) ) ;
#23784=CARTESIAN_POINT ( 'NONE',  ( -20.88891245741970693, -21.40461089374386461, 58.76662411742747594 ) ) ;
#23785=CARTESIAN_POINT ( 'NONE',  ( -23.80941655268207668, -18.64734661885979961, 72.80722282987319716 ) ) ;
#23786=FACE_OUTER_BOUND ( 'NONE', #30744, .T. ) ;
#23788=CARTESIAN_POINT ( 'NONE',  ( -14.22441497990486958, -8.081217732231424478, 67.44470516081543110 ) ) ;
#23789=CARTESIAN_POINT ( 'NONE',  ( -17.19167086870822203, -7.760035283349824731, 66.90551000485606892 ) ) ;
#23790=CARTESIAN_POINT ( 'NONE',  ( -24.39763799706551950, -15.84669482609578317, 69.54779622430706354 ) ) ;
#23791=ORIENTED_EDGE ( 'NONE', *, *, #31104, .F. ) ;
#23793=( BOUNDED_CURVE ( )  B_SPLINE_CURVE ( 3, ( #16771, #1522, #42421, #8691 ),
 .UNSPECIFIED., .F., .F. ) 
 B_SPLINE_CURVE_WITH_KNOTS ( ( 4, 4 ),
 ( 0.5000000000000000000, 0.9074455897393663983 ),
 .UNSPECIFIED. ) 
 CURVE ( )  GEOMETRIC_REPRESENTATION_ITEM ( )  RATIONAL_B_SPLINE_CURVE ( ( 1.000000000000007994, 0.4567392136813297476, 0.3561768502900237165, 0.6983129098260987266 ) ) 
 REPRESENTATION_ITEM ( '' )  );
#23795=CARTESIAN_POINT ( 'NONE',  ( -21.52726260838264949, -9.076274878514672295, 70.13132538915753855 ) ) ;
#23796=LINE ( 'NONE', #5078, #726 ) ;
#23797=ORIENTED_EDGE ( 'NONE', *, *, #41449, .F. ) ;
#23798=B_SPLINE_CURVE_WITH_KNOTS ( 'NONE', 3,
 ( #2895, #6607, #40816, #25324, #40102, #10779, #47722, #25799, #25553, #44057 ),
 .UNSPECIFIED., .F., .F.,
 ( 4, 2, 2, 2, 4 ),
 ( 0.000000000000000000, 0.2500000000000000000, 0.5000000000000000000, 0.7500000000000000000, 1.000000000000000000 ),
 .UNSPECIFIED. ) ;
#23799=PLANE ( 'NONE',  #16907 ) ;
#23800=FACE_BOUND ( 'NONE', #8651, .T. ) ;
#23802=ORIENTED_EDGE ( 'NONE', *, *, #38164, .F. ) ;
#23804=EDGE_CURVE ( 'NONE', #16133, #8440, #23722, .T. ) ;
#23808=FACE_OUTER_BOUND ( 'NONE', #32578, .T. ) ;
#23809=CARTESIAN_POINT ( 'NONE',  ( -14.51896091561126489, -8.440036020032167130, 67.54358485890664099 ) ) ;
#23810=CARTESIAN_POINT ( 'NONE',  ( -12.68381401182790569, -19.95991009262169413, 68.33657438305763776 ) ) ;
#23811=CARTESIAN_POINT ( 'NONE',  ( -10.74141550158114455, -16.89327759150595654, 57.98760574264920109 ) ) ;
#23813=VERTEX_POINT ( 'NONE', #31142 ) ;
#23814=EDGE_CURVE ( 'NONE', #28527, #28606, #19089, .T. ) ;
#23816=CARTESIAN_POINT ( 'NONE',  ( -21.59671027634132656, -20.98115415594247324, 72.56800473755950520 ) ) ;
#23817=CARTESIAN_POINT ( 'NONE',  ( -12.64995480627295521, -19.99670077279894898, 68.48657438322858582 ) ) ;
#23818=CARTESIAN_POINT ( 'NONE',  ( -21.60699152411756074, -9.194825043480776117, 70.35962493737054047 ) ) ;
#23819=ORIENTED_EDGE ( 'NONE', *, *, #15829, .F. ) ;
#23820=EDGE_CURVE ( 'NONE', #35582, #24088, #18403, .T. ) ;
#23822=ORIENTED_EDGE ( 'NONE', *, *, #30640, .T. ) ;
#23823=CARTESIAN_POINT ( 'NONE',  ( -23.05110005139504636, -10.64472189410646230, 59.61820115093192385 ) ) ;
#23824=CARTESIAN_POINT ( 'NONE',  ( -12.48641702280725951, -19.77161301655056036, 64.88291470187951404 ) ) ;
#23825=ORIENTED_EDGE ( 'NONE', *, *, #11737, .T. ) ;
#23826=CARTESIAN_POINT ( 'NONE',  ( -11.63855442814814367, -18.75048355864383609, 68.50073137068018525 ) ) ;
#23827=B_SPLINE_CURVE_WITH_KNOTS ( 'NONE', 3,
 ( #41855, #8130, #4413, #19433, #34438, #31974, #27556, #23875, #9819, #35417 ),
 .UNSPECIFIED., .F., .F.,
 ( 4, 2, 2, 2, 4 ),
 ( 0.6272669072878033214, 0.7522669073073137147, 0.8772669073268239970, 1.002266907346334390, 1.127266907365844784 ),
 .UNSPECIFIED. ) ;
#23828=CARTESIAN_POINT ( 'NONE',  ( -10.78898398081525301, -17.19290454168847404, 61.44271037915215317 ) ) ;
#23829=CARTESIAN_POINT ( 'NONE',  ( -10.42774853574490201, -14.58114972691745947, 68.14334793592969675 ) ) ;
#23830=FACE_OUTER_BOUND ( 'NONE', #45018, .T. ) ;
#23831=VERTEX_POINT ( 'NONE', #31641 ) ;
#23832=CARTESIAN_POINT ( 'NONE',  ( -15.97284114023201695, -21.71201116376809992, 58.58585868367167393 ) ) ;
#23834=EDGE_CURVE ( 'NONE', #38000, #28514, #28968, .T. ) ;
#23835=CARTESIAN_POINT ( 'NONE',  ( -17.46222794319647775, -7.759011850482251837, 67.03511641684839617 ) ) ;
#23836=CARTESIAN_POINT ( 'NONE',  ( -20.10974094956083746, -7.859941204851112140, 73.85950125338895589 ) ) ;
#23837=ORIENTED_EDGE ( 'NONE', *, *, #17489, .T. ) ;
#23838=PLANE ( 'NONE',  #44065 ) ;
#23840=CARTESIAN_POINT ( 'NONE',  ( -19.22059177161013110, -7.579041592493069857, 63.53114993777460029 ) ) ;
#23841=CARTESIAN_POINT ( 'NONE',  ( -14.65746096889331263, -8.316078616448901784, 57.00567256703398300 ) ) ;
#23842=ORIENTED_EDGE ( 'NONE', *, *, #21154, .T. ) ;
#23844=CARTESIAN_POINT ( 'NONE',  ( -24.64680953583212286, -12.98235456786829367, 62.99297500150433393 ) ) ;
#23846=CYLINDRICAL_SURFACE ( 'NONE', #26667, 0.1499999999999963862 ) ;
#23848=CARTESIAN_POINT ( 'NONE',  ( -23.66043351732632871, -18.11420823279021519, 59.14811234476497503 ) ) ;
#23849=CARTESIAN_POINT ( 'NONE',  ( -15.18822458420557453, -21.91583580787659713, 68.76867073792189444 ) ) ;
#23851=CARTESIAN_POINT ( 'NONE',  ( -15.43182990062313742, -8.046249867383863830, 74.36513541778452918 ) ) ;
#23852=B_SPLINE_CURVE_WITH_KNOTS ( 'NONE', 1,
 ( #41463, #30887 ),
 .UNSPECIFIED., .F., .F.,
 ( 2, 2 ),
 ( 0.000000000000000000, 1.000000000000000000 ),
 .UNSPECIFIED. ) ;
#23853=ORIENTED_EDGE ( 'NONE', *, *, #19836, .F. ) ;
#23854=EDGE_CURVE ( 'NONE', #25935, #16796, #23999, .T. ) ;
#23855=CARTESIAN_POINT ( 'NONE',  ( -10.64264583514116147, -11.72452599650507565, 74.66566005422028240 ) ) ;
#23856=( BOUNDED_SURFACE ( )  B_SPLINE_SURFACE ( 3, 1, ( 
 ( #4488, #19026 ),
 ( #26911, #38204 ),
 ( #4742, #7966 ),
 ( #45149, #37473 ),
 ( #3765, #802 ),
 ( #18777, #15067 ),
 ( #4019, #11392 ) ),
 .UNSPECIFIED., .T., .F., .F. ) 
 B_SPLINE_SURFACE_WITH_KNOTS ( ( 4, 3, 4 ),
 ( 2, 2 ),
 ( 0.000000000000000000, 0.5000000000000000000, 1.000000000000000000 ),
 ( 0.000000000000000000, 1.000000000000000000 ),
 .UNSPECIFIED. ) 
 GEOMETRIC_REPRESENTATION_ITEM ( )  RATIONAL_B_SPLINE_SURFACE ( (
 ( 1.000000000000000000, 1.000000000000000000),
 ( 0.3333333333333335369, 0.3333333333333330373),
 ( 0.3333333333333335369, 0.3333333333333330373),
 ( 1.000000000000000000, 1.000000000000000000),
 ( 0.3333333333333333703, 0.3333333333333333703),
 ( 0.3333333333333333703, 0.3333333333333333703),
 ( 1.000000000000000000, 1.000000000000000000) ) ) 
 REPRESENTATION_ITEM ( '' )  SURFACE ( )  );
#23857=CARTESIAN_POINT ( 'NONE',  ( -24.74075724160099554, -16.21284971877490122, 62.77824058731629009 ) ) ;
#23858=VERTEX_POINT ( 'NONE', #2073 ) ;
#23859=ORIENTED_EDGE ( 'NONE', *, *, #47997, .T. ) ;
#23860=CARTESIAN_POINT ( 'NONE',  ( -20.60942684424193416, -21.09890871138989965, 58.65947248567252359 ) ) ;
#23861=CARTESIAN_POINT ( 'NONE',  ( -13.07007069224803786, -8.763865476245500830, 64.16592477169881192 ) ) ;
#23862=CARTESIAN_POINT ( 'NONE',  ( -10.42619869066336591, -14.62054329830827193, 71.61166091316889037 ) ) ;
#23865=DIRECTION ( 'NONE',  ( 0.9577883914167855117, 0.2682351919075576796, 0.1033986416233888400 ) ) ;
#23866=CARTESIAN_POINT ( 'NONE',  ( -18.63708974648904615, -7.458494484969275362, 74.01877187527500723 ) ) ;
#23867=CARTESIAN_POINT ( 'NONE',  ( -23.70580769785572883, -18.01777564070315663, 59.30378467840713341 ) ) ;
#23868=ORIENTED_EDGE ( 'NONE', *, *, #19788, .F. ) ;
#23875=CARTESIAN_POINT ( 'NONE',  ( -24.55229515441413923, -12.64323416470515582, 69.87268757599312607 ) ) ;
#23876=EDGE_CURVE ( 'NONE', #33222, #32753, #13689, .T. ) ;
#23877=LINE ( 'NONE', #15726, #45720 ) ;
#23879=CARTESIAN_POINT ( 'NONE',  ( -14.99986034619465158, -21.37608775269596961, 61.65102924131838336 ) ) ;
#23880=CARTESIAN_POINT ( 'NONE',  ( -24.46812100523181499, -14.51191712007779522, 66.19764790277996269 ) ) ;
#23882=CARTESIAN_POINT ( 'NONE',  ( -24.46506355971582991, -17.24406257311080992, 72.99840714145864240 ) ) ;
#23884=VERTEX_POINT ( 'NONE', #27932 ) ;
#23885=ADVANCED_FACE ( 'NONE', ( #6012 ), #9484, .T. ) ;
#23886=CARTESIAN_POINT ( 'NONE',  ( -20.78451513435706133, -21.00713107796517320, 62.12943504870421663 ) ) ;
#23888=EDGE_CURVE ( 'NONE', #10981, #38205, #17788, .T. ) ;
#23889=ADVANCED_FACE ( 'NONE', ( #31876 ), #43209, .T. ) ;
#23890=ORIENTED_EDGE ( 'NONE', *, *, #25774, .F. ) ;
#23891=CARTESIAN_POINT ( 'NONE',  ( -12.88852986233651876, -20.14113829381898668, 71.82156135014017195 ) ) ;
#23892=CARTESIAN_POINT ( 'NONE',  ( -22.09360120700997854, -20.02631313764212706, 65.81494753366123973 ) ) ;
#23893=ORIENTED_EDGE ( 'NONE', *, *, #41325, .T. ) ;
#23894=CARTESIAN_POINT ( 'NONE',  ( -21.89826263122328953, -8.852228171720549099, 66.84645388252840803 ) ) ;
#23895=ORIENTED_EDGE ( 'NONE', *, *, #36502, .F. ) ;
#23897=CARTESIAN_POINT ( 'NONE',  ( -21.67609690912980014, -8.690862426448951794, 73.78784151156415305 ) ) ;
#23900=CARTESIAN_POINT ( 'NONE',  ( -10.27345454978659944, -12.71824136398891980, 64.45331520391344782 ) ) ;
#23903=ORIENTED_EDGE ( 'NONE', *, *, #45645, .T. ) ;
#23905=CARTESIAN_POINT ( 'NONE',  ( -19.17247957453286844, -7.567181637230756763, 63.61584517348745038 ) ) ;
#23906=LINE ( 'NONE', #24142, #25835 ) ;
#23907=VERTEX_POINT ( 'NONE', #47626 ) ;
#23909=CARTESIAN_POINT ( 'NONE',  ( -23.83833616213321704, -17.61232902345998141, 62.77360984984811410 ) ) ;
#23911=CARTESIAN_POINT ( 'NONE',  ( -12.91576191806997365, -9.388722997169709927, 71.13453240065665284 ) ) ;
#23912=CARTESIAN_POINT ( 'NONE',  ( -19.23866403772855449, -21.62168293227472660, 58.67507384656568092 ) ) ;
#23913=EDGE_CURVE ( 'NONE', #10765, #5443, #133, .T. ) ;
#23916=CARTESIAN_POINT ( 'NONE',  ( -23.75972628784533569, -10.79550978475970346, 53.49999999999994316 ) ) ;
#23917=CARTESIAN_POINT ( 'NONE',  ( -15.09857480863590062, -8.145354156905789011, 60.46428990550709415 ) ) ;
#23919=CARTESIAN_POINT ( 'NONE',  ( -24.49635653881819408, -12.46679777644911447, 73.35730153580948354 ) ) ;
#23922=CARTESIAN_POINT ( 'NONE',  ( -12.60227155074094441, -19.95281705956671559, 68.35129494334645983 ) ) ;
#23923=CARTESIAN_POINT ( 'NONE',  ( -11.23768813171194836, -11.42793793434924154, 64.44322231037519089 ) ) ;
#23924=ORIENTED_EDGE ( 'NONE', *, *, #22928, .F. ) ;
#23925=EDGE_CURVE ( 'NONE', #25179, #9970, #13612, .T. ) ;
#23926=CARTESIAN_POINT ( 'NONE',  ( -22.52619951119469022, -19.67884242972143483, 69.05929390617204433 ) ) ;
#23927=CARTESIAN_POINT ( 'NONE',  ( -20.73702204056089826, -8.642680056431577995, 59.84125279967195610 ) ) ;
#23928=CARTESIAN_POINT ( 'NONE',  ( -12.32158608955787393, -9.943909642237139579, 60.57390139315987909 ) ) ;
#23930=CARTESIAN_POINT ( 'NONE',  ( -12.96596342764269316, -9.347744029417796696, 71.14925352873375175 ) ) ;
#23931=VERTEX_POINT ( 'NONE', #47144 ) ;
#23932=ORIENTED_EDGE ( 'NONE', *, *, #4313, .F. ) ;
#23935=CARTESIAN_POINT ( 'NONE',  ( -23.04402284766838349, -19.06632961612601918, 59.16938527523783620 ) ) ;
#23936=AXIS2_PLACEMENT_3D ( 'NONE', #9907, #42913, #20745 ) ;
#23937=CARTESIAN_POINT ( 'NONE',  ( -24.09502166851904903, -12.68799014041620055, 69.78745416573572413 ) ) ;
#23938=EDGE_LOOP ( 'NONE', ( #43529, #39876, #19417, #44369, #46971 ) ) ;
#23939=B_SPLINE_CURVE_WITH_KNOTS ( 'NONE', 1,
 ( #9432, #9678 ),
 .UNSPECIFIED., .F., .F.,
 ( 2, 2 ),
 ( 0.000000000000000000, 1.000000000000000000 ),
 .UNSPECIFIED. ) ;
#23940=ADVANCED_FACE ( 'NONE', ( #6261 ), #29148, .T. ) ;
#23941=CARTESIAN_POINT ( 'NONE',  ( -21.89826351590202336, -8.852228842849337198, 66.84645279485334868 ) ) ;
#23942=FACE_OUTER_BOUND ( 'NONE', #13771, .T. ) ;
#23945=ORIENTED_EDGE ( 'NONE', *, *, #22863, .F. ) ;
#23946=CARTESIAN_POINT ( 'NONE',  ( -20.95083147400204382, -8.246703318114343872, 60.01938016961330646 ) ) ;
#23947=CARTESIAN_POINT ( 'NONE',  ( -19.23951954158338751, -22.03540154427634334, 58.71162761787055473 ) ) ;
#23948=ORIENTED_EDGE ( 'NONE', *, *, #31774, .T. ) ;
#23949=CARTESIAN_POINT ( 'NONE',  ( -11.37640603946425522, -11.28103799867411894, 64.25955191458184856 ) ) ;
#23950=LINE ( 'NONE', #8694, #44798 ) ;
#23952=EDGE_CURVE ( 'NONE', #15615, #4181, #28728, .T. ) ;
#23953=CARTESIAN_POINT ( 'NONE',  ( -22.79734292848665689, -10.24514101169484448, 66.84182257473258915 ) ) ;
#23955=CARTESIAN_POINT ( 'NONE',  ( -19.45676940763031837, -21.56358822076535375, 58.73327141882466407 ) ) ;
#23956=ORIENTED_EDGE ( 'NONE', *, *, #6598, .F. ) ;
#23959=CARTESIAN_POINT ( 'NONE',  ( -17.87433636498385781, -21.79471166626661827, 58.59656648677060531 ) ) ;
#23961=CARTESIAN_POINT ( 'NONE',  ( -24.32752865423570654, -15.96790753223159598, 66.36324927017490438 ) ) ;
#23965=CARTESIAN_POINT ( 'NONE',  ( -10.98557813051190202, -17.68114236276378293, 71.56718193507127523 ) ) ;
#23966=CARTESIAN_POINT ( 'NONE',  ( -24.86610167639389246, -14.46236660854407674, 66.29797298380238146 ) ) ;
#23968=CARTESIAN_POINT ( 'NONE',  ( -14.19679379891342741, -21.02091897117797004, 71.99895702512269224 ) ) ;
#23970=EDGE_CURVE ( 'NONE', #22263, #9283, #13857, .T. ) ;
#23971=AXIS2_PLACEMENT_3D ( 'NONE', #3176, #24867, #18182 ) ;
#23972=ORIENTED_EDGE ( 'NONE', *, *, #4051, .T. ) ;
#23973=DIRECTION ( 'NONE',  ( -5.731567514496413899E-31, -1.020425574103664789E-16, -1.000000000000000000 ) ) ;
#23974=CARTESIAN_POINT ( 'NONE',  ( -19.17247849636888901, -7.567181371456696226, 63.61584626116109575 ) ) ;
#23975=VERTEX_POINT ( 'NONE', #22488 ) ;
#23976=CARTESIAN_POINT ( 'NONE',  ( -24.45714095472541771, -14.31630891555219165, 69.66747352629326429 ) ) ;
#23978=CARTESIAN_POINT ( 'NONE',  ( -11.25989503537269698, -11.38792718504117829, 64.29882039368452240 ) ) ;
#23979=CARTESIAN_POINT ( 'NONE',  ( -22.94192455449829993, -9.803488759991966006, 70.05532601532212311 ) ) ;
#23981=( BOUNDED_SURFACE ( )  B_SPLINE_SURFACE ( 3, 1, ( 
 ( #13230, #16455 ),
 ( #31487, #12775 ),
 ( #34930, #9093 ),
 ( #39360, #27789 ),
 ( #35169, #28282 ),
 ( #42334, #24602 ),
 ( #15965, #16202 ) ),
 .UNSPECIFIED., .T., .F., .F. ) 
 B_SPLINE_SURFACE_WITH_KNOTS ( ( 4, 3, 4 ),
 ( 2, 2 ),
 ( 0.000000000000000000, 0.5000000000000000000, 1.000000000000000000 ),
 ( 0.000000000000000000, 1.000000000000000000 ),
 .UNSPECIFIED. ) 
 GEOMETRIC_REPRESENTATION_ITEM ( )  RATIONAL_B_SPLINE_SURFACE ( (
 ( 1.000000000000000000, 1.000000000000000000),
 ( 0.3333333333333335369, 0.3333333333333330373),
 ( 0.3333333333333335369, 0.3333333333333330373),
 ( 1.000000000000000000, 1.000000000000000000),
 ( 0.3333333333333333703, 0.3333333333333333703),
 ( 0.3333333333333333703, 0.3333333333333333703),
 ( 1.000000000000000000, 1.000000000000000000) ) ) 
 REPRESENTATION_ITEM ( '' )  SURFACE ( )  );
#23983=CARTESIAN_POINT ( 'NONE',  ( -24.79781836340079337, -15.87314503134675014, 69.64812095075065201 ) ) ;
#23985=CARTESIAN_POINT ( 'NONE',  ( -12.50648677543191134, -9.746390325112967545, 60.70350793514798937 ) ) ;
#23986=EDGE_CURVE ( 'NONE', #48343, #1260, #32549, .T. ) ;
#23987=ORIENTED_EDGE ( 'NONE', *, *, #44706, .T. ) ;
#23988=DIRECTION ( 'NONE',  ( 2.723496474639940985E-06, 1.584719855340916648E-07, 0.9999999999962787545 ) ) ;
#23989=CARTESIAN_POINT ( 'NONE',  ( -24.20884313412962285, -11.73171478914054155, 59.59740407230526671 ) ) ;
#23991=CARTESIAN_POINT ( 'NONE',  ( -21.78913961794832588, -8.771810275399618106, 70.24637145832762997 ) ) ;
#23992=CARTESIAN_POINT ( 'NONE',  ( -10.71495605983455590, -12.81234157828920850, 64.26836111193937029 ) ) ;
#23993=( BOUNDED_SURFACE ( )  B_SPLINE_SURFACE ( 3, 1, ( 
 ( #23600, #34409 ),
 ( #30266, #33936 ),
 ( #45286, #22620 ),
 ( #3917, #19166 ),
 ( #38109, #464 ),
 ( #8577, #37874 ),
 ( #11535, #7616 ) ),
 .UNSPECIFIED., .T., .F., .F. ) 
 B_SPLINE_SURFACE_WITH_KNOTS ( ( 4, 3, 4 ),
 ( 2, 2 ),
 ( 0.000000000000000000, 0.5000000000000000000, 1.000000000000000000 ),
 ( 0.000000000000000000, 1.000000000000000000 ),
 .UNSPECIFIED. ) 
 GEOMETRIC_REPRESENTATION_ITEM ( )  RATIONAL_B_SPLINE_SURFACE ( (
 ( 1.000000000000000000, 1.000000000000000000),
 ( 0.3333333333333335369, 0.3333333333333330373),
 ( 0.3333333333333335369, 0.3333333333333330373),
 ( 1.000000000000000000, 1.000000000000000000),
 ( 0.3333333333333333703, 0.3333333333333333703),
 ( 0.3333333333333333703, 0.3333333333333333703),
 ( 1.000000000000000000, 1.000000000000000000) ) ) 
 REPRESENTATION_ITEM ( '' )  SURFACE ( )  );
#23995=ORIENTED_EDGE ( 'NONE', *, *, #12269, .T. ) ;
#23997=CARTESIAN_POINT ( 'NONE',  ( -24.87123160714014958, -14.59964084223042491, 62.89791924484052998 ) ) ;
#23998=CARTESIAN_POINT ( 'NONE',  ( -20.02766308627097303, -8.311286154507662616, 73.72096589762166730 ) ) ;
#23999=( BOUNDED_CURVE ( )  B_SPLINE_CURVE ( 3, ( #13626, #35797, #1592, #28185 ),
 .UNSPECIFIED., .F., .F. ) 
 B_SPLINE_CURVE_WITH_KNOTS ( ( 4, 4 ),
 ( 0.5000000000000000000, 0.9074455897393656212 ),
 .UNSPECIFIED. ) 
 CURVE ( )  GEOMETRIC_REPRESENTATION_ITEM ( )  RATIONAL_B_SPLINE_CURVE ( ( 1.000000000000009992, 0.4567392136813407388, 0.3561768502900264366, 0.6983129098260781875 ) ) 
 REPRESENTATION_ITEM ( '' )  );
#24000=CIRCLE ( 'NONE', #12967, 7.500000000000002665 ) ;
#24001=LINE ( 'NONE', #43445, #3281 ) ;
#24002=EDGE_CURVE ( 'NONE', #35502, #21615, #32826, .T. ) ;
#24004=AXIS2_PLACEMENT_3D ( 'NONE', #19477, #4714, #4461 ) ;
#24005=ORIENTED_EDGE ( 'NONE', *, *, #24132, .T. ) ;
#24006=CARTESIAN_POINT ( 'NONE',  ( -12.40133225487197066, -17.08293507921495191, 53.69233794759168887 ) ) ;
#24007=CARTESIAN_POINT ( 'NONE',  ( -18.05316936118225968, -22.23335149483498085, 65.53187476518867527 ) ) ;
#24009=CARTESIAN_POINT ( 'NONE',  ( -21.84891708756835982, -9.316868653145983004, 67.07638807817237137 ) ) ;
#24011=VERTEX_POINT ( 'NONE', #44918 ) ;
#24013=B_SPLINE_CURVE_WITH_KNOTS ( 'NONE', 3,
 ( #40437, #13353, #2537, #10171, #36712, #31848, #13110, #32091, #5981, #24714 ),
 .UNSPECIFIED., .F., .F.,
 ( 4, 2, 2, 2, 4 ),
 ( 0.000000000000000000, 0.2500000000000000000, 0.5000000000000000000, 0.7500000000000000000, 1.000000000000000000 ),
 .UNSPECIFIED. ) ;
#24016=CARTESIAN_POINT ( 'NONE',  ( -14.78766009005058635, -21.34800739930362568, 58.45145834864037937 ) ) ;
#24017=ORIENTED_EDGE ( 'NONE', *, *, #28188, .T. ) ;
#24018=CARTESIAN_POINT ( 'NONE',  ( -17.77920954038207668, -22.25082405446125122, 58.59048702730397196 ) ) ;
#24019=ADVANCED_FACE ( 'NONE', ( #33294 ), #34039, .T. ) ;
#24020=CARTESIAN_POINT ( 'NONE',  ( -11.86838291625971742, -9.845553222893467904, 64.14418898700822069 ) ) ;
#24022=CARTESIAN_POINT ( 'NONE',  ( -10.34976723757024253, -12.47327135604617787, 60.89879317984863860 ) ) ;
#24023=CARTESIAN_POINT ( 'NONE',  ( -24.30537518760159088, -16.09989623713234863, 66.29154897911506339 ) ) ;
#24024=EDGE_LOOP ( 'NONE', ( #4193, #26351, #34762, #9541, #20220 ) ) ;
#24025=CARTESIAN_POINT ( 'NONE',  ( -10.31364510401727053, -17.03300888149450998, 57.80265138661536639 ) ) ;
#24026=CARTESIAN_POINT ( 'NONE',  ( -24.83515304063678286, -14.04764234229505959, 73.23776096988058271 ) ) ;
#24027=FACE_OUTER_BOUND ( 'NONE', #2709, .T. ) ;
#24030=CARTESIAN_POINT ( 'NONE',  ( -11.42128300986745515, -11.20812281556079171, 60.67885827005227384 ) ) ;
#24031=EDGE_CURVE ( 'NONE', #6094, #20234, #1983, .T. ) ;
#24032=CARTESIAN_POINT ( 'NONE',  ( -24.37499929849812119, -16.00910627056057223, 69.83307750944575787 ) ) ;
#24033=ORIENTED_EDGE ( 'NONE', *, *, #24228, .F. ) ;
#24034=CARTESIAN_POINT ( 'NONE',  ( -12.10507042601503080, -10.25792974195034901, 67.51513498652721523 ) ) ;
#24035=EDGE_LOOP ( 'NONE', ( #2885, #19999 ) ) ;
#24036=CARTESIAN_POINT ( 'NONE',  ( -11.79630000206883977, -19.05592701419838519, 71.97213747039440079 ) ) ;
#24037=CARTESIAN_POINT ( 'NONE',  ( -20.64108208740726624, -21.08661300460041232, 62.41471558431330635 ) ) ;
#24039=CARTESIAN_POINT ( 'NONE',  ( -23.52949419687348964, -11.28347464189849525, 70.17738639980606763 ) ) ;
#24041=FACE_BOUND ( 'NONE', #16492, .T. ) ;
#24042=VERTEX_POINT ( 'NONE', #42179 ) ;
#24043=ORIENTED_EDGE ( 'NONE', *, *, #42286, .T. ) ;
#24045=CARTESIAN_POINT ( 'NONE',  ( -10.01366804335076210, -15.58332129913256381, 61.22444385224647334 ) ) ;
#24047=CARTESIAN_POINT ( 'NONE',  ( -21.21196263389317949, -8.922607336573463499, 73.71014652413226997 ) ) ;
#24048=CARTESIAN_POINT ( 'NONE',  ( -12.62620118243013856, -19.90688802239219868, 68.35274030346421625 ) ) ;
#24049=DIRECTION ( 'NONE',  ( 0.4415479322351505975, 0.8912598635915908174, 0.1033986416233889788 ) ) ;
#24050=ORIENTED_EDGE ( 'NONE', *, *, #4779, .F. ) ;
#24051=ORIENTED_EDGE ( 'NONE', *, *, #29389, .T. ) ;
#24053=CARTESIAN_POINT ( 'NONE',  ( -21.39967327233876659, -20.63170314183283693, 72.80974286114339122 ) ) ;
#24055=CARTESIAN_POINT ( 'NONE',  ( -24.07511766164941491, -16.99203022981017952, 72.89838494284886394 ) ) ;
#24058=ORIENTED_EDGE ( 'NONE', *, *, #41790, .T. ) ;
#24060=EDGE_CURVE ( 'NONE', #35848, #18422, #33743, .T. ) ;
#24061=LINE ( 'NONE', #43003, #10373 ) ;
#24062=CARTESIAN_POINT ( 'NONE',  ( -24.47325573560893730, -17.21999967669226450, 73.08347230323211363 ) ) ;
#24063=ORIENTED_EDGE ( 'NONE', *, *, #28982, .F. ) ;
#24064=CARTESIAN_POINT ( 'NONE',  ( -18.44528782684011858, -21.78515541812411982, 72.29983070759432451 ) ) ;
#24065=CARTESIAN_POINT ( 'NONE',  ( -22.30326020397728115, -9.709333660337318150, 73.63728338005337548 ) ) ;
#24066=CARTESIAN_POINT ( 'NONE',  ( -24.16575376147898169, -12.74704232990201724, 69.77243002240838621 ) ) ;
#24067=CARTESIAN_POINT ( 'NONE',  ( -22.18998830427771196, -20.00468049915955859, 65.71893796558269685 ) ) ;
#24068=EDGE_CURVE ( 'NONE', #23164, #27130, #38801, .T. ) ;
#24069=ORIENTED_EDGE ( 'NONE', *, *, #38450, .F. ) ;
#24071=EDGE_CURVE ( 'NONE', #33156, #41728, #7281, .T. ) ;
#24072=CARTESIAN_POINT ( 'NONE',  ( -22.87317432090156899, -19.20579874941482856, 59.07337760154523920 ) ) ;
#24074=ORIENTED_EDGE ( 'NONE', *, *, #22499, .F. ) ;
#24075=DIRECTION ( 'NONE',  ( -0.2664710960620865765, 0.9638429098994649724, -4.833213314675864069E-08 ) ) ;
#24076=ORIENTED_EDGE ( 'NONE', *, *, #11581, .T. ) ;
#24077=CARTESIAN_POINT ( 'NONE',  ( -16.36003703953564070, -21.72797270546592330, 62.05568179787937311 ) ) ;
#24078=EDGE_CURVE ( 'NONE', #34107, #2258, #21401, .T. ) ;
#24080=CARTESIAN_POINT ( 'NONE',  ( -16.36834346081282732, -22.18410778960565466, 61.94063409281806543 ) ) ;
#24081=CARTESIAN_POINT ( 'NONE',  ( -12.18719842096713357, -10.08886484896570934, 64.04386393395434141 ) ) ;
#24082=CARTESIAN_POINT ( 'NONE',  ( -10.80773916950031399, -18.37978238154741462, 54.02312124697530749 ) ) ;
#24083=ORIENTED_EDGE ( 'NONE', *, *, #39163, .F. ) ;
#24084=CARTESIAN_POINT ( 'NONE',  ( -10.63418523514201652, -17.87528017975677130, 71.61072290056861789 ) ) ;
#24086=CARTESIAN_POINT ( 'NONE',  ( -20.72450927900464634, -21.03929139025763106, 58.93003081252663833 ) ) ;
#24087=CARTESIAN_POINT ( 'NONE',  ( -22.22951888192506686, -9.116124670579511147, 59.91445369977274282 ) ) ;
#24088=VERTEX_POINT ( 'NONE', #11902 ) ;
#24089=B_SPLINE_CURVE_WITH_KNOTS ( 'NONE', 1,
 ( #47588, #20756 ),
 .UNSPECIFIED., .F., .F.,
 ( 2, 2 ),
 ( 0.000000000000000000, 1.000000000000000000 ),
 .UNSPECIFIED. ) ;
#24090=CARTESIAN_POINT ( 'NONE',  ( -21.69457540385530336, -9.196023516753362159, 70.54621400560100142 ) ) ;
#24092=ORIENTED_EDGE ( 'NONE', *, *, #10488, .F. ) ;
#24093=DIRECTION ( 'NONE',  ( -0.9998756790481364565, -0.01576789294826319576, -3.907472230461691850E-09 ) ) ;
#24094=CARTESIAN_POINT ( 'NONE',  ( -13.22529448846758804, -9.145569705956512863, 64.19474388871357462 ) ) ;
#24095=CARTESIAN_POINT ( 'NONE',  ( -10.96069698787312596, -18.51437578577013809, 57.92219301334858272 ) ) ;
#24097=CARTESIAN_POINT ( 'NONE',  ( -12.12786991918758339, -13.32596279628197600, 53.49999999999995026 ) ) ;
#24098=DIRECTION ( 'NONE',  ( 0.1555549491741979040, 0.4192882752801622703, 0.8944271909999156334 ) ) ;
#24099=CARTESIAN_POINT ( 'NONE',  ( -24.28579947082789303, -13.18942387424446316, 62.84736316175410309 ) ) ;
#24100=CARTESIAN_POINT ( 'NONE',  ( -18.72680718162379065, -7.880610904852765941, 70.67068030199192208 ) ) ;
#24101=AXIS2_PLACEMENT_3D ( 'NONE', #25044, #39327, #39569 ) ;
#24103=ORIENTED_EDGE ( 'NONE', *, *, #44209, .F. ) ;
#24105=CARTESIAN_POINT ( 'NONE',  ( -24.43827367352892210, -15.52193379869737200, 73.28831629023289906 ) ) ;
#24108=CARTESIAN_POINT ( 'NONE',  ( -14.90981281861414587, -21.39562369906352757, 61.78600440604535748 ) ) ;
#24110=EDGE_CURVE ( 'NONE', #33575, #17355, #5157, .T. ) ;
#24112=CARTESIAN_POINT ( 'NONE',  ( -20.16542227925740249, -21.73660035250202327, 72.44832829956453679 ) ) ;
#24113=CARTESIAN_POINT ( 'NONE',  ( -15.19549097431359463, -21.91815212410659086, 68.76088336006283441 ) ) ;
#24115=CARTESIAN_POINT ( 'NONE',  ( -13.89389072038462025, -21.36980434119256600, 72.11103101793651149 ) ) ;
#24116=( BOUNDED_SURFACE ( )  B_SPLINE_SURFACE ( 3, 1, ( 
 ( #7807, #9433 ),
 ( #19111, #37817 ),
 ( #17025, #19347 ),
 ( #13094, #34117 ),
 ( #11725, #34354 ),
 ( #408, #42916 ),
 ( #28134, #26500 ) ),
 .UNSPECIFIED., .T., .F., .F. ) 
 B_SPLINE_SURFACE_WITH_KNOTS ( ( 4, 3, 4 ),
 ( 2, 2 ),
 ( 0.000000000000000000, 0.5000000000000000000, 1.000000000000000000 ),
 ( 0.000000000000000000, 1.000000000000000000 ),
 .UNSPECIFIED. ) 
 GEOMETRIC_REPRESENTATION_ITEM ( )  RATIONAL_B_SPLINE_SURFACE ( (
 ( 1.000000000000000000, 1.000000000000000000),
 ( 0.3333333333333335369, 0.3333333333333330373),
 ( 0.3333333333333335369, 0.3333333333333330373),
 ( 1.000000000000000000, 1.000000000000000000),
 ( 0.3333333333333333703, 0.3333333333333333703),
 ( 0.3333333333333333703, 0.3333333333333333703),
 ( 1.000000000000000000, 1.000000000000000000) ) ) 
 REPRESENTATION_ITEM ( '' )  SURFACE ( )  );
#24117=ORIENTED_EDGE ( 'NONE', *, *, #12067, .F. ) ;
#24118=B_SPLINE_CURVE_WITH_KNOTS ( 'NONE', 1,
 ( #25161, #40409 ),
 .UNSPECIFIED., .F., .F.,
 ( 2, 2 ),
 ( 0.000000000000000000, 1.000000000000000000 ),
 .UNSPECIFIED. ) ;
#24119=CARTESIAN_POINT ( 'NONE',  ( -20.15023299215415875, -8.307456060669188957, 70.54540580827605822 ) ) ;
#24122=EDGE_CURVE ( 'NONE', #21656, #11148, #44864, .T. ) ;
#24123=CARTESIAN_POINT ( 'NONE',  ( -10.10901086070973420, -13.39385379864076242, 74.79162305847758319 ) ) ;
#24124=CARTESIAN_POINT ( 'NONE',  ( -22.65368503412153700, -20.11523923737162178, 69.37429185709522983 ) ) ;
#24125=CARTESIAN_POINT ( 'NONE',  ( -23.51785832295892931, -11.36449550514380036, 69.89210750611785272 ) ) ;
#24127=CARTESIAN_POINT ( 'NONE',  ( -20.32439191831477032, -7.946881181506595837, 70.35762050598125938 ) ) ;
#24128=( BOUNDED_CURVE ( )  B_SPLINE_CURVE ( 3, ( #30960, #19625, #4605, #26528 ),
 .UNSPECIFIED., .F., .F. ) 
 B_SPLINE_CURVE_WITH_KNOTS ( ( 4, 4 ),
 ( 0.5000000000000000000, 0.9074455897393722825 ),
 .UNSPECIFIED. ) 
 CURVE ( )  GEOMETRIC_REPRESENTATION_ITEM ( )  RATIONAL_B_SPLINE_CURVE ( ( 0.9999999999999737987, 0.4567392136813237524, 0.3561768502900454769, 0.6983129098261104950 ) ) 
 REPRESENTATION_ITEM ( '' )  );
#24129=VECTOR ( 'NONE', #7444, 1000.000000000000227 ) ;
#24130=EDGE_LOOP ( 'NONE', ( #3116, #35315, #32809, #39744, #12400 ) ) ;
#24131=CARTESIAN_POINT ( 'NONE',  ( -17.91451193640577344, -22.24313339626381847, 61.99040498927033127 ) ) ;
#24132=EDGE_CURVE ( 'NONE', #26764, #7211, #19276, .T. ) ;
#24133=CARTESIAN_POINT ( 'NONE',  ( -18.53556661698576136, -22.17591588139245573, 72.40015654177148008 ) ) ;
#24134=VERTEX_POINT ( 'NONE', #38215 ) ;
#24135=DIRECTION ( 'NONE',  ( -5.731567514496413899E-31, -1.020425574103664789E-16, -1.000000000000000000 ) ) ;
#24139=CARTESIAN_POINT ( 'NONE',  ( -15.08687585379459506, -21.46369733121157708, 68.99081615631787656 ) ) ;
#24140=EDGE_CURVE ( 'NONE', #40764, #24808, #9020, .T. ) ;
#24142=CARTESIAN_POINT ( 'NONE',  ( -11.35824856342118494, -11.21643317443627019, 60.97885780702566905 ) ) ;
#24145=CARTESIAN_POINT ( 'NONE',  ( -10.44938425464750331, -17.42781160170326871, 64.88385290183622089 ) ) ;
#24146=CARTESIAN_POINT ( 'NONE',  ( -22.14090652532222236, -20.04928072148792495, 62.51967078134249078 ) ) ;
#24148=CARTESIAN_POINT ( 'NONE',  ( -12.20309502476489882, -20.12380431889209831, 64.98179558605960437 ) ) ;
#24152=CARTESIAN_POINT ( 'NONE',  ( -21.90458132784462109, -18.02218142073060747, 53.69233794759168887 ) ) ;
#24154=CARTESIAN_POINT ( 'NONE',  ( -15.89079584495563502, -7.517933547575396780, 67.32662675182959333 ) ) ;
#24155=CARTESIAN_POINT ( 'NONE',  ( -10.67383815757964527, -12.77521617179723457, 64.26836124819834595 ) ) ;
#24157=CARTESIAN_POINT ( 'NONE',  ( -24.38756562526642213, -15.91227465074931935, 66.34852784166324113 ) ) ;
#24159=CARTESIAN_POINT ( 'NONE',  ( -17.73224099643095286, -22.30287356026373047, 47.99999999999994316 ) ) ;
#24160=CARTESIAN_POINT ( 'NONE',  ( -15.73541995410094785, -8.015833115459232161, 70.90989886597125746 ) ) ;
#24161=EDGE_CURVE ( 'NONE', #20341, #21691, #44146, .T. ) ;
#24162=VERTEX_POINT ( 'NONE', #13082 ) ;
#24164=ADVANCED_FACE ( 'NONE', ( #13322 ), #5485, .T. ) ;
#24165=CARTESIAN_POINT ( 'NONE',  ( -23.75972628784533569, -10.79550978475969991, 54.27966884056655061 ) ) ;
#24167=CARTESIAN_POINT ( 'NONE',  ( -22.85412030071255174, -9.708305165406962089, 73.60444179007319576 ) ) ;
#24168=CARTESIAN_POINT ( 'NONE',  ( -12.77099661245330076, -20.03938978082239331, 72.09037095764423952 ) ) ;
#24169=ORIENTED_EDGE ( 'NONE', *, *, #33890, .F. ) ;
#24171=ORIENTED_EDGE ( 'NONE', *, *, #6809, .T. ) ;
#24172=AXIS2_PLACEMENT_3D ( 'NONE', #20177, #35190, #27807 ) ;
#24174=CARTESIAN_POINT ( 'NONE',  ( -24.46737407909346373, -14.43901797238471474, 62.59807894131280648 ) ) ;
#24177=B_SPLINE_CURVE_WITH_KNOTS ( 'NONE', 3,
 ( #38425, #7939, #15280, #37698, #27355, #26888, #8176, #34005, #23683, #30830 ),
 .UNSPECIFIED., .F., .F.,
 ( 4, 2, 2, 2, 4 ),
 ( 0.6272669072877551377, 0.7522669073072753010, 0.8772669073267955753, 1.002266907346315739, 1.127266907365835902 ),
 .UNSPECIFIED. ) ;
#24178=ORIENTED_EDGE ( 'NONE', *, *, #38220, .F. ) ;
#24181=ORIENTED_EDGE ( 'NONE', *, *, #36170, .T. ) ;
#24182=CARTESIAN_POINT ( 'NONE',  ( -11.19706266256277694, -11.50303319689152737, 67.63336710488009373 ) ) ;
#24183=DIRECTION ( 'NONE',  ( 0.7029450532227031756, 0.7112441579020042370, -7.405715380709557223E-09 ) ) ;
#24185=CARTESIAN_POINT ( 'NONE',  ( -19.99669925590731268, -21.37628624441394010, 68.81993804536961079 ) ) ;
#24186=ORIENTED_EDGE ( 'NONE', *, *, #33187, .F. ) ;
#24187=CARTESIAN_POINT ( 'NONE',  ( -13.47893868739161860, -21.12894084225150237, 65.09354747223889603 ) ) ;
#24188=ORIENTED_EDGE ( 'NONE', *, *, #4183, .T. ) ;
#24189=CARTESIAN_POINT ( 'NONE',  ( -24.47432067347917695, -14.77756146504815327, 59.52828185648635184 ) ) ;
#24191=EDGE_CURVE ( 'NONE', #28056, #34212, #2257, .T. ) ;
#24192=CARTESIAN_POINT ( 'NONE',  ( -24.04523827240123879, -12.53716690146120349, 73.54225551603398969 ) ) ;
#24193=ORIENTED_EDGE ( 'NONE', *, *, #33815, .T. ) ;
#24195=CARTESIAN_POINT ( 'NONE',  ( -14.67111564601650997, -7.886426081561471513, 60.43500846974642116 ) ) ;
#24196=CARTESIAN_POINT ( 'NONE',  ( -21.78444843227217120, -20.35286453386188299, 59.17931667745679647 ) ) ;
#24197=EDGE_CURVE ( 'NONE', #45841, #34358, #10193, .T. ) ;
#24198=CARTESIAN_POINT ( 'NONE',  ( -24.46146587544552276, -14.38248120490118787, 66.46820668217904426 ) ) ;
#24199=CARTESIAN_POINT ( 'NONE',  ( -19.28352822169459202, -22.07505156356299381, 54.27966884056655061 ) ) ;
#24200=CARTESIAN_POINT ( 'NONE',  ( -10.40639875119161495, -17.31059493320988807, 61.29596613180959963 ) ) ;
#24203=VECTOR ( 'NONE', #39441, 1000.000000000000114 ) ;
#24204=CARTESIAN_POINT ( 'NONE',  ( -11.88446955661387783, -10.44372876568607467, 67.38408161429789800 ) ) ;
#24205=CARTESIAN_POINT ( 'NONE',  ( -24.86282145624321771, -14.39856946235243740, 66.37566895130898104 ) ) ;
#24206=CARTESIAN_POINT ( 'NONE',  ( -19.85909425162068942, -21.37257694502213567, 72.64634926892956912 ) ) ;
#24210=CARTESIAN_POINT ( 'NONE',  ( -22.73240514691177339, -10.24592387063649213, 66.84182232556784697 ) ) ;
#24211=CARTESIAN_POINT ( 'NONE',  ( -24.36317976709624489, -13.54274187105164096, 59.66268222191824577 ) ) ;
#24213=CARTESIAN_POINT ( 'NONE',  ( -8.870383383897287644, -17.98261270965173964, 54.44843099904672812 ) ) ;
#24214=CARTESIAN_POINT ( 'NONE',  ( -10.65090795921773292, -13.04125047316982844, 67.73832310984637672 ) ) ;
#24215=( BOUNDED_CURVE ( )  B_SPLINE_CURVE ( 3, ( #37895, #33955, #34429, #23138 ),
 .UNSPECIFIED., .F., .F. ) 
 B_SPLINE_CURVE_WITH_KNOTS ( ( 4, 4 ),
 ( 0.000000000000000000, 0.4074455897393590154 ),
 .UNSPECIFIED. ) 
 CURVE ( )  GEOMETRIC_REPRESENTATION_ITEM ( )  RATIONAL_B_SPLINE_CURVE ( ( 1.000000000000000000, 0.4567392136813477332, 0.3561768502900360955, 0.6983129098260651979 ) ) 
 REPRESENTATION_ITEM ( '' )  );
#24216=CARTESIAN_POINT ( 'NONE',  ( -23.01445215836851688, -10.50074233538543211, 66.68615203886294296 ) ) ;
#24218=CARTESIAN_POINT ( 'NONE',  ( -22.89146017634119090, -10.34570183799575105, 70.15611359559922278 ) ) ;
#24219=CARTESIAN_POINT ( 'NONE',  ( -15.40811923343077083, -21.56513327689926030, 72.06047564147742435 ) ) ;
#24220=ORIENTED_EDGE ( 'NONE', *, *, #8676, .T. ) ;
#24222=CARTESIAN_POINT ( 'NONE',  ( -22.36119861860539970, -19.84690848826603826, 72.73580505782045691 ) ) ;
#24223=EDGE_CURVE ( 'NONE', #38799, #8569, #17362, .T. ) ;
#24225=B_SPLINE_CURVE_WITH_KNOTS ( 'NONE', 3,
 ( #18452, #33460, #19198, #22658, #41124, #26845, #48496, #34205, #29804, #496 ),
 .UNSPECIFIED., .F., .F.,
 ( 4, 2, 2, 2, 4 ),
 ( 0.6272669072794416767, 0.7522669073010392893, 0.8772669073226370129, 1.002266907344234736, 1.127266907365832349 ),
 .UNSPECIFIED. ) ;
#24226=CARTESIAN_POINT ( 'NONE',  ( -24.01466881428832423, -11.33545808864497317, 66.62225715447883090 ) ) ;
#24228=EDGE_CURVE ( 'NONE', #41313, #46985, #15193, .T. ) ;
#24229=ADVANCED_FACE ( 'NONE', ( #38957 ), #20243, .T. ) ;
#24231=CARTESIAN_POINT ( 'NONE',  ( -17.22281099395510751, -7.361840332823870625, 70.60540513140719554 ) ) ;
#24232=CARTESIAN_POINT ( 'NONE',  ( -13.24261801534493088, -8.643248549050911222, 60.55454889300790455 ) ) ;
#24233=CARTESIAN_POINT ( 'NONE',  ( -24.56094871161024074, -12.67152442997557138, 69.89526119744265031 ) ) ;
#24234=PLANE ( 'NONE',  #46457 ) ;
#24235=CARTESIAN_POINT ( 'NONE',  ( -10.72615842429304323, -12.77470339663601884, 64.26836133915887217 ) ) ;
#24236=ORIENTED_EDGE ( 'NONE', *, *, #16767, .F. ) ;
#24239=CARTESIAN_POINT ( 'NONE',  ( -14.94951841260375680, -8.207726002052595504, 57.14999999999999147 ) ) ;
#24241=B_SPLINE_CURVE_WITH_KNOTS ( 'NONE', 1,
 ( #7684, #3729 ),
 .UNSPECIFIED., .F., .F.,
 ( 2, 2 ),
 ( 0.000000000000000000, 1.000000000000000000 ),
 .UNSPECIFIED. ) ;
#24242=FACE_OUTER_BOUND ( 'NONE', #9978, .T. ) ;
#24244=CARTESIAN_POINT ( 'NONE',  ( -11.93195840498443516, -10.38844327383712773, 70.98365212470247343 ) ) ;
#24246=AXIS2_PLACEMENT_3D ( 'NONE', #35442, #5423, #46784 ) ;
#24249=CARTESIAN_POINT ( 'NONE',  ( -19.69746735473979271, -8.127384799358436496, 73.87663944647505332 ) ) ;
#24250=CARTESIAN_POINT ( 'NONE',  ( -24.46244378207920533, -14.40150055328341416, 66.47732963455544564 ) ) ;
#24252=CARTESIAN_POINT ( 'NONE',  ( -22.37418574346156674, -19.75878307522992117, 69.47417994538778885 ) ) ;
#24253=CARTESIAN_POINT ( 'NONE',  ( -17.00708426123225436, -7.821638799215111071, 74.26018273346642218 ) ) ;
#24254=VERTEX_POINT ( 'NONE', #10388 ) ;
#24255=CARTESIAN_POINT ( 'NONE',  ( -13.36999615062635627, -21.05974885748268477, 61.65499767053672997 ) ) ;
#24258=CARTESIAN_POINT ( 'NONE',  ( -10.04821600842096174, -15.85811274820897410, 64.62276192103250594 ) ) ;
#24259=CARTESIAN_POINT ( 'NONE',  ( -23.96075635701088657, -17.45014263229036899, 66.09357239682297802 ) ) ;
#24260=ADVANCED_FACE ( 'NONE', ( #36935 ), #48038, .F. ) ;
#24261=( BOUNDED_CURVE ( )  B_SPLINE_CURVE ( 3, ( #36628, #29508, #32938, #40579 ),
 .UNSPECIFIED., .F., .F. ) 
 B_SPLINE_CURVE_WITH_KNOTS ( ( 4, 4 ),
 ( 0.4074455897393696180, 0.5000000000000000000 ),
 .UNSPECIFIED. ) 
 CURVE ( )  GEOMETRIC_REPRESENTATION_ITEM ( )  RATIONAL_B_SPLINE_CURVE ( ( 0.6983129098261057210, 0.7760317562607019770, 0.8765941196519980716, 0.9999999999999885647 ) ) 
 REPRESENTATION_ITEM ( '' )  );
#24263=LINE ( 'NONE', #35568, #6386 ) ;
#24266=CARTESIAN_POINT ( 'NONE',  ( -24.22593759466564123, -12.94379566627669753, 70.18731784193515466 ) ) ;
#24272=CARTESIAN_POINT ( 'NONE',  ( -12.15107435476290476, -10.20293192550022887, 67.60969940840475090 ) ) ;
#24274=CARTESIAN_POINT ( 'NONE',  ( -21.34371786970645957, -8.944908702776254827, 70.33952284808852085 ) ) ;
#24276=ORIENTED_EDGE ( 'NONE', *, *, #23462, .T. ) ;
#24277=( BOUNDED_SURFACE ( )  B_SPLINE_SURFACE ( 3, 1, ( 
 ( #43281, #5849 ),
 ( #16428, #46496 ),
 ( #46244, #35388 ),
 ( #12501, #5125 ),
 ( #39083, #20385 ),
 ( #47210, #1664 ),
 ( #46731, #16671 ) ),
 .UNSPECIFIED., .T., .F., .F. ) 
 B_SPLINE_SURFACE_WITH_KNOTS ( ( 4, 3, 4 ),
 ( 2, 2 ),
 ( 0.000000000000000000, 0.5000000000000000000, 1.000000000000000000 ),
 ( 0.000000000000000000, 1.000000000000000000 ),
 .UNSPECIFIED. ) 
 GEOMETRIC_REPRESENTATION_ITEM ( )  RATIONAL_B_SPLINE_SURFACE ( (
 ( 1.000000000000000000, 1.000000000000000000),
 ( 0.3333333333333335369, 0.3333333333333330373),
 ( 0.3333333333333335369, 0.3333333333333330373),
 ( 1.000000000000000000, 1.000000000000000000),
 ( 0.3333333333333333703, 0.3333333333333333703),
 ( 0.3333333333333333703, 0.3333333333333333703),
 ( 1.000000000000000000, 1.000000000000000000) ) ) 
 REPRESENTATION_ITEM ( '' )  SURFACE ( )  );
#24278=CARTESIAN_POINT ( 'NONE',  ( -19.97164249076357478, -21.81019033462135326, 69.11977790463622284 ) ) ;
#24279=VERTEX_POINT ( 'NONE', #25875 ) ;
#24280=EDGE_CURVE ( 'NONE', #18615, #26011, #25285, .T. ) ;
#24281=EDGE_CURVE ( 'NONE', #19220, #43790, #27438, .T. ) ;
#24283=ORIENTED_EDGE ( 'NONE', *, *, #7382, .F. ) ;
#24286=CARTESIAN_POINT ( 'NONE',  ( -23.11004506455387286, -18.89484730755139097, 65.93462627863057435 ) ) ;
#24287=CARTESIAN_POINT ( 'NONE',  ( -17.43929471692764110, -7.359095739104631662, 67.14322671830493050 ) ) ;
#24288=CARTESIAN_POINT ( 'NONE',  ( -22.18998830427770841, -20.00468049915955859, 65.71893796558269685 ) ) ;
#24289=CARTESIAN_POINT ( 'NONE',  ( -13.35680526357598907, -9.112014215067329559, 60.51238218377614686 ) ) ;
#24290=( BOUNDED_CURVE ( )  B_SPLINE_CURVE ( 3, ( #18969, #48506, #25863, #26352 ),
 .UNSPECIFIED., .F., .F. ) 
 B_SPLINE_CURVE_WITH_KNOTS ( ( 4, 4 ),
 ( 0.5000000000000000000, 0.9074455897393624015 ),
 .UNSPECIFIED. ) 
 CURVE ( )  GEOMETRIC_REPRESENTATION_ITEM ( )  RATIONAL_B_SPLINE_CURVE ( ( 0.9999999999999961142, 0.4567392136813360204, 0.3561768502900343747, 0.6983129098260869583 ) ) 
 REPRESENTATION_ITEM ( '' )  );
#24291=EDGE_LOOP ( 'NONE', ( #28974, #4489, #17404, #3103, #46340 ) ) ;
#24292=VERTEX_POINT ( 'NONE', #2966 ) ;
#24293=EDGE_CURVE ( 'NONE', #19018, #16518, #40176, .T. ) ;
#24294=ADVANCED_FACE ( 'NONE', ( #3220, #29083 ), #40406, .F. ) ;
#24296=EDGE_CURVE ( 'NONE', #20914, #35358, #43737, .T. ) ;
#24298=B_SPLINE_CURVE_WITH_KNOTS ( 'NONE', 1,
 ( #16308, #31350 ),
 .UNSPECIFIED., .F., .F.,
 ( 2, 2 ),
 ( 0.000000000000000000, 1.000000000000000000 ),
 .UNSPECIFIED. ) ;
#24299=CARTESIAN_POINT ( 'NONE',  ( -21.06634951290973845, -21.30826427787840771, 62.29966696806321380 ) ) ;
#24300=CARTESIAN_POINT ( 'NONE',  ( -11.78496890316388601, -19.04062034903473943, 71.98126064821275349 ) ) ;
#24302=ORIENTED_EDGE ( 'NONE', *, *, #24669, .T. ) ;
#24304=EDGE_CURVE ( 'NONE', #28056, #34569, #3870, .T. ) ;
#24305=DIRECTION ( 'NONE',  ( -0.6323592902076722311, -0.7746752403995150749, 4.984538757074984646E-08 ) ) ;
#24307=FACE_OUTER_BOUND ( 'NONE', #5598, .T. ) ;
#24308=ORIENTED_EDGE ( 'NONE', *, *, #11323, .T. ) ;
#24309=CARTESIAN_POINT ( 'NONE',  ( -11.74354864239398033, -18.98466756590228144, 71.68685913525695241 ) ) ;
#24310=PLANE ( 'NONE',  #29999 ) ;
#24311=CARTESIAN_POINT ( 'NONE',  ( -10.98696356482225944, -12.05889540143101080, 74.78513726815877760 ) ) ;
#24313=ORIENTED_EDGE ( 'NONE', *, *, #21918, .T. ) ;
#24314=VECTOR ( 'NONE', #21597, 1000.000000000000227 ) ;
#24315=CARTESIAN_POINT ( 'NONE',  ( -19.10440546280604934, -7.959287935654189461, 59.84604209533176089 ) ) ;
#24316=CARTESIAN_POINT ( 'NONE',  ( -17.36015951656348832, -7.359395083792595216, 67.20534920880687935 ) ) ;
#24318=ORIENTED_EDGE ( 'NONE', *, *, #38034, .T. ) ;
#24322=CARTESIAN_POINT ( 'NONE',  ( -16.39887994223181167, -21.73372354711506560, 61.75568132718285597 ) ) ;
#24323=EDGE_LOOP ( 'NONE', ( #26359, #42112, #10715, #34766, #47617 ) ) ;
#24325=CARTESIAN_POINT ( 'NONE',  ( -24.20601044598569374, -16.76383555912477874, 73.03903240339252534 ) ) ;
#24326=FACE_OUTER_BOUND ( 'NONE', #28291, .T. ) ;
#24327=ORIENTED_EDGE ( 'NONE', *, *, #5735, .T. ) ;
#24328=CARTESIAN_POINT ( 'NONE',  ( -9.996238285358009179, -14.23362990587628296, 64.56616619773187438 ) ) ;
#24329=CARTESIAN_POINT ( 'NONE',  ( -20.60942684424193772, -21.09890871138989965, 58.65947248567252359 ) ) ;
#24330=EDGE_CURVE ( 'NONE', #29080, #12494, #26126, .T. ) ;
#24331=CARTESIAN_POINT ( 'NONE',  ( -22.27163966896734593, -9.151951230621104827, 59.91509514496314637 ) ) ;
#24332=ORIENTED_EDGE ( 'NONE', *, *, #30908, .F. ) ;
#24333=CARTESIAN_POINT ( 'NONE',  ( -11.46028008028683942, -18.56947564720590194, 61.56238700194530367 ) ) ;
#24334=EDGE_CURVE ( 'NONE', #16426, #2092, #48274, .T. ) ;
#24335=ORIENTED_EDGE ( 'NONE', *, *, #39217, .F. ) ;
#24336=VERTEX_POINT ( 'NONE', #29565 ) ;
#24339=AXIS2_PLACEMENT_3D ( 'NONE', #48061, #14775, #11128 ) ;
#24340=CARTESIAN_POINT ( 'NONE',  ( -10.42558330013516255, -14.65956652655194503, 71.62782690272038622 ) ) ;
#24343=CARTESIAN_POINT ( 'NONE',  ( -10.21764033814386963, -12.91954908504599331, 67.92327745040803677 ) ) ;
#24346=CARTESIAN_POINT ( 'NONE',  ( -13.91686280105865947, -8.236299372188803147, 74.31459218752463869 ) ) ;
#24347=VERTEX_POINT ( 'NONE', #14036 ) ;
#24349=ADVANCED_FACE ( 'NONE', ( #2503 ), #44595, .T. ) ;
#24350=CARTESIAN_POINT ( 'NONE',  ( -22.94085508618206859, -9.802298960702817254, 70.19673832247809742 ) ) ;
#24352=EDGE_CURVE ( 'NONE', #29632, #188, #41264, .T. ) ;
#24356=CARTESIAN_POINT ( 'NONE',  ( -13.35550522631041837, -8.568183888810063209, 57.15463030501995689 ) ) ;
#24357=CARTESIAN_POINT ( 'NONE',  ( -11.12358174778395714, -11.75903488045733347, 71.38860871064898106 ) ) ;
#24358=ADVANCED_FACE ( 'NONE', ( #15498 ), #26612, .T. ) ;
#24360=CARTESIAN_POINT ( 'NONE',  ( -22.95183339692489710, -10.43328498706183360, 63.07745801613410919 ) ) ;
#24361=CARTESIAN_POINT ( 'NONE',  ( -20.66696756681432490, -21.06910030335248152, 58.64475164910061267 ) ) ;
#24362=FACE_OUTER_BOUND ( 'NONE', #18604, .T. ) ;
#24364=ORIENTED_EDGE ( 'NONE', *, *, #17512, .T. ) ;
#24365=B_SPLINE_CURVE_WITH_KNOTS ( 'NONE', 3,
 ( #41537, #38068, #30227, #41051, #4354, #45251, #45013, #48426, #26272, #11493 ),
 .UNSPECIFIED., .F., .F.,
 ( 4, 2, 2, 2, 4 ),
 ( 0.6272669072877629093, 0.7522669073072766333, 0.8772669073267902462, 1.002266907346303970, 1.127266907365817694 ),
 .UNSPECIFIED. ) ;
#24366=B_SPLINE_CURVE_WITH_KNOTS ( 'NONE', 3,
 ( #41209, #40253, #10458, #25465, #40475, #18057, #26436, #41445, #45401, #7744 ),
 .UNSPECIFIED., .F., .F.,
 ( 4, 2, 2, 2, 4 ),
 ( 0.000000000000000000, 0.2500000000000000000, 0.5000000000000000000, 0.7500000000000000000, 1.000000000000000000 ),
 .UNSPECIFIED. ) ;
#24368=B_SPLINE_CURVE_WITH_KNOTS ( 'NONE', 3,
 ( #30001, #48212, #21867, #11519, #7846, #25564, #26540, #10785, #11037, #25807 ),
 .UNSPECIFIED., .F., .F.,
 ( 4, 2, 2, 2, 4 ),
 ( 0.000000000000000000, 0.2500000000000000000, 0.5000000000000000000, 0.7500000000000000000, 1.000000000000000000 ),
 .UNSPECIFIED. ) ;
#24370=CARTESIAN_POINT ( 'NONE',  ( -12.78905762515450917, -9.563515353937917851, 74.33425404606212794 ) ) ;
#24373=DIRECTION ( 'NONE',  ( -0.3824554607245533866, 0.9239739285077094300, -8.917814418161383551E-09 ) ) ;
#24374=CARTESIAN_POINT ( 'NONE',  ( -21.18000274887674905, -20.77541536365158592, 69.05450184741354747 ) ) ;
#24375=ORIENTED_EDGE ( 'NONE', *, *, #25328, .F. ) ;
#24376=CARTESIAN_POINT ( 'NONE',  ( -13.30064747678972203, -9.086267117603348709, 67.67943031933630493 ) ) ;
#24379=CARTESIAN_POINT ( 'NONE',  ( -10.23981800866728342, -12.83659613830724489, 67.87799002222476474 ) ) ;
#24380=FACE_OUTER_BOUND ( 'NONE', #16378, .T. ) ;
#24381=VERTEX_POINT ( 'NONE', #8382 ) ;
#24382=CARTESIAN_POINT ( 'NONE',  ( -18.39951258112534305, -22.19516185762106275, 69.00009993223443416 ) ) ;
#24383=CARTESIAN_POINT ( 'NONE',  ( -11.42104402874289804, -10.39690533886297885, 74.59918334245951144 ) ) ;
#24384=ORIENTED_EDGE ( 'NONE', *, *, #36939, .T. ) ;
#24385=CARTESIAN_POINT ( 'NONE',  ( -10.56627859465609376, -16.21290490039525167, 71.44750383612122846 ) ) ;
#24386=VECTOR ( 'NONE', #23133, 1000.000000000000227 ) ;
#24388=CARTESIAN_POINT ( 'NONE',  ( -15.03263910315855512, -8.176888424288380364, 56.86472059657746314 ) ) ;
#24389=ORIENTED_EDGE ( 'NONE', *, *, #40147, .F. ) ;
#24392=CARTESIAN_POINT ( 'NONE',  ( -24.59934351769828709, -12.80445480200731012, 66.40908417132197883 ) ) ;
#24397=CARTESIAN_POINT ( 'NONE',  ( -22.67545590913884013, -19.51856332474398670, 72.64400582244574878 ) ) ;
#24398=DIRECTION ( 'NONE',  ( -0.4251432040024066272, -0.9051260995521939190, -1.185120001106687566E-09 ) ) ;
#24400=CARTESIAN_POINT ( 'NONE',  ( -16.20274916913749408, -7.857711080649619539, 67.28440454693885897 ) ) ;
#24401=CARTESIAN_POINT ( 'NONE',  ( -21.81751094647485445, -9.290807395701664362, 59.72171140566239700 ) ) ;
#24403=CARTESIAN_POINT ( 'NONE',  ( -23.81054795188011397, -10.97308734706811428, 73.56204507097986323 ) ) ;
#24404=CARTESIAN_POINT ( 'NONE',  ( -24.25070531508703553, -16.58426240227147375, 59.21512694191572024 ) ) ;
#24406=EDGE_LOOP ( 'NONE', ( #3189, #26008, #42257, #37534, #46681 ) ) ;
#24407=CARTESIAN_POINT ( 'NONE',  ( -16.57554779340669882, -22.21081089906203943, 65.41059674993448425 ) ) ;
#24408=CARTESIAN_POINT ( 'NONE',  ( -10.42615540542738195, -15.66473329960067140, 61.33789027493194368 ) ) ;
#24409=EDGE_CURVE ( 'NONE', #14239, #37402, #3681, .T. ) ;
#24410=AXIS2_PLACEMENT_3D ( 'NONE', #39624, #6620, #36154 ) ;
#24411=CARTESIAN_POINT ( 'NONE',  ( -23.95183236677831928, -17.48193434775220823, 69.71339772309136151 ) ) ;
#24412=CARTESIAN_POINT ( 'NONE',  ( -19.78614017500849087, -21.39864787494504839, 68.93482476778672208 ) ) ;
#24413=CARTESIAN_POINT ( 'NONE',  ( -10.79250418411942292, -11.41415947502061456, 67.74051841629483306 ) ) ;
#24414=EDGE_CURVE ( 'NONE', #40988, #19087, #9535, .T. ) ;
#24415=( BOUNDED_CURVE ( )  B_SPLINE_CURVE ( 3, ( #30735, #14940, #29750, #26538 ),
 .UNSPECIFIED., .F., .F. ) 
 B_SPLINE_CURVE_WITH_KNOTS ( ( 4, 4 ),
 ( 0.9074455897393687298, 1.000000000000000000 ),
 .UNSPECIFIED. ) 
 CURVE ( )  GEOMETRIC_REPRESENTATION_ITEM ( )  RATIONAL_B_SPLINE_CURVE ( ( 0.6983129098261068313, 0.7760317562607100816, 0.8765941196520078416, 1.000000000000000000 ) ) 
 REPRESENTATION_ITEM ( '' )  );
#24416=AXIS2_PLACEMENT_3D ( 'NONE', #10300, #44049, #33395 ) ;
#24417=ORIENTED_EDGE ( 'NONE', *, *, #33248, .F. ) ;
#24418=VERTEX_POINT ( 'NONE', #510 ) ;
#24419=ADVANCED_FACE ( 'NONE', ( #46052 ), #45589, .T. ) ;
#24421=CARTESIAN_POINT ( 'NONE',  ( -11.14114473067313682, -10.80566704772025233, 57.32407823191172014 ) ) ;
#24422=CARTESIAN_POINT ( 'NONE',  ( -23.64049396042644702, -11.59094511257166360, 63.02506373711870680 ) ) ;
#24424=B_SPLINE_CURVE_WITH_KNOTS ( 'NONE', 1,
 ( #44889, #41173 ),
 .UNSPECIFIED., .F., .F.,
 ( 2, 2 ),
 ( 0.000000000000000000, 1.000000000000000000 ),
 .UNSPECIFIED. ) ;
#24426=ADVANCED_FACE ( 'NONE', ( #27 ), #32475, .T. ) ;
#24427=ORIENTED_EDGE ( 'NONE', *, *, #29866, .T. ) ;
#24429=( BOUNDED_CURVE ( )  B_SPLINE_CURVE ( 3, ( #4472, #39172, #31068, #8670 ),
 .UNSPECIFIED., .F., .F. ) 
 B_SPLINE_CURVE_WITH_KNOTS ( ( 4, 4 ),
 ( 0.4074455897393673975, 0.5000000000000000000 ),
 .UNSPECIFIED. ) 
 CURVE ( )  GEOMETRIC_REPRESENTATION_ITEM ( )  RATIONAL_B_SPLINE_CURVE ( ( 0.6983129098260982826, 0.7760317562607005337, 0.8765941196520004031, 0.9999999999999964473 ) ) 
 REPRESENTATION_ITEM ( '' )  );
#24431=CARTESIAN_POINT ( 'NONE',  ( -10.40860991809309155, -15.50898095412354571, 57.85320721669017985 ) ) ;
#24432=ORIENTED_EDGE ( 'NONE', *, *, #19290, .F. ) ;
#24434=CARTESIAN_POINT ( 'NONE',  ( -19.56272746357835501, -21.53536514712069305, 58.68074270823246508 ) ) ;
#24435=B_SPLINE_CURVE_WITH_KNOTS ( 'NONE', 1,
 ( #36824, #3356 ),
 .UNSPECIFIED., .F., .F.,
 ( 2, 2 ),
 ( 0.000000000000000000, 1.000000000000000000 ),
 .UNSPECIFIED. ) ;
#24437=CARTESIAN_POINT ( 'NONE',  ( -21.89826263122328953, -8.852228171720549099, 66.84645388252840803 ) ) ;
#24439=CARTESIAN_POINT ( 'NONE',  ( -10.55435033023172764, -13.22452456802019327, 71.50268769994818285 ) ) ;
#24440=VERTEX_POINT ( 'NONE', #19711 ) ;
#24441=CARTESIAN_POINT ( 'NONE',  ( -24.47371109942907808, -14.90716652360855754, 59.25772288469824645 ) ) ;
#24442=CARTESIAN_POINT ( 'NONE',  ( -20.72574062298286179, -8.580111251864034116, 59.84125250080548852 ) ) ;
#24443=DIRECTION ( 'NONE',  ( -0.5652317888644006194, -0.8249321334856242194, 7.911723905267717726E-08 ) ) ;
#24444=ORIENTED_EDGE ( 'NONE', *, *, #42800, .F. ) ;
#24446=DIRECTION ( 'NONE',  ( -5.731567514496413899E-31, -1.020425574103664789E-16, -1.000000000000000000 ) ) ;
#24447=CARTESIAN_POINT ( 'NONE',  ( -22.10033346171958257, -20.08913226167895871, 58.64954131300479645 ) ) ;
#24451=CARTESIAN_POINT ( 'NONE',  ( -21.18536505927766456, -21.24010891514583221, 65.84099883884408655 ) ) ;
#24452=DIRECTION ( 'NONE',  ( -0.8201047403141394909, 0.5722134347551369737, 7.883065731424289661E-08 ) ) ;
#24453=EDGE_LOOP ( 'NONE', ( #5258, #29141, #5187, #1827 ) ) ;
#24455=FACE_OUTER_BOUND ( 'NONE', #8209, .T. ) ;
#24456=CARTESIAN_POINT ( 'NONE',  ( -24.67067787691205893, -13.07946411363355388, 62.99410723793601363 ) ) ;
#24457=CARTESIAN_POINT ( 'NONE',  ( -24.35706380436459995, -15.77560588608014136, 69.83307488757523629 ) ) ;
#24458=DIRECTION ( 'NONE',  ( -0.7300417127692488961, -0.6834025882427879894, -6.612978995310452690E-09 ) ) ;
#24459=CARTESIAN_POINT ( 'NONE',  ( -19.90432934692537614, -21.83431937171774706, 69.04987052938618319 ) ) ;
#24461=ORIENTED_EDGE ( 'NONE', *, *, #43640, .T. ) ;
#24462=CARTESIAN_POINT ( 'NONE',  ( -16.26183769579148475, -7.855670737815882987, 60.50028478907630358 ) ) ;
#24464=ORIENTED_EDGE ( 'NONE', *, *, #21330, .T. ) ;
#24465=CARTESIAN_POINT ( 'NONE',  ( -9.975558569371616002, -14.65758674969880104, 71.58428599250275681 ) ) ;
#24466=CARTESIAN_POINT ( 'NONE',  ( -10.62784674774485971, -13.13233953042942304, 67.96505635084706398 ) ) ;
#24468=CARTESIAN_POINT ( 'NONE',  ( -14.62687775177895766, -8.392386291203132842, 63.78978840643812021 ) ) ;
#24469=CARTESIAN_POINT ( 'NONE',  ( -19.10440546280604934, -7.959287935654189461, 59.84604209533176089 ) ) ;
#24470=CARTESIAN_POINT ( 'NONE',  ( -24.82869252881341637, -15.63043612719190811, 73.15303745911135991 ) ) ;
#24472=B_SPLINE_CURVE_WITH_KNOTS ( 'NONE', 1,
 ( #20278, #13346 ),
 .UNSPECIFIED., .F., .F.,
 ( 2, 2 ),
 ( 0.000000000000000000, 1.000000000000000000 ),
 .UNSPECIFIED. ) ;
#24473=B_SPLINE_CURVE_WITH_KNOTS ( 'NONE', 3,
 ( #2387, #31217, #23844, #38844, #25761, #6575, #6327, #21360, #25519, #17401 ),
 .UNSPECIFIED., .F., .F.,
 ( 4, 2, 2, 2, 4 ),
 ( 0.6272669072878317431, 0.7522669073073130486, 0.8772669073267944650, 1.002266907346275771, 1.127266907365757076 ),
 .UNSPECIFIED. ) ;
#24475=CARTESIAN_POINT ( 'NONE',  ( -24.41273135550727957, -14.40837812317847977, 66.48292728376772232 ) ) ;
#24476=CARTESIAN_POINT ( 'NONE',  ( -13.68201746596516699, -21.25120652447435532, 68.60625134287384697 ) ) ;
#24479=VECTOR ( 'NONE', #37867, 1000.000000000000114 ) ;
#24480=CARTESIAN_POINT ( 'NONE',  ( -23.48885007022674998, -11.31111499345109195, 73.59023240731526982 ) ) ;
#24481=CARTESIAN_POINT ( 'NONE',  ( -24.23813412381375088, -12.99935709875259704, 66.31718868320673721 ) ) ;
#24482=CARTESIAN_POINT ( 'NONE',  ( -13.80520660347273854, -20.80124399317547201, 65.27163466030602024 ) ) ;
#24483=DIRECTION ( 'NONE',  ( 0.02400335114476204526, -0.9997118780597843424, -1.529429985666831130E-10 ) ) ;
#24484=ORIENTED_EDGE ( 'NONE', *, *, #30640, .F. ) ;
#24485=EDGE_LOOP ( 'NONE', ( #14178, #45195 ) ) ;
#24488=AXIS2_PLACEMENT_3D ( 'NONE', #44570, #21674, #18690 ) ;
#24489=CARTESIAN_POINT ( 'NONE',  ( -21.21476609527666923, -21.22273158816933858, 65.73453942127412120 ) ) ;
#24492=CARTESIAN_POINT ( 'NONE',  ( -15.41750689856725565, -7.634439986883705842, 74.33631595678771475 ) ) ;
#24495=CARTESIAN_POINT ( 'NONE',  ( -14.13966730279324935, -8.627577120331476834, 70.92060855097744820 ) ) ;
#24498=CARTESIAN_POINT ( 'NONE',  ( -11.35824856342118316, -11.21643317443627197, 60.97885780702567615 ) ) ;
#24501=EDGE_LOOP ( 'NONE', ( #36330, #15274, #4410, #183, #34973 ) ) ;
#24502=FACE_OUTER_BOUND ( 'NONE', #27189, .T. ) ;
#24504=CARTESIAN_POINT ( 'NONE',  ( -23.66133310609451712, -18.88359296917171903, 69.40876596050124192 ) ) ;
#24505=ADVANCED_FACE ( 'NONE', ( #1956 ), #13027, .T. ) ;
#24506=ORIENTED_EDGE ( 'NONE', *, *, #9953, .F. ) ;
#24508=CARTESIAN_POINT ( 'NONE',  ( -18.54255121075907553, -21.71939966792950116, 72.28510895949058579 ) ) ;
#24509=ADVANCED_FACE ( 'NONE', ( #13259 ), #23658, .T. ) ;
#24510=ORIENTED_EDGE ( 'NONE', *, *, #43377, .T. ) ;
#24511=EDGE_CURVE ( 'NONE', #22634, #17712, #21315, .T. ) ;
#24512=DIRECTION ( 'NONE',  ( -0.9243256318339801991, 0.3816046728418207024, -8.614662759602030584E-09 ) ) ;
#24515=CARTESIAN_POINT ( 'NONE',  ( -11.03124136535102373, -17.66077402989073875, 71.56718193465405875 ) ) ;
#24516=ORIENTED_EDGE ( 'NONE', *, *, #19245, .T. ) ;
#24517=PLANE ( 'NONE',  #26018 ) ;
#24518=CARTESIAN_POINT ( 'NONE',  ( -22.34365193135296579, -19.87012687442179981, 62.39006291346853317 ) ) ;
#24519=CARTESIAN_POINT ( 'NONE',  ( -24.51735291603774058, -12.52900075589524498, 69.88587656176791540 ) ) ;
#24520=DIRECTION ( 'NONE',  ( -2.654446660633206478E-06, 3.134491597800584759E-06, -0.9999999999915644144 ) ) ;
#24524=CARTESIAN_POINT ( 'NONE',  ( -17.43166475307565122, -7.359124600834268115, 67.13544264266099049 ) ) ;
#24525=AXIS2_PLACEMENT_3D ( 'NONE', #1071, #30884, #20273 ) ;
#24526=FACE_OUTER_BOUND ( 'NONE', #19871, .T. ) ;
#24527=VERTEX_POINT ( 'NONE', #16718 ) ;
#24529=CARTESIAN_POINT ( 'NONE',  ( -20.10829901998359759, -21.75890299870832578, 72.59817030071424426 ) ) ;
#24530=CARTESIAN_POINT ( 'NONE',  ( -10.00194981992954801, -15.45342389922025639, 57.76131113159441810 ) ) ;
#24532=DIRECTION ( 'NONE',  ( 0.8967515337576289491, -0.4425343904188010491, 9.546469656967252871E-09 ) ) ;
#24533=ORIENTED_EDGE ( 'NONE', *, *, #19500, .F. ) ;
#24534=EDGE_CURVE ( 'NONE', #25477, #10558, #7177, .T. ) ;
#24536=VERTEX_POINT ( 'NONE', #46553 ) ;
#24537=CARTESIAN_POINT ( 'NONE',  ( -13.94586905867137361, -20.88575599516291703, 72.11534825290704021 ) ) ;
#24541=CARTESIAN_POINT ( 'NONE',  ( -16.98991503782990975, -22.24662993548692214, 72.35038528954983406 ) ) ;
#24542=CARTESIAN_POINT ( 'NONE',  ( -16.29760673242258306, -22.17363489859456038, 61.87072740723333197 ) ) ;
#24543=ORIENTED_EDGE ( 'NONE', *, *, #39217, .T. ) ;
#24547=DIRECTION ( 'NONE',  ( -0.6771828760946864145, 0.7358147540815750398, -3.419290845356464415E-09 ) ) ;
#24548=LINE ( 'NONE', #39543, #6482 ) ;
#24550=VERTEX_POINT ( 'NONE', #38658 ) ;
#24551=CARTESIAN_POINT ( 'NONE',  ( -14.75750412239355391, -21.76563565968240965, 61.83611636703810177 ) ) ;
#24552=CARTESIAN_POINT ( 'NONE',  ( -10.90759852523040507, -17.49952041063523822, 68.09721944423129969 ) ) ;
#24553=VECTOR ( 'NONE', #15849, 999.9999999999998863 ) ;
#24554=CARTESIAN_POINT ( 'NONE',  ( -22.09234551867295693, -20.09219114410425178, 62.53439162497838311 ) ) ;
#24555=( BOUNDED_SURFACE ( )  B_SPLINE_SURFACE ( 3, 1, ( 
 ( #22638, #14711 ),
 ( #3671, #37635 ),
 ( #18678, #11313 ),
 ( #18938, #11804 ),
 ( #15223, #33951 ),
 ( #478, #45303 ),
 ( #15463, #45546 ) ),
 .UNSPECIFIED., .T., .F., .F. ) 
 B_SPLINE_SURFACE_WITH_KNOTS ( ( 4, 3, 4 ),
 ( 2, 2 ),
 ( 0.000000000000000000, 0.5000000000000000000, 1.000000000000000000 ),
 ( 0.000000000000000000, 1.000000000000000000 ),
 .UNSPECIFIED. ) 
 GEOMETRIC_REPRESENTATION_ITEM ( )  RATIONAL_B_SPLINE_SURFACE ( (
 ( 1.000000000000000000, 1.000000000000000000),
 ( 0.3333333333333335369, 0.3333333333333330373),
 ( 0.3333333333333335369, 0.3333333333333330373),
 ( 1.000000000000000000, 1.000000000000000000),
 ( 0.3333333333333333703, 0.3333333333333333703),
 ( 0.3333333333333333703, 0.3333333333333333703),
 ( 1.000000000000000000, 1.000000000000000000) ) ) 
 REPRESENTATION_ITEM ( '' )  SURFACE ( )  );
#24556=ORIENTED_EDGE ( 'NONE', *, *, #35096, .F. ) ;
#24557=CYLINDRICAL_SURFACE ( 'NONE', #25711, 0.1500000000000029088 ) ;
#24558=CARTESIAN_POINT ( 'NONE',  ( -9.974456290884534226, -14.72748455880875795, 71.51278017970571454 ) ) ;
#24559=CARTESIAN_POINT ( 'NONE',  ( -11.52461732454066023, -18.67456722079397125, 68.63178522425482697 ) ) ;
#24560=ADVANCED_FACE ( 'NONE', ( #24380 ), #37480, .T. ) ;
#24561=ADVANCED_FACE ( 'NONE', ( #31269 ), #42555, .T. ) ;
#24562=CARTESIAN_POINT ( 'NONE',  ( -19.04042132780597996, -7.536568533962904048, 67.01576502235467103 ) ) ;
#24564=CARTESIAN_POINT ( 'NONE',  ( -19.30746897944592888, -7.600422969554355923, 60.07437648108736994 ) ) ;
#24565=CARTESIAN_POINT ( 'NONE',  ( -23.08009853854674986, -9.960157477770804846, 66.58536326842445874 ) ) ;
#24566=EDGE_LOOP ( 'NONE', ( #15964, #46268, #20699, #8149, #35924 ) ) ;
#24567=CARTESIAN_POINT ( 'NONE',  ( -24.45201643071094111, -14.25170847814747077, 69.65275273439885950 ) ) ;
#24568=( BOUNDED_SURFACE ( )  B_SPLINE_SURFACE ( 3, 1, ( 
 ( #17089, #31891 ),
 ( #42740, #16851 ),
 ( #23789, #32138 ),
 ( #31403, #24524 ),
 ( #46435, #1606 ),
 ( #9008, #20326 ),
 ( #35085, #38789 ) ),
 .UNSPECIFIED., .T., .F., .F. ) 
 B_SPLINE_SURFACE_WITH_KNOTS ( ( 4, 3, 4 ),
 ( 2, 2 ),
 ( 0.000000000000000000, 0.5000000000000000000, 1.000000000000000000 ),
 ( 0.000000000000000000, 1.000000000000000000 ),
 .UNSPECIFIED. ) 
 GEOMETRIC_REPRESENTATION_ITEM ( )  RATIONAL_B_SPLINE_SURFACE ( (
 ( 1.000000000000000000, 1.000000000000000000),
 ( 0.3333333333333335369, 0.3333333333333330373),
 ( 0.3333333333333335369, 0.3333333333333330373),
 ( 1.000000000000000000, 1.000000000000000000),
 ( 0.3333333333333333703, 0.3333333333333333703),
 ( 0.3333333333333333703, 0.3333333333333333703),
 ( 1.000000000000000000, 1.000000000000000000) ) ) 
 REPRESENTATION_ITEM ( '' )  SURFACE ( )  );
#24569=EDGE_LOOP ( 'NONE', ( #38462, #16237 ) ) ;
#24570=DIRECTION ( 'NONE',  ( -1.081321489524789733E-05, -7.211308818607114576E-06, 0.9999999999155356756 ) ) ;
#24571=ADVANCED_FACE ( 'NONE', ( #29696 ), #15144, .T. ) ;
#24572=ADVANCED_FACE ( 'NONE', ( #37807 ), #44251, .T. ) ;
#24573=CARTESIAN_POINT ( 'NONE',  ( -10.37541943412130863, -14.96049300415475436, 75.08306784598362071 ) ) ;
#24574=EDGE_LOOP ( 'NONE', ( #24484, #29473 ) ) ;
#24575=CARTESIAN_POINT ( 'NONE',  ( -14.62687775177895766, -8.392386291203132842, 63.78978840643812021 ) ) ;
#24576=CARTESIAN_POINT ( 'NONE',  ( -20.20125106709443585, -21.29320546917908885, 72.40478744281909940 ) ) ;
#24577=CARTESIAN_POINT ( 'NONE',  ( -16.93941734680483080, -7.775588144984237005, 74.24546186738449194 ) ) ;
#24578=CARTESIAN_POINT ( 'NONE',  ( -21.17181896469314140, -21.24811525286444436, 65.74600479234126738 ) ) ;
#24579=ORIENTED_EDGE ( 'NONE', *, *, #22919, .F. ) ;
#24580=CARTESIAN_POINT ( 'NONE',  ( -11.01197672498280866, -17.74032467813711378, 71.85246142747085685 ) ) ;
#24581=CARTESIAN_POINT ( 'NONE',  ( -20.82063550681992226, -21.43998110257799539, 58.90121085131534784 ) ) ;
#24582=CARTESIAN_POINT ( 'NONE',  ( -14.10256395084115866, -8.140532207465255965, 70.84462205307964666 ) ) ;
#24584=CARTESIAN_POINT ( 'NONE',  ( -10.61354641423966783, -11.78914506505660675, 74.68027500694958576 ) ) ;
#24585=( BOUNDED_CURVE ( )  B_SPLINE_CURVE ( 3, ( #19571, #24006, #42948, #45922 ),
 .UNSPECIFIED., .F., .F. ) 
 B_SPLINE_CURVE_WITH_KNOTS ( ( 4, 4 ),
 ( 4.712388980384691450, 4.921828490624017505 ),
 .UNSPECIFIED. ) 
 CURVE ( )  GEOMETRIC_REPRESENTATION_ITEM ( )  RATIONAL_B_SPLINE_CURVE ( ( 1.000000000000000000, 0.9963479302455153785, 0.9963479302455153785, 1.000000000000000000 ) ) 
 REPRESENTATION_ITEM ( '' )  );
#24586=B_SPLINE_CURVE_WITH_KNOTS ( 'NONE', 1,
 ( #9281, #38580 ),
 .UNSPECIFIED., .F., .F.,
 ( 2, 2 ),
 ( 0.000000000000000000, 1.000000000000000000 ),
 .UNSPECIFIED. ) ;
#24587=CARTESIAN_POINT ( 'NONE',  ( -12.77796340496265692, -17.75258416873320400, 53.49899999999994549 ) ) ;
#24588=EDGE_CURVE ( 'NONE', #22272, #23931, #25753, .T. ) ;
#24590=VERTEX_POINT ( 'NONE', #26009 ) ;
#24591=CARTESIAN_POINT ( 'NONE',  ( -14.74690658000796439, -21.27702444416618732, 58.16617884968206198 ) ) ;
#24592=DIRECTION ( 'NONE',  ( -0.5540494244615070674, 0.8324837747691379297, -2.496966302803655883E-17 ) ) ;
#24593=CARTESIAN_POINT ( 'NONE',  ( -19.85909425162068942, -21.37257694502213567, 72.64634926892956912 ) ) ;
#24596=DIRECTION ( 'NONE',  ( 9.588441152175118139E-09, 2.115493544230230216E-07, 0.9999999999999775735 ) ) ;
#24597=CARTESIAN_POINT ( 'NONE',  ( -23.77312829587014420, -18.70709569252041859, 72.87872954713984086 ) ) ;
#24598=DIRECTION ( 'NONE',  ( -0.9118114225829225816, -0.4106092176842893182, -5.589476761700638731E-08 ) ) ;
#24599=CARTESIAN_POINT ( 'NONE',  ( -16.72074880447151202, -22.22598103032179395, 68.88898962838827345 ) ) ;
#24600=ORIENTED_EDGE ( 'NONE', *, *, #27890, .F. ) ;
#24602=CARTESIAN_POINT ( 'NONE',  ( -11.03149232240643052, -10.98320184173030256, 60.93531726291125494 ) ) ;
#24604=CARTESIAN_POINT ( 'NONE',  ( -19.77283897654775657, -21.87935945976245122, 65.50840285157048015 ) ) ;
#24606=CARTESIAN_POINT ( 'NONE',  ( -20.72450927900464634, -21.03929139025763106, 58.93003081252663833 ) ) ;
#24608=ORIENTED_EDGE ( 'NONE', *, *, #16957, .F. ) ;
#24609=CARTESIAN_POINT ( 'NONE',  ( -15.09857480863590062, -8.145354156905789011, 60.46428990550709415 ) ) ;
#24610=CARTESIAN_POINT ( 'NONE',  ( -11.07163856976715977, -18.70144880307400470, 61.47049154680724570 ) ) ;
#24611=ORIENTED_EDGE ( 'NONE', *, *, #24191, .T. ) ;
#24612=CARTESIAN_POINT ( 'NONE',  ( -11.17855950479832927, -18.87086615690261482, 64.86211796126700335 ) ) ;
#24614=CARTESIAN_POINT ( 'NONE',  ( -19.98190323201305318, -8.235588387909094976, 70.25100363142931315 ) ) ;
#24615=EDGE_CURVE ( 'NONE', #34640, #8636, #39077, .T. ) ;
#24616=CARTESIAN_POINT ( 'NONE',  ( -10.56409641782382813, -13.17052685802803680, 75.09306420679733662 ) ) ;
#24618=CARTESIAN_POINT ( 'NONE',  ( -14.82114783504062139, -7.828710491958731588, 56.94976379657543220 ) ) ;
#24619=CARTESIAN_POINT ( 'NONE',  ( -24.79781836340079337, -15.87314503134675014, 69.64812095075065201 ) ) ;
#24620=VERTEX_POINT ( 'NONE', #168 ) ;
#24621=CARTESIAN_POINT ( 'NONE',  ( -20.85666804334717739, -20.91165978247425272, 65.77381081790800010 ) ) ;
#24622=VERTEX_POINT ( 'NONE', #41026 ) ;
#24623=FACE_OUTER_BOUND ( 'NONE', #13557, .T. ) ;
#24625=EDGE_CURVE ( 'NONE', #2258, #34107, #5439, .T. ) ;
#24626=CARTESIAN_POINT ( 'NONE',  ( -10.01440787728688520, -14.03439562150409969, 61.03325889150411143 ) ) ;
#24627=ORIENTED_EDGE ( 'NONE', *, *, #7851, .F. ) ;
#24628=EDGE_CURVE ( 'NONE', #18657, #4575, #4103, .T. ) ;
#24630=B_SPLINE_CURVE_WITH_KNOTS ( 'NONE', 3,
 ( #17118, #9771, #24785, #39787, #10717, #7035, #21797, #48146, #25734, #6784 ),
 .UNSPECIFIED., .F., .F.,
 ( 4, 2, 2, 2, 4 ),
 ( 0.000000000000000000, 0.2500000000000000000, 0.5000000000000000000, 0.7500000000000000000, 1.000000000000000000 ),
 .UNSPECIFIED. ) ;
#24631=ORIENTED_EDGE ( 'NONE', *, *, #42888, .F. ) ;
#24632=CARTESIAN_POINT ( 'NONE',  ( -14.96339028783852676, -21.42433367428847291, 68.72025781230657060 ) ) ;
#24634=CARTESIAN_POINT ( 'NONE',  ( -17.63906322355374101, -7.762336171902432191, 63.55616794089306865 ) ) ;
#24637=CARTESIAN_POINT ( 'NONE',  ( -16.27008412796014625, -7.904986034540439022, 60.20028479263386600 ) ) ;
#24642=VERTEX_POINT ( 'NONE', #26247 ) ;
#24644=B_SPLINE_CURVE_WITH_KNOTS ( 'NONE', 3,
 ( #27882, #35510, #46614, #2264, #12857, #28847, #39208, #13088, #43153, #39932 ),
 .UNSPECIFIED., .F., .F.,
 ( 4, 2, 2, 2, 4 ),
 ( 0.000000000000000000, 0.2500000000000000000, 0.5000000000000000000, 0.7500000000000000000, 1.000000000000000000 ),
 .UNSPECIFIED. ) ;
#24646=CARTESIAN_POINT ( 'NONE',  ( -20.89619716791787596, -20.95408004043368067, 69.19883325555726117 ) ) ;
#24647=ORIENTED_EDGE ( 'NONE', *, *, #17446, .T. ) ;
#24648=CARTESIAN_POINT ( 'NONE',  ( -24.34870638818816957, -15.83419385995577677, 66.28998161055176297 ) ) ;
#24649=CARTESIAN_POINT ( 'NONE',  ( -19.28643955730387916, -21.55824949740921426, 62.22333559350940391 ) ) ;
#24651=CARTESIAN_POINT ( 'NONE',  ( -23.78676187654788521, -10.93361199230012559, 73.54688693628270357 ) ) ;
#24655=CARTESIAN_POINT ( 'NONE',  ( -16.57554779340669882, -22.21081089906203943, 65.41059674993448425 ) ) ;
#24656=CARTESIAN_POINT ( 'NONE',  ( -13.05361004613213893, -8.775835911160044134, 64.00972289988426667 ) ) ;
#24657=CARTESIAN_POINT ( 'NONE',  ( -22.85875596884486072, -9.713182710008496201, 73.62127706024359952 ) ) ;
#24660=VERTEX_POINT ( 'NONE', #41261 ) ;
#24661=ORIENTED_EDGE ( 'NONE', *, *, #38371, .F. ) ;
#24662=CARTESIAN_POINT ( 'NONE',  ( -17.70854774853812330, -7.363889232077062807, 63.73712292196469065 ) ) ;
#24666=ORIENTED_EDGE ( 'NONE', *, *, #9405, .T. ) ;
#24667=CARTESIAN_POINT ( 'NONE',  ( -24.25719835994319951, -13.28920697710681864, 59.36267871205171076 ) ) ;
#24669=EDGE_CURVE ( 'NONE', #37207, #21625, #8905, .T. ) ;
#24672=CARTESIAN_POINT ( 'NONE',  ( -12.36794899618824317, -19.72224014812425708, 61.69678633597966666 ) ) ;
#24673=CARTESIAN_POINT ( 'NONE',  ( -17.78489980232956569, -21.80118272162682658, 61.94706151667214300 ) ) ;
#24674=ORIENTED_EDGE ( 'NONE', *, *, #47032, .F. ) ;
#24675=CARTESIAN_POINT ( 'NONE',  ( -21.90433870182133802, -8.856837556793539790, 66.85424130413866806 ) ) ;
#24679=CARTESIAN_POINT ( 'NONE',  ( -11.93063564843302160, -19.84155427294366092, 58.12693572425718003 ) ) ;
#24681=CARTESIAN_POINT ( 'NONE',  ( -19.30128557755455176, -21.60500301973953086, 58.81035253397666196 ) ) ;
#24682=ORIENTED_EDGE ( 'NONE', *, *, #38795, .F. ) ;
#24685=EDGE_CURVE ( 'NONE', #12034, #35350, #18956, .T. ) ;
#24686=CARTESIAN_POINT ( 'NONE',  ( -12.55411140858086760, -19.90724249994213935, 65.15202838036978505 ) ) ;
#24687=EDGE_CURVE ( 'NONE', #36936, #7665, #38910, .T. ) ;
#24688=( BOUNDED_SURFACE ( )  B_SPLINE_SURFACE ( 3, 1, ( 
 ( #7141, #22158 ),
 ( #18434, #13998 ),
 ( #10352, #25365 ),
 ( #29787, #6647 ),
 ( #14246, #33443 ),
 ( #29295, #44332 ),
 ( #40603, #6888 ) ),
 .UNSPECIFIED., .T., .F., .F. ) 
 B_SPLINE_SURFACE_WITH_KNOTS ( ( 4, 3, 4 ),
 ( 2, 2 ),
 ( 0.000000000000000000, 0.5000000000000000000, 1.000000000000000000 ),
 ( 0.000000000000000000, 1.000000000000000000 ),
 .UNSPECIFIED. ) 
 GEOMETRIC_REPRESENTATION_ITEM ( )  RATIONAL_B_SPLINE_SURFACE ( (
 ( 1.000000000000000000, 1.000000000000000000),
 ( 0.3333333333333335369, 0.3333333333333330373),
 ( 0.3333333333333335369, 0.3333333333333330373),
 ( 1.000000000000000000, 1.000000000000000000),
 ( 0.3333333333333333703, 0.3333333333333333703),
 ( 0.3333333333333333703, 0.3333333333333333703),
 ( 1.000000000000000000, 1.000000000000000000) ) ) 
 REPRESENTATION_ITEM ( '' )  SURFACE ( )  );
#24689=CARTESIAN_POINT ( 'NONE',  ( -11.41497376296057098, -19.21309731666858411, 71.80190493362104576 ) ) ;
#24691=EDGE_LOOP ( 'NONE', ( #1182, #18310, #16919, #7231, #5172 ) ) ;
#24692=CARTESIAN_POINT ( 'NONE',  ( -14.84764829735760827, -8.246537290690364230, 60.33468334944129197 ) ) ;
#24693=CARTESIAN_POINT ( 'NONE',  ( -11.82258790637234291, -19.00740242323033513, 71.98685835211126971 ) ) ;
#24694=CARTESIAN_POINT ( 'NONE',  ( -12.23220206747517835, -19.57856285391799034, 58.22682373937799127 ) ) ;
#24695=CARTESIAN_POINT ( 'NONE',  ( -13.19632391105088409, -20.94361350779438879, 58.18503525494669049 ) ) ;
#24698=CARTESIAN_POINT ( 'NONE',  ( -24.29232294273250758, -16.16103065725259214, 62.59328677063434299 ) ) ;
#24701=CARTESIAN_POINT ( 'NONE',  ( -24.81704557732260952, -15.73545128243976521, 73.18959105933400622 ) ) ;
#24702=EDGE_LOOP ( 'NONE', ( #39656, #14406, #12427, #25897, #22012 ) ) ;
#24703=LINE ( 'NONE', #13101, #28453 ) ;
#24704=CARTESIAN_POINT ( 'NONE',  ( -19.96994574550859980, -21.32983827578761193, 72.40478737306770540 ) ) ;
#24706=CARTESIAN_POINT ( 'NONE',  ( -23.08487763607990928, -19.01185175973044039, 62.36879011380454330 ) ) ;
#24707=CARTESIAN_POINT ( 'NONE',  ( -16.99752982347189345, -22.24711114454501626, 72.34260117165817405 ) ) ;
#24708=EDGE_CURVE ( 'NONE', #2695, #47031, #3059, .T. ) ;
#24709=( BOUNDED_SURFACE ( )  B_SPLINE_SURFACE ( 3, 1, ( 
 ( #14915, #11256 ),
 ( #29973, #22836 ),
 ( #45483, #189 ),
 ( #34131, #3875 ),
 ( #11742, #26270 ),
 ( #37572, #30225 ),
 ( #43912, #12483 ) ),
 .UNSPECIFIED., .T., .F., .F. ) 
 B_SPLINE_SURFACE_WITH_KNOTS ( ( 4, 3, 4 ),
 ( 2, 2 ),
 ( 0.000000000000000000, 0.5000000000000000000, 1.000000000000000000 ),
 ( 0.000000000000000000, 1.000000000000000000 ),
 .UNSPECIFIED. ) 
 GEOMETRIC_REPRESENTATION_ITEM ( )  RATIONAL_B_SPLINE_SURFACE ( (
 ( 1.000000000000000000, 1.000000000000000000),
 ( 0.3333333333333335369, 0.3333333333333330373),
 ( 0.3333333333333335369, 0.3333333333333330373),
 ( 1.000000000000000000, 1.000000000000000000),
 ( 0.3333333333333333703, 0.3333333333333333703),
 ( 0.3333333333333333703, 0.3333333333333333703),
 ( 1.000000000000000000, 1.000000000000000000) ) ) 
 REPRESENTATION_ITEM ( '' )  SURFACE ( )  );
#24710=ORIENTED_EDGE ( 'NONE', *, *, #4418, .T. ) ;
#24711=CARTESIAN_POINT ( 'NONE',  ( -24.41053240502948896, -14.37272825023783618, 66.19795200961559090 ) ) ;
#24712=CARTESIAN_POINT ( 'NONE',  ( -17.08574859075978480, -7.366143556642608559, 74.14673579026420214 ) ) ;
#24714=CARTESIAN_POINT ( 'NONE',  ( -23.75797280549784318, -17.78947120508452429, 59.30378417803890301 ) ) ;
#24715=ORIENTED_EDGE ( 'NONE', *, *, #18102, .F. ) ;
#24718=DIRECTION ( 'NONE',  ( 0.9729319276368276759, 0.2310918955413240050, -6.827553174550346358E-08 ) ) ;
#24719=CARTESIAN_POINT ( 'NONE',  ( -23.46018740455247809, -11.26354644359006585, 73.64576786816009246 ) ) ;
#24720=CARTESIAN_POINT ( 'NONE',  ( -24.17041903051225304, -17.96986306003213940, 59.10354794152625857 ) ) ;
#24721=CARTESIAN_POINT ( 'NONE',  ( -17.42409385541300892, -14.80920654474439679, 56.49999999999994316 ) ) ;
#24723=( BOUNDED_SURFACE ( )  B_SPLINE_SURFACE ( 3, 1, ( 
 ( #14529, #36390 ),
 ( #24848, #2900 ),
 ( #39857, #20908 ),
 ( #32932, #36622 ),
 ( #20673, #2670 ),
 ( #5889, #13018 ),
 ( #2188, #28044 ) ),
 .UNSPECIFIED., .T., .F., .F. ) 
 B_SPLINE_SURFACE_WITH_KNOTS ( ( 4, 3, 4 ),
 ( 2, 2 ),
 ( 0.000000000000000000, 0.5000000000000000000, 1.000000000000000000 ),
 ( 0.000000000000000000, 1.000000000000000000 ),
 .UNSPECIFIED. ) 
 GEOMETRIC_REPRESENTATION_ITEM ( )  RATIONAL_B_SPLINE_SURFACE ( (
 ( 1.000000000000000000, 1.000000000000000000),
 ( 0.3333333333333335369, 0.3333333333333330373),
 ( 0.3333333333333335369, 0.3333333333333330373),
 ( 1.000000000000000000, 1.000000000000000000),
 ( 0.3333333333333333703, 0.3333333333333333703),
 ( 0.3333333333333333703, 0.3333333333333333703),
 ( 1.000000000000000000, 1.000000000000000000) ) ) 
 REPRESENTATION_ITEM ( '' )  SURFACE ( )  );
#24728=B_SPLINE_CURVE_WITH_KNOTS ( 'NONE', 3,
 ( #22853, #34145, #27014, #42530, #34635, #23573, #19876, #42037, #45975, #1143 ),
 .UNSPECIFIED., .F., .F.,
 ( 4, 2, 2, 2, 4 ),
 ( 0.000000000000000000, 0.2500000000000000000, 0.5000000000000000000, 0.7500000000000000000, 1.000000000000000000 ),
 .UNSPECIFIED. ) ;
#24729=CARTESIAN_POINT ( 'NONE',  ( -15.81671074304997582, -7.936704070960259649, 74.22418700304095296 ) ) ;
#24730=ADVANCED_FACE ( 'NONE', ( #45941 ), #15381, .T. ) ;
#24732=DIRECTION ( 'NONE',  ( 0.9942595023566569434, -0.1069955231469581769, 3.800058679842193584E-08 ) ) ;
#24733=ORIENTED_EDGE ( 'NONE', *, *, #35597, .F. ) ;
#24737=DIRECTION ( 'NONE',  ( -0.8651630202045380580, 0.5014907262059380422, 5.433021001366389699E-08 ) ) ;
#24740=ORIENTED_EDGE ( 'NONE', *, *, #48514, .T. ) ;
#24741=DIRECTION ( 'NONE',  ( 0.4433615477241706904, -0.8963428685495450354, 2.661652803430218851E-08 ) ) ;
#24742=CARTESIAN_POINT ( 'NONE',  ( -14.72778380697628187, -21.32322314059345558, 58.16617885012796307 ) ) ;
#24743=VERTEX_POINT ( 'NONE', #42494 ) ;
#24747=CARTESIAN_POINT ( 'NONE',  ( -24.14854887165027009, -16.95319183457820955, 69.56907079017828721 ) ) ;
#24748=CARTESIAN_POINT ( 'NONE',  ( -16.63457431780823725, -21.76466301827511174, 65.22564349372431991 ) ) ;
#24751=DIRECTION ( 'NONE',  ( -0.04108628546905851442, -0.9991556020692448081, 4.908153721456304258E-18 ) ) ;
#24753=FACE_OUTER_BOUND ( 'NONE', #20117, .T. ) ;
#24754=EDGE_CURVE ( 'NONE', #30663, #32429, #11885, .T. ) ;
#24756=CARTESIAN_POINT ( 'NONE',  ( -22.33041777183100507, -20.41561037748852669, 62.34943743628787161 ) ) ;
#24757=CARTESIAN_POINT ( 'NONE',  ( -16.32575768948312600, -7.844986739114469643, 60.21500614002425777 ) ) ;
#24759=ORIENTED_EDGE ( 'NONE', *, *, #16746, .F. ) ;
#24762=CARTESIAN_POINT ( 'NONE',  ( -12.77796340496265870, -17.75258416873320400, 53.49999999999995026 ) ) ;
#24763=CARTESIAN_POINT ( 'NONE',  ( -10.00054666056749575, -15.43791465228438931, 57.74605562754308608 ) ) ;
#24765=CARTESIAN_POINT ( 'NONE',  ( -21.08382089131013259, -22.19632712819893428, 53.49999999999995026 ) ) ;
#24766=ORIENTED_EDGE ( 'NONE', *, *, #31245, .T. ) ;
#24769=CARTESIAN_POINT ( 'NONE',  ( -13.94586845990913737, -20.88575566452655607, 72.03680843657026855 ) ) ;
#24770=CARTESIAN_POINT ( 'NONE',  ( -12.89674140296688520, -8.892592839661450199, 67.57281105838596602 ) ) ;
#24772=ADVANCED_FACE ( 'NONE', ( #42247 ), #27459, .T. ) ;
#24773=CARTESIAN_POINT ( 'NONE',  ( -24.71495620756359557, -13.27698325404237956, 59.48551063991843790 ) ) ;
#24776=ORIENTED_EDGE ( 'NONE', *, *, #27122, .T. ) ;
#24777=ORIENTED_EDGE ( 'NONE', *, *, #20267, .F. ) ;
#24778=VECTOR ( 'NONE', #15697, 1000.000000000000000 ) ;
#24781=LINE ( 'NONE', #1874, #35432 ) ;
#24784=ORIENTED_EDGE ( 'NONE', *, *, #30180, .T. ) ;
#24785=CARTESIAN_POINT ( 'NONE',  ( -24.36735374303742319, -15.69913859885677176, 69.54809873558210143 ) ) ;
#24786=CARTESIAN_POINT ( 'NONE',  ( -24.87394656424350359, -14.85804368301403500, 59.34325982243593245 ) ) ;
#24787=( BOUNDED_SURFACE ( )  B_SPLINE_SURFACE ( 3, 1, ( 
 ( #23599, #24080 ),
 ( #42561, #1412 ),
 ( #704, #34666 ),
 ( #42063, #942 ),
 ( #46730, #15941 ),
 ( #12500, #8336 ),
 ( #31216, #35141 ) ),
 .UNSPECIFIED., .T., .F., .F. ) 
 B_SPLINE_SURFACE_WITH_KNOTS ( ( 4, 3, 4 ),
 ( 2, 2 ),
 ( 0.000000000000000000, 0.5000000000000000000, 1.000000000000000000 ),
 ( 0.000000000000000000, 1.000000000000000000 ),
 .UNSPECIFIED. ) 
 GEOMETRIC_REPRESENTATION_ITEM ( )  RATIONAL_B_SPLINE_SURFACE ( (
 ( 1.000000000000000000, 1.000000000000000000),
 ( 0.3333333333333335369, 0.3333333333333330373),
 ( 0.3333333333333335369, 0.3333333333333330373),
 ( 1.000000000000000000, 1.000000000000000000),
 ( 0.3333333333333333703, 0.3333333333333333703),
 ( 0.3333333333333333703, 0.3333333333333333703),
 ( 1.000000000000000000, 1.000000000000000000) ) ) 
 REPRESENTATION_ITEM ( '' )  SURFACE ( )  );
#24788=ORIENTED_EDGE ( 'NONE', *, *, #27618, .T. ) ;
#24789=B_SPLINE_CURVE_WITH_KNOTS ( 'NONE', 3,
 ( #26263, #12639, #45897, #41278, #23491, #16310, #45004, #48666, #37320, #14649 ),
 .UNSPECIFIED., .F., .F.,
 ( 4, 2, 2, 2, 4 ),
 ( 0.6272669072877501417, 0.7522669073072613122, 0.8772669073267724826, 1.002266907346283542, 1.127266907365794824 ),
 .UNSPECIFIED. ) ;
#24790=CARTESIAN_POINT ( 'NONE',  ( -22.09234551867295338, -20.09219114410425178, 62.53439162497838311 ) ) ;
#24791=B_SPLINE_CURVE_WITH_KNOTS ( 'NONE', 3,
 ( #46615, #5241, #27883, #1537, #9905, #42911, #36228, #16546, #31586, #6206 ),
 .UNSPECIFIED., .F., .F.,
 ( 4, 2, 2, 2, 4 ),
 ( 0.000000000000000000, 0.2500000000000000000, 0.5000000000000000000, 0.7500000000000000000, 1.000000000000000000 ),
 .UNSPECIFIED. ) ;
#24793=ORIENTED_EDGE ( 'NONE', *, *, #23533, .T. ) ;
#24794=DIRECTION ( 'NONE',  ( 1.504942871710700414E-06, -3.061075848816703091E-06, 0.9999999999941824314 ) ) ;
#24795=CARTESIAN_POINT ( 'NONE',  ( -11.37092239977862640, -11.18788622403751276, 64.44882256896082140 ) ) ;
#24797=ORIENTED_EDGE ( 'NONE', *, *, #2101, .T. ) ;
#24798=CARTESIAN_POINT ( 'NONE',  ( -24.09792882696954663, -17.08130396874204138, 73.03336032035906555 ) ) ;
#24800=CARTESIAN_POINT ( 'NONE',  ( -14.99706723701585354, -21.85287888328288375, 65.29092001793476641 ) ) ;
#24801=ORIENTED_EDGE ( 'NONE', *, *, #36383, .F. ) ;
#24802=EDGE_CURVE ( 'NONE', #25977, #34579, #1936, .T. ) ;
#24803=FACE_OUTER_BOUND ( 'NONE', #9507, .T. ) ;
#24804=CARTESIAN_POINT ( 'NONE',  ( -21.85024312005885250, -20.23279700434262907, 59.04826358179722945 ) ) ;
#24805=VECTOR ( 'NONE', #2926, 1000.000000000000114 ) ;
#24806=CARTESIAN_POINT ( 'NONE',  ( -13.18362886651731358, -8.683667069837246899, 60.62445550483372614 ) ) ;
#24807=CARTESIAN_POINT ( 'NONE',  ( -14.30855566557790404, -8.484641631233271752, 70.74429704309763167 ) ) ;
#24808=VERTEX_POINT ( 'NONE', #15884 ) ;
#24809=DIRECTION ( 'NONE',  ( -0.9998756790481364565, -0.01576789294826319576, -3.907472230461691850E-09 ) ) ;
#24810=CARTESIAN_POINT ( 'NONE',  ( -23.97043363090852353, -12.17094895590152426, 59.62668449103946955 ) ) ;
#24812=ORIENTED_EDGE ( 'NONE', *, *, #6068, .F. ) ;
#24813=CARTESIAN_POINT ( 'NONE',  ( -10.17894133981683247, -13.07414026325376177, 71.30854345628114288 ) ) ;
#24814=CARTESIAN_POINT ( 'NONE',  ( -24.31944129331298399, -13.32629719641017729, 63.24753052856355140 ) ) ;
#24815=VERTEX_POINT ( 'NONE', #1602 ) ;
#24817=CARTESIAN_POINT ( 'NONE',  ( -23.71751471349159601, -11.63122711669449316, 63.23746208799618529 ) ) ;
#24819=CARTESIAN_POINT ( 'NONE',  ( -13.18473975798692877, -20.93551490194142062, 58.23145353898504339 ) ) ;
#24821=CARTESIAN_POINT ( 'NONE',  ( -21.88700264784966976, -8.843686206210612966, 66.80003455143545921 ) ) ;
#24822=CARTESIAN_POINT ( 'NONE',  ( -10.40860991809309155, -15.50898095412354571, 57.85320721669017985 ) ) ;
#24823=CARTESIAN_POINT ( 'NONE',  ( -10.78978129946085929, -12.42417050351721919, 57.47857332104950956 ) ) ;
#24824=CARTESIAN_POINT ( 'NONE',  ( -12.20924706590383302, -20.12979026787678549, 65.06013176247181207 ) ) ;
#24825=B_SPLINE_CURVE_WITH_KNOTS ( 'NONE', 3,
 ( #32761, #17499, #14026, #24673, #24906, #39676, #29076, #5948, #20967, #17256 ),
 .UNSPECIFIED., .F., .F.,
 ( 4, 2, 2, 2, 4 ),
 ( 0.000000000000000000, 0.2500000000000000000, 0.5000000000000000000, 0.7500000000000000000, 1.000000000000000000 ),
 .UNSPECIFIED. ) ;
#24827=CARTESIAN_POINT ( 'NONE',  ( -16.73751461255839601, -22.22750928065944009, 68.89571854458313283 ) ) ;
#24829=VERTEX_POINT ( 'NONE', #2082 ) ;
#24831=ADVANCED_FACE ( 'NONE', ( #39516 ), #47152, .T. ) ;
#24833=CARTESIAN_POINT ( 'NONE',  ( -21.96907604098356970, -20.13311438280304344, 59.04977527294225581 ) ) ;
#24834=CARTESIAN_POINT ( 'NONE',  ( -15.88656107989463706, -7.980151544674868980, 67.14007279409138107 ) ) ;
#24835=CARTESIAN_POINT ( 'NONE',  ( -12.01648241349452917, -10.28590705807702932, 67.49896869922172016 ) ) ;
#24836=LINE ( 'NONE', #39846, #39403 ) ;
#24840=VERTEX_POINT ( 'NONE', #13393 ) ;
#24841=CARTESIAN_POINT ( 'NONE',  ( -15.05456328141641542, -21.39602539821822091, 61.86273865514400683 ) ) ;
#24842=CARTESIAN_POINT ( 'NONE',  ( -10.21583571369164467, -12.92629908267978323, 67.86019570968910841 ) ) ;
#24843=CARTESIAN_POINT ( 'NONE',  ( -17.65810221059773610, -7.762793303104816189, 63.56529088875731759 ) ) ;
#24844=CARTESIAN_POINT ( 'NONE',  ( -18.20795910203089818, -22.21802180157784079, 65.48385643348356666 ) ) ;
#24846=( BOUNDED_CURVE ( )  B_SPLINE_CURVE ( 3, ( #15042, #7450, #30591, #41903 ),
 .UNSPECIFIED., .F., .F. ) 
 B_SPLINE_CURVE_WITH_KNOTS ( ( 4, 4 ),
 ( 0.4074455897393572390, 0.5000000000000000000 ),
 .UNSPECIFIED. ) 
 CURVE ( )  GEOMETRIC_REPRESENTATION_ITEM ( )  RATIONAL_B_SPLINE_CURVE ( ( 0.6983129098260801859, 0.7760317562606920960, 0.8765941196520000700, 1.000000000000007772 ) ) 
 REPRESENTATION_ITEM ( '' )  );
#24848=CARTESIAN_POINT ( 'NONE',  ( -17.45593231491017505, -7.751306502474292870, 60.23627933525208533 ) ) ;
#24849=ADVANCED_FACE ( 'NONE', ( #6517 ), #417, .T. ) ;
#24850=CARTESIAN_POINT ( 'NONE',  ( -15.62778143507988560, -7.578882312233643503, 70.78802623904546465 ) ) ;
#24851=CARTESIAN_POINT ( 'NONE',  ( -11.11547657867172134, -10.84637923393623993, 57.30879572875446826 ) ) ;
#24852=CARTESIAN_POINT ( 'NONE',  ( -10.33531725737393181, -17.10115422170377641, 57.87255955594724810 ) ) ;
#24853=VERTEX_POINT ( 'NONE', #21298 ) ;
#24854=CARTESIAN_POINT ( 'NONE',  ( -19.30272045617997634, -8.014115550771091279, 59.96092997145632353 ) ) ;
#24855=VERTEX_POINT ( 'NONE', #35805 ) ;
#24856=CARTESIAN_POINT ( 'NONE',  ( -21.57995947450667984, -9.113990939708573435, 70.14604673427196246 ) ) ;
#24859=CARTESIAN_POINT ( 'NONE',  ( -20.37299750454370439, -8.405577324698720432, 66.78104082189589974 ) ) ;
#24861=ADVANCED_FACE ( 'NONE', ( #21045 ), #36292, .T. ) ;
#24863=CARTESIAN_POINT ( 'NONE',  ( -18.79452142415569682, -7.944218599080984156, 70.38684728956484093 ) ) ;
#24864=CARTESIAN_POINT ( 'NONE',  ( -10.65167304149821881, -11.70447990960673046, 74.69806764605195326 ) ) ;
#24866=EDGE_LOOP ( 'NONE', ( #16374, #10049 ) ) ;
#24867=DIRECTION ( 'NONE',  ( -0.9848822020395751053, 0.1732254256905498280, 7.367703375004543066E-08 ) ) ;
#24870=CARTESIAN_POINT ( 'NONE',  ( -24.09883172553966091, -12.52826034843049996, 69.77242826584058832 ) ) ;
#24872=ORIENTED_EDGE ( 'NONE', *, *, #18291, .T. ) ;
#24873=EDGE_LOOP ( 'NONE', ( #28814, #40284, #20222, #15062, #10505 ) ) ;
#24874=CARTESIAN_POINT ( 'NONE',  ( -21.36420383812641077, -21.13211724076752773, 69.31096130815059553 ) ) ;
#24875=EDGE_LOOP ( 'NONE', ( #23076, #34955, #3162, #43478, #23457 ) ) ;
#24879=B_SPLINE_CURVE_WITH_KNOTS ( 'NONE', 1,
 ( #44087, #29522 ),
 .UNSPECIFIED., .F., .F.,
 ( 2, 2 ),
 ( 0.000000000000000000, 1.000000000000000000 ),
 .UNSPECIFIED. ) ;
#24881=CARTESIAN_POINT ( 'NONE',  ( -20.57278697373333998, -8.057206101692887756, 66.89608655064280640 ) ) ;
#24883=CARTESIAN_POINT ( 'NONE',  ( -20.66848101912799862, -8.549761622307151754, 60.12653141481577990 ) ) ;
#24884=EDGE_CURVE ( 'NONE', #8174, #14528, #38281, .T. ) ;
#24888=CARTESIAN_POINT ( 'NONE',  ( -13.57572078670752447, -20.65643022133334128, 61.81646323932617548 ) ) ;
#24889=ORIENTED_EDGE ( 'NONE', *, *, #21891, .T. ) ;
#24890=EDGE_CURVE ( 'NONE', #19021, #13315, #15476, .T. ) ;
#24892=EDGE_LOOP ( 'NONE', ( #48145, #14698, #12662, #5227, #47362 ) ) ;
#24893=FACE_OUTER_BOUND ( 'NONE', #30708, .T. ) ;
#24896=CARTESIAN_POINT ( 'NONE',  ( -23.92719435707370224, -11.17417392741853988, 70.00715344888816105 ) ) ;
#24898=ORIENTED_EDGE ( 'NONE', *, *, #12885, .F. ) ;
#24901=VECTOR ( 'NONE', #8136, 1000.000000000000114 ) ;
#24902=DIRECTION ( 'NONE',  ( -0.9974380310868018462, -0.07153582418399356824, 3.008056591778322057E-08 ) ) ;
#24904=EDGE_LOOP ( 'NONE', ( #41630, #46929, #25256, #33667, #20812 ) ) ;
#24905=FACE_OUTER_BOUND ( 'NONE', #46889, .T. ) ;
#24906=CARTESIAN_POINT ( 'NONE',  ( -17.76877427553128896, -21.80232428101829711, 61.98608964106817609 ) ) ;
#24907=CARTESIAN_POINT ( 'NONE',  ( -23.38560432932743538, -19.27844084936127800, 58.99755287451023378 ) ) ;
#24908=ORIENTED_EDGE ( 'NONE', *, *, #10177, .F. ) ;
#24909=DIRECTION ( 'NONE',  ( -0.3824554607245533866, 0.9239739285077093189, -8.917814418161381897E-09 ) ) ;
#24910=ORIENTED_EDGE ( 'NONE', *, *, #25442, .T. ) ;
#24915=CARTESIAN_POINT ( 'NONE',  ( -19.36683724782897897, -21.58655468785150688, 62.00975759738177118 ) ) ;
#24918=DIRECTION ( 'NONE',  ( 0.6827297667453423591, 0.7306709694519485376, 5.176517822219622992E-09 ) ) ;
#24920=ORIENTED_EDGE ( 'NONE', *, *, #22163, .F. ) ;
#24921=CARTESIAN_POINT ( 'NONE',  ( -22.49805064719525305, -9.986866608920609067, 73.48161091687566682 ) ) ;
#24922=CARTESIAN_POINT ( 'NONE',  ( -17.42409385541300892, -14.80920654474439324, 75.49999999999994316 ) ) ;
#24923=FACE_OUTER_BOUND ( 'NONE', #10006, .T. ) ;
#24927=ORIENTED_EDGE ( 'NONE', *, *, #16936, .T. ) ;
#24929=CARTESIAN_POINT ( 'NONE',  ( -14.03870967672415304, -8.172720116890397790, 70.91453050697840865 ) ) ;
#24930=DIRECTION ( 'NONE',  ( 0.1847813031241905823, -0.9827796650397888634, 7.910442904995644076E-08 ) ) ;
#24932=CARTESIAN_POINT ( 'NONE',  ( -23.98503169607928953, -17.39005800936845603, 66.22885190747201989 ) ) ;
#24933=CYLINDRICAL_SURFACE ( 'NONE', #29028, 0.1500000000000015488 ) ;
#24935=CARTESIAN_POINT ( 'NONE',  ( -13.01616685277437391, -9.306763517318227485, 70.86397465682092900 ) ) ;
#24936=CARTESIAN_POINT ( 'NONE',  ( -19.24025795797341942, -7.996846695050864540, 60.24620885950562865 ) ) ;
#24937=CARTESIAN_POINT ( 'NONE',  ( -17.92193035392796929, -21.84160718002658541, 61.87535923543195082 ) ) ;
#24939=EDGE_LOOP ( 'NONE', ( #29025, #43013, #15499, #25036, #19743 ) ) ;
#24940=FACE_BOUND ( 'NONE', #40238, .T. ) ;
#24944=CARTESIAN_POINT ( 'NONE',  ( -20.49170831689750827, -8.461258797198503601, 63.59649424907591708 ) ) ;
#24946=EDGE_LOOP ( 'NONE', ( #18922, #30601, #14121, #12931, #38339 ) ) ;
#24947=CARTESIAN_POINT ( 'NONE',  ( -11.97224129167519280, -8.309940731205241349, 54.49999999999995026 ) ) ;
#24948=VECTOR ( 'NONE', #2961, 999.9999999999998863 ) ;
#24949=CARTESIAN_POINT ( 'NONE',  ( -16.95842795909200618, -7.774453609861648573, 74.25458489456045186 ) ) ;
#24950=CARTESIAN_POINT ( 'NONE',  ( -20.87593624383936941, -21.41133309587159417, 58.83749320122741722 ) ) ;
#24952=LINE ( 'NONE', #2549, #40158 ) ;
#24953=ORIENTED_EDGE ( 'NONE', *, *, #24409, .T. ) ;
#24956=CARTESIAN_POINT ( 'NONE',  ( -10.00368807899092971, -15.89896712085359098, 47.99999999999994316 ) ) ;
#24961=CARTESIAN_POINT ( 'NONE',  ( -24.38391081516821401, -14.06024225110868464, 73.12271507915593816 ) ) ;
#24962=ORIENTED_EDGE ( 'NONE', *, *, #33099, .F. ) ;
#24963=CARTESIAN_POINT ( 'NONE',  ( -20.98580030992770418, -20.83533690608478040, 65.88453944791919525 ) ) ;
#24966=( BOUNDED_CURVE ( )  B_SPLINE_CURVE ( 3, ( #9854, #40133, #24870, #36411 ),
 .UNSPECIFIED., .F., .F. ) 
 B_SPLINE_CURVE_WITH_KNOTS ( ( 4, 4 ),
 ( 0.000000000000000000, 0.4074455897393582937 ),
 .UNSPECIFIED. ) 
 CURVE ( )  GEOMETRIC_REPRESENTATION_ITEM ( )  RATIONAL_B_SPLINE_CURVE ( ( 1.000000000000000000, 0.4567392136813337444, 0.3561768502900309330, 0.6983129098260915102 ) ) 
 REPRESENTATION_ITEM ( '' )  );
#24968=CARTESIAN_POINT ( 'NONE',  ( -24.42173158938954813, -14.58342408866059614, 66.25462932207040012 ) ) ;
#24970=AXIS2_PLACEMENT_3D ( 'NONE', #17428, #22103, #32460 ) ;
#24972=VERTEX_POINT ( 'NONE', #18295 ) ;
#24975=VERTEX_POINT ( 'NONE', #10457 ) ;
#24977=CARTESIAN_POINT ( 'NONE',  ( -24.84263255441417328, -14.11714595057820354, 73.30926835346492965 ) ) ;
#24978=VECTOR ( 'NONE', #15083, 999.9999999999998863 ) ;
#24980=CARTESIAN_POINT ( 'NONE',  ( -16.74292201677715752, -21.77598521546333643, 65.41667504381256038 ) ) ;
#24981=FACE_OUTER_BOUND ( 'NONE', #43387, .T. ) ;
#24983=CARTESIAN_POINT ( 'NONE',  ( -23.79168800850164800, -18.67653690130417132, 72.91368233453137293 ) ) ;
#24984=( BOUNDED_CURVE ( )  B_SPLINE_CURVE ( 3, ( #10071, #20676, #1949, #9603 ),
 .UNSPECIFIED., .F., .F. ) 
 B_SPLINE_CURVE_WITH_KNOTS ( ( 4, 4 ),
 ( 0.000000000000000000, 0.4074455897393627346 ),
 .UNSPECIFIED. ) 
 CURVE ( )  GEOMETRIC_REPRESENTATION_ITEM ( )  RATIONAL_B_SPLINE_CURVE ( ( 1.000000000000000000, 0.4567392136813296366, 0.3561768502900294342, 0.6983129098260993928 ) ) 
 REPRESENTATION_ITEM ( '' )  );
#24986=CARTESIAN_POINT ( 'NONE',  ( -12.27604185553471616, -19.62628656662749549, 58.21210303282668264 ) ) ;
#24987=CARTESIAN_POINT ( 'NONE',  ( -19.81804402429900236, -8.174913897241847138, 73.60608030023824710 ) ) ;
#24989=CARTESIAN_POINT ( 'NONE',  ( -16.57921203443829583, -21.81142124131518756, 69.11049422539112186 ) ) ;
#24990=DIRECTION ( 'NONE',  ( 0.8565259173193582320, -0.5161040137028850561, 6.301967848571305848E-08 ) ) ;
#24992=CARTESIAN_POINT ( 'NONE',  ( -16.57554889599778747, -22.21081103083016117, 65.41059783760971413 ) ) ;
#24993=CARTESIAN_POINT ( 'NONE',  ( -12.05615918852498680, -19.97535170061420828, 61.51183199568394144 ) ) ;
#24994=CARTESIAN_POINT ( 'NONE',  ( -13.34910555009277111, -20.50135914746042687, 58.33033577015955728 ) ) ;
#24995=ADVANCED_FACE ( 'NONE', ( #14579 ), #37010, .T. ) ;
#24997=CARTESIAN_POINT ( 'NONE',  ( -10.04612636579397389, -15.84390794478046338, 64.64738251167817396 ) ) ;
#24998=( BOUNDED_CURVE ( )  B_SPLINE_CURVE ( 3, ( #46891, #38769, #13131, #28182 ),
 .UNSPECIFIED., .F., .F. ) 
 B_SPLINE_CURVE_WITH_KNOTS ( ( 4, 4 ),
 ( 0.5000000000000000000, 0.9074455897393592929 ),
 .UNSPECIFIED. ) 
 CURVE ( )  GEOMETRIC_REPRESENTATION_ITEM ( )  RATIONAL_B_SPLINE_CURVE ( ( 1.000000000000007550, 0.4567392136813483439, 0.3561768502900309330, 0.6983129098260637546 ) ) 
 REPRESENTATION_ITEM ( '' )  );
#24999=ORIENTED_EDGE ( 'NONE', *, *, #31669, .T. ) ;
#25001=EDGE_LOOP ( 'NONE', ( #17221, #31954, #21289, #22279, #42176 ) ) ;
#25004=CARTESIAN_POINT ( 'NONE',  ( -24.22092292145011072, -12.93687797069018153, 66.60246741374322710 ) ) ;
#25005=CYLINDRICAL_SURFACE ( 'NONE', #15, 0.1500000000000008549 ) ;
#25006=CARTESIAN_POINT ( 'NONE',  ( -22.62394951084894146, -10.04809318868971424, 70.29706442286226320 ) ) ;
#25007=VECTOR ( 'NONE', #22556, 1000.000000000000227 ) ;
#25009=ORIENTED_EDGE ( 'NONE', *, *, #21348, .F. ) ;
#25015=CARTESIAN_POINT ( 'NONE',  ( -24.06395315815399272, -17.02595776467518363, 73.18336026098602076 ) ) ;
#25019=ORIENTED_EDGE ( 'NONE', *, *, #37606, .T. ) ;
#25020=EDGE_CURVE ( 'NONE', #32027, #47544, #33067, .T. ) ;
#25021=CARTESIAN_POINT ( 'NONE',  ( -23.30963478160716562, -18.69084381296369557, 69.30844128244088154 ) ) ;
#25023=ORIENTED_EDGE ( 'NONE', *, *, #11020, .F. ) ;
#25024=FACE_OUTER_BOUND ( 'NONE', #32944, .T. ) ;
#25025=EDGE_LOOP ( 'NONE', ( #21893, #30222 ) ) ;
#25026=DIRECTION ( 'NONE',  ( 0.9629498065864410261, 0.2696806815386222911, 3.246020392366875918E-17 ) ) ;
#25027=CARTESIAN_POINT ( 'NONE',  ( -11.29476715451500723, -19.04418240398407391, 68.47335581180095687 ) ) ;
#25031=CARTESIAN_POINT ( 'NONE',  ( -19.24025795797341942, -7.996846695050864540, 60.24620885950562865 ) ) ;
#25032=VECTOR ( 'NONE', #2530, 1000.000000000000000 ) ;
#25036=ORIENTED_EDGE ( 'NONE', *, *, #47532, .F. ) ;
#25037=CARTESIAN_POINT ( 'NONE',  ( -20.64396943983181743, -21.02470340508176250, 58.94475165022391394 ) ) ;
#25038=AXIS2_PLACEMENT_3D ( 'NONE', #11733, #41776, #37079 ) ;
#25042=ORIENTED_EDGE ( 'NONE', *, *, #12884, .F. ) ;
#25043=CARTESIAN_POINT ( 'NONE',  ( -15.15660932275500095, -21.48492473237050859, 65.39124617759186719 ) ) ;
#25044=CARTESIAN_POINT ( 'NONE',  ( -18.53201889041905659, -7.846807422456379300, 73.99064401781672018 ) ) ;
#25046=DIRECTION ( 'NONE',  ( 0.7224352045700188629, 0.6914386272098739239, -9.340627245513718311E-09 ) ) ;
#25047=CARTESIAN_POINT ( 'NONE',  ( -13.57572078670752447, -20.65643022133334128, 61.81646323932617548 ) ) ;
#25048=B_SPLINE_CURVE_WITH_KNOTS ( 'NONE', 1,
 ( #25237, #8837 ),
 .UNSPECIFIED., .F., .F.,
 ( 2, 2 ),
 ( 0.000000000000000000, 1.000000000000000000 ),
 .UNSPECIFIED. ) ;
#25049=EDGE_LOOP ( 'NONE', ( #32849, #15570, #32845, #23577, #14255 ) ) ;
#25052=CARTESIAN_POINT ( 'NONE',  ( -18.97799580819609844, -7.523008705935653850, 67.09345912586260852 ) ) ;
#25053=ADVANCED_FACE ( 'NONE', ( #37494 ), #36753, .T. ) ;
#25054=CARTESIAN_POINT ( 'NONE',  ( -23.38308684513804891, -18.48213489539728371, 69.48475052504386440 ) ) ;
#25055=ORIENTED_EDGE ( 'NONE', *, *, #9875, .T. ) ;
#25056=CARTESIAN_POINT ( 'NONE',  ( -10.18401502636761968, -13.05277926903019470, 71.32333192088977114 ) ) ;
#25057=CARTESIAN_POINT ( 'NONE',  ( -24.77581774434673889, -16.01560321267006159, 66.16986595299408691 ) ) ;
#25058=EDGE_LOOP ( 'NONE', ( #43947, #45838 ) ) ;
#25059=VERTEX_POINT ( 'NONE', #18798 ) ;
#25060=CARTESIAN_POINT ( 'NONE',  ( -10.70034849704600788, -12.85632423166505944, 67.92759470734964111 ) ) ;
#25061=CARTESIAN_POINT ( 'NONE',  ( -15.69736699998981422, -8.025519224215527103, 70.60989840319118116 ) ) ;
#25062=CARTESIAN_POINT ( 'NONE',  ( -13.18342752238402582, -20.93459749068556874, 58.09004124675303160 ) ) ;
#25063=CARTESIAN_POINT ( 'NONE',  ( -10.48020486909296523, -13.57339180249324784, 74.56328874061136958 ) ) ;
#25064=DIRECTION ( 'NONE',  ( -5.731567514496413899E-31, -1.020425574103664789E-16, -1.000000000000000000 ) ) ;
#25065=CYLINDRICAL_SURFACE ( 'NONE', #29898, 0.1499999999999995226 ) ;
#25068=CARTESIAN_POINT ( 'NONE',  ( -17.84735443592641602, -7.371153788697909270, 60.19565345827741965 ) ) ;
#25069=ORIENTED_EDGE ( 'NONE', *, *, #961, .T. ) ;
#25070=ORIENTED_EDGE ( 'NONE', *, *, #45007, .F. ) ;
#25071=CARTESIAN_POINT ( 'NONE',  ( -24.46809763383182101, -15.25302497427750303, 73.15870697135122214 ) ) ;
#25074=CARTESIAN_POINT ( 'NONE',  ( -14.92764441971231726, -21.34891144748960201, 61.93600440564248544 ) ) ;
#25075=CARTESIAN_POINT ( 'NONE',  ( -10.97013626231024830, -17.52378408739619431, 71.75645163686851902 ) ) ;
#25079=VECTOR ( 'NONE', #31409, 1000.000000000000000 ) ;
#25080=ORIENTED_EDGE ( 'NONE', *, *, #21678, .F. ) ;
#25081=EDGE_CURVE ( 'NONE', #7578, #8735, #33548, .T. ) ;
#25082=CARTESIAN_POINT ( 'NONE',  ( -15.10203878652056630, -21.46900354431040725, 61.52111843893123933 ) ) ;
#25085=CARTESIAN_POINT ( 'NONE',  ( -14.72744631621160494, -8.295007313424175521, 60.60524229057013201 ) ) ;
#25086=CARTESIAN_POINT ( 'NONE',  ( -11.21364313603757168, -18.92425114470789538, 64.93981204116175832 ) ) ;
#25087=AXIS2_PLACEMENT_3D ( 'NONE', #20137, #1173, #5622 ) ;
#25089=CARTESIAN_POINT ( 'NONE',  ( -13.76849323099554567, -20.83774554052356365, 65.27156739751333703 ) ) ;
#25091=EDGE_CURVE ( 'NONE', #10114, #2367, #43636, .T. ) ;
#25094=DIRECTION ( 'NONE',  ( 0.07061531369766044230, 0.9975036227860933913, 1.268851335910971019E-08 ) ) ;
#25102=EDGE_CURVE ( 'NONE', #32937, #37435, #43008, .T. ) ;
#25103=CARTESIAN_POINT ( 'NONE',  ( -11.05034076241727625, -11.79557573020262318, 71.37388789199357575 ) ) ;
#25104=CARTESIAN_POINT ( 'NONE',  ( -12.61446418420489124, -20.49964817803554595, 71.91998392462126333 ) ) ;
#25106=DIRECTION ( 'NONE',  ( 0.5589780652556124441, -0.8291824422665291516, 7.938832475108296738E-08 ) ) ;
#25107=CARTESIAN_POINT ( 'NONE',  ( -16.93025400261081614, -7.375423323426211653, 74.12051638600156878 ) ) ;
#25109=ORIENTED_EDGE ( 'NONE', *, *, #37983, .T. ) ;
#25110=CARTESIAN_POINT ( 'NONE',  ( -17.11594671439511828, -7.315539529225058679, 54.27966884056655061 ) ) ;
#25114=CARTESIAN_POINT ( 'NONE',  ( -23.29918339618657086, -19.39037464299967439, 58.99915238703562181 ) ) ;
#25115=CARTESIAN_POINT ( 'NONE',  ( -23.38410522734749009, -10.33907873996118276, 59.71708144416061970 ) ) ;
#25116=ORIENTED_EDGE ( 'NONE', *, *, #33091, .T. ) ;
#25117=ORIENTED_EDGE ( 'NONE', *, *, #32459, .T. ) ;
#25118=CARTESIAN_POINT ( 'NONE',  ( -22.53429316287767392, -9.952421288698296564, 73.63161091678163928 ) ) ;
#25119=CARTESIAN_POINT ( 'NONE',  ( -21.42336286209559759, -21.09487474236010485, 69.23945462178221533 ) ) ;
#25120=VERTEX_POINT ( 'NONE', #27165 ) ;
#25121=CARTESIAN_POINT ( 'NONE',  ( -10.44568875397917296, -15.81166898614220706, 64.50771614034250945 ) ) ;
#25124=CARTESIAN_POINT ( 'NONE',  ( -10.03035368457962662, -15.72374687363213575, 61.22284448286259817 ) ) ;
#25125=( BOUNDED_CURVE ( )  B_SPLINE_CURVE ( 3, ( #37517, #41230, #45913, #7518 ),
 .UNSPECIFIED., .F., .F. ) 
 B_SPLINE_CURVE_WITH_KNOTS ( ( 4, 4 ),
 ( 0.000000000000000000, 0.4074455897393693959 ),
 .UNSPECIFIED. ) 
 CURVE ( )  GEOMETRIC_REPRESENTATION_ITEM ( )  RATIONAL_B_SPLINE_CURVE ( ( 1.000000000000000000, 0.4567392136813228087, 0.3561768502900268807, 0.6983129098261122714 ) ) 
 REPRESENTATION_ITEM ( '' )  );
#25126=CARTESIAN_POINT ( 'NONE',  ( -16.93783521594581387, -21.79229702504021304, 68.80446639304301470 ) ) ;
#25128=ORIENTED_EDGE ( 'NONE', *, *, #11208, .F. ) ;
#25129=CARTESIAN_POINT ( 'NONE',  ( -13.38462656077074442, -20.58719956993326861, 58.19650077713541947 ) ) ;
#25131=CARTESIAN_POINT ( 'NONE',  ( -13.95122194917832914, -8.664767797030865637, 70.88524802578001527 ) ) ;
#25132=CARTESIAN_POINT ( 'NONE',  ( -14.81380287721095357, -8.256357904232213940, 63.88158797558475754 ) ) ;
#25134=( BOUNDED_SURFACE ( )  B_SPLINE_SURFACE ( 3, 1, ( 
 ( #10667, #40692 ),
 ( #3022, #18277 ),
 ( #48573, #44649 ),
 ( #25931, #37228 ),
 ( #22477, #47616 ),
 ( #13847, #25207 ),
 ( #17790, #30125 ) ),
 .UNSPECIFIED., .T., .F., .F. ) 
 B_SPLINE_SURFACE_WITH_KNOTS ( ( 4, 3, 4 ),
 ( 2, 2 ),
 ( 0.000000000000000000, 0.5000000000000000000, 1.000000000000000000 ),
 ( 0.000000000000000000, 1.000000000000000000 ),
 .UNSPECIFIED. ) 
 GEOMETRIC_REPRESENTATION_ITEM ( )  RATIONAL_B_SPLINE_SURFACE ( (
 ( 1.000000000000000000, 1.000000000000000000),
 ( 0.3333333333333335369, 0.3333333333333330373),
 ( 0.3333333333333335369, 0.3333333333333330373),
 ( 1.000000000000000000, 1.000000000000000000),
 ( 0.3333333333333333703, 0.3333333333333333703),
 ( 0.3333333333333333703, 0.3333333333333333703),
 ( 1.000000000000000000, 1.000000000000000000) ) ) 
 REPRESENTATION_ITEM ( '' )  SURFACE ( )  );
#25135=ORIENTED_EDGE ( 'NONE', *, *, #38105, .T. ) ;
#25137=CARTESIAN_POINT ( 'NONE',  ( -24.46506320217640962, -17.24406362331221132, 72.99840605271779737 ) ) ;
#25139=AXIS2_PLACEMENT_3D ( 'NONE', #41931, #8207, #23224 ) ;
#25140=DIRECTION ( 'NONE',  ( 8.560949391518745609E-06, -2.380493834460222846E-06, 0.9999999999605218015 ) ) ;
#25141=ORIENTED_EDGE ( 'NONE', *, *, #38238, .F. ) ;
#25142=VECTOR ( 'NONE', #10753, 1000.000000000000000 ) ;
#25143=CARTESIAN_POINT ( 'NONE',  ( -24.24928796324336133, -13.25435532323388976, 59.37770298071973230 ) ) ;
#25144=CARTESIAN_POINT ( 'NONE',  ( -23.75797251732913296, -17.78947179557082592, 59.00378417803962350 ) ) ;
#25145=ORIENTED_EDGE ( 'NONE', *, *, #34457, .F. ) ;
#25146=CARTESIAN_POINT ( 'NONE',  ( -11.27262641912073882, -11.35749776731469218, 67.91864759325788725 ) ) ;
#25148=CARTESIAN_POINT ( 'NONE',  ( -12.99758137947571157, -9.386477775907486887, 71.14925353122600882 ) ) ;
#25149=CARTESIAN_POINT ( 'NONE',  ( -23.37084835027744489, -10.32157900363995573, 59.70229188760873740 ) ) ;
#25151=CARTESIAN_POINT ( 'NONE',  ( -24.11794058161805054, -12.76166764465371628, 69.77243002474142486 ) ) ;
#25152=EDGE_LOOP ( 'NONE', ( #47860, #21503, #26812, #33999, #45480 ) ) ;
#25153=CARTESIAN_POINT ( 'NONE',  ( -24.34502386579654498, -17.56683345968398768, 66.12852568699506151 ) ) ;
#25154=DIRECTION ( 'NONE',  ( -0.7171836970970659753, 0.6968841687240312499, -4.479616660400631173E-09 ) ) ;
#25155=CARTESIAN_POINT ( 'NONE',  ( -19.30025855022017112, -21.55315516297060441, 58.54009773080257872 ) ) ;
#25156=B_SPLINE_CURVE_WITH_KNOTS ( 'NONE', 1,
 ( #9165, #17255 ),
 .UNSPECIFIED., .F., .F.,
 ( 2, 2 ),
 ( 0.000000000000000000, 1.000000000000000000 ),
 .UNSPECIFIED. ) ;
#25157=EDGE_LOOP ( 'NONE', ( #21643, #32742 ) ) ;
#25159=EDGE_CURVE ( 'NONE', #20248, #34217, #31622, .T. ) ;
#25160=EDGE_CURVE ( 'NONE', #27722, #6597, #16479, .T. ) ;
#25161=CARTESIAN_POINT ( 'NONE',  ( -23.68653687815194786, -11.57061008776568123, 66.43686604568146947 ) ) ;
#25162=PLANE ( 'NONE',  #10042 ) ;
#25163=FACE_OUTER_BOUND ( 'NONE', #1296, .T. ) ;
#25164=CARTESIAN_POINT ( 'NONE',  ( -13.41559485503361948, -8.529420403834853559, 57.08472365561223683 ) ) ;
#25165=ORIENTED_EDGE ( 'NONE', *, *, #38290, .T. ) ;
#25167=CARTESIAN_POINT ( 'NONE',  ( -11.68672781637937419, -10.05669048882576533, 67.68392176937598492 ) ) ;
#25168=CARTESIAN_POINT ( 'NONE',  ( -14.78754716229542687, -8.270772359302402066, 60.31996282000579157 ) ) ;
#25169=ADVANCED_FACE ( 'NONE', ( #22756 ), #38476, .T. ) ;
#25172=CARTESIAN_POINT ( 'NONE',  ( -10.77303329795002895, -12.62668660113453178, 60.79853568451941470 ) ) ;
#25173=CARTESIAN_POINT ( 'NONE',  ( -11.87700371968174551, -10.45801594763104170, 71.26893088143391708 ) ) ;
#25174=ORIENTED_EDGE ( 'NONE', *, *, #31104, .T. ) ;
#25175=ORIENTED_EDGE ( 'NONE', *, *, #38698, .F. ) ;
#25177=CARTESIAN_POINT ( 'NONE',  ( -21.06702863216100141, -20.84540773593991148, 65.86981821684420879 ) ) ;
#25179=VERTEX_POINT ( 'NONE', #342 ) ;
#25180=CARTESIAN_POINT ( 'NONE',  ( -10.11824992584547545, -16.26811798947522192, 71.56255103782838489 ) ) ;
#25181=CARTESIAN_POINT ( 'NONE',  ( -11.70868151386493672, -18.85353134555335330, 71.87613056707397163 ) ) ;
#25182=CARTESIAN_POINT ( 'NONE',  ( -20.37299714182665866, -8.405577154986387356, 67.08104082189564110 ) ) ;
#25183=CARTESIAN_POINT ( 'NONE',  ( -23.75797251732913296, -17.78947179557082592, 59.00378417803962350 ) ) ;
#25185=ORIENTED_EDGE ( 'NONE', *, *, #10917, .F. ) ;
#25186=CARTESIAN_POINT ( 'NONE',  ( -24.40614610099494541, -15.84163519271677956, 62.74895499471147531 ) ) ;
#25188=AXIS2_PLACEMENT_3D ( 'NONE', #9754, #29182, #2596 ) ;
#25189=CARTESIAN_POINT ( 'NONE',  ( -15.56465948913147557, -7.543361525925788236, 53.49999999999994316 ) ) ;
#25190=( BOUNDED_CURVE ( )  B_SPLINE_CURVE ( 3, ( #32824, #29884, #44916, #29146 ),
 .UNSPECIFIED., .F., .F. ) 
 B_SPLINE_CURVE_WITH_KNOTS ( ( 4, 4 ),
 ( 0.000000000000000000, 0.4074455897393656212 ),
 .UNSPECIFIED. ) 
 CURVE ( )  GEOMETRIC_REPRESENTATION_ITEM ( )  RATIONAL_B_SPLINE_CURVE ( ( 1.000000000000000000, 0.4567392136813309689, 0.3561768502900299338, 0.6983129098260969503 ) ) 
 REPRESENTATION_ITEM ( '' )  );
#25192=ADVANCED_FACE ( 'NONE', ( #15571 ), #15328, .T. ) ;
#25193=ORIENTED_EDGE ( 'NONE', *, *, #35992, .T. ) ;
#25194=DIRECTION ( 'NONE',  ( 0.9990515194385546360, 0.04354378839186318767, -1.103613758316045351E-08 ) ) ;
#25195=CARTESIAN_POINT ( 'NONE',  ( -16.84865286310842336, -21.83598151670433296, 68.98088545748413480 ) ) ;
#25197=CARTESIAN_POINT ( 'NONE',  ( -24.29765692699610113, -13.47630289685046279, 59.55195110948075410 ) ) ;
#25198=CARTESIAN_POINT ( 'NONE',  ( -20.81244001423283407, -21.44422669384312741, 58.76758266138310915 ) ) ;
#25199=CARTESIAN_POINT ( 'NONE',  ( -10.98892314574976226, -11.92244160250971419, 70.97372176798174337 ) ) ;
#25200=LINE ( 'NONE', #36014, #12598 ) ;
#25201=ORIENTED_EDGE ( 'NONE', *, *, #20168, .F. ) ;
#25205=CARTESIAN_POINT ( 'NONE',  ( -11.73260633559210042, -10.00184260618991416, 67.61401560909513364 ) ) ;
#25206=CARTESIAN_POINT ( 'NONE',  ( -21.73098984888145679, -8.730191469543168381, 70.31627926275058371 ) ) ;
#25207=CARTESIAN_POINT ( 'NONE',  ( -16.09495291808068274, -22.13976250616876840, 58.54231521589509413 ) ) ;
#25208=ORIENTED_EDGE ( 'NONE', *, *, #46453, .T. ) ;
#25210=CYLINDRICAL_SURFACE ( 'NONE', #7151, 0.1500000000000029365 ) ;
#25211=CARTESIAN_POINT ( 'NONE',  ( -20.78451513435706133, -21.00713107796517320, 62.12943504870421663 ) ) ;
#25215=CARTESIAN_POINT ( 'NONE',  ( -15.47038549838128674, -21.58309193914155344, 72.19575460769013375 ) ) ;
#25216=ORIENTED_EDGE ( 'NONE', *, *, #29778, .T. ) ;
#25217=CARTESIAN_POINT ( 'NONE',  ( -19.10745041116545906, -21.66349580942223341, 62.13936675129127707 ) ) ;
#25218=LINE ( 'NONE', #39507, #29892 ) ;
#25225=CARTESIAN_POINT ( 'NONE',  ( -16.67010138129746721, -21.76854072801680928, 65.24066787124687039 ) ) ;
#25226=CARTESIAN_POINT ( 'NONE',  ( -10.72530867274958410, -17.00760959713300835, 57.97288447305809456 ) ) ;
#25227=VERTEX_POINT ( 'NONE', #38223 ) ;
#25230=CARTESIAN_POINT ( 'NONE',  ( -24.94227079592050345, -14.76255220537544233, 53.76227901944321275 ) ) ;
#25231=EDGE_CURVE ( 'NONE', #18094, #14812, #4507, .T. ) ;
#25234=EDGE_CURVE ( 'NONE', #7245, #47302, #21208, .T. ) ;
#25235=B_SPLINE_CURVE_WITH_KNOTS ( 'NONE', 3,
 ( #17245, #2948, #32040, #13546, #14259, #43126, #1999, #9397, #36202, #2484 ),
 .UNSPECIFIED., .F., .F.,
 ( 4, 2, 2, 2, 4 ),
 ( 0.000000000000000000, 0.2500000000000000000, 0.5000000000000000000, 0.7500000000000000000, 1.000000000000000000 ),
 .UNSPECIFIED. ) ;
#25237=CARTESIAN_POINT ( 'NONE',  ( -22.83929682888979329, -10.29453308790037980, 66.55654356380499337 ) ) ;
#25238=EDGE_LOOP ( 'NONE', ( #28569, #24058, #10023, #14373, #7416 ) ) ;
#25239=DIRECTION ( 'NONE',  ( -0.04287186434519785205, -0.9990805789562556827, 2.806673972535349411E-09 ) ) ;
#25240=EDGE_CURVE ( 'NONE', #32808, #27374, #28382, .T. ) ;
#25241=CARTESIAN_POINT ( 'NONE',  ( -18.57335281209669731, -21.76520412651811043, 72.57038810541313012 ) ) ;
#25243=ORIENTED_EDGE ( 'NONE', *, *, #9217, .F. ) ;
#25244=CARTESIAN_POINT ( 'NONE',  ( -24.16575310113231012, -12.74704012323608104, 70.07243002239955842 ) ) ;
#25247=ORIENTED_EDGE ( 'NONE', *, *, #36881, .F. ) ;
#25248=ORIENTED_EDGE ( 'NONE', *, *, #34271, .T. ) ;
#25250=CARTESIAN_POINT ( 'NONE',  ( -16.15307827456697254, -21.74383799326970390, 58.29145396122345346 ) ) ;
#25252=DIRECTION ( 'NONE',  ( 3.892913445306193086E-06, 4.639959643356220421E-06, 0.9999999999816580054 ) ) ;
#25255=VERTEX_POINT ( 'NONE', #28848 ) ;
#25256=ORIENTED_EDGE ( 'NONE', *, *, #26946, .T. ) ;
#25258=CARTESIAN_POINT ( 'NONE',  ( -20.13271805750754595, -8.299978134201072777, 70.53628287813307907 ) ) ;
#25259=CYLINDRICAL_SURFACE ( 'NONE', #13408, 0.1500000000000040190 ) ;
#25260=( BOUNDED_CURVE ( )  B_SPLINE_CURVE ( 3, ( #21478, #39939, #5497, #35989 ),
 .UNSPECIFIED., .F., .F. ) 
 B_SPLINE_CURVE_WITH_KNOTS ( ( 4, 4 ),
 ( 0.000000000000000000, 0.4074455897393639559 ),
 .UNSPECIFIED. ) 
 CURVE ( )  GEOMETRIC_REPRESENTATION_ITEM ( )  RATIONAL_B_SPLINE_CURVE ( ( 1.000000000000000000, 0.4567392136813363535, 0.3561768502900319322, 0.6983129098260867362 ) ) 
 REPRESENTATION_ITEM ( '' )  );
#25263=CARTESIAN_POINT ( 'NONE',  ( -15.40811923343076906, -21.56513327689926030, 72.06047564147742435 ) ) ;
#25264=VECTOR ( 'NONE', #22609, 999.9999999999998863 ) ;
#25265=B_SPLINE_CURVE_WITH_KNOTS ( 'NONE', 1,
 ( #10809, #25829 ),
 .UNSPECIFIED., .F., .F.,
 ( 2, 2 ),
 ( 0.000000000000000000, 1.000000000000000000 ),
 .UNSPECIFIED. ) ;
#25266=DIRECTION ( 'NONE',  ( 0.7658821528503445553, 0.6346126762488748518, 0.1033986416233889927 ) ) ;
#25269=DIRECTION ( 'NONE',  ( -0.7107718805962432995, -0.7034225854731134264, -7.722840056494081040E-09 ) ) ;
#25270=( BOUNDED_SURFACE ( )  B_SPLINE_SURFACE ( 3, 1, ( 
 ( #8238, #23022 ),
 ( #38006, #19304 ),
 ( #15589, #23252 ),
 ( #47364, #1807 ),
 ( #16807, #24712 ),
 ( #39717, #31846 ),
 ( #5262, #21256 ) ),
 .UNSPECIFIED., .T., .F., .F. ) 
 B_SPLINE_SURFACE_WITH_KNOTS ( ( 4, 3, 4 ),
 ( 2, 2 ),
 ( 0.000000000000000000, 0.5000000000000000000, 1.000000000000000000 ),
 ( 0.000000000000000000, 1.000000000000000000 ),
 .UNSPECIFIED. ) 
 GEOMETRIC_REPRESENTATION_ITEM ( )  RATIONAL_B_SPLINE_SURFACE ( (
 ( 1.000000000000000000, 1.000000000000000000),
 ( 0.3333333333333335369, 0.3333333333333330373),
 ( 0.3333333333333335369, 0.3333333333333330373),
 ( 1.000000000000000000, 1.000000000000000000),
 ( 0.3333333333333333703, 0.3333333333333333703),
 ( 0.3333333333333333703, 0.3333333333333333703),
 ( 1.000000000000000000, 1.000000000000000000) ) ) 
 REPRESENTATION_ITEM ( '' )  SURFACE ( )  );
#25271=ORIENTED_EDGE ( 'NONE', *, *, #34483, .F. ) ;
#25272=AXIS2_PLACEMENT_3D ( 'NONE', #25856, #14492, #40617 ) ;
#25273=CARTESIAN_POINT ( 'NONE',  ( -12.44869005970189058, -9.885249076858732664, 57.08935532200567309 ) ) ;
#25274=CARTESIAN_POINT ( 'NONE',  ( -11.45045256087476027, -18.56827314959498310, 68.36122809857093330 ) ) ;
#25275=CARTESIAN_POINT ( 'NONE',  ( -20.98580030992770418, -20.83533690608478040, 65.88453944791919525 ) ) ;
#25276=ORIENTED_EDGE ( 'NONE', *, *, #24890, .F. ) ;
#25277=CARTESIAN_POINT ( 'NONE',  ( -19.37638992839121954, -7.619477365241829503, 60.00447059577386710 ) ) ;
#25278=CARTESIAN_POINT ( 'NONE',  ( -11.77169535943213496, -10.59578862612641714, 74.73885051658085388 ) ) ;
#25279=FACE_OUTER_BOUND ( 'NONE', #18303, .T. ) ;
#25280=ORIENTED_EDGE ( 'NONE', *, *, #44068, .T. ) ;
#25284=CARTESIAN_POINT ( 'NONE',  ( -24.26435699358934883, -17.76123410301217120, 62.51715077956382771 ) ) ;
#25285=( BOUNDED_CURVE ( )  B_SPLINE_CURVE ( 3, ( #40638, #6916, #32767, #37172 ),
 .UNSPECIFIED., .F., .F. ) 
 B_SPLINE_CURVE_WITH_KNOTS ( ( 4, 4 ),
 ( 0.4074455897393695625, 0.5000000000000000000 ),
 .UNSPECIFIED. ) 
 CURVE ( )  GEOMETRIC_REPRESENTATION_ITEM ( )  RATIONAL_B_SPLINE_CURVE ( ( 0.6983129098261007250, 0.7760317562606826591, 0.8765941196519758671, 0.9999999999999646949 ) ) 
 REPRESENTATION_ITEM ( '' )  );
#25286=ORIENTED_EDGE ( 'NONE', *, *, #23033, .T. ) ;
#25287=CARTESIAN_POINT ( 'NONE',  ( -13.49409790474204840, -20.66256726344224504, 61.53118467422925164 ) ) ;
#25289=CARTESIAN_POINT ( 'NONE',  ( -13.24261801534493088, -8.643248549050911222, 60.55454889300790455 ) ) ;
#25290=CARTESIAN_POINT ( 'NONE',  ( -13.59065431704403615, -21.19813492939682220, 68.64280514999626348 ) ) ;
#25291=CARTESIAN_POINT ( 'NONE',  ( -13.38575581802539993, -9.030060914960570173, 60.72478133471773987 ) ) ;
#25293=CARTESIAN_POINT ( 'NONE',  ( -21.23898061349145650, -21.20841973409718406, 65.77728081245959402 ) ) ;
#25295=DIRECTION ( 'NONE',  ( -6.446466763177039895E-06, 1.047023821809670710E-05, 0.9999999999244085780 ) ) ;
#25296=AXIS2_PLACEMENT_3D ( 'NONE', #46095, #46593, #16993 ) ;
#25297=EDGE_CURVE ( 'NONE', #11365, #7957, #24791, .T. ) ;
#25298=CARTESIAN_POINT ( 'NONE',  ( -23.91632973644556159, -12.05317525496800357, 59.89724340139424896 ) ) ;
#25299=CARTESIAN_POINT ( 'NONE',  ( -21.57822623285374419, -8.624884721674641597, 73.70105113553994158 ) ) ;
#25300=ORIENTED_EDGE ( 'NONE', *, *, #27547, .F. ) ;
#25301=CARTESIAN_POINT ( 'NONE',  ( -10.16748990304072464, -13.12235252378331651, 71.39323974795351546 ) ) ;
#25303=CARTESIAN_POINT ( 'NONE',  ( -12.41791333049023116, -9.841008508234809327, 60.97406688302051947 ) ) ;
#25305=VERTEX_POINT ( 'NONE', #9427 ) ;
#25309=CYLINDRICAL_SURFACE ( 'NONE', #3846, 0.1499999999999964695 ) ;
#25311=CARTESIAN_POINT ( 'NONE',  ( -14.84266645611046442, -8.302458146920823623, 60.31996277900389458 ) ) ;
#25314=ORIENTED_EDGE ( 'NONE', *, *, #3673, .T. ) ;
#25318=CARTESIAN_POINT ( 'NONE',  ( -19.55442184481404766, -21.52995072282663358, 65.47958309245051112 ) ) ;
#25320=DIRECTION ( 'NONE',  ( -5.329554271033179131E-07, -1.313503372282854535E-06, -0.9999999999989953592 ) ) ;
#25321=CARTESIAN_POINT ( 'NONE',  ( -17.42409385541300892, -14.80920654474439502, 75.49999999999994316 ) ) ;
#25324=CARTESIAN_POINT ( 'NONE',  ( -21.95894689775886377, -20.14334376385412284, 62.30609413755689019 ) ) ;
#25325=CARTESIAN_POINT ( 'NONE',  ( -10.81230840161673967, -17.25685697075765646, 64.64211442681141762 ) ) ;
#25326=CARTESIAN_POINT ( 'NONE',  ( -14.59672178607931414, -8.347720424474937673, 60.20507679337548979 ) ) ;
#25327=CARTESIAN_POINT ( 'NONE',  ( -10.09291371782238045, -16.13494220690481384, 68.16263107114907882 ) ) ;
#25328=EDGE_CURVE ( 'NONE', #7640, #31648, #34721, .T. ) ;
#25329=ORIENTED_EDGE ( 'NONE', *, *, #20014, .T. ) ;
#25330=CARTESIAN_POINT ( 'NONE',  ( -10.59800981977604195, -16.35987635455024503, 71.63853451875513656 ) ) ;
#25332=CARTESIAN_POINT ( 'NONE',  ( -17.37357235347134932, -7.759347209999027051, 67.32039595933659371 ) ) ;
#25333=CYLINDRICAL_SURFACE ( 'NONE', #7092, 0.1499999999999964695 ) ;
#25335=B_SPLINE_CURVE_WITH_KNOTS ( 'NONE', 3,
 ( #3343, #29448, #36809, #14884, #10983, #37802, #22305, #3583, #6797, #30198 ),
 .UNSPECIFIED., .F., .F.,
 ( 4, 2, 2, 2, 4 ),
 ( 0.1272669073658610484, 0.2522669073463410516, 0.3772669073268209994, 0.5022669073073009471, 0.6272669072877810059 ),
 .UNSPECIFIED. ) ;
#25336=EDGE_CURVE ( 'NONE', #36571, #18999, #35512, .T. ) ;
#25338=CARTESIAN_POINT ( 'NONE',  ( -23.84039510144717511, -11.88788025021025874, 59.48235730685867395 ) ) ;
#25339=CARTESIAN_POINT ( 'NONE',  ( -17.64628924239291763, -7.362394388585356886, 63.67340115340124385 ) ) ;
#25340=B_SPLINE_CURVE_WITH_KNOTS ( 'NONE', 3,
 ( #25144, #21455, #3209, #17966, #14264, #6666, #32756, #47552, #36668, #13784 ),
 .UNSPECIFIED., .F., .F.,
 ( 4, 2, 2, 2, 4 ),
 ( 0.000000000000000000, 0.2500000000000000000, 0.5000000000000000000, 0.7500000000000000000, 1.000000000000000000 ),
 .UNSPECIFIED. ) ;
#25341=VERTEX_POINT ( 'NONE', #43154 ) ;
#25342=CARTESIAN_POINT ( 'NONE',  ( -18.35341103611197866, -21.74886582742231766, 72.39584113235251550 ) ) ;
#25343=CARTESIAN_POINT ( 'NONE',  ( -12.50897416063251733, -20.40789074996439112, 72.06299591474957822 ) ) ;
#25345=VERTEX_POINT ( 'NONE', #9674 ) ;
#25347=CARTESIAN_POINT ( 'NONE',  ( -24.86207103330155377, -14.38397445572853961, 66.30479991853488286 ) ) ;
#25348=ORIENTED_EDGE ( 'NONE', *, *, #1987, .F. ) ;
#25349=CARTESIAN_POINT ( 'NONE',  ( -10.95917937052863422, -17.62195967018737619, 71.58190244267143498 ) ) ;
#25350=CARTESIAN_POINT ( 'NONE',  ( -10.95360866178292625, -18.50214713473828709, 57.96861125158908834 ) ) ;
#25351=EDGE_CURVE ( 'NONE', #5623, #18657, #16494, .T. ) ;
#25352=LINE ( 'NONE', #47283, #36131 ) ;
#25354=ORIENTED_EDGE ( 'NONE', *, *, #7163, .F. ) ;
#25355=ORIENTED_EDGE ( 'NONE', *, *, #38895, .T. ) ;
#25356=CARTESIAN_POINT ( 'NONE',  ( -23.36875552208945095, -10.31881635475721737, 59.80214635332909978 ) ) ;
#25357=DIRECTION ( 'NONE',  ( -0.9000732436326449593, -0.4357386327795698122, 2.072980810273451456E-08 ) ) ;
#25358=ORIENTED_EDGE ( 'NONE', *, *, #12075, .F. ) ;
#25359=FACE_OUTER_BOUND ( 'NONE', #7121, .T. ) ;
#25360=B_SPLINE_CURVE_WITH_KNOTS ( 'NONE', 3,
 ( #5836, #27749, #42780, #16889, #1650, #40048, #21092, #47197, #31929, #6065 ),
 .UNSPECIFIED., .F., .F.,
 ( 4, 2, 2, 2, 4 ),
 ( 0.6272669072877643526, 0.7522669073072746349, 0.8772669073267849171, 1.002266907346295088, 1.127266907365805482 ),
 .UNSPECIFIED. ) ;
#25361=( BOUNDED_CURVE ( )  B_SPLINE_CURVE ( 3, ( #11052, #33421, #15206, #30017 ),
 .UNSPECIFIED., .F., .F. ) 
 B_SPLINE_CURVE_WITH_KNOTS ( ( 4, 4 ),
 ( 0.000000000000000000, 0.4074455897393629566 ),
 .UNSPECIFIED. ) 
 CURVE ( )  GEOMETRIC_REPRESENTATION_ITEM ( )  RATIONAL_B_SPLINE_CURVE ( ( 1.000000000000000000, 0.4567392136813351877, 0.3561768502900315436, 0.6983129098260889567 ) ) 
 REPRESENTATION_ITEM ( '' )  );
#25362=EDGE_CURVE ( 'NONE', #42067, #43505, #1113, .T. ) ;
#25364=CARTESIAN_POINT ( 'NONE',  ( -24.05813527555462628, -11.41757595432783745, 63.06562998582658253 ) ) ;
#25365=CARTESIAN_POINT ( 'NONE',  ( -12.84817825325788299, -8.930034686467767102, 67.42296837860310177 ) ) ;
#25366=CARTESIAN_POINT ( 'NONE',  ( -23.70794718243703514, -18.81148055198525171, 69.45405303023558474 ) ) ;
#25368=ORIENTED_EDGE ( 'NONE', *, *, #22323, .T. ) ;
#25369=CARTESIAN_POINT ( 'NONE',  ( -10.56265156832558105, -13.42272637098185939, 74.97817617512852451 ) ) ;
#25370=CARTESIAN_POINT ( 'NONE',  ( -14.10113443798904065, -8.141252799482343150, 70.98603544959661349 ) ) ;
#25371=CARTESIAN_POINT ( 'NONE',  ( -24.87417961795293664, -14.80849281899037884, 59.42795564617806292 ) ) ;
#25372=CARTESIAN_POINT ( 'NONE',  ( -16.58958238669307406, -22.21248813724601234, 65.36417849732876562 ) ) ;
#25374=EDGE_CURVE ( 'NONE', #48128, #36043, #40100, .T. ) ;
#25376=ORIENTED_EDGE ( 'NONE', *, *, #15675, .T. ) ;
#25379=CARTESIAN_POINT ( 'NONE',  ( -23.70135487130767515, -11.71146637837649074, 63.25218278684473461 ) ) ;
#25381=DIRECTION ( 'NONE',  ( -0.9999889394985580493, -0.004703284017506803583, 7.734398264755894983E-09 ) ) ;
#25383=CARTESIAN_POINT ( 'NONE',  ( -24.46986505407297585, -14.47671061003208415, 69.74455334859420930 ) ) ;
#25384=CARTESIAN_POINT ( 'NONE',  ( -13.68510254299556905, -20.79040957969665371, 68.75625391717530022 ) ) ;
#25386=CARTESIAN_POINT ( 'NONE',  ( -22.43638724005049667, -20.32197157274265820, 62.34783858214098728 ) ) ;
#25387=CARTESIAN_POINT ( 'NONE',  ( -24.87126894608573124, -14.60124070896847392, 62.75650584303257062 ) ) ;
#25388=CARTESIAN_POINT ( 'NONE',  ( -15.74023824147349337, -8.014750687795812567, 67.33110349041905351 ) ) ;
#25389=B_SPLINE_CURVE_WITH_KNOTS ( 'NONE', 3,
 ( #9563, #20393, #5857, #43291, #24584, #38615, #9076, #8587, #23855, #23612 ),
 .UNSPECIFIED., .F., .F.,
 ( 4, 2, 2, 2, 4 ),
 ( 0.6272669072782746102, 0.7522669073001777562, 0.8772669073220807912, 1.002266907343983826, 1.127266907365886972 ),
 .UNSPECIFIED. ) ;
#25394=CARTESIAN_POINT ( 'NONE',  ( -11.53247046633659600, -18.68106308600668797, 64.74707076449911369 ) ) ;
#25395=EDGE_LOOP ( 'NONE', ( #32015, #10720 ) ) ;
#25396=CARTESIAN_POINT ( 'NONE',  ( -13.90804716676048258, -20.86209139562971160, 68.45625137333186672 ) ) ;
#25397=CARTESIAN_POINT ( 'NONE',  ( -24.08517543038346531, -12.49907855475201579, 73.52753481283211556 ) ) ;
#25398=VECTOR ( 'NONE', #24732, 1000.000000000000227 ) ;
#25399=CARTESIAN_POINT ( 'NONE',  ( -12.25434508901797770, -20.17367074759813406, 65.05170324716399932 ) ) ;
#25400=( BOUNDED_CURVE ( )  B_SPLINE_CURVE ( 3, ( #39044, #9263, #17108, #35592 ),
 .UNSPECIFIED., .F., .F. ) 
 B_SPLINE_CURVE_WITH_KNOTS ( ( 4, 4 ),
 ( 0.9074455897393715054, 1.000000000000000000 ),
 .UNSPECIFIED. ) 
 CURVE ( )  GEOMETRIC_REPRESENTATION_ITEM ( )  RATIONAL_B_SPLINE_CURVE ( ( 0.6983129098260993928, 0.7760317562607036423, 0.8765941196520038448, 1.000000000000000000 ) ) 
 REPRESENTATION_ITEM ( '' )  );
#25401=CARTESIAN_POINT ( 'NONE',  ( -10.05973382411576189, -15.93640770713343535, 64.68488457034484895 ) ) ;
#25402=CARTESIAN_POINT ( 'NONE',  ( -19.37484620200115160, -7.619050568204919216, 60.14588398245204814 ) ) ;
#25403=CARTESIAN_POINT ( 'NONE',  ( -24.23177493074759425, -12.96287917719623017, 69.86423168924338256 ) ) ;
#25405=CYLINDRICAL_SURFACE ( 'NONE', #9772, 0.1500000000000031863 ) ;
#25406=CARTESIAN_POINT ( 'NONE',  ( -10.76763551407085373, -17.13171859787639661, 61.45743118825841123 ) ) ;
#25409=ADVANCED_FACE ( 'NONE', ( #33483 ), #22196, .T. ) ;
#25410=CARTESIAN_POINT ( 'NONE',  ( -9.908656216309283948, -19.57032361137281384, 53.49999999999995026 ) ) ;
#25412=ORIENTED_EDGE ( 'NONE', *, *, #13516, .F. ) ;
#25413=ORIENTED_EDGE ( 'NONE', *, *, #20460, .T. ) ;
#25414=CARTESIAN_POINT ( 'NONE',  ( -11.10386593012501244, -18.75361831986885974, 61.32064883311096537 ) ) ;
#25415=CARTESIAN_POINT ( 'NONE',  ( -20.88270815654435353, -21.40782497263450068, 58.82970582236164603 ) ) ;
#25416=EDGE_LOOP ( 'NONE', ( #35894, #29991, #47817, #6516, #37492 ) ) ;
#25417=CARTESIAN_POINT ( 'NONE',  ( -23.62594491300536959, -11.45603751788689095, 66.70742424642772050 ) ) ;
#25418=CARTESIAN_POINT ( 'NONE',  ( -20.52359238471669300, -8.472965537638735611, 59.84125077296574347 ) ) ;
#25420=CARTESIAN_POINT ( 'NONE',  ( -23.03538909537400770, -9.907469116741831172, 70.19833813022523827 ) ) ;
#25421=CARTESIAN_POINT ( 'NONE',  ( -22.22371030936713510, -9.111184089457765367, 59.90666523727240644 ) ) ;
#25423=CARTESIAN_POINT ( 'NONE',  ( -24.35389707626741185, -16.10709931453381216, 62.87856533165624029 ) ) ;
#25424=CARTESIAN_POINT ( 'NONE',  ( -24.82675434745867449, -13.96959720065245136, 73.24458743042187336 ) ) ;
#25425=( BOUNDED_CURVE ( )  B_SPLINE_CURVE ( 3, ( #29329, #21698, #17981, #48517 ),
 .UNSPECIFIED., .F., .F. ) 
 B_SPLINE_CURVE_WITH_KNOTS ( ( 4, 4 ),
 ( 0.000000000000000000, 0.4074455897393655657 ),
 .UNSPECIFIED. ) 
 CURVE ( )  GEOMETRIC_REPRESENTATION_ITEM ( )  RATIONAL_B_SPLINE_CURVE ( ( 1.000000000000000000, 0.4567392136813248626, 0.3561768502900276578, 0.6983129098261082746 ) ) 
 REPRESENTATION_ITEM ( '' )  );
#25426=CARTESIAN_POINT ( 'NONE',  ( -10.42278039055306849, -14.74509148815288739, 74.98706025067703251 ) ) ;
#25427=CARTESIAN_POINT ( 'NONE',  ( -14.87282237418130215, -7.809539361298669213, 57.02812736438108487 ) ) ;
#25430=CARTESIAN_POINT ( 'NONE',  ( -10.56016083362581703, -13.18709213229180932, 67.62343541709479666 ) ) ;
#25432=CARTESIAN_POINT ( 'NONE',  ( -24.61605428079846547, -12.86511719609775284, 66.41751453275240635 ) ) ;
#25433=CARTESIAN_POINT ( 'NONE',  ( -13.86779599075735092, -20.83853035579127067, 65.09514786855950774 ) ) ;
#25434=CARTESIAN_POINT ( 'NONE',  ( -11.50273595086851763, -11.07590776185467263, 57.20903212540526539 ) ) ;
#25435=B_SPLINE_CURVE_WITH_KNOTS ( 'NONE', 3,
 ( #20303, #42949, #20059, #27690, #1326, #28179, #5779, #46887, #31382, #8751 ),
 .UNSPECIFIED., .F., .F.,
 ( 4, 2, 2, 2, 4 ),
 ( 0.1272669073658437844, 0.2522669073488139624, 0.3772669073317841959, 0.5022669073147544294, 0.6272669072977246074 ),
 .UNSPECIFIED. ) ;
#25436=ADVANCED_FACE ( 'NONE', ( #18478 ), #29832, .T. ) ;
#25437=ORIENTED_EDGE ( 'NONE', *, *, #5945, .F. ) ;
#25442=EDGE_CURVE ( 'NONE', #19604, #23975, #21551, .T. ) ;
#25445=DIRECTION ( 'NONE',  ( -1.404489950266683237E-08, 6.428047446179355909E-07, 0.9999999999997932765 ) ) ;
#25446=CARTESIAN_POINT ( 'NONE',  ( -21.57946453887431204, -8.565578233975859490, 47.99999999999994316 ) ) ;
#25447=CARTESIAN_POINT ( 'NONE',  ( -16.59344411340201475, -21.75974756046277747, 65.22564390621562325 ) ) ;
#25448=VERTEX_POINT ( 'NONE', #26135 ) ;
#25450=ORIENTED_EDGE ( 'NONE', *, *, #19034, .F. ) ;
#25451=DIRECTION ( 'NONE',  ( 0.7971031148784507581, -0.6038432116460916710, 6.916509187980650173E-08 ) ) ;
#25452=FACE_OUTER_BOUND ( 'NONE', #4297, .T. ) ;
#25453=ORIENTED_EDGE ( 'NONE', *, *, #38434, .F. ) ;
#25454=CARTESIAN_POINT ( 'NONE',  ( -23.16117746674104438, -18.90708040007733359, 62.63934749780565880 ) ) ;
#25455=CARTESIAN_POINT ( 'NONE',  ( -21.42200791050363051, -21.09572771556245740, 69.09804232902482113 ) ) ;
#25457=EDGE_LOOP ( 'NONE', ( #42214, #7429, #20488, #25348, #47647 ) ) ;
#25459=ADVANCED_FACE ( 'NONE', ( #18235 ), #41147, .F. ) ;
#25460=CARTESIAN_POINT ( 'NONE',  ( -23.95986381193147707, -17.46034710541827906, 69.82828398331871256 ) ) ;
#25462=DIRECTION ( 'NONE',  ( 1.006957036571142899E-05, -6.253991264129192257E-06, -0.9999999999297457531 ) ) ;
#25465=CARTESIAN_POINT ( 'NONE',  ( -10.73211873618052969, -12.75535506112652584, 60.87141649276334476 ) ) ;
#25466=CARTESIAN_POINT ( 'NONE',  ( -23.69928304873747038, -18.82488403301566038, 69.33726028187463442 ) ) ;
#25467=CARTESIAN_POINT ( 'NONE',  ( -11.97212546196701943, -10.32690635925306211, 74.58318462221375000 ) ) ;
#25469=CARTESIAN_POINT ( 'NONE',  ( -16.84865286310842336, -21.83598151670433296, 68.98088545748413480 ) ) ;
#25470=CARTESIAN_POINT ( 'NONE',  ( -14.91432061146141663, -8.212540298998538546, 63.93411529719415398 ) ) ;
#25471=ORIENTED_EDGE ( 'NONE', *, *, #44476, .T. ) ;
#25472=CARTESIAN_POINT ( 'NONE',  ( -24.35040279276217845, -17.55351991699908609, 66.10390635504940349 ) ) ;
#25474=CARTESIAN_POINT ( 'NONE',  ( -11.89178903705324863, -10.43929771899554915, 71.26893105542536944 ) ) ;
#25477=VERTEX_POINT ( 'NONE', #29575 ) ;
#25478=ORIENTED_EDGE ( 'NONE', *, *, #24078, .F. ) ;
#25479=CARTESIAN_POINT ( 'NONE',  ( -11.52915434062558120, -10.92788463621912420, 60.82318916367986361 ) ) ;
#25481=CARTESIAN_POINT ( 'NONE',  ( -12.81450749931373245, -9.474957484202729319, 74.31923006089486705 ) ) ;
#25482=ORIENTED_EDGE ( 'NONE', *, *, #46776, .F. ) ;
#25483=EDGE_LOOP ( 'NONE', ( #48553, #30093, #47906, #36997, #7804 ) ) ;
#25485=EDGE_CURVE ( 'NONE', #42753, #48265, #6556, .T. ) ;
#25490=ADVANCED_FACE ( 'NONE', ( #48282 ), #33740, .T. ) ;
#25493=FACE_OUTER_BOUND ( 'NONE', #4923, .T. ) ;
#25494=AXIS2_PLACEMENT_3D ( 'NONE', #22147, #47520, #37129 ) ;
#25495=EDGE_CURVE ( 'NONE', #40380, #48456, #48046, .T. ) ;
#25496=CARTESIAN_POINT ( 'NONE',  ( -14.48548941065489970, -8.400516866317895293, 67.27447142263336843 ) ) ;
#25497=EDGE_CURVE ( 'NONE', #12297, #10202, #23141, .T. ) ;
#25498=CARTESIAN_POINT ( 'NONE',  ( -24.40217300928714650, -14.25566238011515274, 69.65275273531472067 ) ) ;
#25499=VERTEX_POINT ( 'NONE', #45341 ) ;
#25500=CARTESIAN_POINT ( 'NONE',  ( -11.21157628577468657, -11.58358644131346082, 67.61864608155907774 ) ) ;
#25501=ORIENTED_EDGE ( 'NONE', *, *, #12502, .T. ) ;
#25503=CARTESIAN_POINT ( 'NONE',  ( -19.45790264050342699, -21.50891717485947652, 65.57559305958521634 ) ) ;
#25504=CARTESIAN_POINT ( 'NONE',  ( -10.50893933415051507, -13.43540278197274063, 74.96345540680638919 ) ) ;
#25505=CARTESIAN_POINT ( 'NONE',  ( -10.39868982912479645, -12.32967425775121306, 57.50574246823239122 ) ) ;
#25507=EDGE_LOOP ( 'NONE', ( #27991, #13519 ) ) ;
#25514=CARTESIAN_POINT ( 'NONE',  ( -18.76715758977493209, -7.481188742717107765, 70.41422074109146934 ) ) ;
#25516=CARTESIAN_POINT ( 'NONE',  ( -11.73209289625006058, -10.73465601455801099, 74.51172899894849877 ) ) ;
#25517=VERTEX_POINT ( 'NONE', #3974 ) ;
#25518=CARTESIAN_POINT ( 'NONE',  ( -10.33483191699034265, -17.09962811228164270, 57.73114616685904110 ) ) ;
#25519=CARTESIAN_POINT ( 'NONE',  ( -24.66548415425539531, -13.05833320866972613, 62.93990042163805043 ) ) ;
#25521=CARTESIAN_POINT ( 'NONE',  ( -23.41616298382994898, -18.52428493080399008, 72.77840375779385340 ) ) ;
#25522=ORIENTED_EDGE ( 'NONE', *, *, #47592, .F. ) ;
#25523=LINE ( 'NONE', #28975, #18155 ) ;
#25526=ORIENTED_EDGE ( 'NONE', *, *, #8919, .T. ) ;
#25527=CARTESIAN_POINT ( 'NONE',  ( -14.07539681412751165, -8.605278097683305205, 74.49954655214880006 ) ) ;
#25528=AXIS2_PLACEMENT_3D ( 'NONE', #943, #19404, #26810 ) ;
#25530=ORIENTED_EDGE ( 'NONE', *, *, #22571, .T. ) ;
#25531=VERTEX_POINT ( 'NONE', #23174 ) ;
#25532=CARTESIAN_POINT ( 'NONE',  ( -14.92957465851463006, -21.82926012297162899, 65.22101360901100975 ) ) ;
#25533=CARTESIAN_POINT ( 'NONE',  ( -15.34465393633500518, -21.54586957516256263, 68.86120835375241711 ) ) ;
#25534=CARTESIAN_POINT ( 'NONE',  ( -10.13783977983156248, -13.25541127610578762, 74.79322348855123437 ) ) ;
#25535=CARTESIAN_POINT ( 'NONE',  ( -20.36536858953947515, -8.398766899984980938, 63.19632798853695022 ) ) ;
#25536=( BOUNDED_CURVE ( )  B_SPLINE_CURVE ( 3, ( #36476, #40662, #25418, #6943 ),
 .UNSPECIFIED., .F., .F. ) 
 B_SPLINE_CURVE_WITH_KNOTS ( ( 4, 4 ),
 ( 0.000000000000000000, 0.4074455897393672310 ),
 .UNSPECIFIED. ) 
 CURVE ( )  GEOMETRIC_REPRESENTATION_ITEM ( )  RATIONAL_B_SPLINE_CURVE ( ( 1.000000000000000000, 0.4567392136813244186, 0.3561768502900274913, 0.6983129098261091627 ) ) 
 REPRESENTATION_ITEM ( '' )  );
#25538=CARTESIAN_POINT ( 'NONE',  ( -14.87886284476815923, -8.287862385134991072, 60.60379677410870869 ) ) ;
#25539=CARTESIAN_POINT ( 'NONE',  ( -12.19808601445598306, -20.11893053951551735, 65.04487616575880793 ) ) ;
#25541=ORIENTED_EDGE ( 'NONE', *, *, #10436, .T. ) ;
#25546=CARTESIAN_POINT ( 'NONE',  ( -23.76319945593019156, -11.71557033483072985, 66.72214621596255313 ) ) ;
#25548=FACE_OUTER_BOUND ( 'NONE', #24130, .T. ) ;
#25549=ORIENTED_EDGE ( 'NONE', *, *, #19899, .T. ) ;
#25551=( BOUNDED_SURFACE ( )  B_SPLINE_SURFACE ( 3, 1, ( 
 ( #39833, #44039 ),
 ( #40321, #21129 ),
 ( #6591, #36127 ),
 ( #23689, #32908 ),
 ( #31298, #47952 ),
 ( #38686, #17885 ),
 ( #2410, #44276 ) ),
 .UNSPECIFIED., .T., .F., .F. ) 
 B_SPLINE_SURFACE_WITH_KNOTS ( ( 4, 3, 4 ),
 ( 2, 2 ),
 ( 0.000000000000000000, 0.5000000000000000000, 1.000000000000000000 ),
 ( 0.000000000000000000, 1.000000000000000000 ),
 .UNSPECIFIED. ) 
 GEOMETRIC_REPRESENTATION_ITEM ( )  RATIONAL_B_SPLINE_SURFACE ( (
 ( 1.000000000000000000, 1.000000000000000000),
 ( 0.3333333333333335369, 0.3333333333333330373),
 ( 0.3333333333333335369, 0.3333333333333330373),
 ( 1.000000000000000000, 1.000000000000000000),
 ( 0.3333333333333333703, 0.3333333333333333703),
 ( 0.3333333333333333703, 0.3333333333333333703),
 ( 1.000000000000000000, 1.000000000000000000) ) ) 
 REPRESENTATION_ITEM ( '' )  SURFACE ( )  );
#25552=ORIENTED_EDGE ( 'NONE', *, *, #48209, .F. ) ;
#25553=CARTESIAN_POINT ( 'NONE',  ( -22.02981006882838955, -20.08072627601145399, 62.53439177585065778 ) ) ;
#25556=CARTESIAN_POINT ( 'NONE',  ( -16.41515664040973022, -21.78667843868697318, 62.05568103759625842 ) ) ;
#25557=CARTESIAN_POINT ( 'NONE',  ( -11.20449214220105816, -18.91032654392478207, 64.94695843806114510 ) ) ;
#25559=ORIENTED_EDGE ( 'NONE', *, *, #5260, .F. ) ;
#25562=EDGE_CURVE ( 'NONE', #28462, #5991, #18069, .T. ) ;
#25564=CARTESIAN_POINT ( 'NONE',  ( -14.66741299049177094, -8.374868138257010486, 60.51099561025887397 ) ) ;
#25567=DIRECTION ( 'NONE',  ( 3.141253923644155253E-07, -8.288700512985352896E-07, 0.9999999999996072031 ) ) ;
#25568=EDGE_CURVE ( 'NONE', #16133, #1136, #46060, .T. ) ;
#25569=B_SPLINE_CURVE_WITH_KNOTS ( 'NONE', 1,
 ( #42642, #20705 ),
 .UNSPECIFIED., .F., .F.,
 ( 2, 2 ),
 ( 0.000000000000000000, 1.000000000000000000 ),
 .UNSPECIFIED. ) ;
#25570=FACE_OUTER_BOUND ( 'NONE', #16037, .T. ) ;
#25571=ORIENTED_EDGE ( 'NONE', *, *, #18188, .F. ) ;
#25572=CARTESIAN_POINT ( 'NONE',  ( -20.85666738206293047, -20.91166016791921578, 65.69527100157196742 ) ) ;
#25573=ORIENTED_EDGE ( 'NONE', *, *, #3687, .T. ) ;
#25575=EDGE_LOOP ( 'NONE', ( #6421, #37793, #47829, #16421 ) ) ;
#25576=DIRECTION ( 'NONE',  ( -6.385196548387842039E-06, 5.147825516598811523E-06, -0.9999999999663645722 ) ) ;
#25577=DIRECTION ( 'NONE',  ( -3.141253907721240275E-07, 8.288700426223213302E-07, -0.9999999999996070921 ) ) ;
#25578=ORIENTED_EDGE ( 'NONE', *, *, #5551, .T. ) ;
#25579=CYLINDRICAL_SURFACE ( 'NONE', #7969, 0.1500000000000002998 ) ;
#25580=CARTESIAN_POINT ( 'NONE',  ( -19.81157080418587313, -21.44583120317290081, 65.34997476282926243 ) ) ;
#25582=EDGE_LOOP ( 'NONE', ( #41476, #2946 ) ) ;
#25583=CARTESIAN_POINT ( 'NONE',  ( -24.40217295060720204, -14.25566147773195524, 69.95275273531336779 ) ) ;
#25584=DIRECTION ( 'NONE',  ( -1.206829990499677715E-05, -1.995688260022264671E-06, -0.9999999999251866223 ) ) ;
#25585=CARTESIAN_POINT ( 'NONE',  ( -23.74619244455239553, -11.68933966055485030, 63.25218278636739910 ) ) ;
#25586=VERTEX_POINT ( 'NONE', #30571 ) ;
#25588=CARTESIAN_POINT ( 'NONE',  ( -22.84776207900630851, -9.701615188675109636, 73.73807001133110361 ) ) ;
#25589=CARTESIAN_POINT ( 'NONE',  ( -11.93102662126159785, -10.47028825497329585, 70.96893105764984000 ) ) ;
#25590=CARTESIAN_POINT ( 'NONE',  ( -17.65298207767979477, -7.812888375568328492, 60.30734138473366102 ) ) ;
#25592=CARTESIAN_POINT ( 'NONE',  ( -24.12071508562369715, -11.54438765950021306, 63.06722961171875852 ) ) ;
#25593=EDGE_CURVE ( 'NONE', #48265, #37822, #17087, .T. ) ;
#25594=CARTESIAN_POINT ( 'NONE',  ( -16.78865379391102408, -21.78030513117466072, 68.69560651887046276 ) ) ;
#25595=PLANE ( 'NONE',  #10345 ) ;
#25596=VECTOR ( 'NONE', #37213, 1000.000000000000114 ) ;
#25598=CARTESIAN_POINT ( 'NONE',  ( -20.94324281608204430, -8.242681057013424351, 60.09771182510558418 ) ) ;
#25601=CARTESIAN_POINT ( 'NONE',  ( -11.57425704488359841, -18.65360627554439077, 65.04707076833931012 ) ) ;
#25602=EDGE_LOOP ( 'NONE', ( #26088, #40371, #15563, #39154, #18222 ) ) ;
#25604=CARTESIAN_POINT ( 'NONE',  ( -20.63429004897692920, -8.588635981428261346, 60.12659873706649449 ) ) ;
#25605=CARTESIAN_POINT ( 'NONE',  ( -24.86242989439883289, -14.39095395922188558, 66.36788051138485400 ) ) ;
#25606=EDGE_CURVE ( 'NONE', #34242, #42959, #31316, .T. ) ;
#25607=CARTESIAN_POINT ( 'NONE',  ( -23.32859574730126084, -19.35227928776919626, 58.98387009178664186 ) ) ;
#25608=CARTESIAN_POINT ( 'NONE',  ( -24.30978138445934533, -13.29580787541330444, 59.66267893655142984 ) ) ;
#25610=VERTEX_POINT ( 'NONE', #26622 ) ;
#25611=CARTESIAN_POINT ( 'NONE',  ( -11.54646099848356222, -18.70898497394131255, 61.27710574299381108 ) ) ;
#25613=CARTESIAN_POINT ( 'NONE',  ( -10.96142808812597735, -11.10142881709785101, 64.33537400591416144 ) ) ;
#25614=ORIENTED_EDGE ( 'NONE', *, *, #5531, .T. ) ;
#25615=CARTESIAN_POINT ( 'NONE',  ( -13.69193161217391363, -21.25696551969686965, 68.65613906552292178 ) ) ;
#25616=ADVANCED_FACE ( 'NONE', ( #30814 ), #6445, .T. ) ;
#25617=CARTESIAN_POINT ( 'NONE',  ( -12.89377865171026905, -9.472814404202125615, 70.92213358633685516 ) ) ;
#25618=CARTESIAN_POINT ( 'NONE',  ( -22.90738119516900539, -10.37220287249194683, 59.81023178929109463 ) ) ;
#25622=EDGE_LOOP ( 'NONE', ( #37113, #31920, #21122, #13296, #16021 ) ) ;
#25623=CARTESIAN_POINT ( 'NONE',  ( -22.78151580134219500, -19.98625284378301004, 72.75905219260647527 ) ) ;
#25624=CARTESIAN_POINT ( 'NONE',  ( -12.15466845058241674, -8.150045384784233349, 54.38277594638588397 ) ) ;
#25625=ORIENTED_EDGE ( 'NONE', *, *, #31505, .F. ) ;
#25626=DIRECTION ( 'NONE',  ( -0.4415479322351564262, -0.8912598635915878198, 0.1033986416233890898 ) ) ;
#25627=CARTESIAN_POINT ( 'NONE',  ( -24.51865387586880729, -12.53305138704347144, 73.42880879726919829 ) ) ;
#25629=CARTESIAN_POINT ( 'NONE',  ( -14.37872387272655850, -8.506304085067752041, 67.54509766762896561 ) ) ;
#25631=CARTESIAN_POINT ( 'NONE',  ( -10.79541835452027776, -17.05898387227370705, 57.76048578130984623 ) ) ;
#25634=CARTESIAN_POINT ( 'NONE',  ( -20.58080933007877533, -8.501275685423019368, 67.08104112728932478 ) ) ;
#25635=EDGE_CURVE ( 'NONE', #15096, #27258, #20194, .T. ) ;
#25637=CARTESIAN_POINT ( 'NONE',  ( -21.47456293661849713, -9.038556783377254433, 70.41660404402310292 ) ) ;
#25638=CARTESIAN_POINT ( 'NONE',  ( -22.23733827145997566, -19.96043728507621040, 65.70421731380814379 ) ) ;
#25639=CARTESIAN_POINT ( 'NONE',  ( -13.35712140185222019, -20.57241581739411984, 61.81646620894163391 ) ) ;
#25641=CARTESIAN_POINT ( 'NONE',  ( -24.28473927714575353, -16.19956134247464519, 62.59328727871961462 ) ) ;
#25643=ORIENTED_EDGE ( 'NONE', *, *, #16213, .T. ) ;
#25644=CARTESIAN_POINT ( 'NONE',  ( -24.49878988761138388, -12.47402815302071843, 73.36508674653782691 ) ) ;
#25646=CARTESIAN_POINT ( 'NONE',  ( -15.41171220965234134, -7.636089294961081464, 74.18711515319478167 ) ) ;
#25648=EDGE_CURVE ( 'NONE', #28690, #25694, #30030, .T. ) ;
#25650=CARTESIAN_POINT ( 'NONE',  ( -15.47038452772150841, -21.58309165278561537, 72.04575460769355288 ) ) ;
#25652=FACE_BOUND ( 'NONE', #17326, .T. ) ;
#25653=CARTESIAN_POINT ( 'NONE',  ( -24.83000351354337099, -13.99979019377566125, 73.22247878125472198 ) ) ;
#25654=CARTESIAN_POINT ( 'NONE',  ( -11.41951145912443266, -19.21922708312919426, 71.79411749213964811 ) ) ;
#25655=CARTESIAN_POINT ( 'NONE',  ( -17.19811928533322387, -9.313850733363548073, 53.49999999999995026 ) ) ;
#25656=ORIENTED_EDGE ( 'NONE', *, *, #44476, .F. ) ;
#25660=CARTESIAN_POINT ( 'NONE',  ( -10.37462438995674319, -14.89569194323783208, 74.79778901495059529 ) ) ;
#25661=CARTESIAN_POINT ( 'NONE',  ( -24.21645823680271903, -12.90730551592505115, 63.04083907877015491 ) ) ;
#25663=B_SPLINE_CURVE_WITH_KNOTS ( 'NONE', 3,
 ( #29977, #45014, #33899, #26273, #37092, #33149, #48427, #14657, #41538, #7824 ),
 .UNSPECIFIED., .F., .F.,
 ( 4, 2, 2, 2, 4 ),
 ( 0.000000000000000000, 0.2500000000000000000, 0.5000000000000000000, 0.7500000000000000000, 1.000000000000000000 ),
 .UNSPECIFIED. ) ;
#25664=FACE_OUTER_BOUND ( 'NONE', #11628, .T. ) ;
#25671=B_SPLINE_CURVE_WITH_KNOTS ( 'NONE', 3,
 ( #27156, #16536, #31575, #20500, #42178, #41934, #8211, #23471, #4751, #38467 ),
 .UNSPECIFIED., .F., .F.,
 ( 4, 2, 2, 2, 4 ),
 ( 0.1272669073658183603, 0.2522669073463091882, 0.3772669073268000162, 0.5022669073072908441, 0.6272669072877816721 ),
 .UNSPECIFIED. ) ;
#25672=CARTESIAN_POINT ( 'NONE',  ( -16.98261326800368209, -21.79527086262147861, 72.16543221550985265 ) ) ;
#25673=CARTESIAN_POINT ( 'NONE',  ( -23.99919193691511410, -17.21124756729841465, 69.41339796233270931 ) ) ;
#25674=ADVANCED_FACE ( 'NONE', ( #35929 ), #26878, .T. ) ;
#25675=CARTESIAN_POINT ( 'NONE',  ( -15.72937801229072541, -7.965776692693047778, 70.61549658711864197 ) ) ;
#25676=CARTESIAN_POINT ( 'NONE',  ( -10.37210014130659275, -14.68995570394611505, 75.21267707208666309 ) ) ;
#25677=EDGE_LOOP ( 'NONE', ( #43271, #28103, #8214, #29323, #22635, #47074, #8428, #19949, #30130, #5319, #47090, #45331 ) ) ;
#25679=CARTESIAN_POINT ( 'NONE',  ( -23.13465042048557763, -10.02438105578966621, 66.68148899222990167 ) ) ;
#25680=CARTESIAN_POINT ( 'NONE',  ( -12.44533934557844113, -9.817553771701762244, 57.09495291247809945 ) ) ;
#25681=VERTEX_POINT ( 'NONE', #9850 ) ;
#25682=( BOUNDED_CURVE ( )  B_SPLINE_CURVE ( 3, ( #4574, #34851, #34603, #27948 ),
 .UNSPECIFIED., .F., .F. ) 
 B_SPLINE_CURVE_WITH_KNOTS ( ( 4, 4 ),
 ( 0.5000000000000000000, 0.9074455897393659543 ),
 .UNSPECIFIED. ) 
 CURVE ( )  GEOMETRIC_REPRESENTATION_ITEM ( )  RATIONAL_B_SPLINE_CURVE ( ( 0.9999999999999836797, 0.4567392136813330783, 0.3561768502900419797, 0.6983129098260927314 ) ) 
 REPRESENTATION_ITEM ( '' )  );
#25684=CARTESIAN_POINT ( 'NONE',  ( -23.82366785274684418, -10.99486113721019009, 73.47697904737684382 ) ) ;
#25685=ORIENTED_EDGE ( 'NONE', *, *, #15596, .T. ) ;
#25687=CARTESIAN_POINT ( 'NONE',  ( -11.04141120970326462, -11.93494789359697883, 74.55840195308121565 ) ) ;
#25688=CARTESIAN_POINT ( 'NONE',  ( -9.979603215878100286, -14.52052451035377345, 68.04295550616701860 ) ) ;
#25689=ORIENTED_EDGE ( 'NONE', *, *, #23614, .F. ) ;
#25690=CYLINDRICAL_SURFACE ( 'NONE', #44323, 0.1499999999999994671 ) ;
#25691=CARTESIAN_POINT ( 'NONE',  ( -23.36642407317085812, -18.50986088251124073, 73.04751736639515514 ) ) ;
#25694=VERTEX_POINT ( 'NONE', #21173 ) ;
#25695=CARTESIAN_POINT ( 'NONE',  ( -21.58848639831018090, -8.631801418357438749, 73.75128750060586924 ) ) ;
#25696=DIRECTION ( 'NONE',  ( -7.110378524392051906E-06, -9.728165310344191876E-06, 0.9999999999274027385 ) ) ;
#25697=( BOUNDED_SURFACE ( )  B_SPLINE_SURFACE ( 3, 1, ( 
 ( #644, #7810 ),
 ( #15645, #26021 ),
 ( #26755, #41038 ),
 ( #37559, #26256 ),
 ( #37313, #30700 ),
 ( #41271, #11479 ),
 ( #40784, #3863 ) ),
 .UNSPECIFIED., .T., .F., .F. ) 
 B_SPLINE_SURFACE_WITH_KNOTS ( ( 4, 3, 4 ),
 ( 2, 2 ),
 ( 0.000000000000000000, 0.5000000000000000000, 1.000000000000000000 ),
 ( 0.000000000000000000, 1.000000000000000000 ),
 .UNSPECIFIED. ) 
 GEOMETRIC_REPRESENTATION_ITEM ( )  RATIONAL_B_SPLINE_SURFACE ( (
 ( 1.000000000000000000, 1.000000000000000000),
 ( 0.3333333333333335369, 0.3333333333333330373),
 ( 0.3333333333333335369, 0.3333333333333330373),
 ( 1.000000000000000000, 1.000000000000000000),
 ( 0.3333333333333333703, 0.3333333333333333703),
 ( 0.3333333333333333703, 0.3333333333333333703),
 ( 1.000000000000000000, 1.000000000000000000) ) ) 
 REPRESENTATION_ITEM ( '' )  SURFACE ( )  );
#25698=ADVANCED_FACE ( 'NONE', ( #36166 ), #12566, .T. ) ;
#25701=CARTESIAN_POINT ( 'NONE',  ( -16.61787835827217563, -21.81669226458268795, 61.75567858111494246 ) ) ;
#25702=EDGE_CURVE ( 'NONE', #18272, #12703, #23906, .T. ) ;
#25703=EDGE_CURVE ( 'NONE', #11292, #22956, #38507, .T. ) ;
#25705=EDGE_CURVE ( 'NONE', #2873, #17241, #3575, .T. ) ;
#25707=DIRECTION ( 'NONE',  ( -5.731567514496413899E-31, -1.020425574103664789E-16, -1.000000000000000000 ) ) ;
#25710=CARTESIAN_POINT ( 'NONE',  ( -24.22092292145011072, -12.93687797069018153, 66.60246741374322710 ) ) ;
#25711=AXIS2_PLACEMENT_3D ( 'NONE', #4871, #39554, #20614 ) ;
#25718=VERTEX_POINT ( 'NONE', #22380 ) ;
#25720=CARTESIAN_POINT ( 'NONE',  ( -14.40713934193096080, -8.490940502754424912, 70.84030674940029826 ) ) ;
#25721=CARTESIAN_POINT ( 'NONE',  ( -23.34190511704397153, -19.33504077159632573, 58.92764702605110472 ) ) ;
#25722=CARTESIAN_POINT ( 'NONE',  ( -18.11889201384288484, -21.82488578508536747, 65.34532159284481168 ) ) ;
#25723=CARTESIAN_POINT ( 'NONE',  ( -12.91576191806997542, -9.388722997169708151, 71.13453240065665284 ) ) ;
#25724=ORIENTED_EDGE ( 'NONE', *, *, #11299, .F. ) ;
#25728=CARTESIAN_POINT ( 'NONE',  ( -14.56979395989184844, -7.868632093599801536, 54.02222386812614729 ) ) ;
#25729=CARTESIAN_POINT ( 'NONE',  ( -24.47401588851211329, -14.84236380343934592, 59.24300237059242136 ) ) ;
#25733=EDGE_LOOP ( 'NONE', ( #43450, #39021, #12185, #3481, #21525 ) ) ;
#25734=CARTESIAN_POINT ( 'NONE',  ( -24.36278531766821231, -15.73455962487135551, 69.83307441201348809 ) ) ;
#25735=EDGE_CURVE ( 'NONE', #30777, #31226, #5343, .T. ) ;
#25736=CARTESIAN_POINT ( 'NONE',  ( -13.78028125966771178, -8.764572710043150749, 74.35521961121672518 ) ) ;
#25739=ORIENTED_EDGE ( 'NONE', *, *, #28644, .F. ) ;
#25740=CARTESIAN_POINT ( 'NONE',  ( -17.02512887036163747, -21.84805734118084786, 72.45983438422057077 ) ) ;
#25741=EDGE_LOOP ( 'NONE', ( #42501, #36926, #44477, #34404 ) ) ;
#25743=CARTESIAN_POINT ( 'NONE',  ( -20.31445822498897513, -8.433666593767874531, 66.78104076700890346 ) ) ;
#25744=CARTESIAN_POINT ( 'NONE',  ( -24.42383173988974221, -14.88139849484145216, 59.54300232022885808 ) ) ;
#25745=CARTESIAN_POINT ( 'NONE',  ( -24.40658449907488148, -15.78251210865724907, 69.53307488410803217 ) ) ;
#25746=ORIENTED_EDGE ( 'NONE', *, *, #33423, .F. ) ;
#25747=CARTESIAN_POINT ( 'NONE',  ( -23.44246603937665441, -11.23440635791340370, 70.08313896382058772 ) ) ;
#25748=CARTESIAN_POINT ( 'NONE',  ( -22.77624011198484411, -19.99176503748672218, 72.76683626849190034 ) ) ;
#25749=CARTESIAN_POINT ( 'NONE',  ( -19.36749320447652067, -7.617017704847905080, 60.13809874652617538 ) ) ;
#25750=CARTESIAN_POINT ( 'NONE',  ( -21.18398602608336745, -21.24092397535611809, 65.69958545398036165 ) ) ;
#25753=LINE ( 'NONE', #10735, #31320 ) ;
#25754=CARTESIAN_POINT ( 'NONE',  ( -10.70296955259081351, -11.59513340129999648, 71.27356289404251299 ) ) ;
#25755=EDGE_LOOP ( 'NONE', ( #2606, #20311, #31534, #24766, #42523 ) ) ;
#25756=FACE_BOUND ( 'NONE', #6963, .T. ) ;
#25757=VERTEX_POINT ( 'NONE', #13752 ) ;
#25760=CARTESIAN_POINT ( 'NONE',  ( -21.23484681875272528, -20.74088929683185611, 69.33978048267414351 ) ) ;
#25761=CARTESIAN_POINT ( 'NONE',  ( -24.64856881849836157, -12.98951230985249516, 62.95451385596734184 ) ) ;
#25762=LINE ( 'NONE', #33366, #31305 ) ;
#25764=CARTESIAN_POINT ( 'NONE',  ( -15.95864454847012581, -7.504678945485328434, 63.71365074502104875 ) ) ;
#25767=VERTEX_POINT ( 'NONE', #2687 ) ;
#25768=CARTESIAN_POINT ( 'NONE',  ( -12.67420009981309548, -9.069561984988212089, 71.00958696908303125 ) ) ;
#25769=CYLINDRICAL_SURFACE ( 'NONE', #7036, 0.1499999999999953038 ) ;
#25771=CARTESIAN_POINT ( 'NONE',  ( -20.54979434103954006, -8.489990112051950533, 63.61121512946457557 ) ) ;
#25773=ADVANCED_FACE ( 'NONE', ( #7375 ), #48271, .T. ) ;
#25774=EDGE_CURVE ( 'NONE', #21441, #14380, #4210, .T. ) ;
#25775=CARTESIAN_POINT ( 'NONE',  ( -13.52463770777002416, -20.62256002460651061, 58.11938029867636146 ) ) ;
#25777=ORIENTED_EDGE ( 'NONE', *, *, #5941, .T. ) ;
#25780=CARTESIAN_POINT ( 'NONE',  ( -23.22061493458723191, -18.82855841280685993, 69.59372281959836926 ) ) ;
#25782=CARTESIAN_POINT ( 'NONE',  ( -11.55760334190795646, -18.71930654562736507, 65.04147253430677722 ) ) ;
#25783=CARTESIAN_POINT ( 'NONE',  ( -10.32448118053900998, -17.06708155110676728, 57.83760547180983025 ) ) ;
#25785=CARTESIAN_POINT ( 'NONE',  ( -14.30855566557790226, -8.484641631233271752, 70.74429704309763167 ) ) ;
#25790=CARTESIAN_POINT ( 'NONE',  ( -24.43827367352892210, -15.52193379869737377, 73.28831629023289906 ) ) ;
#25791=EDGE_CURVE ( 'NONE', #11764, #8655, #37127, .T. ) ;
#25793=CARTESIAN_POINT ( 'NONE',  ( -21.07871280138893155, -21.30141328949765267, 62.25324875861664964 ) ) ;
#25795=DIRECTION ( 'NONE',  ( 0.9753750245375039096, 0.2205528542287732985, 7.244220459260265297E-08 ) ) ;
#25799=CARTESIAN_POINT ( 'NONE',  ( -22.00056395679878918, -20.10656929443474183, 62.51822596018408262 ) ) ;
#25800=CARTESIAN_POINT ( 'NONE',  ( -14.47983227664519212, -7.965588925009814858, 63.90483403727078837 ) ) ;
#25801=AXIS2_PLACEMENT_3D ( 'NONE', #44013, #9360, #10268 ) ;
#25802=CARTESIAN_POINT ( 'NONE',  ( -10.88286923018596575, -17.43962093083235843, 68.11193994895104709 ) ) ;
#25806=CARTESIAN_POINT ( 'NONE',  ( -10.52647097981341773, -16.26776460278879810, 71.74190558978101251 ) ) ;
#25807=CARTESIAN_POINT ( 'NONE',  ( -14.80624636014071172, -8.317144122717282428, 60.61996281969079803 ) ) ;
#25808=ORIENTED_EDGE ( 'NONE', *, *, #16613, .F. ) ;
#25809=CARTESIAN_POINT ( 'NONE',  ( -15.25374053646965855, -21.46424723517000643, 65.21482766330532854 ) ) ;
#25811=EDGE_LOOP ( 'NONE', ( #15581, #39972 ) ) ;
#25813=EDGE_LOOP ( 'NONE', ( #44799, #29069 ) ) ;
#25814=CARTESIAN_POINT ( 'NONE',  ( -10.30936164548169565, -17.01954009666350842, 57.84907067837097827 ) ) ;
#25815=CARTESIAN_POINT ( 'NONE',  ( -24.87306303946944652, -14.67811516855542742, 62.89109217698693755 ) ) ;
#25817=EDGE_CURVE ( 'NONE', #14105, #47823, #33445, .T. ) ;
#25818=CARTESIAN_POINT ( 'NONE',  ( -12.84817825325788299, -8.930034686467767102, 67.42296837860310177 ) ) ;
#25819=CARTESIAN_POINT ( 'NONE',  ( -18.60622205832422082, -22.16490843864383109, 72.47006330605313451 ) ) ;
#25820=ORIENTED_EDGE ( 'NONE', *, *, #39665, .F. ) ;
#25821=CARTESIAN_POINT ( 'NONE',  ( -18.79451800406743800, -7.944217934494487210, 70.65451536062514037 ) ) ;
#25822=( BOUNDED_CURVE ( )  B_SPLINE_CURVE ( 3, ( #22758, #37248, #30147, #34054 ),
 .UNSPECIFIED., .F., .F. ) 
 B_SPLINE_CURVE_WITH_KNOTS ( ( 4, 4 ),
 ( 0.5000000000000000000, 0.9074455897393649551 ),
 .UNSPECIFIED. ) 
 CURVE ( )  GEOMETRIC_REPRESENTATION_ITEM ( )  RATIONAL_B_SPLINE_CURVE ( ( 0.9999999999999769074, 0.4567392136813299697, 0.3561768502900456435, 0.6983129098260987266 ) ) 
 REPRESENTATION_ITEM ( '' )  );
#25823=LINE ( 'NONE', #11059, #7064 ) ;
#25824=CARTESIAN_POINT ( 'NONE',  ( -21.56516322056021195, -8.616078523729070682, 73.79402879848014152 ) ) ;
#25827=B_SPLINE_CURVE_WITH_KNOTS ( 'NONE', 3,
 ( #28333, #2212, #27835, #36416, #39409, #20938, #28805, #2463, #43097, #39155 ),
 .UNSPECIFIED., .F., .F.,
 ( 4, 2, 2, 2, 4 ),
 ( 0.000000000000000000, 0.2500000000000000000, 0.5000000000000000000, 0.7500000000000000000, 1.000000000000000000 ),
 .UNSPECIFIED. ) ;
#25828=ADVANCED_FACE ( 'NONE', ( #3416 ), #34177, .T. ) ;
#25829=CARTESIAN_POINT ( 'NONE',  ( -11.41497376296057098, -19.21309731666858411, 71.80190493362104576 ) ) ;
#25830=ORIENTED_EDGE ( 'NONE', *, *, #31436, .T. ) ;
#25831=ORIENTED_EDGE ( 'NONE', *, *, #24296, .T. ) ;
#25832=EDGE_CURVE ( 'NONE', #12513, #20130, #37673, .T. ) ;
#25833=CARTESIAN_POINT ( 'NONE',  ( -22.84886394736722792, -9.702774549906752810, 73.59665770010028041 ) ) ;
#25834=CYLINDRICAL_SURFACE ( 'NONE', #28150, 0.1500000000000014932 ) ;
#25835=VECTOR ( 'NONE', #38906, 1000.000000000000000 ) ;
#25836=CARTESIAN_POINT ( 'NONE',  ( -10.42546210075913748, -12.25520342886974845, 57.44361899967025664 ) ) ;
#25838=EDGE_CURVE ( 'NONE', #20038, #21687, #236, .T. ) ;
#25839=CARTESIAN_POINT ( 'NONE',  ( -23.13305522301093120, -10.65917872773856878, 63.21619042434998903 ) ) ;
#25840=VECTOR ( 'NONE', #30110, 1000.000000000000000 ) ;
#25841=CARTESIAN_POINT ( 'NONE',  ( -19.23866243364646422, -21.62168334911581269, 58.52507384657483414 ) ) ;
#25842=CARTESIAN_POINT ( 'NONE',  ( -24.34442481654545176, -17.56831618823577301, 65.98711337262309939 ) ) ;
#25843=( BOUNDED_CURVE ( )  B_SPLINE_CURVE ( 3, ( #11993, #46692, #23565, #27003 ),
 .UNSPECIFIED., .F., .F. ) 
 B_SPLINE_CURVE_WITH_KNOTS ( ( 4, 4 ),
 ( 0.5000000000000000000, 0.9074455897393653991 ),
 .UNSPECIFIED. ) 
 CURVE ( )  GEOMETRIC_REPRESENTATION_ITEM ( )  RATIONAL_B_SPLINE_CURVE ( ( 0.9999999999999921174, 0.4567392136813264170, 0.3561768502900336530, 0.6983129098261052770 ) ) 
 REPRESENTATION_ITEM ( '' )  );
#25846=DIRECTION ( 'NONE',  ( 0.9132646967824439299, -0.4073666574609056124, 8.344532078871960245E-09 ) ) ;
#25848=CARTESIAN_POINT ( 'NONE',  ( -20.94465692579565896, -8.243430592510261334, 59.95629952546280350 ) ) ;
#25849=FACE_OUTER_BOUND ( 'NONE', #16928, .T. ) ;
#25852=VERTEX_POINT ( 'NONE', #710 ) ;
#25853=( BOUNDED_CURVE ( )  B_SPLINE_CURVE ( 3, ( #42170, #42419, #8689, #19509 ),
 .UNSPECIFIED., .F., .F. ) 
 B_SPLINE_CURVE_WITH_KNOTS ( ( 4, 4 ),
 ( 0.000000000000000000, 0.4074455897393610693 ),
 .UNSPECIFIED. ) 
 CURVE ( )  GEOMETRIC_REPRESENTATION_ITEM ( )  RATIONAL_B_SPLINE_CURVE ( ( 1.000000000000000000, 0.4567392136813320791, 0.3561768502900303779, 0.6983129098260949519 ) ) 
 REPRESENTATION_ITEM ( '' )  );
#25854=VERTEX_POINT ( 'NONE', #3659 ) ;
#25856=CARTESIAN_POINT ( 'NONE',  ( -10.42334078895570926, -15.64104556165006521, 61.18789045260545834 ) ) ;
#25857=CARTESIAN_POINT ( 'NONE',  ( -15.40060450416582860, -21.97927049188689708, 72.16762693854772692 ) ) ;
#25858=CARTESIAN_POINT ( 'NONE',  ( -11.85162103594838001, -10.49015045520576983, 71.25420998615621215 ) ) ;
#25859=ORIENTED_EDGE ( 'NONE', *, *, #15875, .T. ) ;
#25860=CARTESIAN_POINT ( 'NONE',  ( -24.49635653881819408, -12.46679777644911447, 73.35730153580948354 ) ) ;
#25861=CARTESIAN_POINT ( 'NONE',  ( -10.85887813628090015, -11.28619579020030628, 64.26226673522833721 ) ) ;
#25862=ORIENTED_EDGE ( 'NONE', *, *, #34274, .F. ) ;
#25863=CARTESIAN_POINT ( 'NONE',  ( -22.01912385291013408, -9.457520419221951968, 63.49153900988868315 ) ) ;
#25865=CARTESIAN_POINT ( 'NONE',  ( -23.06443888862362002, -10.57364818883473667, 63.16366193195977985 ) ) ;
#25867=CARTESIAN_POINT ( 'NONE',  ( -24.75383108144848165, -16.14659837148148824, 66.24980321609697853 ) ) ;
#25868=ADVANCED_FACE ( 'NONE', ( #41584 ), #15949, .T. ) ;
#25869=ORIENTED_EDGE ( 'NONE', *, *, #21730, .T. ) ;
#25870=CARTESIAN_POINT ( 'NONE',  ( -24.15708737698322395, -12.88964658164904620, 70.00072905108670795 ) ) ;
#25872=VECTOR ( 'NONE', #36466, 1000.000000000000114 ) ;
#25873=EDGE_LOOP ( 'NONE', ( #23085, #40584, #20678, #3963, #44282 ) ) ;
#25874=CARTESIAN_POINT ( 'NONE',  ( -22.47245519635065492, -19.73066437834766873, 72.65872596779033188 ) ) ;
#25875=CARTESIAN_POINT ( 'NONE',  ( -23.62594491300536959, -11.45603751788689451, 66.70742424642772050 ) ) ;
#25876=ORIENTED_EDGE ( 'NONE', *, *, #28302, .F. ) ;
#25877=DIRECTION ( 'NONE',  ( 0.7248509490090241369, -0.6889057277456160922, 1.880377065355303572E-09 ) ) ;
#25878=CARTESIAN_POINT ( 'NONE',  ( -10.29339667142563819, -12.65123896477911103, 64.52482037846105811 ) ) ;
#25882=CARTESIAN_POINT ( 'NONE',  ( -10.05964041407737497, -15.93577270795842615, 64.62958807307776965 ) ) ;
#25883=CARTESIAN_POINT ( 'NONE',  ( -24.43362369560107794, -14.05489154181400124, 73.27271507725298250 ) ) ;
#25884=CARTESIAN_POINT ( 'NONE',  ( -16.12334351384450670, -20.16700684834330914, 53.88362224778186516 ) ) ;
#25885=VERTEX_POINT ( 'NONE', #19667 ) ;
#25887=DIRECTION ( 'NONE',  ( -1.916827911674356108E-06, -6.156520247306097078E-06, 0.9999999999792114069 ) ) ;
#25889=CARTESIAN_POINT ( 'NONE',  ( -22.22619444978876757, -20.50513558618911958, 58.94938304221643222 ) ) ;
#25891=CARTESIAN_POINT ( 'NONE',  ( -17.05186597850482144, -7.819110227248425637, 70.59921951062938206 ) ) ;
#25893=VERTEX_POINT ( 'NONE', #38351 ) ;
#25894=EDGE_CURVE ( 'NONE', #4171, #28824, #47636, .T. ) ;
#25895=CARTESIAN_POINT ( 'NONE',  ( -23.75243126011088890, -11.69520888738364306, 66.83703234806088744 ) ) ;
#25896=CARTESIAN_POINT ( 'NONE',  ( -24.87290000513101873, -14.67112934921935974, 62.82801050733710468 ) ) ;
#25897=ORIENTED_EDGE ( 'NONE', *, *, #32376, .F. ) ;
#25898=CARTESIAN_POINT ( 'NONE',  ( -23.56005053104643210, -11.33143871826892912, 66.30725794404830253 ) ) ;
#25900=CARTESIAN_POINT ( 'NONE',  ( -11.36795091080559850, -18.31963851737709348, 58.10714594516144871 ) ) ;
#25901=CARTESIAN_POINT ( 'NONE',  ( -14.25068793291388047, -8.513811817964199946, 71.02957628655769895 ) ) ;
#25903=CARTESIAN_POINT ( 'NONE',  ( -10.54994933093899867, -13.24305344519376781, 71.49356453765415154 ) ) ;
#25904=FACE_BOUND ( 'NONE', #20937, .T. ) ;
#25906=CARTESIAN_POINT ( 'NONE',  ( -10.03450206504577125, -13.86240527909647824, 57.59825032318321547 ) ) ;
#25909=ORIENTED_EDGE ( 'NONE', *, *, #36773, .F. ) ;
#25910=FACE_OUTER_BOUND ( 'NONE', #21383, .T. ) ;
#25911=CARTESIAN_POINT ( 'NONE',  ( -10.66644504159021878, -12.78954850062448578, 68.15321152835137752 ) ) ;
#25913=CARTESIAN_POINT ( 'NONE',  ( -19.84060227527380249, -21.38033787448792467, 72.62034542409985249 ) ) ;
#25914=CARTESIAN_POINT ( 'NONE',  ( -24.29765713679916317, -13.47630389642528215, 59.47341129314763464 ) ) ;
#25917=CARTESIAN_POINT ( 'NONE',  ( -13.70502021987594077, -20.80197949353049580, 68.87113990053892110 ) ) ;
#25918=CARTESIAN_POINT ( 'NONE',  ( -23.42915847708036381, -11.11517115755410146, 73.64721174900437006 ) ) ;
#25919=EDGE_CURVE ( 'NONE', #37096, #16722, #18931, .T. ) ;
#25921=AXIS2_PLACEMENT_3D ( 'NONE', #40602, #40377, #14475 ) ;
#25923=EDGE_LOOP ( 'NONE', ( #11836, #29285, #21932, #27269, #47572 ) ) ;
#25925=ORIENTED_EDGE ( 'NONE', *, *, #4999, .F. ) ;
#25927=CARTESIAN_POINT ( 'NONE',  ( -18.59285626271963210, -7.848678033734123538, 67.05638626395584367 ) ) ;
#25929=B_SPLINE_CURVE_WITH_KNOTS ( 'NONE', 1,
 ( #31404, #5310 ),
 .UNSPECIFIED., .F., .F.,
 ( 2, 2 ),
 ( 0.000000000000000000, 1.000000000000000000 ),
 .UNSPECIFIED. ) ;
#25931=CARTESIAN_POINT ( 'NONE',  ( -16.13432406759100246, -21.74052631579560568, 58.30057715624173653 ) ) ;
#25933=CARTESIAN_POINT ( 'NONE',  ( -24.36668221452861971, -15.71384968925034364, 73.23133671100342212 ) ) ;
#25935=VERTEX_POINT ( 'NONE', #30520 ) ;
#25936=EDGE_CURVE ( 'NONE', #42966, #42781, #6478, .T. ) ;
#25937=CARTESIAN_POINT ( 'NONE',  ( -23.37999588001404661, -18.58199455739222827, 69.57899840282863124 ) ) ;
#25938=VERTEX_POINT ( 'NONE', #24582 ) ;
#25939=CARTESIAN_POINT ( 'NONE',  ( -10.82908108634309663, -17.30933488606310178, 68.51210539238705621 ) ) ;
#25940=CARTESIAN_POINT ( 'NONE',  ( -15.06268261486707338, -8.219072439155830523, 57.13383403554141893 ) ) ;
#25941=CARTESIAN_POINT ( 'NONE',  ( -9.982384861202168835, -14.45670355602896073, 67.96525964217694593 ) ) ;
#25942=VERTEX_POINT ( 'NONE', #20391 ) ;
#25944=CARTESIAN_POINT ( 'NONE',  ( -15.81235419205221504, -7.945607373518417837, 67.42535135806457447 ) ) ;
#25947=CARTESIAN_POINT ( 'NONE',  ( -22.11764131551248269, -20.59576654024708731, 58.95098234965121264 ) ) ;
#25949=DIRECTION ( 'NONE',  ( -0.8037372918934695409, 0.5949843406508663612, 7.322964617522835370E-08 ) ) ;
#25954=CARTESIAN_POINT ( 'NONE',  ( -18.34560609025200861, -9.386954687716537293, 54.07175714974878389 ) ) ;
#25956=EDGE_LOOP ( 'NONE', ( #38655, #9052 ) ) ;
#25958=CARTESIAN_POINT ( 'NONE',  ( -14.47983125967835960, -7.965589368325148634, 63.90483512601500848 ) ) ;
#25959=ORIENTED_EDGE ( 'NONE', *, *, #20845, .T. ) ;
#25960=CARTESIAN_POINT ( 'NONE',  ( -19.57699614054808634, -21.94144247634149281, 62.17999043330664222 ) ) ;
#25961=VECTOR ( 'NONE', #14785, 1000.000000000000000 ) ;
#25962=CARTESIAN_POINT ( 'NONE',  ( -15.36368464484735874, -8.119310132577721717, 74.27088789173198791 ) ) ;
#25963=CARTESIAN_POINT ( 'NONE',  ( -11.74167521261877134, -9.991000739040469369, 67.66043377903119449 ) ) ;
#25964=ORIENTED_EDGE ( 'NONE', *, *, #16620, .F. ) ;
#25965=CARTESIAN_POINT ( 'NONE',  ( -10.04946558025865500, -15.86660702602552320, 64.70109908442724134 ) ) ;
#25966=ADVANCED_FACE ( 'NONE', ( #46251 ), #26580, .T. ) ;
#25967=CARTESIAN_POINT ( 'NONE',  ( -14.62089650835144816, -21.71189251387697894, 58.30471404203333918 ) ) ;
#25968=ORIENTED_EDGE ( 'NONE', *, *, #38034, .F. ) ;
#25969=ORIENTED_EDGE ( 'NONE', *, *, #5934, .T. ) ;
#25971=EDGE_CURVE ( 'NONE', #1137, #39506, #36332, .T. ) ;
#25973=LINE ( 'NONE', #7273, #37388 ) ;
#25974=CARTESIAN_POINT ( 'NONE',  ( -14.08295856548867597, -8.150414966537949724, 70.82983378092882276 ) ) ;
#25975=CARTESIAN_POINT ( 'NONE',  ( -23.12302657392458016, -18.95946740514217765, 62.35406880581413702 ) ) ;
#25976=ORIENTED_EDGE ( 'NONE', *, *, #28663, .F. ) ;
#25977=VERTEX_POINT ( 'NONE', #38853 ) ;
#25980=CARTESIAN_POINT ( 'NONE',  ( -10.83536388074712598, -17.31742051234312640, 64.92739380450886699 ) ) ;
#25982=VECTOR ( 'NONE', #32306, 1000.000000000000114 ) ;
#25983=( BOUNDED_CURVE ( )  B_SPLINE_CURVE ( 3, ( #9181, #28846, #1535, #39454 ),
 .UNSPECIFIED., .F., .F. ) 
 B_SPLINE_CURVE_WITH_KNOTS ( ( 4, 4 ),
 ( 0.9074455897393670645, 1.000000000000000000 ),
 .UNSPECIFIED. ) 
 CURVE ( )  GEOMETRIC_REPRESENTATION_ITEM ( )  RATIONAL_B_SPLINE_CURVE ( ( 0.6983129098260929535, 0.7760317562606982023, 0.8765941196520005141, 1.000000000000000000 ) ) 
 REPRESENTATION_ITEM ( '' )  );
#25985=EDGE_CURVE ( 'NONE', #24088, #15624, #17, .T. ) ;
#25989=EDGE_CURVE ( 'NONE', #25893, #9814, #32867, .T. ) ;
#25990=ADVANCED_FACE ( 'NONE', ( #42570 ), #33164, .T. ) ;
#25991=CYLINDRICAL_SURFACE ( 'NONE', #29331, 0.1500000000000060729 ) ;
#25992=CARTESIAN_POINT ( 'NONE',  ( -22.37985683132060188, -19.82347751554591397, 69.47417989525710880 ) ) ;
#25994=CYLINDRICAL_SURFACE ( 'NONE', #22585, 0.1500000000000050182 ) ;
#25997=( BOUNDED_CURVE ( )  B_SPLINE_CURVE ( 3, ( #22644, #41109, #7394, #3938 ),
 .UNSPECIFIED., .F., .F. ) 
 B_SPLINE_CURVE_WITH_KNOTS ( ( 4, 4 ),
 ( 0.9074455897393646220, 1.000000000000000000 ),
 .UNSPECIFIED. ) 
 CURVE ( )  GEOMETRIC_REPRESENTATION_ITEM ( )  RATIONAL_B_SPLINE_CURVE ( ( 0.6983129098260778544, 0.7760317562606851016, 0.8765941196519925205, 1.000000000000000000 ) ) 
 REPRESENTATION_ITEM ( '' )  );
#25999=FACE_OUTER_BOUND ( 'NONE', #41072, .T. ) ;
#26001=CARTESIAN_POINT ( 'NONE',  ( -9.995738443926455830, -14.24059931954510816, 64.50308448303212572 ) ) ;
#26002=CIRCLE ( 'NONE', #44121, 5.500000000000000000 ) ;
#26003=VERTEX_POINT ( 'NONE', #14647 ) ;
#26005=LINE ( 'NONE', #18348, #39938 ) ;
#26006=FACE_OUTER_BOUND ( 'NONE', #48463, .T. ) ;
#26007=DIRECTION ( 'NONE',  ( 0.5562740912439652075, 0.8309988781043535777, 7.851267780903551505E-08 ) ) ;
#26008=ORIENTED_EDGE ( 'NONE', *, *, #31173, .T. ) ;
#26009=CARTESIAN_POINT ( 'NONE',  ( -15.69736356130078647, -8.025520047610617880, 70.90989840317035942 ) ) ;
#26010=CARTESIAN_POINT ( 'NONE',  ( -12.57223699000811656, -19.85511602558925048, 65.16674893742153074 ) ) ;
#26011=VERTEX_POINT ( 'NONE', #29467 ) ;
#26012=FACE_BOUND ( 'NONE', #32532, .T. ) ;
#26014=FACE_OUTER_BOUND ( 'NONE', #12846, .T. ) ;
#26015=LINE ( 'NONE', #3106, #36507 ) ;
#26016=ADVANCED_FACE ( 'NONE', ( #21116 ), #25769, .T. ) ;
#26017=CARTESIAN_POINT ( 'NONE',  ( -24.42002265954547724, -14.56875473297011681, 62.72798972149294627 ) ) ;
#26018=AXIS2_PLACEMENT_3D ( 'NONE', #47151, #2327, #24751 ) ;
#26019=CARTESIAN_POINT ( 'NONE',  ( -21.61680475328812889, -8.650891705389904374, 73.85774703147257014 ) ) ;
#26020=VERTEX_POINT ( 'NONE', #13932 ) ;
#26021=CARTESIAN_POINT ( 'NONE',  ( -10.14660727810982976, -16.40665786317032371, 71.56094979796495181 ) ) ;
#26024=LINE ( 'NONE', #41043, #39268 ) ;
#26025=ORIENTED_EDGE ( 'NONE', *, *, #46345, .F. ) ;
#26028=CARTESIAN_POINT ( 'NONE',  ( -18.32857646159318676, -22.20418385865972155, 68.93019298464047040 ) ) ;
#26029=ADVANCED_FACE ( 'NONE', ( #47463 ), #40788, .F. ) ;
#26030=ORIENTED_EDGE ( 'NONE', *, *, #46365, .T. ) ;
#26031=ORIENTED_EDGE ( 'NONE', *, *, #8199, .F. ) ;
#26033=CARTESIAN_POINT ( 'NONE',  ( -22.24952096526922318, -19.88199321984651391, 69.40247773061638270 ) ) ;
#26035=CARTESIAN_POINT ( 'NONE',  ( -12.56051219783612538, -20.45271961000943861, 71.85007761110178137 ) ) ;
#26036=CARTESIAN_POINT ( 'NONE',  ( -10.04087064144442110, -13.81269952487260078, 57.58791698818001947 ) ) ;
#26037=CARTESIAN_POINT ( 'NONE',  ( -11.55573786329523855, -10.21941616939416342, 71.15388509157428132 ) ) ;
#26041=EDGE_LOOP ( 'NONE', ( #12750, #36896 ) ) ;
#26042=CARTESIAN_POINT ( 'NONE',  ( -15.93106588071581697, -7.910958181831522218, 60.35595345230024833 ) ) ;
#26045=CARTESIAN_POINT ( 'NONE',  ( -14.95256263785226203, -21.41194290305684333, 61.93040681845756268 ) ) ;
#26046=DIRECTION ( 'NONE',  ( -5.731567514496413899E-31, -1.020425574103664789E-16, -1.000000000000000000 ) ) ;
#26050=ORIENTED_EDGE ( 'NONE', *, *, #16635, .F. ) ;
#26051=VECTOR ( 'NONE', #45687, 1000.000000000000000 ) ;
#26052=EDGE_CURVE ( 'NONE', #12496, #29452, #18356, .T. ) ;
#26055=CARTESIAN_POINT ( 'NONE',  ( -11.86614749421525339, -19.77135288044581429, 58.11337654531251218 ) ) ;
#26058=ORIENTED_EDGE ( 'NONE', *, *, #42506, .F. ) ;
#26060=AXIS2_PLACEMENT_3D ( 'NONE', #11958, #19088, #37536 ) ;
#26061=EDGE_CURVE ( 'NONE', #6771, #8867, #11183, .T. ) ;
#26063=CARTESIAN_POINT ( 'NONE',  ( -14.98927377128279304, -8.246306944878790901, 75.49999999999994316 ) ) ;
#26065=EDGE_LOOP ( 'NONE', ( #32182, #4628 ) ) ;
#26068=CARTESIAN_POINT ( 'NONE',  ( -21.89130958583942288, -9.354787850460871468, 63.20625856529903075 ) ) ;
#26070=CARTESIAN_POINT ( 'NONE',  ( -24.68120957711303731, -16.49402054639926263, 59.30145216245190909 ) ) ;
#26071=VERTEX_POINT ( 'NONE', #29711 ) ;
#26072=CARTESIAN_POINT ( 'NONE',  ( -10.16749015965427105, -13.12235144340169235, 71.39323866028058774 ) ) ;
#26073=CARTESIAN_POINT ( 'NONE',  ( -24.30574759568347787, -16.34084296935221303, 59.42332403323545265 ) ) ;
#26076=EDGE_CURVE ( 'NONE', #6043, #3502, #36613, .T. ) ;
#26077=CARTESIAN_POINT ( 'NONE',  ( -16.32575768948312600, -7.844986739114469643, 60.21500614002425777 ) ) ;
#26079=DIRECTION ( 'NONE',  ( -0.3478314405900309048, -0.9375570856950864451, 0.000000000000000000 ) ) ;
#26080=( BOUNDED_CURVE ( )  B_SPLINE_CURVE ( 3, ( #20768, #46201, #36257, #42269 ),
 .UNSPECIFIED., .F., .F. ) 
 B_SPLINE_CURVE_WITH_KNOTS ( ( 4, 4 ),
 ( 0.000000000000000000, 0.4074455897393662318 ),
 .UNSPECIFIED. ) 
 CURVE ( )  GEOMETRIC_REPRESENTATION_ITEM ( )  RATIONAL_B_SPLINE_CURVE ( ( 1.000000000000000000, 0.4567392136813269721, 0.3561768502900284350, 0.6983129098261046108 ) ) 
 REPRESENTATION_ITEM ( '' )  );
#26085=CARTESIAN_POINT ( 'NONE',  ( -23.29491342820895028, -19.39590518005356756, 59.06223412631987912 ) ) ;
#26086=AXIS2_PLACEMENT_3D ( 'NONE', #44780, #6845, #45265 ) ;
#26087=CARTESIAN_POINT ( 'NONE',  ( -24.38556453292044424, -15.94620486698431350, 62.59328380657402846 ) ) ;
#26088=ORIENTED_EDGE ( 'NONE', *, *, #18256, .F. ) ;
#26091=CYLINDRICAL_SURFACE ( 'NONE', #12563, 0.1500000000000061562 ) ;
#26094=CARTESIAN_POINT ( 'NONE',  ( -23.83724620116612058, -11.87385095858915207, 63.36706934938042934 ) ) ;
#26095=CARTESIAN_POINT ( 'NONE',  ( -24.11138715268779364, -17.05307659639229101, 69.41339812867973080 ) ) ;
#26096=CARTESIAN_POINT ( 'NONE',  ( -16.96792471375929523, -7.373175173468426102, 74.05994646750021104 ) ) ;
#26099=CARTESIAN_POINT ( 'NONE',  ( -22.89146017634119090, -10.34570183799575105, 70.15611359559922278 ) ) ;
#26100=VECTOR ( 'NONE', #37725, 1000.000000000000114 ) ;
#26101=CARTESIAN_POINT ( 'NONE',  ( -14.98249323814573941, -9.880861343182303358, 53.49899999999994549 ) ) ;
#26102=CARTESIAN_POINT ( 'NONE',  ( -16.52634554021970104, -22.20493084912042292, 65.32590148269446217 ) ) ;
#26104=ORIENTED_EDGE ( 'NONE', *, *, #6688, .F. ) ;
#26107=CARTESIAN_POINT ( 'NONE',  ( -10.62264718916325279, -13.15334866428350047, 71.20828630685304006 ) ) ;
#26108=FACE_OUTER_BOUND ( 'NONE', #14200, .T. ) ;
#26109=CARTESIAN_POINT ( 'NONE',  ( -13.82494607736302683, -21.33227806808298865, 72.10420475123025597 ) ) ;
#26111=LINE ( 'NONE', #7406, #36856 ) ;
#26112=EDGE_CURVE ( 'NONE', #14380, #21441, #19372, .T. ) ;
#26113=EDGE_CURVE ( 'NONE', #42055, #30264, #19991, .T. ) ;
#26114=DIRECTION ( 'NONE',  ( -0.3126464228004096069, -0.3197690014840522399, 0.8944271909999157444 ) ) ;
#26115=ORIENTED_EDGE ( 'NONE', *, *, #23970, .T. ) ;
#26116=ADVANCED_FACE ( 'NONE', ( #26759 ), #4872, .T. ) ;
#26117=CIRCLE ( 'NONE', #41062, 2.499999999999999556 ) ;
#26120=( BOUNDED_CURVE ( )  B_SPLINE_CURVE ( 3, ( #41786, #10758, #25780, #4127 ),
 .UNSPECIFIED., .F., .F. ) 
 B_SPLINE_CURVE_WITH_KNOTS ( ( 4, 4 ),
 ( 0.5000000000000000000, 0.9074455897393678416 ),
 .UNSPECIFIED. ) 
 CURVE ( )  GEOMETRIC_REPRESENTATION_ITEM ( )  RATIONAL_B_SPLINE_CURVE ( ( 1.000000000000018430, 0.4567392136813228642, 0.3561768502900140021, 0.6983129098261117162 ) ) 
 REPRESENTATION_ITEM ( '' )  );
#26121=CARTESIAN_POINT ( 'NONE',  ( -21.94239013569476171, -20.22099906679998327, 58.76442899523448204 ) ) ;
#26124=ORIENTED_EDGE ( 'NONE', *, *, #6694, .F. ) ;
#26125=DIRECTION ( 'NONE',  ( 1.140458104654002173E-06, 1.256740833599404314E-06, -0.9999999999985599297 ) ) ;
#26126=LINE ( 'NONE', #21222, #28167 ) ;
#26128=CARTESIAN_POINT ( 'NONE',  ( -16.36339736119901289, -21.78261100941413986, 65.31744608471964852 ) ) ;
#26129=FACE_OUTER_BOUND ( 'NONE', #2035, .T. ) ;
#26132=CARTESIAN_POINT ( 'NONE',  ( -17.68496328886486424, -21.80445416477857279, 58.70553376440283699 ) ) ;
#26133=CARTESIAN_POINT ( 'NONE',  ( -24.86242989439883289, -14.39095395922188558, 66.36788051138485400 ) ) ;
#26135=CARTESIAN_POINT ( 'NONE',  ( -10.23610968374255314, -12.85046669463587143, 67.85336945107273721 ) ) ;
#26136=ORIENTED_EDGE ( 'NONE', *, *, #19866, .F. ) ;
#26137=( BOUNDED_SURFACE ( )  B_SPLINE_SURFACE ( 3, 1, ( 
 ( #20525, #32083 ),
 ( #6223, #12874 ),
 ( #2038, #27901 ),
 ( #42926, #43665 ),
 ( #24216, #5507 ),
 ( #1802, #28145 ),
 ( #5754, #35756 ) ),
 .UNSPECIFIED., .T., .F., .F. ) 
 B_SPLINE_SURFACE_WITH_KNOTS ( ( 4, 3, 4 ),
 ( 2, 2 ),
 ( 0.000000000000000000, 0.5000000000000000000, 1.000000000000000000 ),
 ( 0.000000000000000000, 1.000000000000000000 ),
 .UNSPECIFIED. ) 
 GEOMETRIC_REPRESENTATION_ITEM ( )  RATIONAL_B_SPLINE_SURFACE ( (
 ( 1.000000000000000000, 1.000000000000000000),
 ( 0.3333333333333335369, 0.3333333333333330373),
 ( 0.3333333333333335369, 0.3333333333333330373),
 ( 1.000000000000000000, 1.000000000000000000),
 ( 0.3333333333333333703, 0.3333333333333333703),
 ( 0.3333333333333333703, 0.3333333333333333703),
 ( 1.000000000000000000, 1.000000000000000000) ) ) 
 REPRESENTATION_ITEM ( '' )  SURFACE ( )  );
#26138=CARTESIAN_POINT ( 'NONE',  ( -16.98230468507255253, -22.24614900656091621, 72.35817375816297670 ) ) ;
#26140=CARTESIAN_POINT ( 'NONE',  ( -13.18473975798692877, -20.93551490194142062, 58.23145353898504339 ) ) ;
#26142=CARTESIAN_POINT ( 'NONE',  ( -17.42409385541300892, -14.80920654474439679, 47.99999999999994316 ) ) ;
#26143=CARTESIAN_POINT ( 'NONE',  ( -17.20139284005516700, -7.812749994621428051, 70.79035839633094440 ) ) ;
#26145=EDGE_LOOP ( 'NONE', ( #6289, #48315, #4386, #40016, #33363 ) ) ;
#26146=CARTESIAN_POINT ( 'NONE',  ( -23.62594491300536959, -11.45603751788689095, 66.70742424642772050 ) ) ;
#26147=CARTESIAN_POINT ( 'NONE',  ( -21.57946453887431204, -8.565578233975859490, 53.49999999999994316 ) ) ;
#26149=CARTESIAN_POINT ( 'NONE',  ( -15.33646109947928338, -7.657507462184680591, 74.24018999459609347 ) ) ;
#26150=CARTESIAN_POINT ( 'NONE',  ( -24.00746416177546294, -17.19188300715374140, 72.95506251513478446 ) ) ;
#26152=CARTESIAN_POINT ( 'NONE',  ( -11.82099749022622426, -9.899105802180386604, 64.21409645106085406 ) ) ;
#26153=CARTESIAN_POINT ( 'NONE',  ( -24.74223048688043747, -16.20536452925702520, 62.77045531336093376 ) ) ;
#26154=CARTESIAN_POINT ( 'NONE',  ( -24.32886716615087153, -16.23426984194678724, 62.60800820172418923 ) ) ;
#26155=CARTESIAN_POINT ( 'NONE',  ( -19.51575165005438706, -21.95960923578041957, 62.10229500050338203 ) ) ;
#26156=CARTESIAN_POINT ( 'NONE',  ( -22.53429316287767392, -9.952421288698296564, 73.63161091678163928 ) ) ;
#26157=( BOUNDED_CURVE ( )  B_SPLINE_CURVE ( 3, ( #19622, #15912, #37340, #34632 ),
 .UNSPECIFIED., .F., .F. ) 
 B_SPLINE_CURVE_WITH_KNOTS ( ( 4, 4 ),
 ( 0.9074455897393781667, 1.000000000000000000 ),
 .UNSPECIFIED. ) 
 CURVE ( )  GEOMETRIC_REPRESENTATION_ITEM ( )  RATIONAL_B_SPLINE_CURVE ( ( 0.6983129098261450229, 0.7760317562607430553, 0.8765941196520280476, 1.000000000000000000 ) ) 
 REPRESENTATION_ITEM ( '' )  );
#26158=CARTESIAN_POINT ( 'NONE',  ( -16.26195973558533581, -21.76306465430365122, 58.57113428431811997 ) ) ;
#26159=CARTESIAN_POINT ( 'NONE',  ( -18.77402089607887348, -7.482479170000134516, 70.47729698164395984 ) ) ;
#26160=ORIENTED_EDGE ( 'NONE', *, *, #23198, .F. ) ;
#26161=CARTESIAN_POINT ( 'NONE',  ( -24.08907074505709645, -11.48026357735065872, 63.13713704106291402 ) ) ;
#26162=CARTESIAN_POINT ( 'NONE',  ( -12.81450749931373423, -9.474957484202729319, 74.31923006089488126 ) ) ;
#26165=CARTESIAN_POINT ( 'NONE',  ( -24.29423998123223782, -13.46050165329320336, 59.59097898989885067 ) ) ;
#26166=CARTESIAN_POINT ( 'NONE',  ( -24.63461978062257174, -12.93251252767717929, 66.48902111634848211 ) ) ;
#26168=CARTESIAN_POINT ( 'NONE',  ( -11.60526899143904345, -18.79015832504765626, 68.23161775275829655 ) ) ;
#26171=VERTEX_POINT ( 'NONE', #29964 ) ;
#26173=VERTEX_POINT ( 'NONE', #26507 ) ;
#26175=CARTESIAN_POINT ( 'NONE',  ( -16.32575768948312600, -7.844986739114469643, 60.21500614002425777 ) ) ;
#26176=CARTESIAN_POINT ( 'NONE',  ( -10.03016176022630646, -13.89628074529801438, 57.49179087295118507 ) ) ;
#26178=B_SPLINE_CURVE_WITH_KNOTS ( 'NONE', 1,
 ( #4179, #3930 ),
 .UNSPECIFIED., .F., .F.,
 ( 2, 2 ),
 ( 0.000000000000000000, 1.000000000000000000 ),
 .UNSPECIFIED. ) ;
#26179=EDGE_CURVE ( 'NONE', #6465, #33214, #37824, .T. ) ;
#26180=CARTESIAN_POINT ( 'NONE',  ( -13.47245494993759607, -21.12492725511472003, 65.10133600691351319 ) ) ;
#26181=CARTESIAN_POINT ( 'NONE',  ( -19.61601425152793254, -21.50980239257335569, 65.61486213821591207 ) ) ;
#26184=CARTESIAN_POINT ( 'NONE',  ( -22.38400322090610217, -20.36826016184844335, 62.41934579407823236 ) ) ;
#26185=CARTESIAN_POINT ( 'NONE',  ( -23.93808066934879619, -17.37550490234871248, 69.64169580580271202 ) ) ;
#26186=ORIENTED_EDGE ( 'NONE', *, *, #15531, .F. ) ;
#26188=FACE_OUTER_BOUND ( 'NONE', #3714, .T. ) ;
#26189=CARTESIAN_POINT ( 'NONE',  ( -19.86401518824997581, -21.42384811948916479, 69.22010401872219632 ) ) ;
#26190=CARTESIAN_POINT ( 'NONE',  ( -22.91943239076679006, -10.38811108791941429, 59.48714571049892896 ) ) ;
#26191=VERTEX_POINT ( 'NONE', #11735 ) ;
#26192=CARTESIAN_POINT ( 'NONE',  ( -11.05034076241727625, -11.79557573020262318, 71.37388789199357575 ) ) ;
#26194=EDGE_CURVE ( 'NONE', #1223, #17754, #18215, .T. ) ;
#26195=CARTESIAN_POINT ( 'NONE',  ( -10.31364510401727053, -17.03300888149450998, 57.80265138661536639 ) ) ;
#26196=CARTESIAN_POINT ( 'NONE',  ( -9.982716954774490503, -14.44908413001617298, 67.97304700561097945 ) ) ;
#26197=VERTEX_POINT ( 'NONE', #38979 ) ;
#26198=CARTESIAN_POINT ( 'NONE',  ( -9.981610056738364989, -14.47448034074775336, 68.05811324665165785 ) ) ;
#26199=CARTESIAN_POINT ( 'NONE',  ( -9.975093145215874202, -14.93635225021824198, 74.98274299234972773 ) ) ;
#26200=CARTESIAN_POINT ( 'NONE',  ( -16.61483489837897309, -21.81624168220134052, 61.96387868409816946 ) ) ;
#26202=ORIENTED_EDGE ( 'NONE', *, *, #32128, .T. ) ;
#26203=CARTESIAN_POINT ( 'NONE',  ( -17.69364751199190522, -22.25449563392884400, 58.56699864565176483 ) ) ;
#26206=CARTESIAN_POINT ( 'NONE',  ( -18.39063358449543983, -7.876195807596681142, 73.91352353256114327 ) ) ;
#26207=CARTESIAN_POINT ( 'NONE',  ( -24.55871722839809834, -12.66422925090921225, 69.88747596251579353 ) ) ;
#26208=FACE_OUTER_BOUND ( 'NONE', #34023, .T. ) ;
#26209=EDGE_LOOP ( 'NONE', ( #43701, #45598, #44046, #41936, #3217 ) ) ;
#26210=DIRECTION ( 'NONE',  ( -0.9629498065864428025, -0.2696806815386155742, -3.246020392366887627E-17 ) ) ;
#26212=ORIENTED_EDGE ( 'NONE', *, *, #7788, .T. ) ;
#26213=AXIS2_PLACEMENT_3D ( 'NONE', #23777, #26482, #38530 ) ;
#26215=CARTESIAN_POINT ( 'NONE',  ( -10.96024275427387984, -11.10349598290784989, 60.79230391164892211 ) ) ;
#26217=EDGE_CURVE ( 'NONE', #12496, #46961, #26024, .T. ) ;
#26218=CARTESIAN_POINT ( 'NONE',  ( -24.85472652781555070, -14.27003188481730689, 69.79241900681766708 ) ) ;
#26219=CARTESIAN_POINT ( 'NONE',  ( -15.50784526261009511, -8.076599967007890513, 74.37985659287807039 ) ) ;
#26220=ORIENTED_EDGE ( 'NONE', *, *, #29490, .T. ) ;
#26223=CARTESIAN_POINT ( 'NONE',  ( -10.45134696456191392, -14.19143820756648644, 60.93323705330102058 ) ) ;
#26226=VERTEX_POINT ( 'NONE', #22324 ) ;
#26227=CARTESIAN_POINT ( 'NONE',  ( -24.80769062643263467, -15.80232089486973557, 69.71802876059763321 ) ) ;
#26229=CARTESIAN_POINT ( 'NONE',  ( -18.86946249347487381, -7.959927237300316705, 67.20071732990344060 ) ) ;
#26230=CARTESIAN_POINT ( 'NONE',  ( -24.77723895724858494, -16.00713575449774595, 66.24820309305337673 ) ) ;
#26231=ORIENTED_EDGE ( 'NONE', *, *, #8686, .F. ) ;
#26232=CARTESIAN_POINT ( 'NONE',  ( -12.32278866559117780, -19.67576434477648917, 61.41150688479135766 ) ) ;
#26233=ORIENTED_EDGE ( 'NONE', *, *, #36867, .F. ) ;
#26234=EDGE_CURVE ( 'NONE', #20100, #8067, #24089, .T. ) ;
#26235=CARTESIAN_POINT ( 'NONE',  ( -10.38752013045322009, -14.36951432065623813, 64.67331771650336236 ) ) ;
#26236=CARTESIAN_POINT ( 'NONE',  ( -19.60046948880987117, -21.46228020301366257, 65.76486213989072382 ) ) ;
#26238=CARTESIAN_POINT ( 'NONE',  ( -21.52687325878983415, -21.02790335591837589, 72.68592979288212064 ) ) ;
#26240=VERTEX_POINT ( 'NONE', #24704 ) ;
#26241=CARTESIAN_POINT ( 'NONE',  ( -17.85728874018075985, -21.84618329174708151, 61.89007996730683203 ) ) ;
#26243=CYLINDRICAL_SURFACE ( 'NONE', #4622, 0.1499999999999999667 ) ;
#26245=ORIENTED_EDGE ( 'NONE', *, *, #17013, .T. ) ;
#26247=CARTESIAN_POINT ( 'NONE',  ( -21.80947398209100285, -9.353160252369512762, 63.49153755919518005 ) ) ;
#26249=FACE_BOUND ( 'NONE', #15355, .T. ) ;
#26250=ORIENTED_EDGE ( 'NONE', *, *, #7513, .F. ) ;
#26251=CARTESIAN_POINT ( 'NONE',  ( -13.11436666535386664, -20.88631628731643630, 58.18616748667333383 ) ) ;
#26253=CARTESIAN_POINT ( 'NONE',  ( -19.24025795797341942, -7.996846695050864540, 60.24620885950562865 ) ) ;
#26254=DIRECTION ( 'NONE',  ( -0.9968684284758858594, 0.07907803935364896009, -1.831731158650941667E-08 ) ) ;
#26255=VERTEX_POINT ( 'NONE', #21245 ) ;
#26256=CARTESIAN_POINT ( 'NONE',  ( -10.11824992584547545, -16.26811798947522192, 71.56255103782838489 ) ) ;
#26258=CARTESIAN_POINT ( 'NONE',  ( -12.67990993908946429, -9.064901105426571348, 70.97112579386727305 ) ) ;
#26260=CARTESIAN_POINT ( 'NONE',  ( -14.41428275390769365, -7.994163218335415877, 63.97474169571218283 ) ) ;
#26262=EDGE_LOOP ( 'NONE', ( #2994, #6176 ) ) ;
#26263=CARTESIAN_POINT ( 'NONE',  ( -16.16379449968008331, -22.15191876840708929, 58.47080954035841671 ) ) ;
#26264=EDGE_CURVE ( 'NONE', #26764, #30116, #5974, .T. ) ;
#26265=CARTESIAN_POINT ( 'NONE',  ( -10.95381480682210373, -17.48044017699314523, 68.09721944380058289 ) ) ;
#26267=ADVANCED_FACE ( 'NONE', ( #20523 ), #24933, .T. ) ;
#26270=CARTESIAN_POINT ( 'NONE',  ( -15.25801600794807555, -21.93814553200309092, 72.23230793488828283 ) ) ;
#26271=DIRECTION ( 'NONE',  ( 1.027096116490394736E-05, 2.598167872976484874E-06, 0.9999999999438784481 ) ) ;
#26272=CARTESIAN_POINT ( 'NONE',  ( -19.31443854130040449, -22.01544605587237768, 58.63233246516547581 ) ) ;
#26273=CARTESIAN_POINT ( 'NONE',  ( -10.59838470211619565, -13.25112858161469021, 74.74987944841035414 ) ) ;
#26274=( BOUNDED_SURFACE ( )  B_SPLINE_SURFACE ( 3, 1, ( 
 ( #9727, #17804 ),
 ( #24747, #36289 ),
 ( #2571, #40712 ),
 ( #32604, #6987 ),
 ( #39749, #33063 ),
 ( #25460, #13861 ),
 ( #40470, #6748 ) ),
 .UNSPECIFIED., .T., .F., .F. ) 
 B_SPLINE_SURFACE_WITH_KNOTS ( ( 4, 3, 4 ),
 ( 2, 2 ),
 ( 0.000000000000000000, 0.5000000000000000000, 1.000000000000000000 ),
 ( 0.000000000000000000, 1.000000000000000000 ),
 .UNSPECIFIED. ) 
 GEOMETRIC_REPRESENTATION_ITEM ( )  RATIONAL_B_SPLINE_SURFACE ( (
 ( 1.000000000000000000, 1.000000000000000000),
 ( 0.3333333333333335369, 0.3333333333333330373),
 ( 0.3333333333333335369, 0.3333333333333330373),
 ( 1.000000000000000000, 1.000000000000000000),
 ( 0.3333333333333333703, 0.3333333333333333703),
 ( 0.3333333333333333703, 0.3333333333333333703),
 ( 1.000000000000000000, 1.000000000000000000) ) ) 
 REPRESENTATION_ITEM ( '' )  SURFACE ( )  );
#26275=CARTESIAN_POINT ( 'NONE',  ( -24.13143191548659416, -12.80630458298108110, 66.41132680564976454 ) ) ;
#26278=ORIENTED_EDGE ( 'NONE', *, *, #9613, .F. ) ;
#26279=ORIENTED_EDGE ( 'NONE', *, *, #23820, .F. ) ;
#26281=CARTESIAN_POINT ( 'NONE',  ( -12.18170072908086965, -10.17053062278287889, 64.32914326641392222 ) ) ;
#26283=CARTESIAN_POINT ( 'NONE',  ( -10.97897535230521449, -21.25982559335476552, 54.49999999999995026 ) ) ;
#26284=CARTESIAN_POINT ( 'NONE',  ( -21.87050360319829778, -9.402213735156793817, 63.20770402078916561 ) ) ;
#26285=CARTESIAN_POINT ( 'NONE',  ( -18.55203529891204539, -7.444959873133314865, 74.01781259684146619 ) ) ;
#26286=EDGE_LOOP ( 'NONE', ( #38397, #13412, #25109, #27759 ) ) ;
#26288=( BOUNDED_CURVE ( )  B_SPLINE_CURVE ( 3, ( #34943, #43068, #27322, #20175 ),
 .UNSPECIFIED., .F., .F. ) 
 B_SPLINE_CURVE_WITH_KNOTS ( ( 4, 4 ),
 ( 0.9074455897393710613, 1.000000000000000000 ),
 .UNSPECIFIED. ) 
 CURVE ( )  GEOMETRIC_REPRESENTATION_ITEM ( )  RATIONAL_B_SPLINE_CURVE ( ( 0.6983129098261089407, 0.7760317562607119690, 0.8765941196520089518, 1.000000000000000000 ) ) 
 REPRESENTATION_ITEM ( '' )  );
#26289=EDGE_LOOP ( 'NONE', ( #47373, #33629 ) ) ;
#26292=CARTESIAN_POINT ( 'NONE',  ( -10.02995829593802668, -13.89786868041111667, 57.63320316755233819 ) ) ;
#26293=ORIENTED_EDGE ( 'NONE', *, *, #6660, .F. ) ;
#26295=EDGE_CURVE ( 'NONE', #29883, #10137, #6470, .T. ) ;
#26296=CARTESIAN_POINT ( 'NONE',  ( -24.17913852840423417, -12.79079990135933897, 69.77802802196565324 ) ) ;
#26298=VERTEX_POINT ( 'NONE', #46861 ) ;
#26299=DIRECTION ( 'NONE',  ( -5.468526094916624094E-08, -8.832527036150760808E-06, 0.9999999999609917589 ) ) ;
#26300=CARTESIAN_POINT ( 'NONE',  ( -10.13399043377362929, -16.34501826020601811, 71.56937588126346839 ) ) ;
#26301=CARTESIAN_POINT ( 'NONE',  ( -24.37121093718953446, -17.50201705633955740, 66.05701994492248730 ) ) ;
#26302=VERTEX_POINT ( 'NONE', #16800 ) ;
#26303=CARTESIAN_POINT ( 'NONE',  ( -11.18894271684748887, -11.62402355859291170, 71.27787913046262247 ) ) ;
#26305=AXIS2_PLACEMENT_3D ( 'NONE', #18887, #36842, #48429 ) ;
#26306=CARTESIAN_POINT ( 'NONE',  ( -10.30929367908409766, -17.01932638214790927, 57.82727192363577018 ) ) ;
#26309=FACE_OUTER_BOUND ( 'NONE', #23302, .T. ) ;
#26310=VECTOR ( 'NONE', #40540, 1000.000000000000114 ) ;
#26311=CARTESIAN_POINT ( 'NONE',  ( -18.55725912610375516, -22.17253639328876602, 72.38536699639935534 ) ) ;
#26312=ORIENTED_EDGE ( 'NONE', *, *, #42506, .T. ) ;
#26313=CARTESIAN_POINT ( 'NONE',  ( -22.09944621541271914, -9.008888719317940996, 63.39164957891247099 ) ) ;
#26314=CARTESIAN_POINT ( 'NONE',  ( -22.30100230481251344, -19.83081991958632884, 65.77709836140900279 ) ) ;
#26315=CARTESIAN_POINT ( 'NONE',  ( -11.99471263755300576, -9.707784190782769329, 60.65943832103737776 ) ) ;
#26316=ORIENTED_EDGE ( 'NONE', *, *, #28234, .F. ) ;
#26317=CARTESIAN_POINT ( 'NONE',  ( -17.36015840614627592, -7.359395087992972151, 67.20535029649403214 ) ) ;
#26318=EDGE_CURVE ( 'NONE', #41394, #33214, #47014, .T. ) ;
#26319=CARTESIAN_POINT ( 'NONE',  ( -21.79482124383139308, -8.775876708292097206, 70.30945321915166346 ) ) ;
#26320=PLANE ( 'NONE',  #6696 ) ;
#26321=ADVANCED_FACE ( 'NONE', ( #2280 ), #23417, .T. ) ;
#26322=ADVANCED_FACE ( 'NONE', ( #28144 ), #14891, .T. ) ;
#26324=ORIENTED_EDGE ( 'NONE', *, *, #26179, .F. ) ;
#26325=CARTESIAN_POINT ( 'NONE',  ( -22.37985709289073455, -19.82347726015160205, 69.17417989525732480 ) ) ;
#26326=CARTESIAN_POINT ( 'NONE',  ( -10.16749015965427105, -13.12235144340169235, 71.39323866028058774 ) ) ;
#26328=CARTESIAN_POINT ( 'NONE',  ( -10.39215600595210631, -14.30487551902977827, 64.38803863383273551 ) ) ;
#26330=CARTESIAN_POINT ( 'NONE',  ( -12.40380833417894912, -19.68739609921301792, 61.39678633575574906 ) ) ;
#26331=CARTESIAN_POINT ( 'NONE',  ( -12.80135276601915528, -20.13603490024450693, 68.22168825917964341 ) ) ;
#26334=ORIENTED_EDGE ( 'NONE', *, *, #38434, .T. ) ;
#26335=CARTESIAN_POINT ( 'NONE',  ( -15.88655729437939534, -7.980152340574909076, 67.44007279406643818 ) ) ;
#26337=CARTESIAN_POINT ( 'NONE',  ( -10.53536195276627829, -13.30851587854854579, 74.69289754060230280 ) ) ;
#26338=ORIENTED_EDGE ( 'NONE', *, *, #27799, .F. ) ;
#26339=VECTOR ( 'NONE', #29662, 1000.000000000000114 ) ;
#26340=ORIENTED_EDGE ( 'NONE', *, *, #18573, .F. ) ;
#26341=EDGE_CURVE ( 'NONE', #17056, #31648, #27049, .T. ) ;
#26345=CARTESIAN_POINT ( 'NONE',  ( -21.57940561823839332, -9.104090476609597360, 63.34720799502051847 ) ) ;
#26346=CARTESIAN_POINT ( 'NONE',  ( -10.18733296281416045, -13.03881024611776418, 71.34795252663174381 ) ) ;
#26347=VERTEX_POINT ( 'NONE', #18248 ) ;
#26348=LINE ( 'NONE', #41618, #48650 ) ;
#26350=EDGE_CURVE ( 'NONE', #9970, #30992, #35052, .T. ) ;
#26351=ORIENTED_EDGE ( 'NONE', *, *, #35650, .F. ) ;
#26352=CARTESIAN_POINT ( 'NONE',  ( -21.84079810191280657, -9.314188493807273872, 63.49153755726583626 ) ) ;
#26354=( BOUNDED_CURVE ( )  B_SPLINE_CURVE ( 3, ( #21378, #2877, #36365, #10759 ),
 .UNSPECIFIED., .F., .F. ) 
 B_SPLINE_CURVE_WITH_KNOTS ( ( 4, 4 ),
 ( 0.9074455897393595150, 1.000000000000000000 ),
 .UNSPECIFIED. ) 
 CURVE ( )  GEOMETRIC_REPRESENTATION_ITEM ( )  RATIONAL_B_SPLINE_CURVE ( ( 0.6983129098260925094, 0.7760317562606977582, 0.8765941196520002920, 1.000000000000000000 ) ) 
 REPRESENTATION_ITEM ( '' )  );
#26355=DIRECTION ( 'NONE',  ( -0.8743548079231422410, -0.4852872034802500067, 5.778319183281968808E-08 ) ) ;
#26356=CARTESIAN_POINT ( 'NONE',  ( -10.85423594767881283, -17.22645656662391289, 64.64355980017001002 ) ) ;
#26357=ORIENTED_EDGE ( 'NONE', *, *, #31434, .T. ) ;
#26358=CARTESIAN_POINT ( 'NONE',  ( -19.98727432552137984, -8.241621372411282564, 74.02096606371280529 ) ) ;
#26359=ORIENTED_EDGE ( 'NONE', *, *, #6611, .F. ) ;
#26360=CARTESIAN_POINT ( 'NONE',  ( -10.44378636108426583, -17.41310671260886167, 64.78885870823729931 ) ) ;
#26361=CARTESIAN_POINT ( 'NONE',  ( -12.35277332135121675, -20.26681466537264242, 68.45162004874669037 ) ) ;
#26362=ORIENTED_EDGE ( 'NONE', *, *, #15766, .F. ) ;
#26364=CARTESIAN_POINT ( 'NONE',  ( -20.10740643985815268, -21.75925148913131579, 72.51204570001823413 ) ) ;
#26366=FACE_OUTER_BOUND ( 'NONE', #31635, .T. ) ;
#26367=CARTESIAN_POINT ( 'NONE',  ( -10.79553443930103285, -17.05933049762642639, 57.91433868669456331 ) ) ;
#26368=CARTESIAN_POINT ( 'NONE',  ( -10.51874523558227636, -17.60584231662749843, 68.23688550535284492 ) ) ;
#26369=CARTESIAN_POINT ( 'NONE',  ( -13.42765988558316792, -8.521637316299758069, 57.10934427942139280 ) ) ;
#26375=CARTESIAN_POINT ( 'NONE',  ( -18.67683868338968978, -7.922091914708606630, 70.67067976651917149 ) ) ;
#26376=CARTESIAN_POINT ( 'NONE',  ( -23.77312771997254615, -18.70709664074277612, 72.87872845841107505 ) ) ;
#26377=ADVANCED_FACE ( 'NONE', ( #40427 ), #44874, .T. ) ;
#26378=EDGE_CURVE ( 'NONE', #11687, #36713, #17607, .T. ) ;
#26380=EDGE_LOOP ( 'NONE', ( #7856, #14120, #4677, #45681, #772 ) ) ;
#26381=CARTESIAN_POINT ( 'NONE',  ( -16.83291232462568132, -21.78581065439753317, 72.27616290343694061 ) ) ;
#26384=CARTESIAN_POINT ( 'NONE',  ( -13.49459827716768423, -24.71111635512870208, 54.60745305979834541 ) ) ;
#26385=CARTESIAN_POINT ( 'NONE',  ( -24.04646079654614255, -17.23801300935436132, 65.94357277538750850 ) ) ;
#26386=CARTESIAN_POINT ( 'NONE',  ( -21.84079810191280657, -9.314188493807273872, 63.49153755726583626 ) ) ;
#26387=CARTESIAN_POINT ( 'NONE',  ( -10.45984680026578495, -15.51639866492744169, 57.85327457721793110 ) ) ;
#26388=CARTESIAN_POINT ( 'NONE',  ( -21.60384785555947929, -20.97637623824866182, 72.64633634696070885 ) ) ;
#26389=CARTESIAN_POINT ( 'NONE',  ( -18.79049830835916524, -7.892586073225762000, 70.38540174208183942 ) ) ;
#26394=CARTESIAN_POINT ( 'NONE',  ( -22.51726279860821478, -19.68384809141796765, 72.64400547081167758 ) ) ;
#26395=CARTESIAN_POINT ( 'NONE',  ( -24.12697024258913103, -11.55706310638292500, 63.11364774580268033 ) ) ;
#26397=EDGE_CURVE ( 'NONE', #897, #20341, #16197, .T. ) ;
#26398=B_SPLINE_CURVE_WITH_KNOTS ( 'NONE', 3,
 ( #34010, #45126, #30350, #11611, #4238, #26643, #41658, #22963, #42393, #46329 ),
 .UNSPECIFIED., .F., .F.,
 ( 4, 2, 2, 2, 4 ),
 ( 0.6272669072782640631, 0.7522669073001383433, 0.8772669073220125124, 1.002266907343886793, 1.127266907365761073 ),
 .UNSPECIFIED. ) ;
#26399=CARTESIAN_POINT ( 'NONE',  ( -15.58315248484016102, -8.055165849531416455, 74.36369132414399985 ) ) ;
#26400=ADVANCED_FACE ( 'NONE', ( #47818 ), #24723, .T. ) ;
#26401=CARTESIAN_POINT ( 'NONE',  ( -17.74207408025691279, -7.814823900549897395, 63.66130038185828255 ) ) ;
#26404=CARTESIAN_POINT ( 'NONE',  ( -18.32364513544568752, -21.80460793730824420, 65.23043427352648393 ) ) ;
#26406=EDGE_LOOP ( 'NONE', ( #5618, #9491, #46179, #18492, #25412 ) ) ;
#26408=ORIENTED_EDGE ( 'NONE', *, *, #31951, .F. ) ;
#26409=EDGE_CURVE ( 'NONE', #6140, #7043, #11469, .T. ) ;
#26410=CARTESIAN_POINT ( 'NONE',  ( -23.55055098682252890, -19.04828202743015098, 66.01727754597818887 ) ) ;
#26412=( BOUNDED_CURVE ( )  B_SPLINE_CURVE ( 3, ( #27435, #1321, #8978, #12894 ),
 .UNSPECIFIED., .F., .F. ) 
 B_SPLINE_CURVE_WITH_KNOTS ( ( 4, 4 ),
 ( 0.5000000000000000000, 0.9074455897393632897 ),
 .UNSPECIFIED. ) 
 CURVE ( )  GEOMETRIC_REPRESENTATION_ITEM ( )  RATIONAL_B_SPLINE_CURVE ( ( 1.000000000000027534, 0.4567392136813411829, 0.3561768502900142797, 0.6983129098260767442 ) ) 
 REPRESENTATION_ITEM ( '' )  );
#26415=CARTESIAN_POINT ( 'NONE',  ( -16.07945710171498988, -22.13702619746868905, 58.44732121985853723 ) ) ;
#26418=CARTESIAN_POINT ( 'NONE',  ( -19.77436091090941517, -21.87886160397694368, 65.64981624214608757 ) ) ;
#26419=ORIENTED_EDGE ( 'NONE', *, *, #16384, .T. ) ;
#26421=( BOUNDED_CURVE ( )  B_SPLINE_CURVE ( 3, ( #16916, #30993, #39091, #20873 ),
 .UNSPECIFIED., .F., .F. ) 
 B_SPLINE_CURVE_WITH_KNOTS ( ( 4, 4 ),
 ( 0.9074455897393656212, 1.000000000000000000 ),
 .UNSPECIFIED. ) 
 CURVE ( )  GEOMETRIC_REPRESENTATION_ITEM ( )  RATIONAL_B_SPLINE_CURVE ( ( 0.6983129098260816292, 0.7760317562606884323, 0.8765941196519945189, 1.000000000000000000 ) ) 
 REPRESENTATION_ITEM ( '' )  );
#26422=PLANE ( 'NONE',  #25139 ) ;
#26423=ORIENTED_EDGE ( 'NONE', *, *, #9992, .F. ) ;
#26424=CARTESIAN_POINT ( 'NONE',  ( -11.10707449861472007, -10.85970573603012035, 57.40177339602415429 ) ) ;
#26426=CARTESIAN_POINT ( 'NONE',  ( -23.34481640033246208, -18.63641755246779752, 69.59371984262205046 ) ) ;
#26428=CARTESIAN_POINT ( 'NONE',  ( -10.60148393199744632, -13.03252788045845811, 68.03272542065271011 ) ) ;
#26429=DIRECTION ( 'NONE',  ( 0.9968684284758859704, -0.07907803935364898784, 1.831731161803828914E-08 ) ) ;
#26431=CARTESIAN_POINT ( 'NONE',  ( -10.52215041504658188, -13.37196039468858011, 74.97817647370040106 ) ) ;
#26432=CARTESIAN_POINT ( 'NONE',  ( -22.10033346171958257, -20.08913226167895871, 58.64954131300479645 ) ) ;
#26433=ORIENTED_EDGE ( 'NONE', *, *, #37212, .T. ) ;
#26434=CARTESIAN_POINT ( 'NONE',  ( -10.64577699202231287, -11.71757285455929853, 74.67344842241411129 ) ) ;
#26436=CARTESIAN_POINT ( 'NONE',  ( -10.73201024307833862, -12.75570352104612581, 61.02526939955659202 ) ) ;
#26437=( BOUNDED_CURVE ( )  B_SPLINE_CURVE ( 3, ( #48367, #7020, #368, #40738 ),
 .UNSPECIFIED., .F., .F. ) 
 B_SPLINE_CURVE_WITH_KNOTS ( ( 4, 4 ),
 ( 0.9074455897393690629, 1.000000000000000000 ),
 .UNSPECIFIED. ) 
 CURVE ( )  GEOMETRIC_REPRESENTATION_ITEM ( )  RATIONAL_B_SPLINE_CURVE ( ( 0.6983129098261016132, 0.7760317562607056407, 0.8765941196520050660, 1.000000000000000000 ) ) 
 REPRESENTATION_ITEM ( '' )  );
#26438=CARTESIAN_POINT ( 'NONE',  ( -18.06756654779004734, -21.77956830110077391, 61.98421986606183509 ) ) ;
#26439=CARTESIAN_POINT ( 'NONE',  ( -23.89200480383413350, -11.11192299349349533, 70.07706151945906470 ) ) ;
#26442=VERTEX_POINT ( 'NONE', #9352 ) ;
#26443=CARTESIAN_POINT ( 'NONE',  ( -14.47836531470152188, -7.966228403338186936, 64.04624744032878425 ) ) ;
#26446=CARTESIAN_POINT ( 'NONE',  ( -15.36434817278061615, -8.119105809824066711, 74.18871620572336667 ) ) ;
#26448=ORIENTED_EDGE ( 'NONE', *, *, #20210, .F. ) ;
#26449=CARTESIAN_POINT ( 'NONE',  ( -23.55072138245576596, -11.31379833372481691, 66.63034415663315713 ) ) ;
#26451=CARTESIAN_POINT ( 'NONE',  ( -10.49796979654650642, -16.16706115165171198, 64.66338504953419886 ) ) ;
#26456=EDGE_CURVE ( 'NONE', #4981, #39185, #42319, .T. ) ;
#26457=B_SPLINE_CURVE_WITH_KNOTS ( 'NONE', 3,
 ( #12239, #31437, #15680, #22860, #19634, #12007, #37855, #8551, #34642, #26787 ),
 .UNSPECIFIED., .F., .F.,
 ( 4, 2, 2, 2, 4 ),
 ( 0.000000000000000000, 0.2500000000000000000, 0.5000000000000000000, 0.7500000000000000000, 1.000000000000000000 ),
 .UNSPECIFIED. ) ;
#26459=CARTESIAN_POINT ( 'NONE',  ( -11.39127492490111315, -11.16067319722467666, 60.69357916181100876 ) ) ;
#26460=CARTESIAN_POINT ( 'NONE',  ( -24.79586717699802279, -15.88714297609664072, 69.69454031355697055 ) ) ;
#26461=CARTESIAN_POINT ( 'NONE',  ( -13.24261801534493088, -8.643248549050911222, 60.55454889300790455 ) ) ;
#26464=EDGE_LOOP ( 'NONE', ( #23211, #9519, #25141, #42022, #2675 ) ) ;
#26466=CARTESIAN_POINT ( 'NONE',  ( -20.44655245503490448, -7.999037100505644204, 70.43755594487680582 ) ) ;
#26470=CARTESIAN_POINT ( 'NONE',  ( -16.29054414310137489, -7.847273438603864726, 63.76191313215372247 ) ) ;
#26471=CARTESIAN_POINT ( 'NONE',  ( -10.19958527806322302, -12.98708191879287455, 67.85176988805619658 ) ) ;
#26472=CARTESIAN_POINT ( 'NONE',  ( -18.83448644433554620, -7.952703815611509519, 66.91574162229849776 ) ) ;
#26474=EDGE_LOOP ( 'NONE', ( #48338, #1805, #32403, #42333, #2965 ) ) ;
#26475=CARTESIAN_POINT ( 'NONE',  ( -22.99430600995192719, -19.05128598164557729, 62.46480054767778967 ) ) ;
#26477=AXIS2_PLACEMENT_3D ( 'NONE', #32749, #3441, #21680 ) ;
#26478=ORIENTED_EDGE ( 'NONE', *, *, #14927, .F. ) ;
#26479=CARTESIAN_POINT ( 'NONE',  ( -13.07007069224803786, -8.763865476245500830, 64.16592477169881192 ) ) ;
#26481=CARTESIAN_POINT ( 'NONE',  ( -12.52014422847536856, -9.200672045504624919, 74.49639875428626112 ) ) ;
#26482=DIRECTION ( 'NONE',  ( 0.9501515917649786536, 0.3117883138709296453, -1.594035198779740729E-08 ) ) ;
#26483=ORIENTED_EDGE ( 'NONE', *, *, #38094, .F. ) ;
#26484=FACE_OUTER_BOUND ( 'NONE', #875, .T. ) ;
#26485=CARTESIAN_POINT ( 'NONE',  ( -22.77668345155328566, -19.99130182265360745, 72.82213277323756984 ) ) ;
#26489=DIRECTION ( 'NONE',  ( 1.504942871710700414E-06, -3.061075848816703091E-06, 0.9999999999941824314 ) ) ;
#26490=EDGE_LOOP ( 'NONE', ( #41554, #3478 ) ) ;
#26491=CARTESIAN_POINT ( 'NONE',  ( -23.08487763607990928, -19.01185175973044039, 62.36879011380454330 ) ) ;
#26492=CARTESIAN_POINT ( 'NONE',  ( -18.60622096112062707, -22.16490860957766529, 72.47006221837980888 ) ) ;
#26493=CARTESIAN_POINT ( 'NONE',  ( -12.54253407177667512, -19.82621502378690082, 65.16674886820000268 ) ) ;
#26494=FACE_BOUND ( 'NONE', #43124, .T. ) ;
#26496=B_SPLINE_CURVE_WITH_KNOTS ( 'NONE', 3,
 ( #38624, #5869, #20886, #35410, #28021, #27545, #4909, #35881, #9325, #19920 ),
 .UNSPECIFIED., .F., .F.,
 ( 4, 2, 2, 2, 4 ),
 ( 0.000000000000000000, 0.2500000000000000000, 0.5000000000000000000, 0.7500000000000000000, 1.000000000000000000 ),
 .UNSPECIFIED. ) ;
#26497=ORIENTED_EDGE ( 'NONE', *, *, #10569, .T. ) ;
#26498=CARTESIAN_POINT ( 'NONE',  ( -13.18474066807476675, -20.93551553819402855, 58.23145462665691241 ) ) ;
#26499=CARTESIAN_POINT ( 'NONE',  ( -10.55840457303676061, -16.17443647754080871, 71.74750434597797266 ) ) ;
#26500=CARTESIAN_POINT ( 'NONE',  ( -23.58616457878146377, -18.99640866789479432, 66.00884704819274873 ) ) ;
#26502=VERTEX_POINT ( 'NONE', #28304 ) ;
#26503=DIRECTION ( 'NONE',  ( 0.7437128929774846631, -0.6684991644116392573, 1.736198598216997869E-08 ) ) ;
#26504=ORIENTED_EDGE ( 'NONE', *, *, #23587, .T. ) ;
#26505=CARTESIAN_POINT ( 'NONE',  ( -20.83700022493355775, -19.12221826660256951, 54.07175714974878389 ) ) ;
#26506=CARTESIAN_POINT ( 'NONE',  ( -17.22281099395510751, -7.361840332823870625, 70.60540513140719554 ) ) ;
#26507=CARTESIAN_POINT ( 'NONE',  ( -22.11926001268504294, -9.024814352312150234, 63.30658345311071855 ) ) ;
#26509=PLANE ( 'NONE',  #34555 ) ;
#26511=ORIENTED_EDGE ( 'NONE', *, *, #45847, .F. ) ;
#26512=VERTEX_POINT ( 'NONE', #32702 ) ;
#26514=EDGE_CURVE ( 'NONE', #21258, #37232, #46993, .T. ) ;
#26515=CARTESIAN_POINT ( 'NONE',  ( -20.18610667881221232, -8.319513185189903126, 66.66615430743608783 ) ) ;
#26517=EDGE_CURVE ( 'NONE', #25885, #10223, #28160, .T. ) ;
#26518=DIRECTION ( 'NONE',  ( 0.9529680021988314875, -0.3030709269876716849, -3.918663087574881996E-08 ) ) ;
#26519=CARTESIAN_POINT ( 'NONE',  ( -23.56138462120852495, -11.33988936615837950, 70.04210750373424332 ) ) ;
#26520=CARTESIAN_POINT ( 'NONE',  ( -11.42962470904260464, -10.38539412368214521, 74.62380407152070916 ) ) ;
#26521=VECTOR ( 'NONE', #44506, 999.9999999999998863 ) ;
#26522=VECTOR ( 'NONE', #35763, 1000.000000000000000 ) ;
#26526=CARTESIAN_POINT ( 'NONE',  ( -17.63866143434000833, -7.362211242860705163, 63.66561706598076853 ) ) ;
#26527=CARTESIAN_POINT ( 'NONE',  ( -14.73375560093340120, -21.75656996136207866, 61.75105004614717785 ) ) ;
#26528=CARTESIAN_POINT ( 'NONE',  ( -20.54979434103954006, -8.489990112051950533, 63.61121512946457557 ) ) ;
#26529=VERTEX_POINT ( 'NONE', #23393 ) ;
#26530=EDGE_CURVE ( 'NONE', #35456, #14012, #46713, .T. ) ;
#26531=B_SPLINE_CURVE_WITH_KNOTS ( 'NONE', 3,
 ( #22890, #19174, #22382, #34676, #37883, #15215, #4172, #34179, #22629, #30276 ),
 .UNSPECIFIED., .F., .F.,
 ( 4, 2, 2, 2, 4 ),
 ( 0.000000000000000000, 0.2500000000000000000, 0.5000000000000000000, 0.7500000000000000000, 1.000000000000000000 ),
 .UNSPECIFIED. ) ;
#26533=ORIENTED_EDGE ( 'NONE', *, *, #7075, .T. ) ;
#26534=CARTESIAN_POINT ( 'NONE',  ( -14.66844689667836299, -21.73163918518723037, 61.82255689998408599 ) ) ;
#26535=CARTESIAN_POINT ( 'NONE',  ( -10.95917937052863422, -17.62195967018737619, 71.58190244267143498 ) ) ;
#26536=CARTESIAN_POINT ( 'NONE',  ( -10.02995829593802668, -13.89786868041111667, 57.63320316755233819 ) ) ;
#26538=CARTESIAN_POINT ( 'NONE',  ( -22.48964968825576705, -9.905448439006629968, 73.76689030015370463 ) ) ;
#26539=EDGE_CURVE ( 'NONE', #46952, #10750, #27453, .T. ) ;
#26540=CARTESIAN_POINT ( 'NONE',  ( -14.68116061496366065, -8.368928989582258282, 60.54669703003625614 ) ) ;
#26541=VERTEX_POINT ( 'NONE', #15740 ) ;
#26542=CARTESIAN_POINT ( 'NONE',  ( -22.69351926024366861, -21.46836770470456202, 54.38277594638588397 ) ) ;
#26545=DIRECTION ( 'NONE',  ( 0.3739781583979218671, 0.9274375111247651349, 6.296758467538776703E-09 ) ) ;
#26546=CARTESIAN_POINT ( 'NONE',  ( -16.29760673242258306, -22.17363489859456038, 61.87072740723333197 ) ) ;
#26547=ORIENTED_EDGE ( 'NONE', *, *, #33188, .T. ) ;
#26548=DIRECTION ( 'NONE',  ( -1.235321096432344812E-06, -4.801898932798036189E-07, -0.9999999999991217026 ) ) ;
#26550=ORIENTED_EDGE ( 'NONE', *, *, #47350, .F. ) ;
#26553=EDGE_LOOP ( 'NONE', ( #7750, #40045, #47205, #2679, #25128 ) ) ;
#26554=CARTESIAN_POINT ( 'NONE',  ( -12.84691039585993444, -8.931012183600500975, 67.56438067310742213 ) ) ;
#26555=CARTESIAN_POINT ( 'NONE',  ( -23.80139567369806741, -11.92276173358724201, 59.48235729430358987 ) ) ;
#26556=CARTESIAN_POINT ( 'NONE',  ( -20.17268378225416825, -8.371407738384645469, 70.25100341248858626 ) ) ;
#26558=CARTESIAN_POINT ( 'NONE',  ( -11.27147141364421401, -11.36706973555563494, 64.14882062048422995 ) ) ;
#26560=CARTESIAN_POINT ( 'NONE',  ( -16.30881670716104992, -7.898512009833411618, 60.20028524975941764 ) ) ;
#26561=( BOUNDED_SURFACE ( )  B_SPLINE_SURFACE ( 3, 1, ( 
 ( #11833, #1217 ),
 ( #19452, #8374 ),
 ( #31031, #4204 ),
 ( #4682, #1458 ),
 ( #41874, #23399 ),
 ( #19705, #8148 ),
 ( #747, #16470 ) ),
 .UNSPECIFIED., .T., .F., .F. ) 
 B_SPLINE_SURFACE_WITH_KNOTS ( ( 4, 3, 4 ),
 ( 2, 2 ),
 ( 0.000000000000000000, 0.5000000000000000000, 1.000000000000000000 ),
 ( 0.000000000000000000, 1.000000000000000000 ),
 .UNSPECIFIED. ) 
 GEOMETRIC_REPRESENTATION_ITEM ( )  RATIONAL_B_SPLINE_SURFACE ( (
 ( 1.000000000000000000, 1.000000000000000000),
 ( 0.3333333333333335369, 0.3333333333333330373),
 ( 0.3333333333333335369, 0.3333333333333330373),
 ( 1.000000000000000000, 1.000000000000000000),
 ( 0.3333333333333333703, 0.3333333333333333703),
 ( 0.3333333333333333703, 0.3333333333333333703),
 ( 1.000000000000000000, 1.000000000000000000) ) ) 
 REPRESENTATION_ITEM ( '' )  SURFACE ( )  );
#26562=CARTESIAN_POINT ( 'NONE',  ( -10.90274307526027542, -17.35673385334968089, 68.16892125527850510 ) ) ;
#26563=VERTEX_POINT ( 'NONE', #39377 ) ;
#26565=( BOUNDED_CURVE ( )  B_SPLINE_CURVE ( 3, ( #12737, #15930, #27511, #38332 ),
 .UNSPECIFIED., .F., .F. ) 
 B_SPLINE_CURVE_WITH_KNOTS ( ( 4, 4 ),
 ( 0.9074455897393608472, 1.000000000000000000 ),
 .UNSPECIFIED. ) 
 CURVE ( )  GEOMETRIC_REPRESENTATION_ITEM ( )  RATIONAL_B_SPLINE_CURVE ( ( 0.6983129098260804080, 0.7760317562606873221, 0.8765941196519938527, 1.000000000000000000 ) ) 
 REPRESENTATION_ITEM ( '' )  );
#26566=CARTESIAN_POINT ( 'NONE',  ( -14.42683414290149813, -8.428067600363897682, 67.25975083869262505 ) ) ;
#26568=B_SPLINE_CURVE_WITH_KNOTS ( 'NONE', 3,
 ( #17789, #21746, #36731, #39982, #44186, #28889, #18520, #44904, #43937, #2556 ),
 .UNSPECIFIED., .F., .F.,
 ( 4, 2, 2, 2, 4 ),
 ( 0.1272669073658494465, 0.2522669073463357781, 0.3772669073268221096, 0.5022669073073084967, 0.6272669072877947727 ),
 .UNSPECIFIED. ) ;
#26569=CARTESIAN_POINT ( 'NONE',  ( -21.73099075187129614, -8.730192115828774746, 70.31627817507801126 ) ) ;
#26572=CARTESIAN_POINT ( 'NONE',  ( -21.65477468606848532, -9.232349032746775208, 66.96149992608901869 ) ) ;
#26573=CARTESIAN_POINT ( 'NONE',  ( -10.73412848974934874, -11.53077067998621175, 71.20365450754333381 ) ) ;
#26574=DIRECTION ( 'NONE',  ( -0.4501286257827956661, -0.8929637284072021730, 1.500157795982635103E-08 ) ) ;
#26575=CARTESIAN_POINT ( 'NONE',  ( -10.39542940759278267, -14.25923383539692146, 64.39363650855324295 ) ) ;
#26577=CARTESIAN_POINT ( 'NONE',  ( -20.25220558506708102, -7.916061535415647832, 70.36445088532752834 ) ) ;
#26578=CARTESIAN_POINT ( 'NONE',  ( -12.35395094432871410, -20.26789845123980527, 68.59303345011528563 ) ) ;
#26579=CARTESIAN_POINT ( 'NONE',  ( -17.01596769717176372, -7.370308014455987156, 74.07522855441366971 ) ) ;
#26580=( BOUNDED_SURFACE ( )  B_SPLINE_SURFACE ( 3, 1, ( 
 ( #5375, #16914 ),
 ( #35396, #13462 ),
 ( #27772, #39089 ),
 ( #1419, #42798 ),
 ( #35149, #20869 ),
 ( #1674, #16434 ),
 ( #34912, #35868 ) ),
 .UNSPECIFIED., .T., .F., .F. ) 
 B_SPLINE_SURFACE_WITH_KNOTS ( ( 4, 3, 4 ),
 ( 2, 2 ),
 ( 0.000000000000000000, 0.5000000000000000000, 1.000000000000000000 ),
 ( 0.000000000000000000, 1.000000000000000000 ),
 .UNSPECIFIED. ) 
 GEOMETRIC_REPRESENTATION_ITEM ( )  RATIONAL_B_SPLINE_SURFACE ( (
 ( 1.000000000000000000, 1.000000000000000000),
 ( 0.3333333333333335369, 0.3333333333333330373),
 ( 0.3333333333333335369, 0.3333333333333330373),
 ( 1.000000000000000000, 1.000000000000000000),
 ( 0.3333333333333333703, 0.3333333333333333703),
 ( 0.3333333333333333703, 0.3333333333333333703),
 ( 1.000000000000000000, 1.000000000000000000) ) ) 
 REPRESENTATION_ITEM ( '' )  SURFACE ( )  );
#26581=CARTESIAN_POINT ( 'NONE',  ( -12.41315173547891781, -9.850077678253004621, 57.38935532239157311 ) ) ;
#26584=CARTESIAN_POINT ( 'NONE',  ( -11.51937024597566328, -18.66112914712196158, 64.74707106785028543 ) ) ;
#26587=CARTESIAN_POINT ( 'NONE',  ( -19.40149108948937240, -21.57997799771671765, 65.55666331783336886 ) ) ;
#26588=CARTESIAN_POINT ( 'NONE',  ( -13.53206926677945887, -8.990420089060579656, 60.45566976265779147 ) ) ;
#26592=ORIENTED_EDGE ( 'NONE', *, *, #17267, .F. ) ;
#26594=CARTESIAN_POINT ( 'NONE',  ( -15.40122101639776808, -21.97944830692560458, 72.22292343801429126 ) ) ;
#26598=ORIENTED_EDGE ( 'NONE', *, *, #786, .F. ) ;
#26599=EDGE_CURVE ( 'NONE', #26956, #10314, #26288, .T. ) ;
#26600=CARTESIAN_POINT ( 'NONE',  ( -14.36817892824948650, -8.455618309860652104, 67.54503025475185041 ) ) ;
#26602=ADVANCED_FACE ( 'NONE', ( #38889 ), #4569, .T. ) ;
#26604=ORIENTED_EDGE ( 'NONE', *, *, #48243, .T. ) ;
#26605=CARTESIAN_POINT ( 'NONE',  ( -9.976686065099853451, -14.58608982656816622, 71.51437949254577120 ) ) ;
#26606=CARTESIAN_POINT ( 'NONE',  ( -10.37382936219775154, -14.83089353207902228, 74.81251018390588570 ) ) ;
#26607=CARTESIAN_POINT ( 'NONE',  ( -23.04402284766838349, -19.06632961612601918, 59.16938527523783620 ) ) ;
#26609=CARTESIAN_POINT ( 'NONE',  ( -12.25434429315920859, -20.17366997322574562, 65.05170215947674706 ) ) ;
#26611=CARTESIAN_POINT ( 'NONE',  ( -23.77935182056019414, -10.92131427075145211, 73.52226634401078798 ) ) ;
#26612=CYLINDRICAL_SURFACE ( 'NONE', #15552, 0.1499999999999991063 ) ;
#26613=ORIENTED_EDGE ( 'NONE', *, *, #13065, .F. ) ;
#26614=CARTESIAN_POINT ( 'NONE',  ( -16.36034204477525478, -21.78224588847237086, 65.52564618146095654 ) ) ;
#26617=AXIS2_PLACEMENT_3D ( 'NONE', #13147, #39273, #12918 ) ;
#26618=CARTESIAN_POINT ( 'NONE',  ( -24.47066272824306665, -14.57993217219608972, 62.99824437345091610 ) ) ;
#26620=CARTESIAN_POINT ( 'NONE',  ( -23.00454255336054743, -10.50046069577333441, 59.88731295783226471 ) ) ;
#26621=CARTESIAN_POINT ( 'NONE',  ( -10.52131307627743340, -17.61206215953548337, 68.22005024680343865 ) ) ;
#26622=CARTESIAN_POINT ( 'NONE',  ( -20.84119928492008000, -20.97572016636869918, 62.41471400470057773 ) ) ;
#26625=AXIS2_PLACEMENT_3D ( 'NONE', #16856, #27232, #8521 ) ;
#26627=CARTESIAN_POINT ( 'NONE',  ( -13.12744695462171407, -20.89546087334666069, 58.30296024829184631 ) ) ;
#26628=CARTESIAN_POINT ( 'NONE',  ( -22.38400322090610217, -20.36826016184844335, 62.41934579407823236 ) ) ;
#26629=DIRECTION ( 'NONE',  ( -0.9529680021988313765, 0.3030709269876716849, 3.918663088761644638E-08 ) ) ;
#26630=CARTESIAN_POINT ( 'NONE',  ( -24.22177629109872399, -13.13842424187848934, 63.13264177643409880 ) ) ;
#26632=VERTEX_POINT ( 'NONE', #6851 ) ;
#26633=ORIENTED_EDGE ( 'NONE', *, *, #31345, .F. ) ;
#26634=FACE_OUTER_BOUND ( 'NONE', #2403, .T. ) ;
#26635=CARTESIAN_POINT ( 'NONE',  ( -14.97837282748989729, -8.193824179639600302, 60.73484884663594130 ) ) ;
#26636=ORIENTED_EDGE ( 'NONE', *, *, #40110, .T. ) ;
#26637=CARTESIAN_POINT ( 'NONE',  ( -24.83263378688676326, -15.59489965655864374, 73.18799144572807336 ) ) ;
#26640=CARTESIAN_POINT ( 'NONE',  ( -10.26935876326470876, -12.73200256517937312, 64.42869467744635870 ) ) ;
#26641=CARTESIAN_POINT ( 'NONE',  ( -24.73118759497682362, -16.26147063645814583, 62.69354438008230090 ) ) ;
#26642=CARTESIAN_POINT ( 'NONE',  ( -21.60997298628545593, -20.97227605400240336, 72.68479748740878676 ) ) ;
#26643=CARTESIAN_POINT ( 'NONE',  ( -23.58130562506259764, -19.00348601836356721, 65.93051099385326097 ) ) ;
#26645=CARTESIAN_POINT ( 'NONE',  ( -11.58430515049292886, -10.18324995017449908, 71.16904308454122940 ) ) ;
#26646=B_SPLINE_CURVE_WITH_KNOTS ( 'NONE', 1,
 ( #967, #23629 ),
 .UNSPECIFIED., .F., .F.,
 ( 2, 2 ),
 ( 0.000000000000000000, 1.000000000000000000 ),
 .UNSPECIFIED. ) ;
#26647=CARTESIAN_POINT ( 'NONE',  ( -10.54994933093899867, -13.24305344519376781, 71.49356453765415154 ) ) ;
#26649=CARTESIAN_POINT ( 'NONE',  ( -24.20371252810814866, -12.87440185077122834, 66.58774614429587757 ) ) ;
#26650=CARTESIAN_POINT ( 'NONE',  ( -23.28952267755650851, -10.88343168269180339, 73.51760210707182353 ) ) ;
#26651=ORIENTED_EDGE ( 'NONE', *, *, #47059, .F. ) ;
#26654=ORIENTED_EDGE ( 'NONE', *, *, #1067, .F. ) ;
#26656=FACE_OUTER_BOUND ( 'NONE', #37830, .T. ) ;
#26657=( BOUNDED_CURVE ( )  B_SPLINE_CURVE ( 3, ( #1233, #30218, #41274, #2457 ),
 .UNSPECIFIED., .F., .F. ) 
 B_SPLINE_CURVE_WITH_KNOTS ( ( 4, 4 ),
 ( 0.000000000000000000, 0.4074455897393574055 ),
 .UNSPECIFIED. ) 
 CURVE ( )  GEOMETRIC_REPRESENTATION_ITEM ( )  RATIONAL_B_SPLINE_CURVE ( ( 1.000000000000000000, 0.4567392136813416270, 0.3561768502900338751, 0.6983129098260767442 ) ) 
 REPRESENTATION_ITEM ( '' )  );
#26659=B_SPLINE_CURVE_WITH_KNOTS ( 'NONE', 3,
 ( #41866, #27079, #19700, #31503, #42833, #31023, #1711, #46540, #34710, #12298 ),
 .UNSPECIFIED., .F., .F.,
 ( 4, 2, 2, 2, 4 ),
 ( 0.000000000000000000, 0.2500000000000000000, 0.5000000000000000000, 0.7500000000000000000, 1.000000000000000000 ),
 .UNSPECIFIED. ) ;
#26661=CARTESIAN_POINT ( 'NONE',  ( -24.34138250757122179, -16.17068267630804357, 62.89328676667766160 ) ) ;
#26663=EDGE_CURVE ( 'NONE', #5991, #39328, #8051, .T. ) ;
#26664=CARTESIAN_POINT ( 'NONE',  ( -16.09337498760136853, -22.13948385882417824, 58.40090183616962349 ) ) ;
#26665=EDGE_LOOP ( 'NONE', ( #28834, #47551 ) ) ;
#26666=CARTESIAN_POINT ( 'NONE',  ( -13.89388974506275787, -21.36980381032900667, 72.11102993026078423 ) ) ;
#26667=AXIS2_PLACEMENT_3D ( 'NONE', #19900, #27768, #34906 ) ;
#26668=CARTESIAN_POINT ( 'NONE',  ( -17.63866254341385442, -7.362211269489866261, 63.66561597723832477 ) ) ;
#26669=ORIENTED_EDGE ( 'NONE', *, *, #17708, .F. ) ;
#26670=CARTESIAN_POINT ( 'NONE',  ( -22.36580195822040906, -20.38434351641670972, 62.43427942229939731 ) ) ;
#26671=CARTESIAN_POINT ( 'NONE',  ( -23.77487038158592014, -11.74745262826995429, 62.96690348473899235 ) ) ;
#26675=CARTESIAN_POINT ( 'NONE',  ( -14.37682202087475680, -19.38786730597468022, 53.49899999999994549 ) ) ;
#26676=CARTESIAN_POINT ( 'NONE',  ( -15.11475081961186540, -8.199755259496424031, 56.92170200118545154 ) ) ;
#26677=CARTESIAN_POINT ( 'NONE',  ( -17.22281210278579167, -7.361840297529252730, 70.60540404266352255 ) ) ;
#26679=FACE_OUTER_BOUND ( 'NONE', #39465, .T. ) ;
#26681=CARTESIAN_POINT ( 'NONE',  ( -15.40811923343077083, -21.56513327689926030, 72.06047564147742435 ) ) ;
#26682=CARTESIAN_POINT ( 'NONE',  ( -10.52483499103918874, -17.62059296423454313, 68.35367848399930324 ) ) ;
#26683=EDGE_LOOP ( 'NONE', ( #36357, #33959, #207, #14147, #47098 ) ) ;
#26685=CARTESIAN_POINT ( 'NONE',  ( -13.65828898514496359, -20.76952646431350757, 65.00101022825411690 ) ) ;
#26686=CARTESIAN_POINT ( 'NONE',  ( -10.39670887254123954, -15.41691257807914184, 61.12969206769774644 ) ) ;
#26688=CARTESIAN_POINT ( 'NONE',  ( -11.08897232857050597, -11.71577735905851902, 71.08860879097652230 ) ) ;
#26690=ADVANCED_FACE ( 'NONE', ( #10068 ), #41679, .T. ) ;
#26691=VERTEX_POINT ( 'NONE', #2186 ) ;
#26693=CARTESIAN_POINT ( 'NONE',  ( -17.70078711893434331, -22.25418926393874486, 58.58366112844367279 ) ) ;
#26694=CARTESIAN_POINT ( 'NONE',  ( -24.26830686446636776, -16.27808571390248105, 59.40867021969434347 ) ) ;
#26696=CARTESIAN_POINT ( 'NONE',  ( -19.49109506855409180, -21.54969648977046148, 62.28031529404344013 ) ) ;
#26697=VERTEX_POINT ( 'NONE', #16944 ) ;
#26699=VECTOR ( 'NONE', #7943, 1000.000000000000000 ) ;
#26701=CARTESIAN_POINT ( 'NONE',  ( -20.81921389985186721, -21.44071754855728784, 58.75979745677555854 ) ) ;
#26702=ORIENTED_EDGE ( 'NONE', *, *, #16466, .F. ) ;
#26704=B_SPLINE_CURVE_WITH_KNOTS ( 'NONE', 1,
 ( #24064, #38829 ),
 .UNSPECIFIED., .F., .F.,
 ( 2, 2 ),
 ( 0.000000000000000000, 1.000000000000000000 ),
 .UNSPECIFIED. ) ;
#26705=AXIS2_PLACEMENT_3D ( 'NONE', #42136, #30582, #526 ) ;
#26707=CARTESIAN_POINT ( 'NONE',  ( -18.60622205832422082, -22.16490843864383109, 72.47006330605313451 ) ) ;
#26708=B_SPLINE_CURVE_WITH_KNOTS ( 'NONE', 3,
 ( #14532, #10880, #7205, #22211, #33501, #29848, #44877, #12336, #38427, #1244 ),
 .UNSPECIFIED., .F., .F.,
 ( 4, 2, 2, 2, 4 ),
 ( 0.6272669072878269692, 0.7522669073073300350, 0.8772669073268331008, 1.002266907346336167, 1.127266907365839232 ),
 .UNSPECIFIED. ) ;
#26709=( BOUNDED_SURFACE ( )  B_SPLINE_SURFACE ( 3, 1, ( 
 ( #14994, #30058 ),
 ( #26345, #41358 ),
 ( #8138, #15481 ),
 ( #30547, #45567 ),
 ( #16705, #38884 ),
 ( #46536, #19695 ),
 ( #20169, #16461 ) ),
 .UNSPECIFIED., .T., .F., .F. ) 
 B_SPLINE_SURFACE_WITH_KNOTS ( ( 4, 3, 4 ),
 ( 2, 2 ),
 ( 0.000000000000000000, 0.5000000000000000000, 1.000000000000000000 ),
 ( 0.000000000000000000, 1.000000000000000000 ),
 .UNSPECIFIED. ) 
 GEOMETRIC_REPRESENTATION_ITEM ( )  RATIONAL_B_SPLINE_SURFACE ( (
 ( 1.000000000000000000, 1.000000000000000000),
 ( 0.3333333333333335369, 0.3333333333333330373),
 ( 0.3333333333333335369, 0.3333333333333330373),
 ( 1.000000000000000000, 1.000000000000000000),
 ( 0.3333333333333333703, 0.3333333333333333703),
 ( 0.3333333333333333703, 0.3333333333333333703),
 ( 1.000000000000000000, 1.000000000000000000) ) ) 
 REPRESENTATION_ITEM ( '' )  SURFACE ( )  );
#26710=CARTESIAN_POINT ( 'NONE',  ( -15.62100938680255524, -7.580606089661849012, 70.72494556531428600 ) ) ;
#26711=LINE ( 'NONE', #22522, #63 ) ;
#26713=ORIENTED_EDGE ( 'NONE', *, *, #4645, .F. ) ;
#26716=CARTESIAN_POINT ( 'NONE',  ( -10.44644826855572006, -14.24945678126164061, 61.14494592119106642 ) ) ;
#26719=B_SPLINE_CURVE_WITH_KNOTS ( 'NONE', 1,
 ( #31652, #9494 ),
 .UNSPECIFIED., .F., .F.,
 ( 2, 2 ),
 ( 0.000000000000000000, 1.000000000000000000 ),
 .UNSPECIFIED. ) ;
#26720=( BOUNDED_CURVE ( )  B_SPLINE_CURVE ( 3, ( #26685, #27166, #8221, #46121 ),
 .UNSPECIFIED., .F., .F. ) 
 B_SPLINE_CURVE_WITH_KNOTS ( ( 4, 4 ),
 ( 0.5000000000000000000, 0.9074455897393781667 ),
 .UNSPECIFIED. ) 
 CURVE ( )  GEOMETRIC_REPRESENTATION_ITEM ( )  RATIONAL_B_SPLINE_CURVE ( ( 0.9999999999999985567, 0.4567392136813051007, 0.3561768502900212741, 0.6983129098261455781 ) ) 
 REPRESENTATION_ITEM ( '' )  );
#26722=EDGE_CURVE ( 'NONE', #28688, #47772, #7613, .T. ) ;
#26723=CARTESIAN_POINT ( 'NONE',  ( -10.66644504159021878, -12.78954850062448578, 68.15321152835137752 ) ) ;
#26724=AXIS2_PLACEMENT_3D ( 'NONE', #43568, #41311, #44785 ) ;
#26727=ORIENTED_EDGE ( 'NONE', *, *, #45921, .T. ) ;
#26728=CARTESIAN_POINT ( 'NONE',  ( -24.47744085606393583, -14.87036544990968423, 62.80476446885626984 ) ) ;
#26731=ADVANCED_FACE ( 'NONE', ( #17676 ), #6126, .T. ) ;
#26732=CARTESIAN_POINT ( 'NONE',  ( -21.73633048181673999, -9.221757950931626979, 59.87738363463013513 ) ) ;
#26733=CARTESIAN_POINT ( 'NONE',  ( -24.90891992605694227, -15.28604896337863472, 54.27966884056655061 ) ) ;
#26734=DIRECTION ( 'NONE',  ( 0.2393415023380396356, -0.9709354485539014590, 6.438601123316498798E-08 ) ) ;
#26735=CARTESIAN_POINT ( 'NONE',  ( -13.24069677618990504, -9.134368938356168144, 64.20386707414483851 ) ) ;
#26737=ORIENTED_EDGE ( 'NONE', *, *, #23518, .F. ) ;
#26738=CARTESIAN_POINT ( 'NONE',  ( -10.70532053225239366, -12.67267096592666675, 61.08381491717225487 ) ) ;
#26741=CARTESIAN_POINT ( 'NONE',  ( -12.23220172533775241, -19.57856247689574403, 57.92682373937842044 ) ) ;
#26742=CARTESIAN_POINT ( 'NONE',  ( -24.48534228222961673, -17.18449783053895530, 72.98997734255360115 ) ) ;
#26744=PLANE ( 'NONE',  #37781 ) ;
#26746=CARTESIAN_POINT ( 'NONE',  ( -23.41616298382994898, -18.52428493080399363, 72.77840375779385340 ) ) ;
#26747=FACE_BOUND ( 'NONE', #37357, .T. ) ;
#26749=DIRECTION ( 'NONE',  ( 0.1261685609230672744, 0.9920088176193796459, 5.058037262945178220E-08 ) ) ;
#26754=ORIENTED_EDGE ( 'NONE', *, *, #20068, .T. ) ;
#26755=CARTESIAN_POINT ( 'NONE',  ( -10.55855397105558779, -16.42450592920206276, 71.33261492083846633 ) ) ;
#26756=VERTEX_POINT ( 'NONE', #47003 ) ;
#26757=CYLINDRICAL_SURFACE ( 'NONE', #28965, 0.1499999999999956923 ) ;
#26758=CARTESIAN_POINT ( 'NONE',  ( -22.97806169198474535, -10.54588128516193102, 63.26113122312534642 ) ) ;
#26759=FACE_OUTER_BOUND ( 'NONE', #29576, .T. ) ;
#26760=ORIENTED_EDGE ( 'NONE', *, *, #20338, .T. ) ;
#26761=CARTESIAN_POINT ( 'NONE',  ( -11.64235026963700292, -18.84330375823651949, 68.21689631561287115 ) ) ;
#26762=ORIENTED_EDGE ( 'NONE', *, *, #5545, .T. ) ;
#26764=VERTEX_POINT ( 'NONE', #43329 ) ;
#26765=CARTESIAN_POINT ( 'NONE',  ( -14.99706723701585354, -21.85287888328288375, 65.29092001793476641 ) ) ;
#26767=CARTESIAN_POINT ( 'NONE',  ( -20.44433886619616914, -7.998055119120133227, 66.89448804686142580 ) ) ;
#26768=CARTESIAN_POINT ( 'NONE',  ( -21.90510274986183603, -8.857417179619462289, 66.76811671267451231 ) ) ;
#26769=CARTESIAN_POINT ( 'NONE',  ( -17.11594671439511828, -7.315539529225058679, 53.49999999999994316 ) ) ;
#26771=CARTESIAN_POINT ( 'NONE',  ( -12.40538917401127961, -20.31523793222865493, 68.52152763170285255 ) ) ;
#26772=CARTESIAN_POINT ( 'NONE',  ( -22.83095763869631512, -19.93459457198476770, 72.82895875648904394 ) ) ;
#26773=AXIS2_PLACEMENT_3D ( 'NONE', #42462, #41972, #8971 ) ;
#26774=ORIENTED_EDGE ( 'NONE', *, *, #6281, .T. ) ;
#26775=ORIENTED_EDGE ( 'NONE', *, *, #46941, .T. ) ;
#26776=( BOUNDED_SURFACE ( )  B_SPLINE_SURFACE ( 3, 1, ( 
 ( #45043, #25153 ),
 ( #6447, #26301 ),
 ( #30008, #36217 ),
 ( #10134, #29081 ),
 ( #30503, #11524 ),
 ( #11289, #14034 ),
 ( #15435, #21462 ) ),
 .UNSPECIFIED., .T., .F., .F. ) 
 B_SPLINE_SURFACE_WITH_KNOTS ( ( 4, 3, 4 ),
 ( 2, 2 ),
 ( 0.000000000000000000, 0.5000000000000000000, 1.000000000000000000 ),
 ( 0.000000000000000000, 1.000000000000000000 ),
 .UNSPECIFIED. ) 
 GEOMETRIC_REPRESENTATION_ITEM ( )  RATIONAL_B_SPLINE_SURFACE ( (
 ( 1.000000000000000000, 1.000000000000000000),
 ( 0.3333333333333335369, 0.3333333333333330373),
 ( 0.3333333333333335369, 0.3333333333333330373),
 ( 1.000000000000000000, 1.000000000000000000),
 ( 0.3333333333333333703, 0.3333333333333333703),
 ( 0.3333333333333333703, 0.3333333333333333703),
 ( 1.000000000000000000, 1.000000000000000000) ) ) 
 REPRESENTATION_ITEM ( '' )  SURFACE ( )  );
#26777=CARTESIAN_POINT ( 'NONE',  ( -12.13372751330810928, -16.36162385676421493, 53.88362224778185805 ) ) ;
#26778=CARTESIAN_POINT ( 'NONE',  ( -10.52991759648590531, -16.02177972226642311, 68.27767831073917648 ) ) ;
#26780=LINE ( 'NONE', #5097, #31531 ) ;
#26782=ADVANCED_FACE ( 'NONE', ( #17189 ), #47258, .T. ) ;
#26783=B_SPLINE_CURVE_WITH_KNOTS ( 'NONE', 3,
 ( #8099, #45045, #41572, #45995, #20624, #31451, #46234, #23594, #38595, #4882 ),
 .UNSPECIFIED., .F., .F.,
 ( 4, 2, 2, 2, 4 ),
 ( 0.1272669073658330152, 0.2522669073463136846, 0.3772669073267943540, 0.5022669073072749679, 0.6272669072877556928 ),
 .UNSPECIFIED. ) ;
#26785=VERTEX_POINT ( 'NONE', #44531 ) ;
#26786=CARTESIAN_POINT ( 'NONE',  ( -10.62512194321859127, -12.94411275245784410, 67.74392152479347828 ) ) ;
#26787=CARTESIAN_POINT ( 'NONE',  ( -15.29809733969474195, -21.47854975192407778, 68.87592918283094434 ) ) ;
#26788=CARTESIAN_POINT ( 'NONE',  ( -15.22349691269893057, -21.45476926339652479, 68.59209542689700356 ) ) ;
#26789=EDGE_LOOP ( 'NONE', ( #8383, #40122, #7469, #40055, #23453 ) ) ;
#26791=CARTESIAN_POINT ( 'NONE',  ( -10.60264614768167846, -13.01441009583156472, 64.47655987029209257 ) ) ;
#26792=CARTESIAN_POINT ( 'NONE',  ( -22.84088606172599967, -19.92422106693271999, 72.80433942285431215 ) ) ;
#26793=B_SPLINE_CURVE_WITH_KNOTS ( 'NONE', 3,
 ( #469, #23121, #235, #26314, #41331, #45290, #33675, #15448, #11538, #7620 ),
 .UNSPECIFIED., .F., .F.,
 ( 4, 2, 2, 2, 4 ),
 ( 0.000000000000000000, 0.2500000000000000000, 0.5000000000000000000, 0.7500000000000000000, 1.000000000000000000 ),
 .UNSPECIFIED. ) ;
#26794=EDGE_CURVE ( 'NONE', #44919, #38482, #16395, .T. ) ;
#26796=ORIENTED_EDGE ( 'NONE', *, *, #3898, .F. ) ;
#26799=DIRECTION ( 'NONE',  ( 0.6408936281290997794, 0.7676297007174212039, 4.260501105223829885E-08 ) ) ;
#26800=VERTEX_POINT ( 'NONE', #26063 ) ;
#26803=ORIENTED_EDGE ( 'NONE', *, *, #7232, .F. ) ;
#26806=CARTESIAN_POINT ( 'NONE',  ( -12.36794914932409561, -19.72224030764921565, 61.39678633597973345 ) ) ;
#26807=EDGE_CURVE ( 'NONE', #34499, #7578, #31899, .T. ) ;
#26809=DIRECTION ( 'NONE',  ( -0.3668819201507741989, 0.9245033139891488672, 0.1033986416233889649 ) ) ;
#26810=DIRECTION ( 'NONE',  ( -1.261798974855884165E-05, 2.391811520720373553E-06, -0.9999999999175327448 ) ) ;
#26811=CARTESIAN_POINT ( 'NONE',  ( -21.99213670719075253, -20.17946569659695299, 59.04970794435396897 ) ) ;
#26812=ORIENTED_EDGE ( 'NONE', *, *, #6866, .T. ) ;
#26813=AXIS2_PLACEMENT_3D ( 'NONE', #27496, #34633, #15913 ) ;
#26815=EDGE_CURVE ( 'NONE', #12408, #35856, #19682, .T. ) ;
#26816=CARTESIAN_POINT ( 'NONE',  ( -19.67760665824181388, -21.48965406232008490, 65.75014118398131302 ) ) ;
#26817=DIRECTION ( 'NONE',  ( 0.3374354101627464186, 0.9413486835218386473, 1.423378189492272593E-08 ) ) ;
#26818=B_SPLINE_CURVE_WITH_KNOTS ( 'NONE', 3,
 ( #34552, #31354, #8721, #46384, #15585, #34302, #34803, #38003, #4060, #23493 ),
 .UNSPECIFIED., .F., .F.,
 ( 4, 2, 2, 2, 4 ),
 ( 0.000000000000000000, 0.2500000000000000000, 0.5000000000000000000, 0.7500000000000000000, 1.000000000000000000 ),
 .UNSPECIFIED. ) ;
#26820=CARTESIAN_POINT ( 'NONE',  ( -12.05451961919647630, -9.643808529799599683, 57.20280282899455671 ) ) ;
#26821=CARTESIAN_POINT ( 'NONE',  ( -21.01124108229941001, -20.87838065962769463, 65.88453944495783787 ) ) ;
#26823=VERTEX_POINT ( 'NONE', #22125 ) ;
#26824=ORIENTED_EDGE ( 'NONE', *, *, #11648, .F. ) ;
#26825=CARTESIAN_POINT ( 'NONE',  ( -24.84978522997450767, -14.20774122709759801, 69.75251648635047275 ) ) ;
#26827=CARTESIAN_POINT ( 'NONE',  ( -21.76006473383504414, -8.751000872772104699, 70.28132536106762984 ) ) ;
#26830=CARTESIAN_POINT ( 'NONE',  ( -12.12077823425219414, -9.576857651715958042, 57.28924319034693013 ) ) ;
#26831=CARTESIAN_POINT ( 'NONE',  ( -23.98503169607928953, -17.39005800936845603, 66.22885190747201989 ) ) ;
#26832=CARTESIAN_POINT ( 'NONE',  ( -9.975093145215874202, -14.93635225021824198, 74.98274299234972773 ) ) ;
#26833=ORIENTED_EDGE ( 'NONE', *, *, #14134, .F. ) ;
#26836=CIRCLE ( 'NONE', #5606, 7.500000000000001776 ) ;
#26837=DIRECTION ( 'NONE',  ( -1.143861050413982909E-05, 2.837703136207094791E-06, -0.9999999999305527743 ) ) ;
#26838=CARTESIAN_POINT ( 'NONE',  ( -18.52460027084869765, -7.842592186127370191, 70.25579138408188840 ) ) ;
#26841=ORIENTED_EDGE ( 'NONE', *, *, #29431, .T. ) ;
#26842=ORIENTED_EDGE ( 'NONE', *, *, #14617, .F. ) ;
#26844=CARTESIAN_POINT ( 'NONE',  ( -10.70532053225239544, -12.67267096592666498, 61.08381491717225487 ) ) ;
#26845=CARTESIAN_POINT ( 'NONE',  ( -11.69223540468882838, -10.05010615616768810, 67.60558564255768488 ) ) ;
#26846=FACE_OUTER_BOUND ( 'NONE', #44523, .T. ) ;
#26848=( BOUNDED_CURVE ( )  B_SPLINE_CURVE ( 3, ( #2866, #44026, #36830, #47692 ),
 .UNSPECIFIED., .F., .F. ) 
 B_SPLINE_CURVE_WITH_KNOTS ( ( 4, 4 ),
 ( 0.9074455897393659543, 1.000000000000000000 ),
 .UNSPECIFIED. ) 
 CURVE ( )  GEOMETRIC_REPRESENTATION_ITEM ( )  RATIONAL_B_SPLINE_CURVE ( ( 0.6983129098260867362, 0.7760317562606927622, 0.8765941196519971834, 1.000000000000000000 ) ) 
 REPRESENTATION_ITEM ( '' )  );
#26850=EDGE_CURVE ( 'NONE', #36512, #30726, #9622, .T. ) ;
#26851=CARTESIAN_POINT ( 'NONE',  ( -13.05823701642829882, -9.336965241264831405, 71.13308820894700091 ) ) ;
#26852=DIRECTION ( 'NONE',  ( 2.201155577252676169E-06, 7.355553122608190330E-06, 0.9999999999705252440 ) ) ;
#26853=AXIS2_PLACEMENT_3D ( 'NONE', #32425, #47446, #28724 ) ;
#26854=ORIENTED_EDGE ( 'NONE', *, *, #32635, .T. ) ;
#26855=ADVANCED_FACE ( 'NONE', ( #29753 ), #30000, .T. ) ;
#26856=CARTESIAN_POINT ( 'NONE',  ( -10.96921284960095377, -11.97350354382807680, 74.84368195529052059 ) ) ;
#26857=CARTESIAN_POINT ( 'NONE',  ( -22.09360125616737136, -20.02631309226648781, 65.89348735000095303 ) ) ;
#26858=( BOUNDED_CURVE ( )  B_SPLINE_CURVE ( 3, ( #13763, #46571, #28573, #47034 ),
 .UNSPECIFIED., .F., .F. ) 
 B_SPLINE_CURVE_WITH_KNOTS ( ( 4, 4 ),
 ( 0.5000000000000000000, 0.9074455897393687298 ),
 .UNSPECIFIED. ) 
 CURVE ( )  GEOMETRIC_REPRESENTATION_ITEM ( )  RATIONAL_B_SPLINE_CURVE ( ( 1.000000000000017542, 0.4567392136813246406, 0.3561768502900152789, 0.6983129098261083856 ) ) 
 REPRESENTATION_ITEM ( '' )  );
#26859=ORIENTED_EDGE ( 'NONE', *, *, #43624, .T. ) ;
#26860=( BOUNDED_CURVE ( )  B_SPLINE_CURVE ( 3, ( #28307, #25332, #5893, #6616 ),
 .UNSPECIFIED., .F., .F. ) 
 B_SPLINE_CURVE_WITH_KNOTS ( ( 4, 4 ),
 ( 0.9074455897393722825, 1.000000000000000000 ),
 .UNSPECIFIED. ) 
 CURVE ( )  GEOMETRIC_REPRESENTATION_ITEM ( )  RATIONAL_B_SPLINE_CURVE ( ( 0.6983129098261113832, 0.7760317562607140784, 0.8765941196520102840, 1.000000000000000000 ) ) 
 REPRESENTATION_ITEM ( '' )  );
#26861=CARTESIAN_POINT ( 'NONE',  ( -19.94917705995926482, -8.226604131702123013, 74.00624557436877637 ) ) ;
#26862=ORIENTED_EDGE ( 'NONE', *, *, #10650, .T. ) ;
#26863=CARTESIAN_POINT ( 'NONE',  ( -26.22630854578367021, -13.51651355179587632, 53.49999999999995026 ) ) ;
#26864=EDGE_CURVE ( 'NONE', #28015, #47684, #28461, .T. ) ;
#26867=VERTEX_POINT ( 'NONE', #37111 ) ;
#26869=CARTESIAN_POINT ( 'NONE',  ( -24.32493921937862424, -13.34866582089179055, 63.13264457041533007 ) ) ;
#26872=CARTESIAN_POINT ( 'NONE',  ( -17.86643179882426935, -7.822757671798997947, 60.09677386199297899 ) ) ;
#26873=EDGE_CURVE ( 'NONE', #5898, #48128, #14593, .T. ) ;
#26874=CARTESIAN_POINT ( 'NONE',  ( -22.22370946352282672, -9.111183370010303761, 59.90666632495347699 ) ) ;
#26877=CARTESIAN_POINT ( 'NONE',  ( -24.47293982775255472, -15.07115001610720562, 59.54300207942560519 ) ) ;
#26878=( BOUNDED_SURFACE ( )  B_SPLINE_SURFACE ( 3, 1, ( 
 ( #12801, #46790 ),
 ( #5907, #46310 ),
 ( #2203, #5681 ),
 ( #47278, #13518 ),
 ( #20691, #5432 ),
 ( #27826, #43348 ),
 ( #9619, #42855 ) ),
 .UNSPECIFIED., .T., .F., .F. ) 
 B_SPLINE_SURFACE_WITH_KNOTS ( ( 4, 3, 4 ),
 ( 2, 2 ),
 ( 0.000000000000000000, 0.5000000000000000000, 1.000000000000000000 ),
 ( 0.000000000000000000, 1.000000000000000000 ),
 .UNSPECIFIED. ) 
 GEOMETRIC_REPRESENTATION_ITEM ( )  RATIONAL_B_SPLINE_SURFACE ( (
 ( 1.000000000000000000, 1.000000000000000000),
 ( 0.3333333333333335369, 0.3333333333333330373),
 ( 0.3333333333333335369, 0.3333333333333330373),
 ( 1.000000000000000000, 1.000000000000000000),
 ( 0.3333333333333333703, 0.3333333333333333703),
 ( 0.3333333333333333703, 0.3333333333333333703),
 ( 1.000000000000000000, 1.000000000000000000) ) ) 
 REPRESENTATION_ITEM ( '' )  SURFACE ( )  );
#26881=DIRECTION ( 'NONE',  ( -0.7670373483544791204, -0.6416024518573234525, 2.496223344567222868E-08 ) ) ;
#26882=CARTESIAN_POINT ( 'NONE',  ( -23.78632397794047648, -18.68536885113667623, 72.96379443305436041 ) ) ;
#26884=ORIENTED_EDGE ( 'NONE', *, *, #41307, .T. ) ;
#26885=CARTESIAN_POINT ( 'NONE',  ( -10.81219955438992741, -11.37622629119364603, 67.76864606346147468 ) ) ;
#26888=CARTESIAN_POINT ( 'NONE',  ( -16.35985130318476166, -22.18285048229636303, 61.86229803363791291 ) ) ;
#26891=EDGE_CURVE ( 'NONE', #25305, #21669, #43561, .T. ) ;
#26892=CARTESIAN_POINT ( 'NONE',  ( -11.35824856342118316, -11.21643317443627197, 60.97885780702566905 ) ) ;
#26896=ORIENTED_EDGE ( 'NONE', *, *, #4999, .T. ) ;
#26897=PLANE ( 'NONE',  #31227 ) ;
#26898=EDGE_CURVE ( 'NONE', #4886, #13644, #42222, .T. ) ;
#26900=CARTESIAN_POINT ( 'NONE',  ( -13.77834422207524412, -20.78674875190709415, 68.64552295153497141 ) ) ;
#26901=CARTESIAN_POINT ( 'NONE',  ( -19.77500964849970799, -21.45962299806434359, 72.70478730350133389 ) ) ;
#26902=CARTESIAN_POINT ( 'NONE',  ( -17.91414045948978639, -21.84516348726148394, 65.76020891215902964 ) ) ;
#26903=VERTEX_POINT ( 'NONE', #14682 ) ;
#26904=VERTEX_POINT ( 'NONE', #46163 ) ;
#26907=CARTESIAN_POINT ( 'NONE',  ( -11.41947236009895228, -18.50911967460687535, 65.16195962094886340 ) ) ;
#26909=CARTESIAN_POINT ( 'NONE',  ( -16.54784415797146480, -21.75414618367045350, 61.94671215975959910 ) ) ;
#26911=CARTESIAN_POINT ( 'NONE',  ( -17.45593231491017505, -7.751306502474292870, 60.23627933525208533 ) ) ;
#26913=CARTESIAN_POINT ( 'NONE',  ( -17.79108452803360763, -21.84994637594637368, 58.69081321602850920 ) ) ;
#26914=CARTESIAN_POINT ( 'NONE',  ( -21.89130958583942288, -9.354787850460871468, 63.20625856529903075 ) ) ;
#26915=ORIENTED_EDGE ( 'NONE', *, *, #44137, .F. ) ;
#26917=CARTESIAN_POINT ( 'NONE',  ( -12.20309422964675150, -20.12380354524033521, 64.98179449731530610 ) ) ;
#26918=EDGE_LOOP ( 'NONE', ( #2152, #40088, #48256, #37362, #1159 ) ) ;
#26920=CARTESIAN_POINT ( 'NONE',  ( -22.18815592092731137, -20.53689392896745503, 58.86468654123366662 ) ) ;
#26921=ADVANCED_FACE ( 'NONE', ( #36868 ), #3152, .T. ) ;
#26922=CARTESIAN_POINT ( 'NONE',  ( -12.84615363328625648, -20.17103110633857455, 72.09181604382622766 ) ) ;
#26924=CARTESIAN_POINT ( 'NONE',  ( -19.64493829067500030, -21.44926303942544266, 69.12409502726751498 ) ) ;
#26925=CARTESIAN_POINT ( 'NONE',  ( -23.03238438629518114, -19.08140394072652768, 59.17850838485211540 ) ) ;
#26926=CARTESIAN_POINT ( 'NONE',  ( -11.55573786329523855, -10.21941616939416342, 71.15388509157428132 ) ) ;
#26928=EDGE_LOOP ( 'NONE', ( #23379, #17006, #2308, #1041, #3353 ) ) ;
#26929=DIRECTION ( 'NONE',  ( -1.474291233076046698E-06, -1.298191854940810726E-06, 0.9999999999980706544 ) ) ;
#26931=CARTESIAN_POINT ( 'NONE',  ( -13.76038152179329543, -18.92930211169645105, 53.69233794759168887 ) ) ;
#26932=CARTESIAN_POINT ( 'NONE',  ( -12.50766595982653584, -19.86205097402751463, 65.01674886870775083 ) ) ;
#26935=VERTEX_POINT ( 'NONE', #29498 ) ;
#26937=CARTESIAN_POINT ( 'NONE',  ( -11.03230881600246427, -10.98182333549695322, 60.79390388117851529 ) ) ;
#26939=CARTESIAN_POINT ( 'NONE',  ( -22.94085508618206859, -9.802298960702817254, 70.19673832247809742 ) ) ;
#26940=CARTESIAN_POINT ( 'NONE',  ( -10.76785811675246940, -12.48515291162924434, 57.61385273545094066 ) ) ;
#26941=ORIENTED_EDGE ( 'NONE', *, *, #19226, .T. ) ;
#26942=CARTESIAN_POINT ( 'NONE',  ( -10.37599212182869124, -14.63324797960940593, 71.34254748307667171 ) ) ;
#26943=EDGE_CURVE ( 'NONE', #7654, #45579, #17521, .T. ) ;
#26944=CARTESIAN_POINT ( 'NONE',  ( -24.42401385028228589, -14.76496886756241622, 59.25802720181223293 ) ) ;
#26945=CARTESIAN_POINT ( 'NONE',  ( -24.03316043928017720, -11.37042366253971259, 66.58361025287214829 ) ) ;
#26946=EDGE_CURVE ( 'NONE', #12909, #43562, #2870, .T. ) ;
#26947=EDGE_CURVE ( 'NONE', #27374, #1012, #45147, .T. ) ;
#26948=ORIENTED_EDGE ( 'NONE', *, *, #42546, .T. ) ;
#26950=( BOUNDED_CURVE ( )  B_SPLINE_CURVE ( 3, ( #2849, #6563, #10007, #32653 ),
 .UNSPECIFIED., .F., .F. ) 
 B_SPLINE_CURVE_WITH_KNOTS ( ( 4, 4 ),
 ( 0.9074455897393647330, 1.000000000000000000 ),
 .UNSPECIFIED. ) 
 CURVE ( )  GEOMETRIC_REPRESENTATION_ITEM ( )  RATIONAL_B_SPLINE_CURVE ( ( 0.6983129098260990597, 0.7760317562607034203, 0.8765941196520037337, 1.000000000000000000 ) ) 
 REPRESENTATION_ITEM ( '' )  );
#26951=CARTESIAN_POINT ( 'NONE',  ( -12.89750100592999971, -8.892007198426925996, 67.48668646829932527 ) ) ;
#26952=LINE ( 'NONE', #848, #24553 ) ;
#26953=CARTESIAN_POINT ( 'NONE',  ( -23.26206559395185991, -18.76176001737956511, 66.11829607788916974 ) ) ;
#26954=CARTESIAN_POINT ( 'NONE',  ( -23.12773592331248551, -18.86744558261350946, 62.36909269548800694 ) ) ;
#26955=VERTEX_POINT ( 'NONE', #12903 ) ;
#26956=VERTEX_POINT ( 'NONE', #17322 ) ;
#26958=CARTESIAN_POINT ( 'NONE',  ( -24.14679772577363437, -12.68507108172156705, 70.05770892828130059 ) ) ;
#26962=FACE_OUTER_BOUND ( 'NONE', #22784, .T. ) ;
#26963=CARTESIAN_POINT ( 'NONE',  ( -20.12437885760196110, -7.865711196993452781, 73.76450701231766516 ) ) ;
#26965=ORIENTED_EDGE ( 'NONE', *, *, #34543, .T. ) ;
#26966=CARTESIAN_POINT ( 'NONE',  ( -10.82867520472564848, -11.34449427682889677, 67.73369198428547122 ) ) ;
#26967=ORIENTED_EDGE ( 'NONE', *, *, #32406, .T. ) ;
#26968=CARTESIAN_POINT ( 'NONE',  ( -12.56078782956467421, -9.165549844850980676, 74.51934210929164237 ) ) ;
#26970=CARTESIAN_POINT ( 'NONE',  ( -24.41597802456916710, -17.38151951243146698, 69.52001501703639974 ) ) ;
#26971=DIRECTION ( 'NONE',  ( -5.731567514496413899E-31, -1.020425574103664789E-16, -1.000000000000000000 ) ) ;
#26972=EDGE_LOOP ( 'NONE', ( #27787, #28137, #7251, #42234, #27981 ) ) ;
#26975=CARTESIAN_POINT ( 'NONE',  ( -13.54823245630065998, -20.69819609872914157, 61.81646323537677290 ) ) ;
#26976=CARTESIAN_POINT ( 'NONE',  ( -20.86878983561329548, -8.203218349707368517, 60.00158597527717319 ) ) ;
#26977=ORIENTED_EDGE ( 'NONE', *, *, #43931, .T. ) ;
#26978=CARTESIAN_POINT ( 'NONE',  ( -18.60463909989377385, -22.16515503909319307, 72.32864992405023941 ) ) ;
#26979=DIRECTION ( 'NONE',  ( -1.209056809376604527E-06, -5.657077721962264774E-07, -0.9999999999991091570 ) ) ;
#26981=DIRECTION ( 'NONE',  ( -0.9087012777736582780, 0.4174469879787381932, 4.853707507795134418E-09 ) ) ;
#26984=LINE ( 'NONE', #42009, #44428 ) ;
#26985=LINE ( 'NONE', #5744, #37574 ) ;
#26988=LINE ( 'NONE', #19598, #30810 ) ;
#26990=CARTESIAN_POINT ( 'NONE',  ( -11.79630000206883977, -19.05592701419838519, 71.97213747039440079 ) ) ;
#26991=CARTESIAN_POINT ( 'NONE',  ( -20.78451513435706133, -21.00713107796517320, 62.12943504870421663 ) ) ;
#26992=( BOUNDED_CURVE ( )  B_SPLINE_CURVE ( 3, ( #48234, #14241, #33200, #40853 ),
 .UNSPECIFIED., .F., .F. ) 
 B_SPLINE_CURVE_WITH_KNOTS ( ( 4, 4 ),
 ( 0.000000000000000000, 0.4074455897393673975 ),
 .UNSPECIFIED. ) 
 CURVE ( )  GEOMETRIC_REPRESENTATION_ITEM ( )  RATIONAL_B_SPLINE_CURVE ( ( 1.000000000000000000, 0.4567392136813311909, 0.3561768502900300448, 0.6983129098260966172 ) ) 
 REPRESENTATION_ITEM ( '' )  );
#26993=ORIENTED_EDGE ( 'NONE', *, *, #37704, .F. ) ;
#26994=FACE_BOUND ( 'NONE', #13559, .T. ) ;
#26995=ORIENTED_EDGE ( 'NONE', *, *, #30174, .F. ) ;
#26997=ORIENTED_EDGE ( 'NONE', *, *, #46210, .F. ) ;
#26998=ORIENTED_EDGE ( 'NONE', *, *, #11267, .T. ) ;
#26999=FACE_OUTER_BOUND ( 'NONE', #27469, .T. ) ;
#27000=CARTESIAN_POINT ( 'NONE',  ( -21.91688961498890720, -8.866358848214497712, 66.76126358204035682 ) ) ;
#27001=CARTESIAN_POINT ( 'NONE',  ( -16.50613596612109646, -22.20251566029174128, 65.48210330380625521 ) ) ;
#27002=CARTESIAN_POINT ( 'NONE',  ( -13.01353307917097268, -8.804980454159759162, 64.09441913135431435 ) ) ;
#27003=CARTESIAN_POINT ( 'NONE',  ( -13.60238289842206072, -8.884932333444998775, 57.26967755503795843 ) ) ;
#27005=( BOUNDED_CURVE ( )  B_SPLINE_CURVE ( 3, ( #35367, #21334, #36325, #24552 ),
 .UNSPECIFIED., .F., .F. ) 
 B_SPLINE_CURVE_WITH_KNOTS ( ( 4, 4 ),
 ( 0.000000000000000000, 0.4074455897393594594 ),
 .UNSPECIFIED. ) 
 CURVE ( )  GEOMETRIC_REPRESENTATION_ITEM ( )  RATIONAL_B_SPLINE_CURVE ( ( 1.000000000000000000, 0.4567392136813387404, 0.3561768502900328204, 0.6983129098260824064 ) ) 
 REPRESENTATION_ITEM ( '' )  );
#27006=ORIENTED_EDGE ( 'NONE', *, *, #23814, .F. ) ;
#27007=ORIENTED_EDGE ( 'NONE', *, *, #1495, .F. ) ;
#27008=EDGE_CURVE ( 'NONE', #4981, #39185, #31674, .T. ) ;
#27010=CARTESIAN_POINT ( 'NONE',  ( -16.16063142123006813, -7.467037929575190525, 60.38523757159160965 ) ) ;
#27011=EDGE_CURVE ( 'NONE', #46585, #17249, #28664, .T. ) ;
#27012=CARTESIAN_POINT ( 'NONE',  ( -11.83709238739359648, -9.880916174117215789, 64.22903110108937597 ) ) ;
#27014=CARTESIAN_POINT ( 'NONE',  ( -19.67368922737015424, -21.43794379858934107, 65.47988644745025510 ) ) ;
#27015=EDGE_CURVE ( 'NONE', #7024, #47122, #28430, .T. ) ;
#27019=CARTESIAN_POINT ( 'NONE',  ( -16.20683845212634111, -21.70255763714999020, 58.58585572420326315 ) ) ;
#27022=VECTOR ( 'NONE', #25626, 1000.000000000000227 ) ;
#27023=CARTESIAN_POINT ( 'NONE',  ( -17.26224459804799238, -7.811016595343872382, 67.24713020387331142 ) ) ;
#27026=CARTESIAN_POINT ( 'NONE',  ( -11.33476804054750531, -19.10151225439055978, 68.40184904730287485 ) ) ;
#27029=LINE ( 'NONE', #5355, #45440 ) ;
#27030=CARTESIAN_POINT ( 'NONE',  ( -24.83263378688676326, -15.59489965655864374, 73.18799144572807336 ) ) ;
#27033=CARTESIAN_POINT ( 'NONE',  ( -10.01440776720603765, -14.03439672543145988, 61.03325998023760235 ) ) ;
#27035=DIRECTION ( 'NONE',  ( -5.731567514496413899E-31, -1.020425574103664789E-16, -1.000000000000000000 ) ) ;
#27037=ORIENTED_EDGE ( 'NONE', *, *, #14610, .T. ) ;
#27038=DIRECTION ( 'NONE',  ( 1.075201461790892195E-05, -1.608194661606879754E-06, -0.9999999999409039386 ) ) ;
#27039=CARTESIAN_POINT ( 'NONE',  ( -7.540694356433003342, -14.17955609235691661, 53.49999999999995026 ) ) ;
#27044=CARTESIAN_POINT ( 'NONE',  ( -16.40208429260315626, -7.882922619732885217, 60.42858434934230871 ) ) ;
#27045=CARTESIAN_POINT ( 'NONE',  ( -12.55296927903122040, -9.172306255172346212, 74.46923003722106671 ) ) ;
#27046=EDGE_LOOP ( 'NONE', ( #14189, #4960, #25355, #852, #28937 ) ) ;
#27047=CARTESIAN_POINT ( 'NONE',  ( -12.17725024227025621, -10.08844384719822429, 57.24502831558379512 ) ) ;
#27048=AXIS2_PLACEMENT_3D ( 'NONE', #2807, #48348, #43712 ) ;
#27049=B_SPLINE_CURVE_WITH_KNOTS ( 'NONE', 1,
 ( #33498, #6702 ),
 .UNSPECIFIED., .F., .F.,
 ( 2, 2 ),
 ( 0.000000000000000000, 1.000000000000000000 ),
 .UNSPECIFIED. ) ;
#27050=CARTESIAN_POINT ( 'NONE',  ( -23.29040906673546729, -19.40173929881165193, 59.02377295306128957 ) ) ;
#27051=EDGE_CURVE ( 'NONE', #10001, #10295, #24998, .T. ) ;
#27053=ORIENTED_EDGE ( 'NONE', *, *, #15245, .T. ) ;
#27055=CARTESIAN_POINT ( 'NONE',  ( -24.84733312566341823, -14.17682965153389674, 69.82992173574167794 ) ) ;
#27057=DIRECTION ( 'NONE',  ( 8.329294198805576557E-07, -2.487164606213012505E-06, 0.9999999999965599740 ) ) ;
#27059=CARTESIAN_POINT ( 'NONE',  ( -24.83515292193595769, -14.04764123926324082, 73.23776205861604183 ) ) ;
#27062=VERTEX_POINT ( 'NONE', #24504 ) ;
#27064=B_SPLINE_CURVE_WITH_KNOTS ( 'NONE', 1,
 ( #46510, #2404 ),
 .UNSPECIFIED., .F., .F.,
 ( 2, 2 ),
 ( 0.000000000000000000, 1.000000000000000000 ),
 .UNSPECIFIED. ) ;
#27065=CARTESIAN_POINT ( 'NONE',  ( -11.50733966670835784, -18.64282282746206576, 64.75266899466718939 ) ) ;
#27067=CARTESIAN_POINT ( 'NONE',  ( -18.63018970549565978, -7.457396494496333794, 73.95569010969242640 ) ) ;
#27068=CARTESIAN_POINT ( 'NONE',  ( -20.72450927900464634, -21.03929139025763106, 58.93003081252663833 ) ) ;
#27069=ADVANCED_FACE ( 'NONE', ( #10201 ), #9951, .T. ) ;
#27071=EDGE_CURVE ( 'NONE', #3400, #27869, #29742, .T. ) ;
#27072=ORIENTED_EDGE ( 'NONE', *, *, #44407, .T. ) ;
#27074=CARTESIAN_POINT ( 'NONE',  ( -24.86251202286899442, -14.39255128295101471, 66.22646819999783929 ) ) ;
#27076=CARTESIAN_POINT ( 'NONE',  ( -11.53247254227971652, -18.68106628708273931, 65.04707076447483871 ) ) ;
#27078=ORIENTED_EDGE ( 'NONE', *, *, #21393, .F. ) ;
#27079=CARTESIAN_POINT ( 'NONE',  ( -10.53709241384829909, -16.06257281177559904, 67.97767780858876563 ) ) ;
#27085=CARTESIAN_POINT ( 'NONE',  ( -22.63008487438422733, -10.12971324841507581, 70.31178520543817001 ) ) ;
#27087=ORIENTED_EDGE ( 'NONE', *, *, #25351, .T. ) ;
#27088=CARTESIAN_POINT ( 'NONE',  ( -17.54761332253163886, -7.808689223265699475, 67.20966559432535803 ) ) ;
#27092=VERTEX_POINT ( 'NONE', #3516 ) ;
#27096=CARTESIAN_POINT ( 'NONE',  ( -10.83008762082782006, -12.29245259246931354, 60.94286399630310314 ) ) ;
#27098=CARTESIAN_POINT ( 'NONE',  ( -19.43707224927095822, -8.044379180677138308, 63.57522333692026706 ) ) ;
#27099=CARTESIAN_POINT ( 'NONE',  ( -14.80056043599933524, -21.78207186541723317, 61.82095768364339960 ) ) ;
#27100=ORIENTED_EDGE ( 'NONE', *, *, #9712, .T. ) ;
#27103=CARTESIAN_POINT ( 'NONE',  ( -18.45621107931398797, -21.73269801629363940, 69.00617840904642719 ) ) ;
#27104=CARTESIAN_POINT ( 'NONE',  ( -20.69990079259183702, -20.99685563420014489, 62.18641693201382736 ) ) ;
#27105=VERTEX_POINT ( 'NONE', #18529 ) ;
#27106=ORIENTED_EDGE ( 'NONE', *, *, #15368, .F. ) ;
#27107=PLANE ( 'NONE',  #32225 ) ;
#27108=CARTESIAN_POINT ( 'NONE',  ( -22.88264614489240856, -10.34704276773305764, 63.35713876973677827 ) ) ;
#27109=ORIENTED_EDGE ( 'NONE', *, *, #14011, .F. ) ;
#27110=CARTESIAN_POINT ( 'NONE',  ( -10.39693166811831304, -15.37990016280386918, 57.58264896457095006 ) ) ;
#27111=CARTESIAN_POINT ( 'NONE',  ( -15.76121213363234119, -7.547108953211918880, 67.24668947344561332 ) ) ;
#27113=DIRECTION ( 'NONE',  ( 2.430360955834641685E-06, 9.751098515052924655E-07, -0.9999999999965711872 ) ) ;
#27114=CARTESIAN_POINT ( 'NONE',  ( -17.98657259272421172, -21.83703102787368167, 62.16063850355641307 ) ) ;
#27115=CARTESIAN_POINT ( 'NONE',  ( -15.77324524160535191, -8.006205000634873059, 70.62606529040051839 ) ) ;
#27118=ORIENTED_EDGE ( 'NONE', *, *, #35841, .T. ) ;
#27119=CARTESIAN_POINT ( 'NONE',  ( -10.02450680348118617, -15.67453976365170831, 61.13814800358835555 ) ) ;
#27122=EDGE_CURVE ( 'NONE', #21395, #24418, #2964, .T. ) ;
#27125=CARTESIAN_POINT ( 'NONE',  ( -21.39967327233876304, -20.63170314183283693, 72.80974286114339122 ) ) ;
#27127=B_SPLINE_CURVE_WITH_KNOTS ( 'NONE', 3,
 ( #3486, #18499, #48544, #23193, #19246, #8179, #4237, #30349, #781, #38684 ),
 .UNSPECIFIED., .F., .F.,
 ( 4, 2, 2, 2, 4 ),
 ( 0.000000000000000000, 0.2500000000000000000, 0.5000000000000000000, 0.7500000000000000000, 1.000000000000000000 ),
 .UNSPECIFIED. ) ;
#27128=( BOUNDED_SURFACE ( )  B_SPLINE_SURFACE ( 3, 1, ( 
 ( #34510, #46091 ),
 ( #20897, #30603 ),
 ( #45628, #11879 ),
 ( #34760, #23210 ),
 ( #15791, #12353 ),
 ( #16267, #794 ),
 ( #1034, #37963 ) ),
 .UNSPECIFIED., .T., .F., .F. ) 
 B_SPLINE_SURFACE_WITH_KNOTS ( ( 4, 3, 4 ),
 ( 2, 2 ),
 ( 0.000000000000000000, 0.5000000000000000000, 1.000000000000000000 ),
 ( 0.000000000000000000, 1.000000000000000000 ),
 .UNSPECIFIED. ) 
 GEOMETRIC_REPRESENTATION_ITEM ( )  RATIONAL_B_SPLINE_SURFACE ( (
 ( 1.000000000000000000, 1.000000000000000000),
 ( 0.3333333333333335369, 0.3333333333333330373),
 ( 0.3333333333333335369, 0.3333333333333330373),
 ( 1.000000000000000000, 1.000000000000000000),
 ( 0.3333333333333333703, 0.3333333333333333703),
 ( 0.3333333333333333703, 0.3333333333333333703),
 ( 1.000000000000000000, 1.000000000000000000) ) ) 
 REPRESENTATION_ITEM ( '' )  SURFACE ( )  );
#27129=CARTESIAN_POINT ( 'NONE',  ( -10.70566866894272984, -16.94585410378973123, 57.98760548748135335 ) ) ;
#27130=VERTEX_POINT ( 'NONE', #25937 ) ;
#27131=ORIENTED_EDGE ( 'NONE', *, *, #42518, .T. ) ;
#27135=CARTESIAN_POINT ( 'NONE',  ( -10.04792990808071984, -13.75760301026566523, 57.63480408467697913 ) ) ;
#27136=ADVANCED_FACE ( 'NONE', ( #25452 ), #43946, .T. ) ;
#27137=B_SPLINE_CURVE_WITH_KNOTS ( 'NONE', 3,
 ( #34244, #30586, #1243, #530, #45843, #27111, #16249, #38179, #42140, #8405 ),
 .UNSPECIFIED., .F., .F.,
 ( 4, 2, 2, 2, 4 ),
 ( 0.6272669072877962160, 0.7522669073073026125, 0.8772669073268088979, 1.002266907346315294, 1.127266907365821691 ),
 .UNSPECIFIED. ) ;
#27138=( BOUNDED_SURFACE ( )  B_SPLINE_SURFACE ( 3, 1, ( 
 ( #35021, #8943 ),
 ( #19044, #8218 ),
 ( #12142, #41700 ),
 ( #7986, #27164 ),
 ( #34535, #34048 ),
 ( #15569, #15325 ),
 ( #37989, #19783 ) ),
 .UNSPECIFIED., .T., .F., .F. ) 
 B_SPLINE_SURFACE_WITH_KNOTS ( ( 4, 3, 4 ),
 ( 2, 2 ),
 ( 0.000000000000000000, 0.5000000000000000000, 1.000000000000000000 ),
 ( 0.000000000000000000, 1.000000000000000000 ),
 .UNSPECIFIED. ) 
 GEOMETRIC_REPRESENTATION_ITEM ( )  RATIONAL_B_SPLINE_SURFACE ( (
 ( 1.000000000000000000, 1.000000000000000000),
 ( 0.3333333333333335369, 0.3333333333333330373),
 ( 0.3333333333333335369, 0.3333333333333330373),
 ( 1.000000000000000000, 1.000000000000000000),
 ( 0.3333333333333333703, 0.3333333333333333703),
 ( 0.3333333333333333703, 0.3333333333333333703),
 ( 1.000000000000000000, 1.000000000000000000) ) ) 
 REPRESENTATION_ITEM ( '' )  SURFACE ( )  );
#27139=ORIENTED_EDGE ( 'NONE', *, *, #36502, .T. ) ;
#27140=( BOUNDED_CURVE ( )  B_SPLINE_CURVE ( 3, ( #1868, #33034, #10891, #28468 ),
 .UNSPECIFIED., .F., .F. ) 
 B_SPLINE_CURVE_WITH_KNOTS ( ( 4, 4 ),
 ( 4.712388980384690562, 4.921828490624010399 ),
 .UNSPECIFIED. ) 
 CURVE ( )  GEOMETRIC_REPRESENTATION_ITEM ( )  RATIONAL_B_SPLINE_CURVE ( ( 1.000000000000000000, 0.9963479302455154896, 0.9963479302455154896, 1.000000000000000000 ) ) 
 REPRESENTATION_ITEM ( '' )  );
#27142=CARTESIAN_POINT ( 'NONE',  ( -10.95381480682210373, -17.48044017699314523, 68.09721944380058289 ) ) ;
#27143=LINE ( 'NONE', #15549, #16732 ) ;
#27144=ORIENTED_EDGE ( 'NONE', *, *, #1008, .F. ) ;
#27146=CARTESIAN_POINT ( 'NONE',  ( -19.30706997687812887, -22.01740875295033462, 58.64012098774584558 ) ) ;
#27147=VERTEX_POINT ( 'NONE', #6506 ) ;
#27149=EDGE_CURVE ( 'NONE', #11955, #31941, #34767, .T. ) ;
#27150=CARTESIAN_POINT ( 'NONE',  ( -23.95744578735505925, -17.32345456025280939, 69.69723189175576294 ) ) ;
#27151=( BOUNDED_CURVE ( )  B_SPLINE_CURVE ( 3, ( #14494, #40873, #44115, #10369 ),
 .UNSPECIFIED., .F., .F. ) 
 B_SPLINE_CURVE_WITH_KNOTS ( ( 4, 4 ),
 ( 0.9074455897393589598, 1.000000000000000000 ),
 .UNSPECIFIED. ) 
 CURVE ( )  GEOMETRIC_REPRESENTATION_ITEM ( )  RATIONAL_B_SPLINE_CURVE ( ( 0.6983129098260724144, 0.7760317562606804387, 0.8765941196519896339, 1.000000000000000000 ) ) 
 REPRESENTATION_ITEM ( '' )  );
#27152=EDGE_CURVE ( 'NONE', #22777, #18177, #48571, .T. ) ;
#27153=VECTOR ( 'NONE', #38069, 1000.000000000000114 ) ;
#27155=CARTESIAN_POINT ( 'NONE',  ( -11.14487098867647674, -10.79975683114651375, 57.38716000137919337 ) ) ;
#27156=CARTESIAN_POINT ( 'NONE',  ( -22.48430581236326731, -20.27711595259535571, 65.81926302645771898 ) ) ;
#27158=ORIENTED_EDGE ( 'NONE', *, *, #34698, .F. ) ;
#27159=CARTESIAN_POINT ( 'NONE',  ( -11.17855889551124982, -18.87086522978130532, 64.86211687253867808 ) ) ;
#27162=B_SPLINE_CURVE_WITH_KNOTS ( 'NONE', 3,
 ( #19491, #34506, #542, #1505, #11874, #8189, #4976, #24168, #12109, #1029 ),
 .UNSPECIFIED., .F., .F.,
 ( 4, 2, 2, 2, 4 ),
 ( 0.000000000000000000, 0.2500000000000000000, 0.5000000000000000000, 0.7500000000000000000, 1.000000000000000000 ),
 .UNSPECIFIED. ) ;
#27163=CARTESIAN_POINT ( 'NONE',  ( -10.83683317046381234, -12.44108562964681219, 57.62857332099802932 ) ) ;
#27164=CARTESIAN_POINT ( 'NONE',  ( -24.49635618495769407, -12.46679672499890046, 73.35730262454691797 ) ) ;
#27165=CARTESIAN_POINT ( 'NONE',  ( -15.49416032233947504, -8.028509233753512220, 74.07985659018983426 ) ) ;
#27166=CARTESIAN_POINT ( 'NONE',  ( -13.52147574634739158, -20.68483581939294780, 65.07809159860286741 ) ) ;
#27167=CARTESIAN_POINT ( 'NONE',  ( -20.75354924259569245, -21.52967727414722532, 54.27966884056655061 ) ) ;
#27168=CARTESIAN_POINT ( 'NONE',  ( -20.94768682599708853, -20.85770162187707299, 62.30574560354166636 ) ) ;
#27169=CARTESIAN_POINT ( 'NONE',  ( -10.49862800246030936, -15.82799116930659622, 64.50771590054291948 ) ) ;
#27171=ORIENTED_EDGE ( 'NONE', *, *, #48076, .T. ) ;
#27172=CARTESIAN_POINT ( 'NONE',  ( -17.91840021365262814, -21.79173196354552644, 62.17535923606572368 ) ) ;
#27173=CARTESIAN_POINT ( 'NONE',  ( -10.47674162631993866, -17.49967561431467544, 64.74926642219794815 ) ) ;
#27175=CARTESIAN_POINT ( 'NONE',  ( -9.974456290884534226, -14.72748455880875795, 71.51278017970571454 ) ) ;
#27176=CARTESIAN_POINT ( 'NONE',  ( -10.59994951589548151, -17.79852801025984732, 71.72864675479873142 ) ) ;
#27177=CARTESIAN_POINT ( 'NONE',  ( -23.25757785049868787, -10.17517560731475967, 63.18690593950643120 ) ) ;
#27178=DIRECTION ( 'NONE',  ( 8.563106566420985232E-06, -6.519503004583679708E-06, 0.9999999999420846608 ) ) ;
#27180=CARTESIAN_POINT ( 'NONE',  ( -18.33016535318852291, -22.20398178282153623, 69.07160637178317586 ) ) ;
#27181=CARTESIAN_POINT ( 'NONE',  ( -21.18000425931230168, -20.77541442555289919, 69.20450184740300870 ) ) ;
#27182=B_SPLINE_CURVE_WITH_KNOTS ( 'NONE', 3,
 ( #15732, #26594, #23152, #4421, #25857, #11332, #40872, #19441, #22409, #7651 ),
 .UNSPECIFIED., .F., .F.,
 ( 4, 2, 2, 2, 4 ),
 ( 0.6272669072976577720, 0.7522669073146923679, 0.8772669073317270749, 1.002266907348761782, 1.127266907365796378 ),
 .UNSPECIFIED. ) ;
#27183=CARTESIAN_POINT ( 'NONE',  ( -19.09948850906665285, -8.012659424734943414, 63.73089235424028942 ) ) ;
#27184=EDGE_LOOP ( 'NONE', ( #10998, #4589, #30946, #30604 ) ) ;
#27185=CARTESIAN_POINT ( 'NONE',  ( -17.29268214306257434, -7.359616301281327821, 70.67691090883880634 ) ) ;
#27188=CARTESIAN_POINT ( 'NONE',  ( -17.79084088774825645, -7.768752266068900347, 60.08060768310445354 ) ) ;
#27189=EDGE_LOOP ( 'NONE', ( #12210, #27072, #27131, #28949, #18312 ) ) ;
#27190=VERTEX_POINT ( 'NONE', #25684 ) ;
#27194=CARTESIAN_POINT ( 'NONE',  ( -10.73296288398890930, -12.58843297884804002, 60.79853574628657498 ) ) ;
#27195=EDGE_CURVE ( 'NONE', #31755, #12655, #3285, .T. ) ;
#27196=CARTESIAN_POINT ( 'NONE',  ( -20.50074447585702941, -8.457105438040551704, 70.39533052524389234 ) ) ;
#27197=CARTESIAN_POINT ( 'NONE',  ( -13.83108299072750391, -21.33561835983412891, 72.04112301026525245 ) ) ;
#27198=CARTESIAN_POINT ( 'NONE',  ( -17.70776945889202736, -22.25388964270624825, 58.52058054029878065 ) ) ;
#27199=CARTESIAN_POINT ( 'NONE',  ( -10.38360249164154325, -14.43747963625415309, 67.87272197508832505 ) ) ;
#27200=CARTESIAN_POINT ( 'NONE',  ( -10.38974003836240634, -14.29666208179129150, 68.27288787427933414 ) ) ;
#27201=CARTESIAN_POINT ( 'NONE',  ( -24.32132670238839012, -16.30692182044891325, 66.20758098450045281 ) ) ;
#27202=VERTEX_POINT ( 'NONE', #19515 ) ;
#27203=CARTESIAN_POINT ( 'NONE',  ( -24.41485940220508510, -14.44976662329334616, 66.18292729254385165 ) ) ;
#27204=ADVANCED_FACE ( 'NONE', ( #38464 ), #26422, .T. ) ;
#27205=CARTESIAN_POINT ( 'NONE',  ( -10.46944733747312917, -15.96661384539355133, 67.99239968927004441 ) ) ;
#27206=EDGE_CURVE ( 'NONE', #19106, #14369, #39792, .T. ) ;
#27209=CARTESIAN_POINT ( 'NONE',  ( -21.84079810191280657, -9.314188493807272096, 63.49153755726581494 ) ) ;
#27210=ADVANCED_FACE ( 'NONE', ( #30620 ), #19272, .T. ) ;
#27212=EDGE_CURVE ( 'NONE', #44794, #13527, #13037, .T. ) ;
#27213=CARTESIAN_POINT ( 'NONE',  ( -18.11578073608761841, -22.22715074075463804, 65.52344916871619773 ) ) ;
#27215=VERTEX_POINT ( 'NONE', #41431 ) ;
#27216=CARTESIAN_POINT ( 'NONE',  ( -16.39888349198502127, -21.73372412438269308, 62.05568132716130236 ) ) ;
#27220=CARTESIAN_POINT ( 'NONE',  ( -22.06352460594304787, -8.980016202103444201, 63.37649054182217867 ) ) ;
#27221=CARTESIAN_POINT ( 'NONE',  ( -20.89545688568268389, -21.40122061776584772, 58.80508532579719372 ) ) ;
#27224=VECTOR ( 'NONE', #36850, 1000.000000000000114 ) ;
#27225=FACE_BOUND ( 'NONE', #43761, .T. ) ;
#27226=CARTESIAN_POINT ( 'NONE',  ( -11.40696025980006389, -18.38620811258373422, 57.82216998879101055 ) ) ;
#27228=CARTESIAN_POINT ( 'NONE',  ( -10.66703363856100317, -12.79807828486586807, 64.26836111018113229 ) ) ;
#27230=CARTESIAN_POINT ( 'NONE',  ( -12.05483347687720475, -10.31798811457585963, 67.79896870046731294 ) ) ;
#27231=VERTEX_POINT ( 'NONE', #11639 ) ;
#27232=DIRECTION ( 'NONE',  ( 0.1539336739619741601, 0.9880811829098681276, 6.607022902453645889E-08 ) ) ;
#27233=CARTESIAN_POINT ( 'NONE',  ( -16.78341213209640159, -22.23169296657789928, 68.88056055876903372 ) ) ;
#27234=B_SPLINE_CURVE_WITH_KNOTS ( 'NONE', 3,
 ( #47155, #9733, #17337, #14343, #37495, #21768, #48346, #44675, #18799, #22014 ),
 .UNSPECIFIED., .F., .F.,
 ( 4, 2, 2, 2, 4 ),
 ( 0.000000000000000000, 0.2500000000000000000, 0.5000000000000000000, 0.7500000000000000000, 1.000000000000000000 ),
 .UNSPECIFIED. ) ;
#27235=VERTEX_POINT ( 'NONE', #7975 ) ;
#27236=CARTESIAN_POINT ( 'NONE',  ( -15.03263910315855512, -8.176888424288378587, 56.86472059657746314 ) ) ;
#27237=CARTESIAN_POINT ( 'NONE',  ( -12.73406765192711987, -9.020692726705027198, 71.04263666671683097 ) ) ;
#27238=ORIENTED_EDGE ( 'NONE', *, *, #9089, .F. ) ;
#27239=EDGE_CURVE ( 'NONE', #27904, #25059, #11694, .T. ) ;
#27240=VERTEX_POINT ( 'NONE', #45643 ) ;
#27241=ORIENTED_EDGE ( 'NONE', *, *, #42193, .F. ) ;
#27242=DIRECTION ( 'NONE',  ( -0.9660698163281072892, -0.2582810677919976650, 5.363434502754641456E-08 ) ) ;
#27243=PRESENTATION_STYLE_ASSIGNMENT (( #38558 ) ) ;
#27244=CARTESIAN_POINT ( 'NONE',  ( -16.57554779340669882, -22.21081089906203943, 65.41059674993448425 ) ) ;
#27245=CARTESIAN_POINT ( 'NONE',  ( -21.22399696191457252, -8.930295582149165412, 73.82801983812771596 ) ) ;
#27247=CARTESIAN_POINT ( 'NONE',  ( -10.43125871347677958, -13.91323993190135155, 57.59825034919892772 ) ) ;
#27251=EDGE_CURVE ( 'NONE', #46448, #32393, #40463, .T. ) ;
#27252=CARTESIAN_POINT ( 'NONE',  ( -10.41614636368765900, -13.97037319380632248, 64.53236772669211518 ) ) ;
#27253=CARTESIAN_POINT ( 'NONE',  ( -21.01047406150117070, -21.33922706731038232, 62.22197251680120189 ) ) ;
#27254=CARTESIAN_POINT ( 'NONE',  ( -21.53009576834440608, -9.139789435051676847, 70.13132584627037147 ) ) ;
#27258=VERTEX_POINT ( 'NONE', #15556 ) ;
#27259=CARTESIAN_POINT ( 'NONE',  ( -14.73525069530193399, -21.75714069359356984, 61.89246344873641448 ) ) ;
#27260=CARTESIAN_POINT ( 'NONE',  ( -10.37462438995674319, -14.89569194323783030, 74.79778901495059529 ) ) ;
#27263=EDGE_LOOP ( 'NONE', ( #43927, #36282, #30512, #31441, #33344 ) ) ;
#27265=DIRECTION ( 'NONE',  ( 0.9562635972186038780, -0.2925062950340272527, 4.666065131241567634E-08 ) ) ;
#27266=EDGE_CURVE ( 'NONE', #30119, #30489, #44848, .T. ) ;
#27268=CARTESIAN_POINT ( 'NONE',  ( -12.98444386793654459, -9.332658658743872238, 70.84925372438172531 ) ) ;
#27269=ORIENTED_EDGE ( 'NONE', *, *, #39329, .F. ) ;
#27270=CARTESIAN_POINT ( 'NONE',  ( -10.44050833889757079, -15.30664536039409107, 57.63963066593323248 ) ) ;
#27271=( BOUNDED_CURVE ( )  B_SPLINE_CURVE ( 3, ( #25655, #7699, #37706, #3999 ),
 .UNSPECIFIED., .F., .F. ) 
 B_SPLINE_CURVE_WITH_KNOTS ( ( 4, 4 ),
 ( 4.712388980384689674, 4.921828490624009511 ),
 .UNSPECIFIED. ) 
 CURVE ( )  GEOMETRIC_REPRESENTATION_ITEM ( )  RATIONAL_B_SPLINE_CURVE ( ( 1.000000000000000000, 0.9963479302455154896, 0.9963479302455154896, 1.000000000000000000 ) ) 
 REPRESENTATION_ITEM ( '' )  );
#27272=CARTESIAN_POINT ( 'NONE',  ( -11.46876066122178095, -18.48806595306161071, 61.57710833523393035 ) ) ;
#27275=ORIENTED_EDGE ( 'NONE', *, *, #32515, .T. ) ;
#27276=CARTESIAN_POINT ( 'NONE',  ( -15.15660932275500095, -21.48492473237050859, 65.39124617759186719 ) ) ;
#27277=EDGE_CURVE ( 'NONE', #14849, #6686, #43267, .T. ) ;
#27278=EDGE_CURVE ( 'NONE', #41019, #918, #16285, .T. ) ;
#27280=ORIENTED_EDGE ( 'NONE', *, *, #37204, .F. ) ;
#27281=CARTESIAN_POINT ( 'NONE',  ( -22.22034002972690203, -20.51002343881169665, 58.95717044630308123 ) ) ;
#27282=CARTESIAN_POINT ( 'NONE',  ( -24.47273122526617684, -14.66856428242425636, 62.71296483725149784 ) ) ;
#27283=CARTESIAN_POINT ( 'NONE',  ( -22.22619444978876757, -20.50513558618911958, 58.94938304221643222 ) ) ;
#27284=ORIENTED_EDGE ( 'NONE', *, *, #24754, .T. ) ;
#27285=FACE_OUTER_BOUND ( 'NONE', #12020, .T. ) ;
#27287=PLANE ( 'NONE',  #46402 ) ;
#27288=CARTESIAN_POINT ( 'NONE',  ( -11.17692863878522225, -11.53409247417484274, 71.18040941340760241 ) ) ;
#27290=CARTESIAN_POINT ( 'NONE',  ( -15.75283698213507755, -7.548994588147243334, 67.32502552484606895 ) ) ;
#27291=( BOUNDED_SURFACE ( )  B_SPLINE_SURFACE ( 3, 1, ( 
 ( #43085, #35925 ),
 ( #17208, #5427 ),
 ( #42369, #39396 ),
 ( #35679, #23663 ),
 ( #24632, #34959 ),
 ( #24139, #39634 ),
 ( #5678, #47020 ) ),
 .UNSPECIFIED., .T., .F., .F. ) 
 B_SPLINE_SURFACE_WITH_KNOTS ( ( 4, 3, 4 ),
 ( 2, 2 ),
 ( 0.000000000000000000, 0.5000000000000000000, 1.000000000000000000 ),
 ( 0.000000000000000000, 1.000000000000000000 ),
 .UNSPECIFIED. ) 
 GEOMETRIC_REPRESENTATION_ITEM ( )  RATIONAL_B_SPLINE_SURFACE ( (
 ( 1.000000000000000000, 1.000000000000000000),
 ( 0.3333333333333335369, 0.3333333333333330373),
 ( 0.3333333333333335369, 0.3333333333333330373),
 ( 1.000000000000000000, 1.000000000000000000),
 ( 0.3333333333333333703, 0.3333333333333333703),
 ( 0.3333333333333333703, 0.3333333333333333703),
 ( 1.000000000000000000, 1.000000000000000000) ) ) 
 REPRESENTATION_ITEM ( '' )  SURFACE ( )  );
#27293=CARTESIAN_POINT ( 'NONE',  ( -11.46028008028683942, -18.56947564720590194, 61.56238700194530367 ) ) ;
#27294=EDGE_CURVE ( 'NONE', #13075, #7864, #6152, .T. ) ;
#27296=EDGE_LOOP ( 'NONE', ( #6169, #19877 ) ) ;
#27297=CARTESIAN_POINT ( 'NONE',  ( -10.48245837418595805, -15.71172178951755427, 61.05291461354959637 ) ) ;
#27302=CARTESIAN_POINT ( 'NONE',  ( -12.41955227442780263, -9.914691306276559146, 57.08935537464338239 ) ) ;
#27304=CARTESIAN_POINT ( 'NONE',  ( -19.78779399205855327, -21.87446732333777888, 65.60339696459925563 ) ) ;
#27306=VERTEX_POINT ( 'NONE', #2010 ) ;
#27308=LINE ( 'NONE', #39110, #4540 ) ;
#27309=CARTESIAN_POINT ( 'NONE',  ( -13.59294679993987565, -20.73687756253419678, 68.60058253670568718 ) ) ;
#27310=FACE_OUTER_BOUND ( 'NONE', #34628, .T. ) ;
#27311=B_SPLINE_CURVE_WITH_KNOTS ( 'NONE', 3,
 ( #179, #3605, #18607, #48662, #22828, #34122, #15393, #27952, #8285, #34855 ),
 .UNSPECIFIED., .F., .F.,
 ( 4, 2, 2, 2, 4 ),
 ( 0.000000000000000000, 0.2500000000000000000, 0.5000000000000000000, 0.7500000000000000000, 1.000000000000000000 ),
 .UNSPECIFIED. ) ;
#27312=ORIENTED_EDGE ( 'NONE', *, *, #17868, .T. ) ;
#27313=ORIENTED_EDGE ( 'NONE', *, *, #9889, .T. ) ;
#27315=CARTESIAN_POINT ( 'NONE',  ( -23.42915847708036381, -11.11517115755410146, 73.64721174900437006 ) ) ;
#27316=CARTESIAN_POINT ( 'NONE',  ( -14.97414238684038068, -21.84485642299321029, 65.30585465654563393 ) ) ;
#27317=CARTESIAN_POINT ( 'NONE',  ( -24.48759320265496342, -17.17788619462897159, 72.92690118282537526 ) ) ;
#27318=ORIENTED_EDGE ( 'NONE', *, *, #42818, .F. ) ;
#27319=CARTESIAN_POINT ( 'NONE',  ( -24.44689184067228638, -14.18710713894228093, 69.93803194250310185 ) ) ;
#27321=VECTOR ( 'NONE', #7480, 1000.000000000000000 ) ;
#27322=CARTESIAN_POINT ( 'NONE',  ( -19.25861376934618363, -8.001921477138727923, 60.25533195930442787 ) ) ;
#27323=EDGE_CURVE ( 'NONE', #14849, #313, #6372, .T. ) ;
#27324=ORIENTED_EDGE ( 'NONE', *, *, #13860, .F. ) ;
#27326=CARTESIAN_POINT ( 'NONE',  ( -22.27817919856018136, -9.157513542003881568, 59.83675792137641736 ) ) ;
#27327=CARTESIAN_POINT ( 'NONE',  ( -24.23444832799638604, -16.42945440209323849, 59.13949121896713024 ) ) ;
#27329=CARTESIAN_POINT ( 'NONE',  ( -23.67513346179213940, -18.86224369876040896, 69.49383191692929529 ) ) ;
#27330=EDGE_LOOP ( 'NONE', ( #15247, #6029, #21466, #24364, #1402 ) ) ;
#27333=CARTESIAN_POINT ( 'NONE',  ( -11.63929734443426867, -10.76555703936739938, 57.35336384308645563 ) ) ;
#27334=ORIENTED_EDGE ( 'NONE', *, *, #23442, .F. ) ;
#27335=CARTESIAN_POINT ( 'NONE',  ( -23.85820194903862657, -17.69173191509663923, 62.48833042115953873 ) ) ;
#27337=EDGE_CURVE ( 'NONE', #15639, #7607, #32289, .T. ) ;
#27339=CYLINDRICAL_SURFACE ( 'NONE', #45685, 0.1500000000000007161 ) ;
#27340=EDGE_CURVE ( 'NONE', #8650, #11545, #9893, .T. ) ;
#27341=CARTESIAN_POINT ( 'NONE',  ( -10.49189908542464522, -16.09426454567519116, 68.26295692486267797 ) ) ;
#27343=CARTESIAN_POINT ( 'NONE',  ( -10.44202790750644461, -14.30845231023897846, 64.38803863533676974 ) ) ;
#27344=CARTESIAN_POINT ( 'NONE',  ( -11.51414000101334345, -10.27201461766008350, 74.62540520127058130 ) ) ;
#27345=CARTESIAN_POINT ( 'NONE',  ( -23.12302755141047683, -18.95946607990388699, 62.50406880580509750 ) ) ;
#27346=DIRECTION ( 'NONE',  ( -0.8398192074808118468, -0.5428661886195298436, -7.907900705248004564E-08 ) ) ;
#27347=DIRECTION ( 'NONE',  ( 0.4408917724886829981, 0.07492959997082451751, 0.8944271909999156334 ) ) ;
#27348=ORIENTED_EDGE ( 'NONE', *, *, #7033, .F. ) ;
#27349=ORIENTED_EDGE ( 'NONE', *, *, #8722, .F. ) ;
#27350=DIRECTION ( 'NONE',  ( -0.09077643883959130022, 0.9958712959773466933, 4.338678762321648003E-08 ) ) ;
#27351=CARTESIAN_POINT ( 'NONE',  ( -14.60479746972646886, -7.913168098764732150, 60.50491608655884335 ) ) ;
#27352=EDGE_LOOP ( 'NONE', ( #44455, #13670, #41420, #35873, #20379 ) ) ;
#27354=CARTESIAN_POINT ( 'NONE',  ( -22.53538519471304369, -20.22938801946909138, 65.74775819791243237 ) ) ;
#27355=CARTESIAN_POINT ( 'NONE',  ( -16.37525608968913460, -22.18513123027473455, 61.87755341768041717 ) ) ;
#27357=CARTESIAN_POINT ( 'NONE',  ( -17.24064252496611971, -7.811500653502258196, 70.49035835121620153 ) ) ;
#27359=CARTESIAN_POINT ( 'NONE',  ( -12.28547924108692335, -10.05564394636707348, 60.85918091186046297 ) ) ;
#27361=CARTESIAN_POINT ( 'NONE',  ( -20.34748183946319244, -8.389919497863246534, 63.51941420704543617 ) ) ;
#27366=CARTESIAN_POINT ( 'NONE',  ( -23.30132152709437676, -10.22970227413176580, 63.25841351925517841 ) ) ;
#27367=AXIS2_PLACEMENT_3D ( 'NONE', #27345, #15763, #4955 ) ;
#27368=CARTESIAN_POINT ( 'NONE',  ( -17.67039273561237778, -7.813102812166079936, 63.56673625629110091 ) ) ;
#27369=CARTESIAN_POINT ( 'NONE',  ( -12.28060247932822691, -9.983304365141403736, 64.44402973226354447 ) ) ;
#27370=VECTOR ( 'NONE', #38176, 1000.000000000000114 ) ;
#27371=ORIENTED_EDGE ( 'NONE', *, *, #20054, .F. ) ;
#27372=ORIENTED_EDGE ( 'NONE', *, *, #10032, .T. ) ;
#27374=VERTEX_POINT ( 'NONE', #35728 ) ;
#27376=CARTESIAN_POINT ( 'NONE',  ( -18.46801905451614445, -7.836623195388688679, 74.12592262855558545 ) ) ;
#27377=EDGE_CURVE ( 'NONE', #16726, #21204, #1139, .T. ) ;
#27378=ORIENTED_EDGE ( 'NONE', *, *, #34087, .T. ) ;
#27379=CARTESIAN_POINT ( 'NONE',  ( -21.89826351590202336, -8.852228842849337198, 66.84645279485334868 ) ) ;
#27380=CARTESIAN_POINT ( 'NONE',  ( -18.30607514908327715, -7.810853278037157565, 73.84064121929586122 ) ) ;
#27381=ORIENTED_EDGE ( 'NONE', *, *, #44078, .T. ) ;
#27382=CARTESIAN_POINT ( 'NONE',  ( -13.89248387370423110, -21.36903859207333412, 71.96961763246901000 ) ) ;
#27383=AXIS2_PLACEMENT_3D ( 'NONE', #24983, #28676, #46903 ) ;
#27384=CARTESIAN_POINT ( 'NONE',  ( -23.83833616213321704, -17.61232902345998141, 62.77360984984811410 ) ) ;
#27385=VECTOR ( 'NONE', #4716, 1000.000000000000227 ) ;
#27386=B_SPLINE_CURVE_WITH_KNOTS ( 'NONE', 1,
 ( #8941, #31821 ),
 .UNSPECIFIED., .F., .F.,
 ( 2, 2 ),
 ( 0.000000000000000000, 1.000000000000000000 ),
 .UNSPECIFIED. ) ;
#27387=VERTEX_POINT ( 'NONE', #8931 ) ;
#27388=CARTESIAN_POINT ( 'NONE',  ( -19.97164249076357478, -21.81019033462135326, 69.11977790463622284 ) ) ;
#27389=CARTESIAN_POINT ( 'NONE',  ( -23.92719435707370224, -11.17417392741853988, 70.00715344888816105 ) ) ;
#27390=AXIS2_PLACEMENT_3D ( 'NONE', #43766, #25046, #31942 ) ;
#27391=ORIENTED_EDGE ( 'NONE', *, *, #21422, .T. ) ;
#27392=CARTESIAN_POINT ( 'NONE',  ( -21.78913961794832588, -8.771810275399618106, 70.24637145832762997 ) ) ;
#27394=CARTESIAN_POINT ( 'NONE',  ( -10.93120642218817729, -11.15588000066243168, 64.27165164367140449 ) ) ;
#27396=FACE_OUTER_BOUND ( 'NONE', #9482, .T. ) ;
#27398=EDGE_CURVE ( 'NONE', #27387, #45387, #23950, .T. ) ;
#27399=LINE ( 'NONE', #5006, #45519 ) ;
#27400=CARTESIAN_POINT ( 'NONE',  ( -10.55151165865014384, -17.68520938540437371, 68.28217272534745064 ) ) ;
#27402=CARTESIAN_POINT ( 'NONE',  ( -10.41794148240616735, -15.59560519520519151, 61.04348844167599708 ) ) ;
#27403=CARTESIAN_POINT ( 'NONE',  ( -10.76763535483202539, -17.13171813241336494, 61.30743118825921556 ) ) ;
#27405=EDGE_CURVE ( 'NONE', #21373, #44738, #30463, .T. ) ;
#27406=CARTESIAN_POINT ( 'NONE',  ( -22.42594789675818845, -19.77792426076253918, 69.45945937764655298 ) ) ;
#27408=ORIENTED_EDGE ( 'NONE', *, *, #4177, .F. ) ;
#27409=DIRECTION ( 'NONE',  ( -9.880513536971593873E-06, -1.241746728590076822E-06, 0.9999999999504166626 ) ) ;
#27410=DIRECTION ( 'NONE',  ( -1.140458109893898545E-06, -1.256740822519431765E-06, 0.9999999999985598187 ) ) ;
#27411=VERTEX_POINT ( 'NONE', #20497 ) ;
#27412=CARTESIAN_POINT ( 'NONE',  ( -24.38078725910958866, -15.95265972659957576, 66.36324896149729113 ) ) ;
#27413=CARTESIAN_POINT ( 'NONE',  ( -12.55198883488284878, -12.25722835735234639, 53.49999999999995026 ) ) ;
#27414=CARTESIAN_POINT ( 'NONE',  ( -24.43362360091611052, -14.05489060867666673, 73.42271507725003232 ) ) ;
#27415=CARTESIAN_POINT ( 'NONE',  ( -24.33677527904861648, -16.19409071606989414, 62.59328707532291247 ) ) ;
#27416=ADVANCED_FACE ( 'NONE', ( #35497 ), #6444, .F. ) ;
#27417=( BOUNDED_SURFACE ( )  B_SPLINE_SURFACE ( 3, 1, ( 
 ( #13921, #21591 ),
 ( #36570, #32661 ),
 ( #10271, #2383 ),
 ( #25287, #36819 ),
 ( #43762, #44254 ),
 ( #17864, #28495 ),
 ( #32888, #10016 ) ),
 .UNSPECIFIED., .T., .F., .F. ) 
 B_SPLINE_SURFACE_WITH_KNOTS ( ( 4, 3, 4 ),
 ( 2, 2 ),
 ( 0.000000000000000000, 0.5000000000000000000, 1.000000000000000000 ),
 ( 0.000000000000000000, 1.000000000000000000 ),
 .UNSPECIFIED. ) 
 GEOMETRIC_REPRESENTATION_ITEM ( )  RATIONAL_B_SPLINE_SURFACE ( (
 ( 1.000000000000000000, 1.000000000000000000),
 ( 0.3333333333333335369, 0.3333333333333330373),
 ( 0.3333333333333335369, 0.3333333333333330373),
 ( 1.000000000000000000, 1.000000000000000000),
 ( 0.3333333333333333703, 0.3333333333333333703),
 ( 0.3333333333333333703, 0.3333333333333333703),
 ( 1.000000000000000000, 1.000000000000000000) ) ) 
 REPRESENTATION_ITEM ( '' )  SURFACE ( )  );
#27418=ORIENTED_EDGE ( 'NONE', *, *, #24669, .F. ) ;
#27419=CARTESIAN_POINT ( 'NONE',  ( -24.80865520860317730, -15.79540089610985021, 69.65494700136302697 ) ) ;
#27420=CARTESIAN_POINT ( 'NONE',  ( -10.05839037049808127, -15.92727522337501611, 64.55125644017783770 ) ) ;
#27421=CARTESIAN_POINT ( 'NONE',  ( -10.08432996298220630, -16.08613878457147450, 68.07793591119110488 ) ) ;
#27422=ORIENTED_EDGE ( 'NONE', *, *, #30013, .T. ) ;
#27423=CARTESIAN_POINT ( 'NONE',  ( -17.79084047922378531, -7.768752242298102573, 60.23060768310389790 ) ) ;
#27424=VECTOR ( 'NONE', #8944, 1000.000000000000000 ) ;
#27425=CARTESIAN_POINT ( 'NONE',  ( -24.38903048123337314, -17.45395020021824450, 69.55306401233070801 ) ) ;
#27426=VECTOR ( 'NONE', #28408, 1000.000000000000000 ) ;
#27429=CARTESIAN_POINT ( 'NONE',  ( -19.24025795797341942, -7.996846695050864540, 60.24620885950562865 ) ) ;
#27430=( BOUNDED_CURVE ( )  B_SPLINE_CURVE ( 3, ( #3007, #47832, #33035, #29123 ),
 .UNSPECIFIED., .F., .F. ) 
 B_SPLINE_CURVE_WITH_KNOTS ( ( 4, 4 ),
 ( 0.5000000000000000000, 0.9074455897393701731 ),
 .UNSPECIFIED. ) 
 CURVE ( )  GEOMETRIC_REPRESENTATION_ITEM ( )  RATIONAL_B_SPLINE_CURVE ( ( 0.9999999999999942268, 0.4567392136813220871, 0.3561768502900305444, 0.6983129098261133816 ) ) 
 REPRESENTATION_ITEM ( '' )  );
#27431=ORIENTED_EDGE ( 'NONE', *, *, #40842, .F. ) ;
#27432=ORIENTED_EDGE ( 'NONE', *, *, #36789, .T. ) ;
#27434=CARTESIAN_POINT ( 'NONE',  ( -19.17437844398820701, -7.979623566120205957, 63.44561363416070776 ) ) ;
#27435=CARTESIAN_POINT ( 'NONE',  ( -19.17604249790256077, -21.63836284480991878, 58.53979515915469278 ) ) ;
#27436=VECTOR ( 'NONE', #46675, 1000.000000000000114 ) ;
#27437=ADVANCED_FACE ( 'NONE', ( #36932 ), #17502, .F. ) ;
#27438=( BOUNDED_CURVE ( )  B_SPLINE_CURVE ( 3, ( #48515, #17506, #32537, #33475 ),
 .UNSPECIFIED., .F., .F. ) 
 B_SPLINE_CURVE_WITH_KNOTS ( ( 4, 4 ),
 ( 0.5000000000000000000, 0.9074455897393645110 ),
 .UNSPECIFIED. ) 
 CURVE ( )  GEOMETRIC_REPRESENTATION_ITEM ( )  RATIONAL_B_SPLINE_CURVE ( ( 1.000000000000020428, 0.4567392136813446801, 0.3561768502900207189, 0.6983129098260705270 ) ) 
 REPRESENTATION_ITEM ( '' )  );
#27439=CARTESIAN_POINT ( 'NONE',  ( -10.77075464306150110, -16.98888295467523335, 61.22913362936283477 ) ) ;
#27440=CARTESIAN_POINT ( 'NONE',  ( -20.81971067820157728, -8.177204663279967534, 59.95469905373763453 ) ) ;
#27441=CARTESIAN_POINT ( 'NONE',  ( -9.979603264230430426, -14.52052340097724148, 68.04295441848455539 ) ) ;
#27442=CARTESIAN_POINT ( 'NONE',  ( -18.19230087906959170, -22.21957251972233749, 65.38886231616686473 ) ) ;
#27444=CARTESIAN_POINT ( 'NONE',  ( -22.45002512565393005, -19.68157916873682467, 69.28304101961816741 ) ) ;
#27445=EDGE_CURVE ( 'NONE', #10296, #26347, #12825, .T. ) ;
#27446=CARTESIAN_POINT ( 'NONE',  ( -20.37299732318518508, -8.405577239842552117, 66.93104082189577753 ) ) ;
#27448=CARTESIAN_POINT ( 'NONE',  ( -18.11889279746774051, -21.82488571228486052, 65.49532159284275679 ) ) ;
#27449=CARTESIAN_POINT ( 'NONE',  ( -9.974122264712642405, -14.85722068285092057, 74.92062023727633857 ) ) ;
#27450=ORIENTED_EDGE ( 'NONE', *, *, #18188, .T. ) ;
#27453=CIRCLE ( 'NONE', #14070, 7.500000000000002665 ) ;
#27454=CARTESIAN_POINT ( 'NONE',  ( -11.76425449931685030, -10.60075661872682140, 70.85404331479517737 ) ) ;
#27455=CARTESIAN_POINT ( 'NONE',  ( -10.33431723597471930, -12.52035407725662886, 60.98348989824278732 ) ) ;
#27458=CARTESIAN_POINT ( 'NONE',  ( -22.00903739223959477, -8.936221312270376416, 63.30498424023031845 ) ) ;
#27459=PLANE ( 'NONE',  #37594 ) ;
#27460=AXIS2_PLACEMENT_3D ( 'NONE', #26142, #15272, #30820 ) ;
#27461=VECTOR ( 'NONE', #37020, 1000.000000000000000 ) ;
#27462=CARTESIAN_POINT ( 'NONE',  ( -23.62389146642398075, -18.18225743695742835, 72.91935080803692415 ) ) ;
#27463=FACE_BOUND ( 'NONE', #1759, .T. ) ;
#27466=CARTESIAN_POINT ( 'NONE',  ( -11.43691971525006679, -18.43613410775878236, 58.03387880510997121 ) ) ;
#27467=EDGE_CURVE ( 'NONE', #38209, #43090, #44592, .T. ) ;
#27469=EDGE_LOOP ( 'NONE', ( #46440, #33750, #3300, #2480, #40422 ) ) ;
#27470=AXIS2_PLACEMENT_3D ( 'NONE', #1297, #42921, #42194 ) ;
#27471=ADVANCED_FACE ( 'NONE', ( #14030 ), #17260, .T. ) ;
#27473=CARTESIAN_POINT ( 'NONE',  ( -11.41592704872699748, -19.21438508446953364, 71.94331831479362904 ) ) ;
#27474=CARTESIAN_POINT ( 'NONE',  ( -11.99264457154321484, -10.30873963881685285, 64.02914301436621258 ) ) ;
#27475=ORIENTED_EDGE ( 'NONE', *, *, #35235, .T. ) ;
#27477=FACE_BOUND ( 'NONE', #28782, .T. ) ;
#27478=EDGE_LOOP ( 'NONE', ( #13229, #48093, #45863, #21552, #13903 ) ) ;
#27479=VERTEX_POINT ( 'NONE', #32533 ) ;
#27480=VERTEX_POINT ( 'NONE', #40401 ) ;
#27481=CARTESIAN_POINT ( 'NONE',  ( -10.61330293760801879, -12.98832031645814844, 67.88832347272310130 ) ) ;
#27482=CARTESIAN_POINT ( 'NONE',  ( -16.07284047765482882, -7.413310693310465993, 54.02312124697527906 ) ) ;
#27485=CARTESIAN_POINT ( 'NONE',  ( -10.64854695470030599, -12.86019059820356958, 64.55364013863997741 ) ) ;
#27486=CARTESIAN_POINT ( 'NONE',  ( -10.70785621775489993, -16.78775467540145527, 57.87687636479810749 ) ) ;
#27487=EDGE_CURVE ( 'NONE', #16763, #26691, #48270, .T. ) ;
#27490=B_SPLINE_CURVE_WITH_KNOTS ( 'NONE', 3,
 ( #16139, #2109, #32159, #9756, #46456, #27486, #27966, #39777, #23811, #12712 ),
 .UNSPECIFIED., .F., .F.,
 ( 4, 2, 2, 2, 4 ),
 ( 0.000000000000000000, 0.2500000000000000000, 0.5000000000000000000, 0.7500000000000000000, 1.000000000000000000 ),
 .UNSPECIFIED. ) ;
#27492=EDGE_CURVE ( 'NONE', #38648, #41019, #1392, .T. ) ;
#27493=EDGE_CURVE ( 'NONE', #18739, #1846, #11197, .T. ) ;
#27494=CARTESIAN_POINT ( 'NONE',  ( -24.00983782305545233, -11.32632323363204385, 66.57214513468635175 ) ) ;
#27496=CARTESIAN_POINT ( 'NONE',  ( -10.72552559342236833, -12.61109755851567549, 60.94853568372188590 ) ) ;
#27497=CARTESIAN_POINT ( 'NONE',  ( -10.56492563526530759, -13.18000101695786341, 71.20828586226983248 ) ) ;
#27498=EDGE_LOOP ( 'NONE', ( #38754, #42846 ) ) ;
#27501=EDGE_LOOP ( 'NONE', ( #48151, #37121 ) ) ;
#27502=CARTESIAN_POINT ( 'NONE',  ( -12.43154959716778940, -9.826441625128287782, 60.65098055540761379 ) ) ;
#27506=EDGE_LOOP ( 'NONE', ( #32904, #35543, #33930, #37293, #43682 ) ) ;
#27507=CARTESIAN_POINT ( 'NONE',  ( -22.05757754724333353, -8.975236167248709762, 63.36870640580771408 ) ) ;
#27511=CARTESIAN_POINT ( 'NONE',  ( -12.26315819337278334, -19.61226149452583911, 58.22122601348936399 ) ) ;
#27512=CARTESIAN_POINT ( 'NONE',  ( -22.96484330895583881, -19.08706763331013434, 59.18410642315183878 ) ) ;
#27514=ORIENTED_EDGE ( 'NONE', *, *, #24002, .T. ) ;
#27515=DIRECTION ( 'NONE',  ( -0.6827297667453423591, -0.7306709694519486487, -5.176517812513565093E-09 ) ) ;
#27516=VERTEX_POINT ( 'NONE', #14272 ) ;
#27517=CARTESIAN_POINT ( 'NONE',  ( -9.974229878692264961, -14.74184183210034149, 71.48816083323411874 ) ) ;
#27518=CARTESIAN_POINT ( 'NONE',  ( -14.91112529534803066, -8.221969756899694559, 57.13527940342243028 ) ) ;
#27522=CARTESIAN_POINT ( 'NONE',  ( -12.50766578132126483, -19.86205079821699115, 65.16674886870754335 ) ) ;
#27526=EDGE_LOOP ( 'NONE', ( #34758, #5611, #29167, #12116, #30397 ) ) ;
#27527=CARTESIAN_POINT ( 'NONE',  ( -23.89081516821958218, -17.62458393556817171, 58.88889748697027926 ) ) ;
#27528=AXIS2_PLACEMENT_3D ( 'NONE', #26863, #19456, #12792 ) ;
#27529=CARTESIAN_POINT ( 'NONE',  ( -15.12070311848097859, -21.89431190412215145, 68.75405669007906795 ) ) ;
#27530=CARTESIAN_POINT ( 'NONE',  ( -12.16129776675651897, -10.11277993467359337, 67.59076956020265925 ) ) ;
#27531=CARTESIAN_POINT ( 'NONE',  ( -22.28350170462084989, -9.162040689504776125, 59.89983962365610637 ) ) ;
#27532=ORIENTED_EDGE ( 'NONE', *, *, #43199, .T. ) ;
#27533=LINE ( 'NONE', #19909, #30267 ) ;
#27534=VECTOR ( 'NONE', #10956, 1000.000000000000000 ) ;
#27535=B_SPLINE_CURVE_WITH_KNOTS ( 'NONE', 3,
 ( #20989, #28621, #31593, #23968, #38971, #5247, #12864, #42917, #9189, #39216 ),
 .UNSPECIFIED., .F., .F.,
 ( 4, 2, 2, 2, 4 ),
 ( 0.000000000000000000, 0.2500000000000000000, 0.5000000000000000000, 0.7500000000000000000, 1.000000000000000000 ),
 .UNSPECIFIED. ) ;
#27536=CARTESIAN_POINT ( 'NONE',  ( -24.73185694657778910, -16.25806987106194512, 62.79339884040287245 ) ) ;
#27537=VERTEX_POINT ( 'NONE', #43632 ) ;
#27538=ORIENTED_EDGE ( 'NONE', *, *, #29312, .T. ) ;
#27539=CARTESIAN_POINT ( 'NONE',  ( -24.84681873822328413, -14.17034522304293098, 69.79128769184926284 ) ) ;
#27540=CARTESIAN_POINT ( 'NONE',  ( -13.54893327507986456, -8.910214905335239521, 64.05379690000981441 ) ) ;
#27544=CARTESIAN_POINT ( 'NONE',  ( -12.34408071644948279, -9.993246969730000373, 57.28038814785139010 ) ) ;
#27545=CARTESIAN_POINT ( 'NONE',  ( -12.37192322991513471, -19.65436620064385664, 58.11785611954050523 ) ) ;
#27546=CARTESIAN_POINT ( 'NONE',  ( -24.85359113602694237, -14.25571898851532460, 69.76779851910008290 ) ) ;
#27547=EDGE_CURVE ( 'NONE', #43778, #30777, #36906, .T. ) ;
#27550=ORIENTED_EDGE ( 'NONE', *, *, #20559, .T. ) ;
#27551=CARTESIAN_POINT ( 'NONE',  ( -11.08030728566740741, -11.72680384936461806, 74.97328630331448096 ) ) ;
#27552=EDGE_CURVE ( 'NONE', #3552, #35369, #39921, .T. ) ;
#27553=EDGE_CURVE ( 'NONE', #45387, #11424, #38532, .T. ) ;
#27555=CARTESIAN_POINT ( 'NONE',  ( -23.67460905091340706, -11.65500745809028338, 66.49384777452590356 ) ) ;
#27556=CARTESIAN_POINT ( 'NONE',  ( -24.54463936542308744, -12.61820580661037106, 69.87219370530908691 ) ) ;
#27557=CARTESIAN_POINT ( 'NONE',  ( -23.88415217903649079, -17.63235132829416685, 62.77360984996715842 ) ) ;
#27559=EDGE_LOOP ( 'NONE', ( #42680, #31137, #19169, #11642, #36063 ) ) ;
#27561=CYLINDRICAL_SURFACE ( 'NONE', #47318, 0.1499999999999974132 ) ;
#27565=( BOUNDED_CURVE ( )  B_SPLINE_CURVE ( 3, ( #4166, #7863, #45287, #7371 ),
 .UNSPECIFIED., .F., .F. ) 
 B_SPLINE_CURVE_WITH_KNOTS ( ( 4, 4 ),
 ( 0.5000000000000000000, 0.9074455897393631787 ),
 .UNSPECIFIED. ) 
 CURVE ( )  GEOMETRIC_REPRESENTATION_ITEM ( )  RATIONAL_B_SPLINE_CURVE ( ( 1.000000000000017319, 0.4567392136813416825, 0.3561768502900215516, 0.6983129098260758560 ) ) 
 REPRESENTATION_ITEM ( '' )  );
#27566=ORIENTED_EDGE ( 'NONE', *, *, #22503, .T. ) ;
#27567=VECTOR ( 'NONE', #46757, 1000.000000000000114 ) ;
#27568=CARTESIAN_POINT ( 'NONE',  ( -24.42549660922115251, -13.91739599595199728, 69.80842429065324950 ) ) ;
#27572=AXIS2_PLACEMENT_3D ( 'NONE', #5990, #43925, #36491 ) ;
#27575=ORIENTED_EDGE ( 'NONE', *, *, #385, .F. ) ;
#27576=CARTESIAN_POINT ( 'NONE',  ( -23.70015292207183322, -18.82353835121273988, 69.47867366044893345 ) ) ;
#27577=( BOUNDED_SURFACE ( )  B_SPLINE_SURFACE ( 3, 1, ( 
 ( #6220, #17531 ),
 ( #21244, #9442 ),
 ( #36243, #46860 ),
 ( #2525, #43421 ),
 ( #20522, #32081 ),
 ( #35525, #9687 ),
 ( #35754, #1800 ) ),
 .UNSPECIFIED., .T., .F., .F. ) 
 B_SPLINE_SURFACE_WITH_KNOTS ( ( 4, 3, 4 ),
 ( 2, 2 ),
 ( 0.000000000000000000, 0.5000000000000000000, 1.000000000000000000 ),
 ( 0.000000000000000000, 1.000000000000000000 ),
 .UNSPECIFIED. ) 
 GEOMETRIC_REPRESENTATION_ITEM ( )  RATIONAL_B_SPLINE_SURFACE ( (
 ( 1.000000000000000000, 1.000000000000000000),
 ( 0.3333333333333335369, 0.3333333333333330373),
 ( 0.3333333333333335369, 0.3333333333333330373),
 ( 1.000000000000000000, 1.000000000000000000),
 ( 0.3333333333333333703, 0.3333333333333333703),
 ( 0.3333333333333333703, 0.3333333333333333703),
 ( 1.000000000000000000, 1.000000000000000000) ) ) 
 REPRESENTATION_ITEM ( '' )  SURFACE ( )  );
#27578=ORIENTED_EDGE ( 'NONE', *, *, #28229, .F. ) ;
#27579=EDGE_LOOP ( 'NONE', ( #18140, #29280 ) ) ;
#27580=CARTESIAN_POINT ( 'NONE',  ( -23.74985771237617627, -17.93965049410213197, 62.61793715156320417 ) ) ;
#27581=CARTESIAN_POINT ( 'NONE',  ( -17.98089531606498781, -21.84518143609853524, 68.95947724711012938 ) ) ;
#27585=CARTESIAN_POINT ( 'NONE',  ( -24.47638328979802225, -14.67261064969091322, 66.27472727418629006 ) ) ;
#27587=ORIENTED_EDGE ( 'NONE', *, *, #26873, .F. ) ;
#27588=FACE_OUTER_BOUND ( 'NONE', #14249, .T. ) ;
#27589=CARTESIAN_POINT ( 'NONE',  ( -10.47425521701617157, -17.49314416303823450, 64.81234701634230078 ) ) ;
#27593=CARTESIAN_POINT ( 'NONE',  ( -24.77321845510417830, -16.03108965430551436, 66.26313693903748003 ) ) ;
#27596=AXIS2_PLACEMENT_3D ( 'NONE', #45055, #468, #15446 ) ;
#27597=CARTESIAN_POINT ( 'NONE',  ( -18.18338144371267617, -21.81849904615365432, 65.63060065626805795 ) ) ;
#27600=CARTESIAN_POINT ( 'NONE',  ( -24.35082266418244146, -15.81936897246520957, 66.25427998382291150 ) ) ;
#27602=CARTESIAN_POINT ( 'NONE',  ( -24.37683822056718697, -15.97618770311995640, 66.06324926631656069 ) ) ;
#27603=CARTESIAN_POINT ( 'NONE',  ( -11.24831865710118173, -11.40878463452673053, 64.44882016688482906 ) ) ;
#27604=CARTESIAN_POINT ( 'NONE',  ( -12.28549284030545508, -10.05562942188838704, 60.55918091183862373 ) ) ;
#27605=AXIS2_PLACEMENT_3D ( 'NONE', #23332, #5596, #20115 ) ;
#27607=CARTESIAN_POINT ( 'NONE',  ( -22.42594789675818845, -19.77792426076253918, 69.45945937764655298 ) ) ;
#27610=VECTOR ( 'NONE', #30959, 1000.000000000000227 ) ;
#27611=CARTESIAN_POINT ( 'NONE',  ( -12.30857103994386925, -9.957812909820729530, 60.56477846553902822 ) ) ;
#27613=CARTESIAN_POINT ( 'NONE',  ( -23.12535539932854078, -10.01343808792704237, 66.65686846082743955 ) ) ;
#27614=ORIENTED_EDGE ( 'NONE', *, *, #14486, .T. ) ;
#27616=ADVANCED_FACE ( 'NONE', ( #45328 ), #21266, .T. ) ;
#27617=DIRECTION ( 'NONE',  ( 8.993561279826231301E-07, -8.977735708137639859E-07, -0.9999999999991926458 ) ) ;
#27618=EDGE_CURVE ( 'NONE', #1270, #8865, #13224, .T. ) ;
#27619=ORIENTED_EDGE ( 'NONE', *, *, #38941, .F. ) ;
#27620=CARTESIAN_POINT ( 'NONE',  ( -12.00971705810820467, -9.691755786776280246, 60.67422651510300113 ) ) ;
#27622=EDGE_CURVE ( 'NONE', #26632, #19018, #41974, .T. ) ;
#27623=CARTESIAN_POINT ( 'NONE',  ( -24.07241877824284160, -12.61836747239114409, 69.96346150519261187 ) ) ;
#27625=ORIENTED_EDGE ( 'NONE', *, *, #34075, .T. ) ;
#27627=B_SPLINE_CURVE_WITH_KNOTS ( 'NONE', 1,
 ( #18682, #249 ),
 .UNSPECIFIED., .F., .F.,
 ( 2, 2 ),
 ( 0.000000000000000000, 1.000000000000000000 ),
 .UNSPECIFIED. ) ;
#27629=CARTESIAN_POINT ( 'NONE',  ( -10.39693166811831304, -15.37990016280386918, 57.58264896457095006 ) ) ;
#27631=VERTEX_POINT ( 'NONE', #28050 ) ;
#27632=CARTESIAN_POINT ( 'NONE',  ( -23.14996626141612523, -18.92247510852853765, 62.64847065521940550 ) ) ;
#27633=VERTEX_POINT ( 'NONE', #35193 ) ;
#27634=CARTESIAN_POINT ( 'NONE',  ( -11.32267065936820316, -11.37785446942383949, 64.14882076995250770 ) ) ;
#27636=CARTESIAN_POINT ( 'NONE',  ( -23.59327504554355315, -11.39630409041826020, 69.90682860766239060 ) ) ;
#27637=EDGE_LOOP ( 'NONE', ( #33435, #30048, #5983, #3836, #16691 ) ) ;
#27638=CARTESIAN_POINT ( 'NONE',  ( -24.47304815678895196, -15.04811744431364140, 59.65788834854969735 ) ) ;
#27639=CARTESIAN_POINT ( 'NONE',  ( -12.36794914932409561, -19.72224030764921565, 61.39678633597973345 ) ) ;
#27640=CARTESIAN_POINT ( 'NONE',  ( -19.03984369153074141, -21.67464089235836511, 58.93996235972087305 ) ) ;
#27641=ORIENTED_EDGE ( 'NONE', *, *, #9354, .T. ) ;
#27642=LINE ( 'NONE', #35734, #1079 ) ;
#27645=CARTESIAN_POINT ( 'NONE',  ( -10.78978129071826686, -12.42417052737943095, 57.32857332104951098 ) ) ;
#27648=VERTEX_POINT ( 'NONE', #38396 ) ;
#27649=DIRECTION ( 'NONE',  ( -5.731567514496413899E-31, -1.020425574103664789E-16, -1.000000000000000000 ) ) ;
#27650=PLANE ( 'NONE',  #44734 ) ;
#27651=CARTESIAN_POINT ( 'NONE',  ( -15.89884937297370193, -7.926133255677830114, 67.14007309771254484 ) ) ;
#27654=ORIENTED_EDGE ( 'NONE', *, *, #13657, .T. ) ;
#27655=CARTESIAN_POINT ( 'NONE',  ( -10.42302287260171312, -13.97751933429587012, 57.73352905910142852 ) ) ;
#27656=DIRECTION ( 'NONE',  ( 0.6264825908887947659, -0.7794354131762692983, 3.858680029754496854E-08 ) ) ;
#27659=CARTESIAN_POINT ( 'NONE',  ( -14.98896517277256635, -21.85004359773310156, 65.21258386126636708 ) ) ;
#27660=( BOUNDED_CURVE ( )  B_SPLINE_CURVE ( 3, ( #39590, #5867, #42811, #42586 ),
 .UNSPECIFIED., .F., .F. ) 
 B_SPLINE_CURVE_WITH_KNOTS ( ( 4, 4 ),
 ( 0.4074455897393656767, 0.5000000000000000000 ),
 .UNSPECIFIED. ) 
 CURVE ( )  GEOMETRIC_REPRESENTATION_ITEM ( )  RATIONAL_B_SPLINE_CURVE ( ( 0.6983129098260891787, 0.7760317562606972031, 0.8765941196520016243, 1.000000000000003775 ) ) 
 REPRESENTATION_ITEM ( '' )  );
#27661=CARTESIAN_POINT ( 'NONE',  ( -21.29196722032537537, -20.70380199363843232, 72.53918572867779346 ) ) ;
#27662=CARTESIAN_POINT ( 'NONE',  ( -22.44308142039503906, -9.846875392603276822, 70.16745681354213104 ) ) ;
#27663=CARTESIAN_POINT ( 'NONE',  ( -20.72573862760241070, -8.580110178657996300, 60.14125250079693785 ) ) ;
#27664=EDGE_CURVE ( 'NONE', #30899, #48422, #34430, .T. ) ;
#27665=ORIENTED_EDGE ( 'NONE', *, *, #22655, .F. ) ;
#27666=DIRECTION ( 'NONE',  ( 0.9999889394985579383, 0.004703284017506803583, -7.734398264755851970E-09 ) ) ;
#27667=DIRECTION ( 'NONE',  ( 1.149299188226319421E-05, -1.849289876324834950E-06, 0.9999999999322456423 ) ) ;
#27669=CARTESIAN_POINT ( 'NONE',  ( -11.91307475890685552, -9.794993484201089728, 60.67262835395951015 ) ) ;
#27671=ORIENTED_EDGE ( 'NONE', *, *, #4365, .T. ) ;
#27672=CARTESIAN_POINT ( 'NONE',  ( -11.43788345834500220, -18.53998761144092455, 58.01534399077101511 ) ) ;
#27675=CARTESIAN_POINT ( 'NONE',  ( -17.19811928533322387, -9.313850733363548073, 54.07175714974879099 ) ) ;
#27678=VERTEX_POINT ( 'NONE', #4940 ) ;
#27682=EDGE_CURVE ( 'NONE', #15747, #31661, #41369, .T. ) ;
#27683=CARTESIAN_POINT ( 'NONE',  ( -14.04552000357412211, -8.169287140739843522, 70.92231787642808172 ) ) ;
#27685=EDGE_CURVE ( 'NONE', #22071, #29021, #33824, .T. ) ;
#27686=CARTESIAN_POINT ( 'NONE',  ( -14.20445937233222367, -8.593517467233848350, 70.74460083025394397 ) ) ;
#27689=CARTESIAN_POINT ( 'NONE',  ( -18.92057809895272058, -7.919864474132484844, 66.90071783790342863 ) ) ;
#27690=CARTESIAN_POINT ( 'NONE',  ( -24.23070293473816506, -17.83824296527514264, 62.63507471626854084 ) ) ;
#27691=EDGE_CURVE ( 'NONE', #43420, #40354, #35566, .T. ) ;
#27693=CARTESIAN_POINT ( 'NONE',  ( -23.77562434277295367, -17.86939608417919345, 59.01850491586762359 ) ) ;
#27694=CARTESIAN_POINT ( 'NONE',  ( -17.14068089774974624, -7.813665893538186857, 74.18848128627297456 ) ) ;
#27695=ORIENTED_EDGE ( 'NONE', *, *, #25485, .T. ) ;
#27697=CARTESIAN_POINT ( 'NONE',  ( -12.41310947992116098, -19.76871611099698001, 61.68206578716802113 ) ) ;
#27698=ORIENTED_EDGE ( 'NONE', *, *, #44407, .F. ) ;
#27700=( BOUNDED_SURFACE ( )  B_SPLINE_SURFACE ( 3, 1, ( 
 ( #4135, #41547 ),
 ( #14666, #37583 ),
 ( #41058, #19134 ),
 ( #45747, #26526 ),
 ( #34142, #435 ),
 ( #38078, #18627 ),
 ( #11997, #11266 ) ),
 .UNSPECIFIED., .T., .F., .F. ) 
 B_SPLINE_SURFACE_WITH_KNOTS ( ( 4, 3, 4 ),
 ( 2, 2 ),
 ( 0.000000000000000000, 0.5000000000000000000, 1.000000000000000000 ),
 ( 0.000000000000000000, 1.000000000000000000 ),
 .UNSPECIFIED. ) 
 GEOMETRIC_REPRESENTATION_ITEM ( )  RATIONAL_B_SPLINE_SURFACE ( (
 ( 1.000000000000000000, 1.000000000000000000),
 ( 0.3333333333333335369, 0.3333333333333330373),
 ( 0.3333333333333335369, 0.3333333333333330373),
 ( 1.000000000000000000, 1.000000000000000000),
 ( 0.3333333333333333703, 0.3333333333333333703),
 ( 0.3333333333333333703, 0.3333333333333333703),
 ( 1.000000000000000000, 1.000000000000000000) ) ) 
 REPRESENTATION_ITEM ( '' )  SURFACE ( )  );
#27701=CARTESIAN_POINT ( 'NONE',  ( -19.28352822169459202, -22.07505156356299381, 53.49999999999994316 ) ) ;
#27702=CARTESIAN_POINT ( 'NONE',  ( -22.53422763456337918, -19.59328113293763352, 72.65903032234385250 ) ) ;
#27703=EDGE_LOOP ( 'NONE', ( #28570, #34777, #33198, #36229, #31911 ) ) ;
#27704=CARTESIAN_POINT ( 'NONE',  ( -11.21783165637758550, -18.93062460193366192, 64.93202459354702683 ) ) ;
#27707=CYLINDRICAL_SURFACE ( 'NONE', #28935, 0.1500000000000039913 ) ;
#27708=CARTESIAN_POINT ( 'NONE',  ( -23.04367560227575140, -10.55211830211007218, 59.60203429193362723 ) ) ;
#27709=CARTESIAN_POINT ( 'NONE',  ( -11.46947271230222931, -11.12676175853379412, 60.90715737523439799 ) ) ;
#27710=LINE ( 'NONE', #27228, #12490 ) ;
#27712=CARTESIAN_POINT ( 'NONE',  ( -12.14070192025202743, -10.21533219252760105, 67.72726724898851103 ) ) ;
#27713=VERTEX_POINT ( 'NONE', #31996 ) ;
#27714=CARTESIAN_POINT ( 'NONE',  ( -11.63532267033605372, -18.83847007233952908, 72.10174756685907482 ) ) ;
#27715=CARTESIAN_POINT ( 'NONE',  ( -17.59331747086620013, -7.761237804118463757, 63.85057029381062677 ) ) ;
#27716=ADVANCED_FACE ( 'NONE', ( #35436, #31265 ), #8631, .F. ) ;
#27718=( BOUNDED_CURVE ( )  B_SPLINE_CURVE ( 3, ( #21603, #17875, #32204, #33141 ),
 .UNSPECIFIED., .F., .F. ) 
 B_SPLINE_CURVE_WITH_KNOTS ( ( 4, 4 ),
 ( 0.000000000000000000, 0.4074455897393596815 ),
 .UNSPECIFIED. ) 
 CURVE ( )  GEOMETRIC_REPRESENTATION_ITEM ( )  RATIONAL_B_SPLINE_CURVE ( ( 1.000000000000000000, 0.4567392136813367975, 0.3561768502900320987, 0.6983129098260858481 ) ) 
 REPRESENTATION_ITEM ( '' )  );
#27719=CARTESIAN_POINT ( 'NONE',  ( -21.52725980274252393, -9.076272844571150245, 70.43132538913751262 ) ) ;
#27720=FACE_BOUND ( 'NONE', #39647, .T. ) ;
#27721=ORIENTED_EDGE ( 'NONE', *, *, #8108, .T. ) ;
#27722=VERTEX_POINT ( 'NONE', #31756 ) ;
#27723=ORIENTED_EDGE ( 'NONE', *, *, #40893, .T. ) ;
#27724=CARTESIAN_POINT ( 'NONE',  ( -17.84478125091072087, -22.24806977446377942, 62.06191208170499607 ) ) ;
#27725=FACE_OUTER_BOUND ( 'NONE', #39427, .T. ) ;
#27727=CARTESIAN_POINT ( 'NONE',  ( -12.58533692436079754, -19.86927994801577668, 68.40827630894551703 ) ) ;
#27728=CARTESIAN_POINT ( 'NONE',  ( -22.82405744922300528, -15.92202671434138672, 53.69233794759168887 ) ) ;
#27729=( BOUNDED_SURFACE ( )  B_SPLINE_SURFACE ( 3, 1, ( 
 ( #31676, #42765 ),
 ( #4856, #1873 ),
 ( #9037, #23816 ),
 ( #16146, #20600 ),
 ( #31189, #35598 ),
 ( #16874, #28221 ),
 ( #24053, #43253 ) ),
 .UNSPECIFIED., .T., .F., .F. ) 
 B_SPLINE_SURFACE_WITH_KNOTS ( ( 4, 3, 4 ),
 ( 2, 2 ),
 ( 0.000000000000000000, 0.5000000000000000000, 1.000000000000000000 ),
 ( 0.000000000000000000, 1.000000000000000000 ),
 .UNSPECIFIED. ) 
 GEOMETRIC_REPRESENTATION_ITEM ( )  RATIONAL_B_SPLINE_SURFACE ( (
 ( 1.000000000000000000, 1.000000000000000000),
 ( 0.3333333333333335369, 0.3333333333333330373),
 ( 0.3333333333333335369, 0.3333333333333330373),
 ( 1.000000000000000000, 1.000000000000000000),
 ( 0.3333333333333333703, 0.3333333333333333703),
 ( 0.3333333333333333703, 0.3333333333333333703),
 ( 1.000000000000000000, 1.000000000000000000) ) ) 
 REPRESENTATION_ITEM ( '' )  SURFACE ( )  );
#27732=CARTESIAN_POINT ( 'NONE',  ( -10.35661267713556022, -12.45241038966069347, 60.91358145539074798 ) ) ;
#27733=EDGE_CURVE ( 'NONE', #20377, #39922, #46431, .T. ) ;
#27735=FACE_OUTER_BOUND ( 'NONE', #45928, .T. ) ;
#27736=DIRECTION ( 'NONE',  ( 0.4683180279402422430, -0.8835599723313412035, 4.589753183357165928E-08 ) ) ;
#27739=EDGE_CURVE ( 'NONE', #27062, #383, #31481, .T. ) ;
#27740=CARTESIAN_POINT ( 'NONE',  ( -14.74177589038128033, -21.75963160520128170, 61.82938730834030849 ) ) ;
#27741=CARTESIAN_POINT ( 'NONE',  ( -12.05615996164320691, -19.97535249625256526, 61.51183308442717390 ) ) ;
#27742=CARTESIAN_POINT ( 'NONE',  ( -12.44661323591510715, -19.73288383789282463, 65.09504664347453229 ) ) ;
#27746=CARTESIAN_POINT ( 'NONE',  ( -12.91576191806997365, -9.388722997169709927, 71.13453240065665284 ) ) ;
#27747=CARTESIAN_POINT ( 'NONE',  ( -24.42218830512229388, -14.64588455312011739, 63.01296487252135137 ) ) ;
#27748=CARTESIAN_POINT ( 'NONE',  ( -10.42892865687001169, -14.54580309686654083, 68.15800118612639835 ) ) ;
#27749=CARTESIAN_POINT ( 'NONE',  ( -14.40728840208385542, -7.997212190190129633, 63.96695762048931755 ) ) ;
#27750=VECTOR ( 'NONE', #28175, 1000.000000000000227 ) ;
#27752=DIRECTION ( 'NONE',  ( -0.8017593358536256876, -0.5976470257363775129, 1.209213344977627448E-07 ) ) ;
#27755=CARTESIAN_POINT ( 'NONE',  ( -11.42761092774205345, -18.42145285602150651, 61.56094325674602885 ) ) ;
#27756=ORIENTED_EDGE ( 'NONE', *, *, #42783, .F. ) ;
#27757=FACE_OUTER_BOUND ( 'NONE', #42169, .T. ) ;
#27758=EDGE_CURVE ( 'NONE', #2612, #33183, #3308, .T. ) ;
#27759=ORIENTED_EDGE ( 'NONE', *, *, #12475, .T. ) ;
#27760=CARTESIAN_POINT ( 'NONE',  ( -19.19517940744574602, -7.572777289964699676, 63.53065599075442549 ) ) ;
#27761=CARTESIAN_POINT ( 'NONE',  ( -14.61275832261265784, -7.909957978881497098, 60.42657991558792219 ) ) ;
#27764=DIRECTION ( 'NONE',  ( -0.9243256318339801991, 0.3816046728418207024, -8.614662759602030584E-09 ) ) ;
#27766=CARTESIAN_POINT ( 'NONE',  ( -24.25372093726098655, -13.26839283772111955, 62.90434541420221137 ) ) ;
#27767=B_SPLINE_CURVE_WITH_KNOTS ( 'NONE', 3,
 ( #30782, #4921, #38136, #31491, #46529, #41607, #15474, #34439, #45561, #37903 ),
 .UNSPECIFIED., .F., .F.,
 ( 4, 2, 2, 2, 4 ),
 ( 0.000000000000000000, 0.2500000000000000000, 0.5000000000000000000, 0.7500000000000000000, 1.000000000000000000 ),
 .UNSPECIFIED. ) ;
#27768=DIRECTION ( 'NONE',  ( -0.4501286257827957216, -0.8929637284072022840, 1.500157795982635434E-08 ) ) ;
#27769=EDGE_LOOP ( 'NONE', ( #45609, #21281 ) ) ;
#27770=CARTESIAN_POINT ( 'NONE',  ( -24.12016595861979695, -18.07666464397348349, 59.19033703419022885 ) ) ;
#27771=CARTESIAN_POINT ( 'NONE',  ( -15.11389443855535220, -21.89214149219162309, 68.73739423610683730 ) ) ;
#27772=CARTESIAN_POINT ( 'NONE',  ( -10.51631473918724780, -16.23308084970759069, 67.86278957288837432 ) ) ;
#27773=ORIENTED_EDGE ( 'NONE', *, *, #46172, .T. ) ;
#27774=CARTESIAN_POINT ( 'NONE',  ( -10.37578944195559494, -14.53307773176141815, 64.38803750143166837 ) ) ;
#27776=ORIENTED_EDGE ( 'NONE', *, *, #23391, .F. ) ;
#27777=ORIENTED_EDGE ( 'NONE', *, *, #31082, .T. ) ;
#27778=CARTESIAN_POINT ( 'NONE',  ( -23.42856991828856650, -18.40753713903406918, 72.76368185885715434 ) ) ;
#27779=CARTESIAN_POINT ( 'NONE',  ( -19.96994565995125015, -21.32983830779690848, 72.70478737306767414 ) ) ;
#27780=CARTESIAN_POINT ( 'NONE',  ( -11.29219319990544079, -18.28864530752396433, 57.82186711835544912 ) ) ;
#27782=LINE ( 'NONE', #8848, #31322 ) ;
#27783=CARTESIAN_POINT ( 'NONE',  ( -16.50258162057404832, -20.23145840177225452, 54.07175714974879099 ) ) ;
#27784=CARTESIAN_POINT ( 'NONE',  ( -24.27602536896142738, -13.14965745380569828, 62.83264206442589028 ) ) ;
#27785=B_SPLINE_CURVE_WITH_KNOTS ( 'NONE', 3,
 ( #40510, #16943, #47001, #2183, #46768, #35902, #14378, #28042, #5658, #3570 ),
 .UNSPECIFIED., .F., .F.,
 ( 4, 2, 2, 2, 4 ),
 ( 0.1272669073657635708, 0.2522669073487474045, 0.3772669073317311828, 0.5022669073147150165, 0.6272669072976988502 ),
 .UNSPECIFIED. ) ;
#27786=CARTESIAN_POINT ( 'NONE',  ( -22.87867891474110849, -19.28048576922455837, 59.29899440274890310 ) ) ;
#27787=ORIENTED_EDGE ( 'NONE', *, *, #21741, .F. ) ;
#27789=CARTESIAN_POINT ( 'NONE',  ( -11.03230825063491594, -10.98182429003440674, 60.79390496990795612 ) ) ;
#27793=CARTESIAN_POINT ( 'NONE',  ( -13.32057209662121267, -9.066726955530414855, 57.12534593251891124 ) ) ;
#27794=CARTESIAN_POINT ( 'NONE',  ( -20.96474559848019226, -20.91483931500396309, 58.80042297414523489 ) ) ;
#27796=EDGE_CURVE ( 'NONE', #23337, #10698, #20314, .T. ) ;
#27798=CARTESIAN_POINT ( 'NONE',  ( -10.33431723597471930, -12.52035407725662886, 60.98348989824278732 ) ) ;
#27799=EDGE_CURVE ( 'NONE', #10314, #31867, #21821, .T. ) ;
#27800=CARTESIAN_POINT ( 'NONE',  ( -15.55847894090159933, -21.55608122201934052, 72.06077882257353906 ) ) ;
#27801=CARTESIAN_POINT ( 'NONE',  ( -11.09194279281618556, -18.73431720802965117, 61.47699602486266457 ) ) ;
#27802=ORIENTED_EDGE ( 'NONE', *, *, #5131, .T. ) ;
#27803=CARTESIAN_POINT ( 'NONE',  ( -20.80117294895647717, -20.99790032493542213, 62.12031196887301121 ) ) ;
#27805=ORIENTED_EDGE ( 'NONE', *, *, #11132, .T. ) ;
#27807=DIRECTION ( 'NONE',  ( 8.262539640598030559E-06, -9.998826076706305650E-07, -0.9999999999653652605 ) ) ;
#27808=CARTESIAN_POINT ( 'NONE',  ( -24.23444905059911392, -16.42945129436568408, 59.40715929003106055 ) ) ;
#27811=ADVANCED_FACE ( 'NONE', ( #39862 ), #14218, .T. ) ;
#27814=CARTESIAN_POINT ( 'NONE',  ( -18.44528782684011503, -21.78515541812411982, 72.29983070759432451 ) ) ;
#27815=ORIENTED_EDGE ( 'NONE', *, *, #30594, .T. ) ;
#27816=CARTESIAN_POINT ( 'NONE',  ( -19.81074488107690001, -24.17086428735163040, 54.49999999999995026 ) ) ;
#27818=EDGE_CURVE ( 'NONE', #47353, #32996, #10557, .T. ) ;
#27824=FACE_OUTER_BOUND ( 'NONE', #13040, .T. ) ;
#27825=CARTESIAN_POINT ( 'NONE',  ( -24.08343163355289818, -12.65065354144157084, 73.52609009109720262 ) ) ;
#27826=CARTESIAN_POINT ( 'NONE',  ( -16.18802525292456096, -21.75305063948447426, 62.17057002965735535 ) ) ;
#27828=CARTESIAN_POINT ( 'NONE',  ( -23.85492384001828725, -17.57437228381108341, 62.47360986607454691 ) ) ;
#27830=CYLINDRICAL_SURFACE ( 'NONE', #40747, 0.1500000000000043243 ) ;
#27831=CARTESIAN_POINT ( 'NONE',  ( -24.61605457543312525, -12.86511826566283290, 66.41751344402152313 ) ) ;
#27832=DIRECTION ( 'NONE',  ( -0.3303050442826436228, 0.9438742382973701606, 3.829623549872328137E-09 ) ) ;
#27835=CARTESIAN_POINT ( 'NONE',  ( -11.72780659764178601, -18.87776260402302597, 68.23192005210353273 ) ) ;
#27836=CARTESIAN_POINT ( 'NONE',  ( -22.29619887594318328, -17.36118473213641167, 54.07175714974878389 ) ) ;
#27837=ORIENTED_EDGE ( 'NONE', *, *, #33689, .F. ) ;
#27839=CARTESIAN_POINT ( 'NONE',  ( -24.17899278864585355, -11.66673636667039027, 59.66731167108189737 ) ) ;
#27841=CARTESIAN_POINT ( 'NONE',  ( -13.01970113850136634, -8.800494951336613525, 64.10220657692070745 ) ) ;
#27842=CARTESIAN_POINT ( 'NONE',  ( -22.42594789675818845, -19.77792426076253918, 69.45945937764655298 ) ) ;
#27843=CARTESIAN_POINT ( 'NONE',  ( -10.74573065459234478, -12.54952415110468422, 60.81325645027152405 ) ) ;
#27845=CARTESIAN_POINT ( 'NONE',  ( -22.79734292848665334, -10.24514101169484448, 66.84182257473258915 ) ) ;
#27846=ADVANCED_FACE ( 'NONE', ( #44306 ), #47267, .T. ) ;
#27847=CARTESIAN_POINT ( 'NONE',  ( -19.31122959855452237, -8.013358182787271744, 63.84578077065769719 ) ) ;
#27849=CARTESIAN_POINT ( 'NONE',  ( -22.84886471163500588, -9.702775354051940582, 73.59665661135821324 ) ) ;
#27850=CARTESIAN_POINT ( 'NONE',  ( -21.37496138168859972, -9.030742569741930126, 70.32235629077148076 ) ) ;
#27851=( BOUNDED_CURVE ( )  B_SPLINE_CURVE ( 3, ( #1534, #20251, #42432, #46115 ),
 .UNSPECIFIED., .F., .F. ) 
 B_SPLINE_CURVE_WITH_KNOTS ( ( 4, 4 ),
 ( 0.000000000000000000, 0.4074455897393636228 ),
 .UNSPECIFIED. ) 
 CURVE ( )  GEOMETRIC_REPRESENTATION_ITEM ( )  RATIONAL_B_SPLINE_CURVE ( ( 1.000000000000000000, 0.4567392136813317460, 0.3561768502900302114, 0.6983129098260953960 ) ) 
 REPRESENTATION_ITEM ( '' )  );
#27852=ORIENTED_EDGE ( 'NONE', *, *, #23191, .T. ) ;
#27853=ORIENTED_EDGE ( 'NONE', *, *, #1831, .T. ) ;
#27855=ORIENTED_EDGE ( 'NONE', *, *, #22104, .T. ) ;
#27856=CARTESIAN_POINT ( 'NONE',  ( -10.83683315258895519, -12.44108567723101899, 57.32857332099802505 ) ) ;
#27858=EDGE_CURVE ( 'NONE', #44291, #20782, #46409, .T. ) ;
#27860=ORIENTED_EDGE ( 'NONE', *, *, #47650, .F. ) ;
#27861=( BOUNDED_CURVE ( )  B_SPLINE_CURVE ( 3, ( #27557, #4414, #46275, #1200 ),
 .UNSPECIFIED., .F., .F. ) 
 B_SPLINE_CURVE_WITH_KNOTS ( ( 4, 4 ),
 ( 0.9074455897393690629, 1.000000000000000000 ),
 .UNSPECIFIED. ) 
 CURVE ( )  GEOMETRIC_REPRESENTATION_ITEM ( )  RATIONAL_B_SPLINE_CURVE ( ( 0.6983129098261063872, 0.7760317562607097486, 0.8765941196520076195, 1.000000000000000000 ) ) 
 REPRESENTATION_ITEM ( '' )  );
#27862=CARTESIAN_POINT ( 'NONE',  ( -10.83518795442179972, -11.33195075051574108, 67.78011127842214023 ) ) ;
#27863=CARTESIAN_POINT ( 'NONE',  ( -10.00761937521931522, -15.51608998476985946, 57.75288115419267854 ) ) ;
#27865=CARTESIAN_POINT ( 'NONE',  ( -10.60570718526854961, -17.81143598018131158, 71.68222757358374508 ) ) ;
#27866=CARTESIAN_POINT ( 'NONE',  ( -23.80698208075059341, -17.68407496960266201, 62.48977578363538044 ) ) ;
#27868=CARTESIAN_POINT ( 'NONE',  ( -19.97013658168673800, -21.81073013994861398, 68.97836559665680056 ) ) ;
#27869=VERTEX_POINT ( 'NONE', #18169 ) ;
#27871=ORIENTED_EDGE ( 'NONE', *, *, #42837, .T. ) ;
#27873=CARTESIAN_POINT ( 'NONE',  ( -16.78341102624552050, -22.23169286577646986, 68.88055947109249644 ) ) ;
#27874=CARTESIAN_POINT ( 'NONE',  ( -19.30861700655685098, -22.01699669475148724, 58.78153328179137560 ) ) ;
#27875=ORIENTED_EDGE ( 'NONE', *, *, #1093, .T. ) ;
#27877=ADVANCED_FACE ( 'NONE', ( #40117 ), #21639, .T. ) ;
#27878=EDGE_CURVE ( 'NONE', #22320, #34081, #20925, .T. ) ;
#27879=CARTESIAN_POINT ( 'NONE',  ( -21.34581862946232889, -20.66775363590295100, 72.52446429492309221 ) ) ;
#27880=CARTESIAN_POINT ( 'NONE',  ( -17.85903083518457635, -21.79574121735856451, 58.47841500721298047 ) ) ;
#27881=CARTESIAN_POINT ( 'NONE',  ( -24.45422819554991278, -14.24171526414585287, 66.06804100909725719 ) ) ;
#27882=CARTESIAN_POINT ( 'NONE',  ( -10.47299139157196990, -15.63514485490427575, 61.03789045487297926 ) ) ;
#27883=CARTESIAN_POINT ( 'NONE',  ( -20.57444551192666538, -21.06071957749239232, 58.66091790465502953 ) ) ;
#27884=ORIENTED_EDGE ( 'NONE', *, *, #11323, .F. ) ;
#27886=FACE_OUTER_BOUND ( 'NONE', #22511, .T. ) ;
#27887=CARTESIAN_POINT ( 'NONE',  ( -16.18369095565973836, -7.463183609464278057, 60.30004841332083743 ) ) ;
#27889=ADVANCED_FACE ( 'NONE', ( #11780 ), #3648, .T. ) ;
#27890=EDGE_CURVE ( 'NONE', #16629, #37435, #38101, .T. ) ;
#27891=CARTESIAN_POINT ( 'NONE',  ( -24.87384330133638599, -14.87999890626018384, 59.35804801245023299 ) ) ;
#27895=EDGE_CURVE ( 'NONE', #18577, #9916, #9158, .T. ) ;
#27897=CARTESIAN_POINT ( 'NONE',  ( -18.72681101482838173, -7.880611649715417499, 70.37068030201731972 ) ) ;
#27898=VERTEX_POINT ( 'NONE', #22133 ) ;
#27900=CARTESIAN_POINT ( 'NONE',  ( -10.53028993777715883, -16.28642212234895226, 71.73278239416407587 ) ) ;
#27901=CARTESIAN_POINT ( 'NONE',  ( -23.08009853854674986, -9.960157477770804846, 66.58536326842445874 ) ) ;
#27902=CARTESIAN_POINT ( 'NONE',  ( -22.88264614489240856, -10.34704276773305764, 63.35713876973677827 ) ) ;
#27903=B_SPLINE_CURVE_WITH_KNOTS ( 'NONE', 3,
 ( #16487, #1227, #46057, #16232, #13265, #12317, #28322, #20923, #28061, #39143 ),
 .UNSPECIFIED., .F., .F.,
 ( 4, 2, 2, 2, 4 ),
 ( 0.000000000000000000, 0.2500000000000000000, 0.5000000000000000000, 0.7500000000000000000, 1.000000000000000000 ),
 .UNSPECIFIED. ) ;
#27904=VERTEX_POINT ( 'NONE', #15437 ) ;
#27905=CARTESIAN_POINT ( 'NONE',  ( -24.80084942886774257, -15.85139998926299398, 69.63333248085599791 ) ) ;
#27907=CARTESIAN_POINT ( 'NONE',  ( -11.96084906401204506, -9.743958800322932490, 60.74413413563605957 ) ) ;
#27909=ORIENTED_EDGE ( 'NONE', *, *, #43522, .T. ) ;
#27910=CARTESIAN_POINT ( 'NONE',  ( -17.08147026401541524, -7.366339275741904835, 70.60380589010705421 ) ) ;
#27911=CARTESIAN_POINT ( 'NONE',  ( -10.43031943402893269, -12.24169207515381785, 57.46823944168010456 ) ) ;
#27912=B_SPLINE_CURVE_WITH_KNOTS ( 'NONE', 1,
 ( #34734, #34967 ),
 .UNSPECIFIED., .F., .F.,
 ( 2, 2 ),
 ( 0.000000000000000000, 1.000000000000000000 ),
 .UNSPECIFIED. ) ;
#27918=B_SPLINE_CURVE_WITH_KNOTS ( 'NONE', 1,
 ( #37957, #17237 ),
 .UNSPECIFIED., .F., .F.,
 ( 2, 2 ),
 ( 0.000000000000000000, 1.000000000000000000 ),
 .UNSPECIFIED. ) ;
#27919=CARTESIAN_POINT ( 'NONE',  ( -15.55648817577099585, -8.010769314271311003, 74.09457776258329886 ) ) ;
#27920=CARTESIAN_POINT ( 'NONE',  ( -24.87401146225354864, -14.84424530793535624, 59.39300237368605906 ) ) ;
#27923=CARTESIAN_POINT ( 'NONE',  ( -12.27729925481933471, -9.991218852276041673, 60.55918086709623083 ) ) ;
#27924=VECTOR ( 'NONE', #18425, 1000.000000000000114 ) ;
#27930=ORIENTED_EDGE ( 'NONE', *, *, #43510, .F. ) ;
#27931=CARTESIAN_POINT ( 'NONE',  ( -10.29245896349820200, -16.96639176515380854, 57.87415878384224044 ) ) ;
#27932=CARTESIAN_POINT ( 'NONE',  ( -18.52415950777489684, -7.896185818571675341, 74.14064402152244782 ) ) ;
#27933=ORIENTED_EDGE ( 'NONE', *, *, #43497, .T. ) ;
#27936=CARTESIAN_POINT ( 'NONE',  ( -10.00551284293887910, -15.49280627557078382, 57.66769182383846726 ) ) ;
#27937=FACE_OUTER_BOUND ( 'NONE', #35552, .T. ) ;
#27939=ORIENTED_EDGE ( 'NONE', *, *, #6730, .T. ) ;
#27940=CARTESIAN_POINT ( 'NONE',  ( -18.57335281209669375, -21.76520412651811043, 72.57038810541313012 ) ) ;
#27943=CARTESIAN_POINT ( 'NONE',  ( -21.14127837747716043, -20.79979359094293656, 69.06010003804692587 ) ) ;
#27944=EDGE_CURVE ( 'NONE', #45965, #24590, #33666, .T. ) ;
#27945=CARTESIAN_POINT ( 'NONE',  ( -24.87417962317557496, -14.80849170857717567, 59.42795673386487465 ) ) ;
#27946=CARTESIAN_POINT ( 'NONE',  ( -23.34452670104532146, -10.97471634670236718, 73.36193064516098161 ) ) ;
#27947=EDGE_CURVE ( 'NONE', #36933, #25852, #46749, .T. ) ;
#27948=CARTESIAN_POINT ( 'NONE',  ( -14.72778340125292829, -21.32322296975913645, 58.46617885012764049 ) ) ;
#27949=ORIENTED_EDGE ( 'NONE', *, *, #47664, .T. ) ;
#27950=CARTESIAN_POINT ( 'NONE',  ( -12.15107414628315574, -10.20293217168262245, 67.68823922474383892 ) ) ;
#27951=ADVANCED_FACE ( 'NONE', ( #458 ), #7365, .T. ) ;
#27952=CARTESIAN_POINT ( 'NONE',  ( -12.23358631666068241, -10.11189219506639247, 64.31297738809925590 ) ) ;
#27954=ORIENTED_EDGE ( 'NONE', *, *, #8083, .T. ) ;
#27955=DIRECTION ( 'NONE',  ( -0.4439273849576907960, -0.8960627639203775363, -1.004702157338010031E-17 ) ) ;
#27957=CARTESIAN_POINT ( 'NONE',  ( -20.31413516131974717, -8.378470924821744603, 67.06632013881642251 ) ) ;
#27958=ORIENTED_EDGE ( 'NONE', *, *, #17755, .T. ) ;
#27959=ORIENTED_EDGE ( 'NONE', *, *, #22499, .T. ) ;
#27960=EDGE_LOOP ( 'NONE', ( #24193, #1163 ) ) ;
#27962=CARTESIAN_POINT ( 'NONE',  ( -12.86614516408948283, -8.916182316271401120, 67.57931555780623967 ) ) ;
#27966=CARTESIAN_POINT ( 'NONE',  ( -10.71275572639902940, -16.80316056253202817, 57.91590435120537705 ) ) ;
#27967=ORIENTED_EDGE ( 'NONE', *, *, #4935, .T. ) ;
#27968=EDGE_LOOP ( 'NONE', ( #47641, #34614, #45771, #46921, #9979 ) ) ;
#27971=CARTESIAN_POINT ( 'NONE',  ( -22.09234551867295693, -20.09219114410425178, 62.53439162497838311 ) ) ;
#27973=DIRECTION ( 'NONE',  ( -0.1186632576870824130, 0.9929345553837299887, 6.051931679537041823E-08 ) ) ;
#27976=DIRECTION ( 'NONE',  ( 1.205044182495138397E-05, 2.694341358818416019E-06, 0.9999999999237635384 ) ) ;
#27978=CYLINDRICAL_SURFACE ( 'NONE', #40952, 0.4000000000000006883 ) ;
#27979=( BOUNDED_SURFACE ( )  B_SPLINE_SURFACE ( 3, 1, ( 
 ( #1632, #24299 ),
 ( #1379, #39303 ),
 ( #32163, #31916 ),
 ( #39781, #35832 ),
 ( #13425, #46932 ),
 ( #6047, #17113 ),
 ( #28475, #43498 ) ),
 .UNSPECIFIED., .T., .F., .F. ) 
 B_SPLINE_SURFACE_WITH_KNOTS ( ( 4, 3, 4 ),
 ( 2, 2 ),
 ( 0.000000000000000000, 0.5000000000000000000, 1.000000000000000000 ),
 ( 0.000000000000000000, 1.000000000000000000 ),
 .UNSPECIFIED. ) 
 GEOMETRIC_REPRESENTATION_ITEM ( )  RATIONAL_B_SPLINE_SURFACE ( (
 ( 1.000000000000000000, 1.000000000000000000),
 ( 0.3333333333333335369, 0.3333333333333330373),
 ( 0.3333333333333335369, 0.3333333333333330373),
 ( 1.000000000000000000, 1.000000000000000000),
 ( 0.3333333333333333703, 0.3333333333333333703),
 ( 0.3333333333333333703, 0.3333333333333333703),
 ( 1.000000000000000000, 1.000000000000000000) ) ) 
 REPRESENTATION_ITEM ( '' )  SURFACE ( )  );
#27980=EDGE_CURVE ( 'NONE', #20878, #1905, #26783, .T. ) ;
#27981=ORIENTED_EDGE ( 'NONE', *, *, #23191, .F. ) ;
#27983=VECTOR ( 'NONE', #13607, 1000.000000000000227 ) ;
#27984=CARTESIAN_POINT ( 'NONE',  ( -10.37599212182869124, -14.63324797960940771, 71.34254748307667171 ) ) ;
#27986=CARTESIAN_POINT ( 'NONE',  ( -22.53655392111809164, -20.22829597721307948, 65.88917050827579658 ) ) ;
#27987=ORIENTED_EDGE ( 'NONE', *, *, #20947, .F. ) ;
#27989=CARTESIAN_POINT ( 'NONE',  ( -24.45577199812615632, -12.20047074031916168, 53.49999999999994316 ) ) ;
#27990=CARTESIAN_POINT ( 'NONE',  ( -20.11579277122780596, -7.862326722158320180, 73.89813526064125426 ) ) ;
#27991=ORIENTED_EDGE ( 'NONE', *, *, #35831, .T. ) ;
#27992=CARTESIAN_POINT ( 'NONE',  ( -17.13503149044196761, -7.764836982087094164, 70.77563787455143540 ) ) ;
#27993=( BOUNDED_CURVE ( )  B_SPLINE_CURVE ( 3, ( #29096, #44153, #10401, #6695 ),
 .UNSPECIFIED., .F., .F. ) 
 B_SPLINE_CURVE_WITH_KNOTS ( ( 4, 4 ),
 ( 0.9074455897393649551, 1.000000000000000000 ),
 .UNSPECIFIED. ) 
 CURVE ( )  GEOMETRIC_REPRESENTATION_ITEM ( )  RATIONAL_B_SPLINE_CURVE ( ( 0.6983129098261113832, 0.7760317562607140784, 0.8765941196520102840, 1.000000000000000000 ) ) 
 REPRESENTATION_ITEM ( '' )  );
#27995=CARTESIAN_POINT ( 'NONE',  ( -23.42915847708036736, -11.11517115755410146, 73.64721174900437006 ) ) ;
#27996=CYLINDRICAL_SURFACE ( 'NONE', #24101, 0.1500000000000061007 ) ;
#27997=ORIENTED_EDGE ( 'NONE', *, *, #39444, .F. ) ;
#27999=CARTESIAN_POINT ( 'NONE',  ( -19.98813040044048606, -21.37641421727040125, 72.40478737316021807 ) ) ;
#28001=B_SPLINE_CURVE_WITH_KNOTS ( 'NONE', 3,
 ( #35680, #28561, #43590, #42854, #1475, #1733, #16490, #27825, #42624, #43347 ),
 .UNSPECIFIED., .F., .F.,
 ( 4, 2, 2, 2, 4 ),
 ( 0.000000000000000000, 0.2500000000000000000, 0.5000000000000000000, 0.7500000000000000000, 1.000000000000000000 ),
 .UNSPECIFIED. ) ;
#28002=ADVANCED_FACE ( 'NONE', ( #30979 ), #35380, .T. ) ;
#28005=CARTESIAN_POINT ( 'NONE',  ( -9.993919958658839420, -14.26595478062693800, 64.58815064441371590 ) ) ;
#28006=ADVANCED_FACE ( 'NONE', ( #31698 ), #46723, .T. ) ;
#28007=CARTESIAN_POINT ( 'NONE',  ( -23.99022880263543200, -10.64948376341961378, 54.30803469517864102 ) ) ;
#28008=CARTESIAN_POINT ( 'NONE',  ( -22.25881579015244682, -9.141043659704909174, 59.92182412794203117 ) ) ;
#28009=ORIENTED_EDGE ( 'NONE', *, *, #22650, .T. ) ;
#28010=CARTESIAN_POINT ( 'NONE',  ( -15.54840433177174397, -8.005034934413657766, 67.29574103338339341 ) ) ;
#28011=( BOUNDED_CURVE ( )  B_SPLINE_CURVE ( 3, ( #46158, #19825, #23519, #12899 ),
 .UNSPECIFIED., .F., .F. ) 
 B_SPLINE_CURVE_WITH_KNOTS ( ( 4, 4 ),
 ( 0.5000000000000000000, 0.9074455897393680637 ),
 .UNSPECIFIED. ) 
 CURVE ( )  GEOMETRIC_REPRESENTATION_ITEM ( )  RATIONAL_B_SPLINE_CURVE ( ( 0.9999999999999972244, 0.4567392136813289705, 0.3561768502900310440, 0.6983129098261003920 ) ) 
 REPRESENTATION_ITEM ( '' )  );
#28013=CARTESIAN_POINT ( 'NONE',  ( -24.73928442521073023, -16.22033272921623848, 62.78602803661277676 ) ) ;
#28014=VERTEX_POINT ( 'NONE', #35136 ) ;
#28015=VERTEX_POINT ( 'NONE', #937 ) ;
#28016=CARTESIAN_POINT ( 'NONE',  ( -14.87212829970780703, -21.32751220717084806, 58.23906021010879641 ) ) ;
#28017=CARTESIAN_POINT ( 'NONE',  ( -10.92563986671175691, -18.45389586190763964, 57.99369949602996854 ) ) ;
#28021=CARTESIAN_POINT ( 'NONE',  ( -12.37144311045842038, -19.65386551827485917, 58.03568442835949526 ) ) ;
#28022=B_SPLINE_CURVE_WITH_KNOTS ( 'NONE', 1,
 ( #12708, #41789 ),
 .UNSPECIFIED., .F., .F.,
 ( 2, 2 ),
 ( 0.000000000000000000, 1.000000000000000000 ),
 .UNSPECIFIED. ) ;
#28023=CARTESIAN_POINT ( 'NONE',  ( -13.88293259567353566, -20.90532631576516209, 68.45625136994867432 ) ) ;
#28025=CARTESIAN_POINT ( 'NONE',  ( -23.29918407416772297, -19.39037376486758646, 58.99915347576865088 ) ) ;
#28027=ORIENTED_EDGE ( 'NONE', *, *, #26815, .F. ) ;
#28029=CARTESIAN_POINT ( 'NONE',  ( -11.13352401182878459, -11.60862911821036292, 74.70272630447266238 ) ) ;
#28030=B_SPLINE_CURVE_WITH_KNOTS ( 'NONE', 3,
 ( #20010, #16289, #5001, #34783, #46359, #8934, #45879, #26920, #15561, #1279 ),
 .UNSPECIFIED., .F., .F.,
 ( 4, 2, 2, 2, 4 ),
 ( 0.6272669072782502964, 0.7522669073001506668, 0.8772669073220509262, 1.002266907343951186, 1.127266907365851667 ),
 .UNSPECIFIED. ) ;
#28032=CARTESIAN_POINT ( 'NONE',  ( -19.63995608841934626, -21.92282860479379991, 65.65141533869274326 ) ) ;
#28033=CARTESIAN_POINT ( 'NONE',  ( -22.37742504188432235, -19.75764164967408831, 72.83327514797355207 ) ) ;
#28037=CARTESIAN_POINT ( 'NONE',  ( -24.01628879148212548, -11.33852128837717999, 66.52240266552541925 ) ) ;
#28038=CYLINDRICAL_SURFACE ( 'NONE', #13459, 0.1500000000000008549 ) ;
#28040=ADVANCED_FACE ( 'NONE', ( #12021 ), #3276, .T. ) ;
#28042=CARTESIAN_POINT ( 'NONE',  ( -10.12821362422299210, -13.30163807797161546, 74.87806422314912425 ) ) ;
#28044=CARTESIAN_POINT ( 'NONE',  ( -17.77594409791816688, -7.367433943401969998, 60.26556080592736464 ) ) ;
#28045=CARTESIAN_POINT ( 'NONE',  ( -18.60148803548772278, -7.908491065787107033, 73.85681094374102429 ) ) ;
#28046=CARTESIAN_POINT ( 'NONE',  ( -11.57017261513264117, -10.87519553945718620, 57.62392099249677102 ) ) ;
#28047=CARTESIAN_POINT ( 'NONE',  ( -11.10300703817161327, -10.86615712478015539, 57.39398594787093089 ) ) ;
#28049=EDGE_CURVE ( 'NONE', #35496, #2258, #15586, .T. ) ;
#28050=CARTESIAN_POINT ( 'NONE',  ( -19.04853579327176760, -7.948602568230340282, 63.71617106789811658 ) ) ;
#28054=CARTESIAN_POINT ( 'NONE',  ( -10.01188548097954012, -14.05969102102910284, 61.11832497397694652 ) ) ;
#28056=VERTEX_POINT ( 'NONE', #39324 ) ;
#28057=CARTESIAN_POINT ( 'NONE',  ( -18.37786432726835883, -21.79469297182707521, 69.10042588711679912 ) ) ;
#28058=CARTESIAN_POINT ( 'NONE',  ( -13.05029276218966672, -20.34859559109395377, 71.96220867596423432 ) ) ;
#28059=B_SPLINE_CURVE_WITH_KNOTS ( 'NONE', 3,
 ( #7479, #3511, #25679, #33051, #18525, #11394, #48325, #48094, #14560, #29876 ),
 .UNSPECIFIED., .F., .F.,
 ( 4, 2, 2, 2, 4 ),
 ( 0.1272669073658321826, 0.2522669073463198464, 0.3772669073268074547, 0.5022669073072951740, 0.6272669072877827823 ),
 .UNSPECIFIED. ) ;
#28060=EDGE_LOOP ( 'NONE', ( #17200, #34119, #9075, #11988, #18879 ) ) ;
#28061=CARTESIAN_POINT ( 'NONE',  ( -11.95536650667902911, -10.43947391085179710, 71.26893134408621222 ) ) ;
#28062=VECTOR ( 'NONE', #6554, 1000.000000000000227 ) ;
#28064=ORIENTED_EDGE ( 'NONE', *, *, #17372, .T. ) ;
#28066=CARTESIAN_POINT ( 'NONE',  ( -10.47425521701617157, -17.49314416303823450, 64.81234701634230078 ) ) ;
#28069=CARTESIAN_POINT ( 'NONE',  ( -24.76682342852691221, -16.06919080767510621, 66.25663251748672167 ) ) ;
#28071=ORIENTED_EDGE ( 'NONE', *, *, #5468, .F. ) ;
#28072=ADVANCED_FACE ( 'NONE', ( #27757 ), #23838, .T. ) ;
#28073=CARTESIAN_POINT ( 'NONE',  ( -23.77708670646326539, -18.70057811943135206, 72.87094101505380195 ) ) ;
#28074=DIRECTION ( 'NONE',  ( 4.436160459547892897E-06, 7.761523768847967188E-06, -0.9999999999600396317 ) ) ;
#28080=CARTESIAN_POINT ( 'NONE',  ( -10.42752915138136238, -15.03043058157462042, 75.02452189207510003 ) ) ;
#28081=CARTESIAN_POINT ( 'NONE',  ( -19.78614017500849087, -21.39864787494504839, 68.93482476778672208 ) ) ;
#28082=CARTESIAN_POINT ( 'NONE',  ( -15.84272952059200712, -7.988518299429712144, 70.79917007911708993 ) ) ;
#28083=ORIENTED_EDGE ( 'NONE', *, *, #44027, .F. ) ;
#28085=CARTESIAN_POINT ( 'NONE',  ( -19.04853579327176760, -7.948602568230340282, 63.71617106789811658 ) ) ;
#28086=CARTESIAN_POINT ( 'NONE',  ( -12.29360062986345525, -9.973804982380832129, 60.55918084114097866 ) ) ;
#28087=CARTESIAN_POINT ( 'NONE',  ( -13.06825169942196752, -9.255684228991221119, 74.46356075877366720 ) ) ;
#28088=CARTESIAN_POINT ( 'NONE',  ( -13.46392603942681276, -20.58285214721693634, 61.74476297758946686 ) ) ;
#28089=EDGE_CURVE ( 'NONE', #2205, #19987, #8319, .T. ) ;
#28091=ORIENTED_EDGE ( 'NONE', *, *, #27622, .F. ) ;
#28093=EDGE_LOOP ( 'NONE', ( #39561, #17908, #32768, #12794, #42581 ) ) ;
#28094=VECTOR ( 'NONE', #39620, 1000.000000000000227 ) ;
#28095=B_SPLINE_CURVE_WITH_KNOTS ( 'NONE', 3,
 ( #2881, #44043, #3375, #37334, #37095, #14661, #28757, #14188, #3622, #40800 ),
 .UNSPECIFIED., .F., .F.,
 ( 4, 2, 2, 2, 4 ),
 ( 0.6272669072782597333, 0.7522669073001514439, 0.8772669073220431546, 1.002266907343934754, 1.127266907365826576 ),
 .UNSPECIFIED. ) ;
#28096=ORIENTED_EDGE ( 'NONE', *, *, #34150, .F. ) ;
#28098=EDGE_CURVE ( 'NONE', #11365, #7957, #10895, .T. ) ;
#28099=CARTESIAN_POINT ( 'NONE',  ( -24.87286266620955288, -14.66952948351439190, 62.96942391020206742 ) ) ;
#28100=CARTESIAN_POINT ( 'NONE',  ( -18.94388778215946445, -7.924927710426770133, 66.90071813243744714 ) ) ;
#28101=CARTESIAN_POINT ( 'NONE',  ( -21.80947544975385810, -9.353161466788067813, 63.19153755920122251 ) ) ;
#28102=VECTOR ( 'NONE', #22, 999.9999999999998863 ) ;
#28103=ORIENTED_EDGE ( 'NONE', *, *, #48459, .T. ) ;
#28104=CARTESIAN_POINT ( 'NONE',  ( -21.95217610637629946, -9.395202297576263462, 66.80583047767832738 ) ) ;
#28105=CARTESIAN_POINT ( 'NONE',  ( -12.54253407177667512, -19.82621502378690082, 65.16674886820000268 ) ) ;
#28106=ORIENTED_EDGE ( 'NONE', *, *, #9613, .T. ) ;
#28107=CARTESIAN_POINT ( 'NONE',  ( -19.30128557755455176, -21.60500301973953086, 58.81035253397666196 ) ) ;
#28108=VERTEX_POINT ( 'NONE', #39566 ) ;
#28109=CARTESIAN_POINT ( 'NONE',  ( -23.35504391816078495, -10.30071636613414832, 59.70179792000674723 ) ) ;
#28110=B_SPLINE_CURVE_WITH_KNOTS ( 'NONE', 3,
 ( #41127, #45085, #11335, #268, #4199, #40877, #22921, #48501, #18457, #7162 ),
 .UNSPECIFIED., .F., .F.,
 ( 4, 2, 2, 2, 4 ),
 ( 0.000000000000000000, 0.2500000000000000000, 0.5000000000000000000, 0.7500000000000000000, 1.000000000000000000 ),
 .UNSPECIFIED. ) ;
#28112=CARTESIAN_POINT ( 'NONE',  ( -10.61357223164714902, -13.19155561173493219, 71.20828586568362084 ) ) ;
#28113=ORIENTED_EDGE ( 'NONE', *, *, #37976, .T. ) ;
#28114=DIRECTION ( 'NONE',  ( -1.066846703571655765E-06, 9.113387012630844478E-06, 0.9999999999579040066 ) ) ;
#28115=CARTESIAN_POINT ( 'NONE',  ( -14.78754745127378634, -8.270772244812135909, 60.61996282000563241 ) ) ;
#28116=DIRECTION ( 'NONE',  ( 1.078386539787844256E-05, -7.293043934967424929E-06, 0.9999999999152597852 ) ) ;
#28120=CARTESIAN_POINT ( 'NONE',  ( -24.42310453963427008, -14.68514377117137570, 63.01296481370926017 ) ) ;
#28122=CARTESIAN_POINT ( 'NONE',  ( -17.72419722990865054, -21.80277058550420577, 58.40553378253839156 ) ) ;
#28123=AXIS2_PLACEMENT_3D ( 'NONE', #41251, #44473, #14149 ) ;
#28124=( BOUNDED_SURFACE ( )  B_SPLINE_SURFACE ( 3, 1, ( 
 ( #28275, #2162 ),
 ( #43303, #5145 ),
 ( #1434, #16447 ),
 ( #31482, #24597 ),
 ( #17163, #3372 ),
 ( #47953, #48188 ),
 ( #32909, #10292 ) ),
 .UNSPECIFIED., .T., .F., .F. ) 
 B_SPLINE_SURFACE_WITH_KNOTS ( ( 4, 3, 4 ),
 ( 2, 2 ),
 ( 0.000000000000000000, 0.5000000000000000000, 1.000000000000000000 ),
 ( 0.000000000000000000, 1.000000000000000000 ),
 .UNSPECIFIED. ) 
 GEOMETRIC_REPRESENTATION_ITEM ( )  RATIONAL_B_SPLINE_SURFACE ( (
 ( 1.000000000000000000, 1.000000000000000000),
 ( 0.3333333333333335369, 0.3333333333333330373),
 ( 0.3333333333333335369, 0.3333333333333330373),
 ( 1.000000000000000000, 1.000000000000000000),
 ( 0.3333333333333333703, 0.3333333333333333703),
 ( 0.3333333333333333703, 0.3333333333333333703),
 ( 1.000000000000000000, 1.000000000000000000) ) ) 
 REPRESENTATION_ITEM ( '' )  SURFACE ( )  );
#28125=CARTESIAN_POINT ( 'NONE',  ( -13.74195172841370649, -8.854398236607520900, 57.19797722959653896 ) ) ;
#28127=CARTESIAN_POINT ( 'NONE',  ( -10.37818533259200748, -17.22973363664382873, 61.27247698181179913 ) ) ;
#28129=CARTESIAN_POINT ( 'NONE',  ( -21.95523322170430092, -8.895446802377390938, 66.77654591769551473 ) ) ;
#28132=CYLINDRICAL_SURFACE ( 'NONE', #10864, 0.1499999999999994671 ) ;
#28133=DIRECTION ( 'NONE',  ( -5.731567514496413899E-31, -1.020425574103664789E-16, -1.000000000000000000 ) ) ;
#28134=CARTESIAN_POINT ( 'NONE',  ( -23.27284462870851911, -18.74605969774991010, 66.10917289053097079 ) ) ;
#28135=CARTESIAN_POINT ( 'NONE',  ( -19.23866564181064831, -21.62168251543364050, 58.82507384655652771 ) ) ;
#28137=ORIENTED_EDGE ( 'NONE', *, *, #23854, .T. ) ;
#28139=CARTESIAN_POINT ( 'NONE',  ( -20.83411228044830210, -20.98307166581800587, 65.99942768993690834 ) ) ;
#28140=LINE ( 'NONE', #5971, #7708 ) ;
#28142=B_SPLINE_CURVE_WITH_KNOTS ( 'NONE', 3,
 ( #19005, #535, #19481, #45615, #3487, #3740, #18500, #33504, #48545, #29851 ),
 .UNSPECIFIED., .F., .F.,
 ( 4, 2, 2, 2, 4 ),
 ( 0.1272669073658269645, 0.2522669073463317813, 0.3772669073268366535, 0.5022669073073414703, 0.6272669072878462870 ),
 .UNSPECIFIED. ) ;
#28143=DIRECTION ( 'NONE',  ( 0.6478992145799701285, -0.7617260713318518839, 1.927832152310587152E-08 ) ) ;
#28144=FACE_OUTER_BOUND ( 'NONE', #9608, .T. ) ;
#28145=CARTESIAN_POINT ( 'NONE',  ( -23.12431869989520550, -10.01221758024046338, 66.79828185159925624 ) ) ;
#28146=AXIS2_PLACEMENT_3D ( 'NONE', #2507, #43888, #32312 ) ;
#28147=CARTESIAN_POINT ( 'NONE',  ( -22.94085508618206859, -9.802298960702817254, 70.19673832247809742 ) ) ;
#28148=( BOUNDED_CURVE ( )  B_SPLINE_CURVE ( 3, ( #40425, #47816, #48536, #3732 ),
 .UNSPECIFIED., .F., .F. ) 
 B_SPLINE_CURVE_WITH_KNOTS ( ( 4, 4 ),
 ( 0.5000000000000000000, 0.9074455897393666204 ),
 .UNSPECIFIED. ) 
 CURVE ( )  GEOMETRIC_REPRESENTATION_ITEM ( )  RATIONAL_B_SPLINE_CURVE ( ( 1.000000000000014655, 0.4567392136813281378, 0.3561768502900183875, 0.6983129098261015022 ) ) 
 REPRESENTATION_ITEM ( '' )  );
#28149=EDGE_LOOP ( 'NONE', ( #11818, #46815, #37800, #38854, #21153 ) ) ;
#28150=AXIS2_PLACEMENT_3D ( 'NONE', #21895, #3425, #36899 ) ;
#28151=DIRECTION ( 'NONE',  ( 1.371992797150048625E-08, -1.272593384837864910E-06, 0.9999999999991900923 ) ) ;
#28153=CARTESIAN_POINT ( 'NONE',  ( -14.87952233054990714, -7.807053693480528800, 57.01146488488941344 ) ) ;
#28154=ORIENTED_EDGE ( 'NONE', *, *, #31379, .T. ) ;
#28155=CARTESIAN_POINT ( 'NONE',  ( -11.31433821118811522, -10.42787716839952239, 53.76227901944321275 ) ) ;
#28156=CARTESIAN_POINT ( 'NONE',  ( -24.41631212572655585, -17.38062150060373767, 69.60613961827247920 ) ) ;
#28158=CARTESIAN_POINT ( 'NONE',  ( -24.10584592916820057, -12.56049825913868645, 73.24225570139947195 ) ) ;
#28159=CARTESIAN_POINT ( 'NONE',  ( -10.71495554099518088, -12.81234323494808436, 64.56836111193433680 ) ) ;
#28160=( BOUNDED_CURVE ( )  B_SPLINE_CURVE ( 3, ( #10319, #43330, #6615, #39618 ),
 .UNSPECIFIED., .F., .F. ) 
 B_SPLINE_CURVE_WITH_KNOTS ( ( 4, 4 ),
 ( 0.000000000000000000, 0.4074455897393627346 ),
 .UNSPECIFIED. ) 
 CURVE ( )  GEOMETRIC_REPRESENTATION_ITEM ( )  RATIONAL_B_SPLINE_CURVE ( ( 1.000000000000000000, 0.4567392136813397396, 0.3561768502900331534, 0.6983129098260801859 ) ) 
 REPRESENTATION_ITEM ( '' )  );
#28162=VERTEX_POINT ( 'NONE', #40298 ) ;
#28167=VECTOR ( 'NONE', #47794, 1000.000000000000114 ) ;
#28168=CYLINDRICAL_SURFACE ( 'NONE', #42605, 0.1500000000000050460 ) ;
#28170=AXIS2_PLACEMENT_3D ( 'NONE', #46182, #15886, #636 ) ;
#28171=AXIS2_PLACEMENT_3D ( 'NONE', #36160, #28319, #25576 ) ;
#28172=ADVANCED_FACE ( 'NONE', ( #29214 ), #10013, .T. ) ;
#28173=ADVANCED_FACE ( 'NONE', ( #6072 ), #36098, .T. ) ;
#28174=CARTESIAN_POINT ( 'NONE',  ( -24.44689184067228638, -14.18710713894228270, 69.93803194250308763 ) ) ;
#28175=DIRECTION ( 'NONE',  ( -0.9950649908465211135, -0.09922531930717196080, 4.894557008102618136E-08 ) ) ;
#28176=ORIENTED_EDGE ( 'NONE', *, *, #12366, .F. ) ;
#28177=DIRECTION ( 'NONE',  ( -0.9974380310868018462, -0.07153582418399356824, 3.008056591778322057E-08 ) ) ;
#28179=CARTESIAN_POINT ( 'NONE',  ( -24.23980054858686728, -17.81742536025289070, 62.66699277536263679 ) ) ;
#28180=VERTEX_POINT ( 'NONE', #2853 ) ;
#28181=CARTESIAN_POINT ( 'NONE',  ( -22.45050777529662511, -19.68108125846770307, 69.36521271289056756 ) ) ;
#28182=CARTESIAN_POINT ( 'NONE',  ( -16.39156059917436181, -21.78318494029796781, 62.05568132351888266 ) ) ;
#28183=ORIENTED_EDGE ( 'NONE', *, *, #34707, .F. ) ;
#28185=CARTESIAN_POINT ( 'NONE',  ( -11.42622260759249286, -18.51434353338492400, 61.57710833179551457 ) ) ;
#28186=ORIENTED_EDGE ( 'NONE', *, *, #42578, .T. ) ;
#28187=CARTESIAN_POINT ( 'NONE',  ( -17.70776945889202736, -22.25388964270624825, 58.52058054029878065 ) ) ;
#28188=EDGE_CURVE ( 'NONE', #9986, #26867, #43171, .T. ) ;
#28190=CARTESIAN_POINT ( 'NONE',  ( -24.40658499505739698, -15.78250870199476630, 69.83307488408829045 ) ) ;
#28193=CARTESIAN_POINT ( 'NONE',  ( -22.00117057250496444, -9.443090202341716477, 63.60642510345682155 ) ) ;
#28194=CARTESIAN_POINT ( 'NONE',  ( -22.14090652532222236, -20.04928072148792495, 62.51967078134249078 ) ) ;
#28195=DIRECTION ( 'NONE',  ( 0.5589780652556124441, -0.8291824422665291516, 7.938832475108296738E-08 ) ) ;
#28196=CARTESIAN_POINT ( 'NONE',  ( -12.45907596150898300, -19.82553632194446180, 58.08249573729000304 ) ) ;
#28197=CARTESIAN_POINT ( 'NONE',  ( -20.18941521006531303, -7.891347330600439136, 73.83601268700121523 ) ) ;
#28198=CARTESIAN_POINT ( 'NONE',  ( -14.36817892824948473, -8.455618309860652104, 67.54503025475186462 ) ) ;
#28199=B_SPLINE_CURVE_WITH_KNOTS ( 'NONE', 3,
 ( #43321, #46996, #13242, #9342, #24842, #32697, #2665, #9593, #32232, #47248 ),
 .UNSPECIFIED., .F., .F.,
 ( 4, 2, 2, 2, 4 ),
 ( 0.6272669072976907456, 0.7522669073147264518, 0.8772669073317622690, 1.002266907348797975, 1.127266907365833681 ),
 .UNSPECIFIED. ) ;
#28200=CARTESIAN_POINT ( 'NONE',  ( -13.11946129443726861, -9.225960368241006293, 67.37942785707225823 ) ) ;
#28201=VERTEX_POINT ( 'NONE', #24567 ) ;
#28202=CARTESIAN_POINT ( 'NONE',  ( -13.91686280105865947, -8.236299372188803147, 74.31459218752463869 ) ) ;
#28204=PLANE ( 'NONE',  #47076 ) ;
#28205=ORIENTED_EDGE ( 'NONE', *, *, #35013, .T. ) ;
#28209=ORIENTED_EDGE ( 'NONE', *, *, #11390, .F. ) ;
#28211=ORIENTED_EDGE ( 'NONE', *, *, #17229, .T. ) ;
#28212=CARTESIAN_POINT ( 'NONE',  ( -14.07761608144266674, -20.95746532167037302, 71.92607703845176559 ) ) ;
#28214=CARTESIAN_POINT ( 'NONE',  ( -23.76770236311157802, -11.84941793196945881, 59.78235735876457824 ) ) ;
#28215=CARTESIAN_POINT ( 'NONE',  ( -14.98927377128267047, -8.246306944878837086, 57.14999999999994884 ) ) ;
#28220=ADVANCED_FACE ( 'NONE', ( #46951 ), #13197, .T. ) ;
#28221=CARTESIAN_POINT ( 'NONE',  ( -21.53994948931798703, -21.01915008201228474, 72.78092378945153484 ) ) ;
#28222=CARTESIAN_POINT ( 'NONE',  ( -20.66696855643225561, -21.06909979829504209, 58.94475164909854925 ) ) ;
#28227=CARTESIAN_POINT ( 'NONE',  ( -10.37462439815953275, -14.89569326811688832, 74.94778901494476031 ) ) ;
#28228=FACE_OUTER_BOUND ( 'NONE', #449, .T. ) ;
#28229=EDGE_CURVE ( 'NONE', #23858, #16276, #32605, .T. ) ;
#28231=B_SPLINE_CURVE_WITH_KNOTS ( 'NONE', 1,
 ( #23673, #15765 ),
 .UNSPECIFIED., .F., .F.,
 ( 2, 2 ),
 ( 0.000000000000000000, 1.000000000000000000 ),
 .UNSPECIFIED. ) ;
#28232=CARTESIAN_POINT ( 'NONE',  ( -24.43499015649444317, -15.57872826220114781, 69.41818628325123086 ) ) ;
#28233=( BOUNDED_SURFACE ( )  B_SPLINE_SURFACE ( 3, 1, ( 
 ( #18229, #29330 ),
 ( #6680, #10391 ),
 ( #35979, #44138 ),
 ( #48041, #2969 ),
 ( #2260, #25627 ),
 ( #14508, #17982 ),
 ( #25397, #21225 ) ),
 .UNSPECIFIED., .T., .F., .F. ) 
 B_SPLINE_SURFACE_WITH_KNOTS ( ( 4, 3, 4 ),
 ( 2, 2 ),
 ( 0.000000000000000000, 0.5000000000000000000, 1.000000000000000000 ),
 ( 0.000000000000000000, 1.000000000000000000 ),
 .UNSPECIFIED. ) 
 GEOMETRIC_REPRESENTATION_ITEM ( )  RATIONAL_B_SPLINE_SURFACE ( (
 ( 1.000000000000000000, 1.000000000000000000),
 ( 0.3333333333333335369, 0.3333333333333330373),
 ( 0.3333333333333335369, 0.3333333333333330373),
 ( 1.000000000000000000, 1.000000000000000000),
 ( 0.3333333333333333703, 0.3333333333333333703),
 ( 0.3333333333333333703, 0.3333333333333333703),
 ( 1.000000000000000000, 1.000000000000000000) ) ) 
 REPRESENTATION_ITEM ( '' )  SURFACE ( )  );
#28234=EDGE_CURVE ( 'NONE', #34362, #21018, #7055, .T. ) ;
#28238=VECTOR ( 'NONE', #31410, 1000.000000000000227 ) ;
#28239=CARTESIAN_POINT ( 'NONE',  ( -10.69985271022639317, -16.93744915505940085, 61.57231810286263141 ) ) ;
#28240=CARTESIAN_POINT ( 'NONE',  ( -11.01006245036516162, -12.00545227084238320, 74.57342739614527716 ) ) ;
#28243=ORIENTED_EDGE ( 'NONE', *, *, #1067, .T. ) ;
#28245=CARTESIAN_POINT ( 'NONE',  ( -19.44376822123183146, -7.638105259791415413, 60.07597700946195829 ) ) ;
#28249=DIRECTION ( 'NONE',  ( 0.9466432954593471116, 0.3222832157619555660, 8.771047036255756069E-09 ) ) ;
#28250=EDGE_LOOP ( 'NONE', ( #22988, #12642, #29078, #44304, #12940 ) ) ;
#28251=CARTESIAN_POINT ( 'NONE',  ( -11.76596577686094847, -10.68774762964470604, 74.45387372083885680 ) ) ;
#28252=CARTESIAN_POINT ( 'NONE',  ( -10.37382936219775154, -14.83089353207902050, 74.81251018390587149 ) ) ;
#28254=CYLINDRICAL_SURFACE ( 'NONE', #27390, 0.1500000000000079881 ) ;
#28255=CARTESIAN_POINT ( 'NONE',  ( -20.04849592361258104, -21.35284569240296548, 72.69006679631317525 ) ) ;
#28256=FACE_OUTER_BOUND ( 'NONE', #26464, .T. ) ;
#28259=CARTESIAN_POINT ( 'NONE',  ( -10.95917937052863245, -17.62195967018737264, 71.58190244267143498 ) ) ;
#28260=UNCERTAINTY_MEASURE_WITH_UNIT (LENGTH_MEASURE( 1.000000000000000082E-05 ), #8127, 'distance_accuracy_value', 'NONE');
#28261=DIRECTION ( 'NONE',  ( 6.023555219429074381E-06, -1.003033500007733605E-05, 0.9999999999315545285 ) ) ;
#28262=CARTESIAN_POINT ( 'NONE',  ( -23.79376783276477525, -17.83917320997471023, 62.56540969546114894 ) ) ;
#28263=EDGE_LOOP ( 'NONE', ( #4963, #48442, #25969, #22082, #15296 ) ) ;
#28264=CARTESIAN_POINT ( 'NONE',  ( -15.93879930885703011, -7.917138641544859468, 67.15479422225766371 ) ) ;
#28265=DIRECTION ( 'NONE',  ( 0.9939059412784551073, 0.1102314832132140626, 5.576311685107536405E-08 ) ) ;
#28266=EDGE_LOOP ( 'NONE', ( #28362, #13655, #43295, #1035, #2055 ) ) ;
#28268=CARTESIAN_POINT ( 'NONE',  ( -23.77487038158592014, -11.74745262826995607, 62.96690348473899235 ) ) ;
#28272=CYLINDRICAL_SURFACE ( 'NONE', #10972, 0.1500000000000015488 ) ;
#28273=CARTESIAN_POINT ( 'NONE',  ( -24.46479344033866710, -14.44719916248949154, 66.33292729247949637 ) ) ;
#28274=EDGE_CURVE ( 'NONE', #29708, #30119, #13317, .T. ) ;
#28275=CARTESIAN_POINT ( 'NONE',  ( -23.48344415125163565, -18.41350569598871090, 73.04896097104848707 ) ) ;
#28276=LINE ( 'NONE', #40550, #5092 ) ;
#28278=VECTOR ( 'NONE', #19355, 1000.000000000000114 ) ;
#28279=CARTESIAN_POINT ( 'NONE',  ( -16.70524046451162548, -22.22456740133032227, 68.87373416885567678 ) ) ;
#28280=ORIENTED_EDGE ( 'NONE', *, *, #14251, .T. ) ;
#28281=EDGE_LOOP ( 'NONE', ( #44703, #47107 ) ) ;
#28282=CARTESIAN_POINT ( 'NONE',  ( -11.06793303470118950, -10.92167721944563397, 60.86541164553911187 ) ) ;
#28283=EDGE_CURVE ( 'NONE', #39949, #5705, #19961, .T. ) ;
#28286=CARTESIAN_POINT ( 'NONE',  ( -11.41368471857665590, -18.49404720395463642, 61.27710860172267360 ) ) ;
#28289=CARTESIAN_POINT ( 'NONE',  ( -20.47136568995129480, -10.23054578351413468, 53.49899999999994549 ) ) ;
#28290=( BOUNDED_SURFACE ( )  B_SPLINE_SURFACE ( 3, 1, ( 
 ( #28887, #14554 ),
 ( #14083, #21516 ),
 ( #10191, #37225 ),
 ( #29376, #25205 ),
 ( #40224, #10433 ),
 ( #29617, #6495 ),
 ( #28653, #36497 ) ),
 .UNSPECIFIED., .T., .F., .F. ) 
 B_SPLINE_SURFACE_WITH_KNOTS ( ( 4, 3, 4 ),
 ( 2, 2 ),
 ( 0.000000000000000000, 0.5000000000000000000, 1.000000000000000000 ),
 ( 0.000000000000000000, 1.000000000000000000 ),
 .UNSPECIFIED. ) 
 GEOMETRIC_REPRESENTATION_ITEM ( )  RATIONAL_B_SPLINE_SURFACE ( (
 ( 1.000000000000000000, 1.000000000000000000),
 ( 0.3333333333333335369, 0.3333333333333330373),
 ( 0.3333333333333335369, 0.3333333333333330373),
 ( 1.000000000000000000, 1.000000000000000000),
 ( 0.3333333333333333703, 0.3333333333333333703),
 ( 0.3333333333333333703, 0.3333333333333333703),
 ( 1.000000000000000000, 1.000000000000000000) ) ) 
 REPRESENTATION_ITEM ( '' )  SURFACE ( )  );
#28291=EDGE_LOOP ( 'NONE', ( #14409, #22469, #32940, #47930, #3336 ) ) ;
#28292=CARTESIAN_POINT ( 'NONE',  ( -19.79646526366146375, -21.45124607735644062, 72.81967355032548994 ) ) ;
#28295=B_SPLINE_CURVE_WITH_KNOTS ( 'NONE', 3,
 ( #46214, #27254, #23321, #38317, #38570, #8801, #23818, #204, #38819, #20106 ),
 .UNSPECIFIED., .F., .F.,
 ( 4, 2, 2, 2, 4 ),
 ( 0.000000000000000000, 0.2500000000000000000, 0.5000000000000000000, 0.7500000000000000000, 1.000000000000000000 ),
 .UNSPECIFIED. ) ;
#28296=CARTESIAN_POINT ( 'NONE',  ( -14.73594855369633905, -7.860282982240396343, 60.50651534380390473 ) ) ;
#28298=EDGE_CURVE ( 'NONE', #12632, #42290, #41507, .T. ) ;
#28299=ORIENTED_EDGE ( 'NONE', *, *, #16767, .T. ) ;
#28300=( BOUNDED_CURVE ( )  B_SPLINE_CURVE ( 3, ( #15344, #361, #44942, #26942 ),
 .UNSPECIFIED., .F., .F. ) 
 B_SPLINE_CURVE_WITH_KNOTS ( ( 4, 4 ),
 ( 0.4074455897393673420, 0.5000000000000000000 ),
 .UNSPECIFIED. ) 
 CURVE ( )  GEOMETRIC_REPRESENTATION_ITEM ( )  RATIONAL_B_SPLINE_CURVE ( ( 0.6983129098260978385, 0.7760317562607030872, 0.8765941196520039558, 1.000000000000001110 ) ) 
 REPRESENTATION_ITEM ( '' )  );
#28301=CARTESIAN_POINT ( 'NONE',  ( -11.21695167451617792, -18.92928555840075688, 64.79061121450172323 ) ) ;
#28302=EDGE_CURVE ( 'NONE', #35582, #11018, #30046, .T. ) ;
#28304=CARTESIAN_POINT ( 'NONE',  ( -16.71219879347879100, -22.22520166962337740, 68.81065243885818461 ) ) ;
#28306=CARTESIAN_POINT ( 'NONE',  ( -10.53536195276627829, -13.30851587854854401, 74.69289754060230280 ) ) ;
#28307=CARTESIAN_POINT ( 'NONE',  ( -17.39742543611924575, -7.759256981132185871, 67.32039592192056432 ) ) ;
#28308=EDGE_CURVE ( 'NONE', #6954, #4804, #30273, .T. ) ;
#28310=CARTESIAN_POINT ( 'NONE',  ( -18.92057629138644970, -7.919864069981281673, 67.05071783789199458 ) ) ;
#28312=CARTESIAN_POINT ( 'NONE',  ( -13.01616685277437568, -9.306763517318225709, 70.86397465682092900 ) ) ;
#28313=VECTOR ( 'NONE', #43730, 1000.000000000000227 ) ;
#28314=ORIENTED_EDGE ( 'NONE', *, *, #5933, .F. ) ;
#28316=B_SPLINE_CURVE_WITH_KNOTS ( 'NONE', 3,
 ( #14805, #14557, #13846, #10665, #7229, #40691, #40944, #29618, #36499, #36274 ),
 .UNSPECIFIED., .F., .F.,
 ( 4, 2, 2, 2, 4 ),
 ( 0.1272669073658274363, 0.2522669073463031930, 0.3772669073267790329, 0.5022669073072547619, 0.6272669072877306018 ),
 .UNSPECIFIED. ) ;
#28318=ORIENTED_EDGE ( 'NONE', *, *, #47660, .T. ) ;
#28319=DIRECTION ( 'NONE',  ( 0.6323592902076723421, 0.7746752403995150749, -4.984538757074893987E-08 ) ) ;
#28322=CARTESIAN_POINT ( 'NONE',  ( -12.01398192529223685, -10.36526672924184389, 71.19723003267655770 ) ) ;
#28324=CARTESIAN_POINT ( 'NONE',  ( -19.79948111938147548, -8.167596747518278022, 73.92916665838981771 ) ) ;
#28325=CARTESIAN_POINT ( 'NONE',  ( -10.88209246082447912, -17.29963176008448400, 64.92739380462948873 ) ) ;
#28327=CARTESIAN_POINT ( 'NONE',  ( -23.86889929688984324, -17.54148027364508877, 62.48863461348566517 ) ) ;
#28328=DIRECTION ( 'NONE',  ( -0.4639960340712762088, 0.8858372764600319638, 1.164945627098518506E-17 ) ) ;
#28331=ORIENTED_EDGE ( 'NONE', *, *, #23650, .T. ) ;
#28332=ORIENTED_EDGE ( 'NONE', *, *, #46106, .T. ) ;
#28333=CARTESIAN_POINT ( 'NONE',  ( -11.68335550665270794, -18.81469308649876737, 68.21689631955439381 ) ) ;
#28334=CARTESIAN_POINT ( 'NONE',  ( -24.31977367176101268, -16.01319989648291653, 62.78431746014856429 ) ) ;
#28335=EDGE_LOOP ( 'NONE', ( #44118, #16169 ) ) ;
#28336=CARTESIAN_POINT ( 'NONE',  ( -24.33438867869370981, -15.92703613221075543, 66.36324874061841683 ) ) ;
#28338=CARTESIAN_POINT ( 'NONE',  ( -23.83107790926975511, -11.00715885964709173, 73.50159964070205376 ) ) ;
#28344=CARTESIAN_POINT ( 'NONE',  ( -10.42874009550524761, -15.68648592809493358, 61.33229246353490538 ) ) ;
#28346=CARTESIAN_POINT ( 'NONE',  ( -24.47432067347917695, -14.77756146504815327, 59.52828185648635184 ) ) ;
#28348=ADVANCED_FACE ( 'NONE', ( #34108, #398 ), #26744, .F. ) ;
#28349=VECTOR ( 'NONE', #1292, 1000.000000000000114 ) ;
#28352=EDGE_LOOP ( 'NONE', ( #22067, #37419, #31999, #42938, #10728 ) ) ;
#28355=EDGE_CURVE ( 'NONE', #1165, #31902, #40203, .T. ) ;
#28356=CARTESIAN_POINT ( 'NONE',  ( -15.35027035934970918, -7.653577032698213323, 74.26481056556292515 ) ) ;
#28357=AXIS2_PLACEMENT_3D ( 'NONE', #7362, #26799, #45042 ) ;
#28358=ORIENTED_EDGE ( 'NONE', *, *, #22104, .F. ) ;
#28362=ORIENTED_EDGE ( 'NONE', *, *, #43199, .F. ) ;
#28363=CARTESIAN_POINT ( 'NONE',  ( -13.26872317195175199, -21.05283485551296607, 53.49999999999994316 ) ) ;
#28364=ADVANCED_FACE ( 'NONE', ( #20318 ), #5871, .T. ) ;
#28365=CARTESIAN_POINT ( 'NONE',  ( -12.96549398033168288, -9.412670339977610823, 70.84925319149679979 ) ) ;
#28366=ORIENTED_EDGE ( 'NONE', *, *, #29572, .F. ) ;
#28368=VERTEX_POINT ( 'NONE', #45714 ) ;
#28369=CARTESIAN_POINT ( 'NONE',  ( -17.52853272358826686, -7.759682304905023642, 63.83584969886392457 ) ) ;
#28371=CARTESIAN_POINT ( 'NONE',  ( -15.73993337224566247, -7.955115359200574332, 63.82577855974437853 ) ) ;
#28373=CARTESIAN_POINT ( 'NONE',  ( -19.23866243364646422, -21.62168334911581269, 58.52507384657483414 ) ) ;
#28379=ADVANCED_FACE ( 'NONE', ( #1342 ), #38276, .T. ) ;
#28381=CARTESIAN_POINT ( 'NONE',  ( -22.48964968825576705, -9.905448439006629968, 73.76689030015370463 ) ) ;
#28382=LINE ( 'NONE', #1788, #27424 ) ;
#28385=CARTESIAN_POINT ( 'NONE',  ( -17.51532316199698158, -7.809739782127767427, 63.83591710975426992 ) ) ;
#28386=ADVANCED_FACE ( 'NONE', ( #9243 ), #4333, .T. ) ;
#28387=FACE_OUTER_BOUND ( 'NONE', #42046, .T. ) ;
#28389=CARTESIAN_POINT ( 'NONE',  ( -13.41658284876181995, -21.09041002232991957, 61.62990919978891924 ) ) ;
#28390=CARTESIAN_POINT ( 'NONE',  ( -10.99582178678916833, -11.91441492378913658, 74.85840195586327184 ) ) ;
#28391=EDGE_CURVE ( 'NONE', #9477, #43598, #29019, .T. ) ;
#28392=CARTESIAN_POINT ( 'NONE',  ( -24.28474004986992796, -16.19955753861012582, 62.89328727869452962 ) ) ;
#28393=ORIENTED_EDGE ( 'NONE', *, *, #13193, .T. ) ;
#28394=CARTESIAN_POINT ( 'NONE',  ( -22.67088471252091963, -10.17541515747705461, 66.61470292127093273 ) ) ;
#28395=CARTESIAN_POINT ( 'NONE',  ( -24.83263366448169762, -15.59490076022755112, 73.18799035805197661 ) ) ;
#28400=DIRECTION ( 'NONE',  ( -5.731567514496413899E-31, -1.020425574103664789E-16, -1.000000000000000000 ) ) ;
#28401=ORIENTED_EDGE ( 'NONE', *, *, #40291, .T. ) ;
#28402=CARTESIAN_POINT ( 'NONE',  ( -23.76058108042893480, -11.83148235802054415, 63.18048099588689581 ) ) ;
#28406=VECTOR ( 'NONE', #26734, 1000.000000000000227 ) ;
#28408=DIRECTION ( 'NONE',  ( 3.549360974554993999E-17, -6.371834667797928663E-18, -1.000000000000000000 ) ) ;
#28409=CARTESIAN_POINT ( 'NONE',  ( -10.40385083531699273, -12.31531819518022353, 57.52131499152729788 ) ) ;
#28410=CARTESIAN_POINT ( 'NONE',  ( -21.04010759901128225, -20.80440105208702661, 69.28280143620438025 ) ) ;
#28411=CARTESIAN_POINT ( 'NONE',  ( -20.47136568995129480, -10.23054578351413468, 54.07175714974879099 ) ) ;
#28414=VERTEX_POINT ( 'NONE', #27704 ) ;
#28417=CARTESIAN_POINT ( 'NONE',  ( -13.49267557974227394, -8.956801037788498121, 60.45422421514565059 ) ) ;
#28418=VECTOR ( 'NONE', #37410, 1000.000000000000000 ) ;
#28420=CARTESIAN_POINT ( 'NONE',  ( -14.20477006803791475, -8.593354865760924000, 71.01492291173906324 ) ) ;
#28421=CARTESIAN_POINT ( 'NONE',  ( -14.02541561442408913, -20.92883260698763692, 68.52913103262484640 ) ) ;
#28422=EDGE_LOOP ( 'NONE', ( #37158, #44314 ) ) ;
#28423=CARTESIAN_POINT ( 'NONE',  ( -11.02842221325288996, -10.98838527758271155, 60.78611644236347189 ) ) ;
#28425=CARTESIAN_POINT ( 'NONE',  ( -24.05420634179087358, -17.20676946999824608, 69.69867738674849988 ) ) ;
#28426=( BOUNDED_CURVE ( )  B_SPLINE_CURVE ( 3, ( #24762, #43967, #2812, #36057 ),
 .UNSPECIFIED., .F., .F. ) 
 B_SPLINE_CURVE_WITH_KNOTS ( ( 4, 4 ),
 ( 4.712388980384691450, 4.921828490624010399 ),
 .UNSPECIFIED. ) 
 CURVE ( )  GEOMETRIC_REPRESENTATION_ITEM ( )  RATIONAL_B_SPLINE_CURVE ( ( 1.000000000000000000, 0.9963479302455156006, 0.9963479302455156006, 1.000000000000000000 ) ) 
 REPRESENTATION_ITEM ( '' )  );
#28427=ORIENTED_EDGE ( 'NONE', *, *, #27739, .T. ) ;
#28428=B_SPLINE_CURVE_WITH_KNOTS ( 'NONE', 1,
 ( #44216, #43965 ),
 .UNSPECIFIED., .F., .F.,
 ( 2, 2 ),
 ( 0.000000000000000000, 1.000000000000000000 ),
 .UNSPECIFIED. ) ;
#28429=CARTESIAN_POINT ( 'NONE',  ( -17.99994007944887286, -22.23708576427155137, 62.01389424133448358 ) ) ;
#28430=LINE ( 'NONE', #5544, #6265 ) ;
#28431=EDGE_LOOP ( 'NONE', ( #12514, #2589 ) ) ;
#28433=CARTESIAN_POINT ( 'NONE',  ( -14.93633297159279216, -21.40954675051312250, 58.37437924742020101 ) ) ;
#28438=B_SPLINE_CURVE_WITH_KNOTS ( 'NONE', 3,
 ( #2572, #24748, #25225, #21041, #9960, #24980, #40249, #6266, #6514, #36290 ),
 .UNSPECIFIED., .F., .F.,
 ( 4, 2, 2, 2, 4 ),
 ( 0.000000000000000000, 0.2500000000000000000, 0.5000000000000000000, 0.7500000000000000000, 1.000000000000000000 ),
 .UNSPECIFIED. ) ;
#28439=( BOUNDED_CURVE ( )  B_SPLINE_CURVE ( 3, ( #13908, #14145, #25740, #28950 ),
 .UNSPECIFIED., .F., .F. ) 
 B_SPLINE_CURVE_WITH_KNOTS ( ( 4, 4 ),
 ( 0.9074455897393647330, 1.000000000000000000 ),
 .UNSPECIFIED. ) 
 CURVE ( )  GEOMETRIC_REPRESENTATION_ITEM ( )  RATIONAL_B_SPLINE_CURVE ( ( 0.6983129098260816292, 0.7760317562606884323, 0.8765941196519945189, 1.000000000000000000 ) ) 
 REPRESENTATION_ITEM ( '' )  );
#28440=CARTESIAN_POINT ( 'NONE',  ( -23.23616409499837943, -18.79948708312782557, 65.82389430043846801 ) ) ;
#28442=ORIENTED_EDGE ( 'NONE', *, *, #19637, .F. ) ;
#28443=CARTESIAN_POINT ( 'NONE',  ( -22.04378365035703879, -20.13510231884741231, 62.24911246861644543 ) ) ;
#28444=( BOUNDED_CURVE ( )  B_SPLINE_CURVE ( 3, ( #43930, #2060, #43193, #1820 ),
 .UNSPECIFIED., .F., .F. ) 
 B_SPLINE_CURVE_WITH_KNOTS ( ( 4, 4 ),
 ( 0.9074455897393670645, 1.000000000000000000 ),
 .UNSPECIFIED. ) 
 CURVE ( )  GEOMETRIC_REPRESENTATION_ITEM ( )  RATIONAL_B_SPLINE_CURVE ( ( 0.6983129098260988377, 0.7760317562607031983, 0.8765941196520036227, 1.000000000000000000 ) ) 
 REPRESENTATION_ITEM ( '' )  );
#28445=LINE ( 'NONE', #9964, #30239 ) ;
#28447=CARTESIAN_POINT ( 'NONE',  ( -15.53817126359833445, -8.015982722819853024, 74.08545464501875699 ) ) ;
#28449=ADVANCED_FACE ( 'NONE', ( #38782 ), #14019, .T. ) ;
#28450=ADVANCED_FACE ( 'NONE', ( #36044 ), #24517, .F. ) ;
#28451=CARTESIAN_POINT ( 'NONE',  ( -20.20088676517873694, -8.325823464045813083, 74.13585170226248522 ) ) ;
#28452=CARTESIAN_POINT ( 'NONE',  ( -11.47771132772901659, -11.11285210769868748, 60.86812947373131522 ) ) ;
#28453=VECTOR ( 'NONE', #28143, 1000.000000000000114 ) ;
#28455=EDGE_LOOP ( 'NONE', ( #30676, #41222, #33998, #21859, #21008 ) ) ;
#28456=CARTESIAN_POINT ( 'NONE',  ( -16.65185932245351452, -21.81708442718849383, 65.51092266128213737 ) ) ;
#28457=CARTESIAN_POINT ( 'NONE',  ( -14.24639973016467742, -8.070891362069774644, 67.45963869169959537 ) ) ;
#28458=LINE ( 'NONE', #43481, #22774 ) ;
#28460=CARTESIAN_POINT ( 'NONE',  ( -13.57571756020798581, -20.65642803140422856, 61.51646323935151628 ) ) ;
#28461=( BOUNDED_CURVE ( )  B_SPLINE_CURVE ( 3, ( #868, #18404, #7107, #48210 ),
 .UNSPECIFIED., .F., .F. ) 
 B_SPLINE_CURVE_WITH_KNOTS ( ( 4, 4 ),
 ( 0.9074455897393649551, 1.000000000000000000 ),
 .UNSPECIFIED. ) 
 CURVE ( )  GEOMETRIC_REPRESENTATION_ITEM ( )  RATIONAL_B_SPLINE_CURVE ( ( 0.6983129098260953960, 0.7760317562607003117, 0.8765941196520018464, 1.000000000000000000 ) ) 
 REPRESENTATION_ITEM ( '' )  );
#28462=VERTEX_POINT ( 'NONE', #13392 ) ;
#28463=ORIENTED_EDGE ( 'NONE', *, *, #29300, .T. ) ;
#28464=ORIENTED_EDGE ( 'NONE', *, *, #11328, .F. ) ;
#28465=CARTESIAN_POINT ( 'NONE',  ( -18.75169300116608184, -7.478281097746903860, 70.50921473615289869 ) ) ;
#28467=CARTESIAN_POINT ( 'NONE',  ( -16.00300465971815811, -7.954912822689343521, 63.68513404597024419 ) ) ;
#28468=CARTESIAN_POINT ( 'NONE',  ( -15.39536932222403287, -19.92137602241599836, 54.07175714974879099 ) ) ;
#28473=B_SPLINE_CURVE_WITH_KNOTS ( 'NONE', 3,
 ( #46944, #28954, #28240, #9287, #12957, #16657, #24311, #39317, #43269, #9538 ),
 .UNSPECIFIED., .F., .F.,
 ( 4, 2, 2, 2, 4 ),
 ( 0.000000000000000000, 0.2500000000000000000, 0.5000000000000000000, 0.7500000000000000000, 1.000000000000000000 ),
 .UNSPECIFIED. ) ;
#28474=EDGE_CURVE ( 'NONE', #15704, #30331, #19085, .T. ) ;
#28475=CARTESIAN_POINT ( 'NONE',  ( -20.89788161767221197, -20.94431024770144489, 62.39999296070408974 ) ) ;
#28476=CARTESIAN_POINT ( 'NONE',  ( -23.19494587819374942, -18.77118419879135303, 66.12389430422854275 ) ) ;
#28478=ORIENTED_EDGE ( 'NONE', *, *, #30081, .F. ) ;
#28480=AXIS2_PLACEMENT_3D ( 'NONE', #23027, #7765, #29916 ) ;
#28482=CARTESIAN_POINT ( 'NONE',  ( -9.985306297970870659, -8.645400713382203506, 54.50428052266513390 ) ) ;
#28484=DIRECTION ( 'NONE',  ( 0.6264825908887947659, -0.7794354131762692983, 3.858680029754496854E-08 ) ) ;
#28485=CARTESIAN_POINT ( 'NONE',  ( -17.79084088774826000, -7.768752266068900347, 60.08060768310445354 ) ) ;
#28486=CARTESIAN_POINT ( 'NONE',  ( -11.33476804054750531, -19.10151225439055978, 68.40184904730287485 ) ) ;
#28487=CARTESIAN_POINT ( 'NONE',  ( -21.99229891970641404, -20.18939897536854389, 65.84854503242263490 ) ) ;
#28489=CARTESIAN_POINT ( 'NONE',  ( -19.36518065869528726, -8.031383756764064685, 59.97565108339750850 ) ) ;
#28490=CARTESIAN_POINT ( 'NONE',  ( -22.66414149941106260, -10.08832384041532926, 66.42693508874704378 ) ) ;
#28492=EDGE_LOOP ( 'NONE', ( #15163, #42038 ) ) ;
#28494=ORIENTED_EDGE ( 'NONE', *, *, #43538, .T. ) ;
#28495=CARTESIAN_POINT ( 'NONE',  ( -13.29979614553676370, -21.01354653661592664, 61.77292273241334186 ) ) ;
#28496=CARTESIAN_POINT ( 'NONE',  ( -10.37210014130659275, -14.68995570394611505, 75.21267707208666309 ) ) ;
#28497=B_SPLINE_CURVE_WITH_KNOTS ( 'NONE', 3,
 ( #33159, #21854, #36849, #25793, #33396, #19875, #8307, #916, #27253, #46212 ),
 .UNSPECIFIED., .F., .F.,
 ( 4, 2, 2, 2, 4 ),
 ( 0.6272669072877905538, 0.7522669073073057211, 0.8772669073268208884, 1.002266907346335945, 1.127266907365851223 ),
 .UNSPECIFIED. ) ;
#28498=ORIENTED_EDGE ( 'NONE', *, *, #32406, .F. ) ;
#28499=ADVANCED_FACE ( 'NONE', ( #43218 ), #39272, .T. ) ;
#28500=CARTESIAN_POINT ( 'NONE',  ( -11.01460970429776332, -11.87269385784942344, 74.56399918325968201 ) ) ;
#28501=CARTESIAN_POINT ( 'NONE',  ( -10.39147815561416621, -17.41829018061022438, 53.49999999999995026 ) ) ;
#28502=CARTESIAN_POINT ( 'NONE',  ( -24.48759320265496342, -17.17788619462897159, 72.92690118282537526 ) ) ;
#28504=ORIENTED_EDGE ( 'NONE', *, *, #27323, .T. ) ;
#28505=CARTESIAN_POINT ( 'NONE',  ( -22.01903163361388494, -9.527854677399155037, 59.73787834519894346 ) ) ;
#28506=CARTESIAN_POINT ( 'NONE',  ( -24.20884313412962285, -11.73171478914054155, 59.59740407230526671 ) ) ;
#28509=CARTESIAN_POINT ( 'NONE',  ( -11.17855889551124982, -18.87086522978130532, 64.86211687253867808 ) ) ;
#28511=EDGE_CURVE ( 'NONE', #21615, #26298, #6708, .T. ) ;
#28512=CARTESIAN_POINT ( 'NONE',  ( -19.55442184481404766, -21.52995072282663358, 65.47958309245051112 ) ) ;
#28513=ORIENTED_EDGE ( 'NONE', *, *, #33873, .F. ) ;
#28514=VERTEX_POINT ( 'NONE', #29333 ) ;
#28515=ADVANCED_FACE ( 'NONE', ( #18473 ), #1847, .T. ) ;
#28516=CARTESIAN_POINT ( 'NONE',  ( -14.05371270701021302, -21.00138147690670820, 71.92607703580544865 ) ) ;
#28518=CARTESIAN_POINT ( 'NONE',  ( -10.70296955259081351, -11.59513340129999648, 71.27356289404251299 ) ) ;
#28522=CARTESIAN_POINT ( 'NONE',  ( -23.47191072790384325, -19.15987225631625179, 62.53123744227819003 ) ) ;
#28523=CARTESIAN_POINT ( 'NONE',  ( -19.45760789423921366, -7.641931476291664360, 60.10059647935476335 ) ) ;
#28524=CARTESIAN_POINT ( 'NONE',  ( -14.94536180354596411, -8.261047468840590824, 60.43069275610791635 ) ) ;
#28525=CARTESIAN_POINT ( 'NONE',  ( -12.19280364807469752, -20.11379078549368771, 65.00641491777591341 ) ) ;
#28526=CARTESIAN_POINT ( 'NONE',  ( -16.75922336650640787, -22.22948809395919056, 68.89549426778991403 ) ) ;
#28527=VERTEX_POINT ( 'NONE', #29827 ) ;
#28528=EDGE_LOOP ( 'NONE', ( #45292, #10428, #27118, #33965, #37263 ) ) ;
#28531=CARTESIAN_POINT ( 'NONE',  ( -18.31357888663955080, -21.80286911112441217, 69.11514702303101387 ) ) ;
#28533=( BOUNDED_CURVE ( )  B_SPLINE_CURVE ( 3, ( #43872, #6182, #14263, #32525 ),
 .UNSPECIFIED., .F., .F. ) 
 B_SPLINE_CURVE_WITH_KNOTS ( ( 4, 4 ),
 ( 0.4074455897393690629, 0.5000000000000000000 ),
 .UNSPECIFIED. ) 
 CURVE ( )  GEOMETRIC_REPRESENTATION_ITEM ( )  RATIONAL_B_SPLINE_CURVE ( ( 0.6983129098261053880, 0.7760317562607058628, 0.8765941196520032896, 0.9999999999999953371 ) ) 
 REPRESENTATION_ITEM ( '' )  );
#28534=FACE_OUTER_BOUND ( 'NONE', #12635, .T. ) ;
#28535=B_SPLINE_CURVE_WITH_KNOTS ( 'NONE', 1,
 ( #26253, #10514 ),
 .UNSPECIFIED., .F., .F.,
 ( 2, 2 ),
 ( 0.000000000000000000, 1.000000000000000000 ),
 .UNSPECIFIED. ) ;
#28540=CARTESIAN_POINT ( 'NONE',  ( -14.53996353315453405, -7.939311612974331744, 60.43341030124493329 ) ) ;
#28541=CARTESIAN_POINT ( 'NONE',  ( -10.02210521578421520, -15.65432817399831045, 61.29434977362033976 ) ) ;
#28542=VERTEX_POINT ( 'NONE', #48279 ) ;
#28543=DIRECTION ( 'NONE',  ( 9.009792911740839922E-08, -1.813722297350279449E-06, 0.9999999999983510968 ) ) ;
#28544=CARTESIAN_POINT ( 'NONE',  ( -10.71238150236930053, -12.63946889494751957, 57.32857335981114488 ) ) ;
#28545=CARTESIAN_POINT ( 'NONE',  ( -15.63470697856566005, -7.577119469675131391, 70.77136384377372735 ) ) ;
#28546=CARTESIAN_POINT ( 'NONE',  ( -23.49747408472488885, -11.32843530181038538, 69.89210718181772108 ) ) ;
#28548=DIRECTION ( 'NONE',  ( 0.3224496555704359779, 0.8691421305882571779, -0.3749909018349807388 ) ) ;
#28549=ORIENTED_EDGE ( 'NONE', *, *, #9134, .T. ) ;
#28552=CYLINDRICAL_SURFACE ( 'NONE', #34402, 0.1500000000000023259 ) ;
#28553=CARTESIAN_POINT ( 'NONE',  ( -11.32087020534491018, -19.08159367390965855, 68.41678398564933161 ) ) ;
#28554=B_SPLINE_CURVE_WITH_KNOTS ( 'NONE', 3,
 ( #47986, #33932, #14954, #40580, #7612, #37614, #14694, #22136, #37120, #22369 ),
 .UNSPECIFIED., .F., .F.,
 ( 4, 2, 2, 2, 4 ),
 ( 0.000000000000000000, 0.2500000000000000000, 0.5000000000000000000, 0.7500000000000000000, 1.000000000000000000 ),
 .UNSPECIFIED. ) ;
#28556=ADVANCED_FACE ( 'NONE', ( #22193 ), #47996, .T. ) ;
#28557=CARTESIAN_POINT ( 'NONE',  ( -18.36938558548794376, -21.74637715204813304, 72.51340886358296700 ) ) ;
#28559=EDGE_LOOP ( 'NONE', ( #45471, #5079 ) ) ;
#28561=CARTESIAN_POINT ( 'NONE',  ( -24.07098339466274339, -12.61366525430951313, 73.24225587970839513 ) ) ;
#28562=CARTESIAN_POINT ( 'NONE',  ( -10.93709114749119493, -17.43956697397788602, 64.81842637974052934 ) ) ;
#28563=ORIENTED_EDGE ( 'NONE', *, *, #3535, .F. ) ;
#28564=DIRECTION ( 'NONE',  ( 5.255974126583346196E-06, -1.684062807769209861E-06, -0.9999999999847694054 ) ) ;
#28566=CARTESIAN_POINT ( 'NONE',  ( -10.66022861425853563, -12.82094205862782310, 64.56836097215892778 ) ) ;
#28567=FACE_OUTER_BOUND ( 'NONE', #11396, .T. ) ;
#28569=ORIENTED_EDGE ( 'NONE', *, *, #46979, .T. ) ;
#28570=ORIENTED_EDGE ( 'NONE', *, *, #46151, .F. ) ;
#28571=EDGE_CURVE ( 'NONE', #31006, #17131, #29636, .T. ) ;
#28573=CARTESIAN_POINT ( 'NONE',  ( -24.28168432700398682, -13.15745033048042067, 66.60246978931142792 ) ) ;
#28574=VERTEX_POINT ( 'NONE', #32 ) ;
#28575=CARTESIAN_POINT ( 'NONE',  ( -17.63870566664756723, -7.812497183136798640, 60.18946821813101877 ) ) ;
#28577=EDGE_CURVE ( 'NONE', #10912, #14795, #15263, .T. ) ;
#28580=FACE_OUTER_BOUND ( 'NONE', #10778, .T. ) ;
#28583=CARTESIAN_POINT ( 'NONE',  ( -20.88147674714181079, -8.209942860146695054, 60.02620543942160225 ) ) ;
#28584=CARTESIAN_POINT ( 'NONE',  ( -22.88419684932020459, -10.42887832691348926, 63.37185995611467604 ) ) ;
#28585=DIRECTION ( 'NONE',  ( -0.9477661110324759886, 0.3189661404888856633, -2.738326504218743831E-08 ) ) ;
#28587=ADVANCED_FACE ( 'NONE', ( #15997 ), #7921, .T. ) ;
#28588=( BOUNDED_CURVE ( )  B_SPLINE_CURVE ( 3, ( #48379, #14139, #3329, #18331 ),
 .UNSPECIFIED., .F., .F. ) 
 B_SPLINE_CURVE_WITH_KNOTS ( ( 4, 4 ),
 ( 0.4074455897393634562, 0.5000000000000000000 ),
 .UNSPECIFIED. ) 
 CURVE ( )  GEOMETRIC_REPRESENTATION_ITEM ( )  RATIONAL_B_SPLINE_CURVE ( ( 0.6983129098260888457, 0.7760317562607014219, 0.8765941196520070644, 1.000000000000010880 ) ) 
 REPRESENTATION_ITEM ( '' )  );
#28589=EDGE_LOOP ( 'NONE', ( #43879, #17135, #23308, #34724, #19508 ) ) ;
#28590=ORIENTED_EDGE ( 'NONE', *, *, #12402, .F. ) ;
#28592=LINE ( 'NONE', #35479, #20931 ) ;
#28594=CARTESIAN_POINT ( 'NONE',  ( -23.88504970037045894, -11.09961929988695317, 70.03064220926479777 ) ) ;
#28595=EDGE_LOOP ( 'NONE', ( #38122, #23948, #28331, #24908, #27431 ) ) ;
#28597=CARTESIAN_POINT ( 'NONE',  ( -21.33694788700791278, -9.004934622526002741, 73.60128753634342047 ) ) ;
#28598=AXIS2_PLACEMENT_3D ( 'NONE', #41937, #19278, #15564 ) ;
#28599=ORIENTED_EDGE ( 'NONE', *, *, #37736, .T. ) ;
#28600=CARTESIAN_POINT ( 'NONE',  ( -10.99655682251556144, -18.57624055219563175, 57.99209882808910521 ) ) ;
#28601=CARTESIAN_POINT ( 'NONE',  ( -20.25191534917340874, -8.350868906188830820, 70.26572394742477456 ) ) ;
#28602=CARTESIAN_POINT ( 'NONE',  ( -21.96131106250977538, -8.900057530352752266, 66.78433116505721046 ) ) ;
#28603=EDGE_CURVE ( 'NONE', #26904, #9441, #19083, .T. ) ;
#28604=ORIENTED_EDGE ( 'NONE', *, *, #4646, .T. ) ;
#28606=VERTEX_POINT ( 'NONE', #38406 ) ;
#28607=CARTESIAN_POINT ( 'NONE',  ( -15.95864454847012581, -7.504678945485328434, 63.71365074502104875 ) ) ;
#28609=ORIENTED_EDGE ( 'NONE', *, *, #45906, .F. ) ;
#28610=CARTESIAN_POINT ( 'NONE',  ( -24.14381533474600161, -18.02640322225578373, 59.14345041050133034 ) ) ;
#28611=CARTESIAN_POINT ( 'NONE',  ( -20.18007907243378796, -21.73087789737553166, 72.54332250421934702 ) ) ;
#28613=CARTESIAN_POINT ( 'NONE',  ( -13.66248663715553846, -8.905660726476867239, 57.26967804941948970 ) ) ;
#28614=CARTESIAN_POINT ( 'NONE',  ( -18.68070144837527735, -7.415226739706411330, 53.49999999999994316 ) ) ;
#28616=ORIENTED_EDGE ( 'NONE', *, *, #38727, .F. ) ;
#28618=CARTESIAN_POINT ( 'NONE',  ( -11.97490362423377164, -10.33561459433851404, 67.78424783647008667 ) ) ;
#28619=CARTESIAN_POINT ( 'NONE',  ( -24.86646048052525515, -14.46934500410477753, 66.36105466539692088 ) ) ;
#28620=FACE_OUTER_BOUND ( 'NONE', #44382, .T. ) ;
#28621=CARTESIAN_POINT ( 'NONE',  ( -14.11399872369470998, -20.97726832089501059, 71.92607667771569879 ) ) ;
#28623=ORIENTED_EDGE ( 'NONE', *, *, #29153, .T. ) ;
#28624=EDGE_LOOP ( 'NONE', ( #31639, #8420, #1994, #6038, #31169 ) ) ;
#28626=CARTESIAN_POINT ( 'NONE',  ( -21.66599004997299360, -9.178097848147587001, 66.96149970124221795 ) ) ;
#28629=CARTESIAN_POINT ( 'NONE',  ( -23.48622163778175675, -11.20987317961282237, 73.36753114030383927 ) ) ;
#28630=CARTESIAN_POINT ( 'NONE',  ( -10.62449938266763638, -13.14622274244411315, 67.84718309729213104 ) ) ;
#28632=CARTESIAN_POINT ( 'NONE',  ( -17.97823402885549271, -22.23862238050489992, 62.06810083693206792 ) ) ;
#28633=CARTESIAN_POINT ( 'NONE',  ( -12.18719842096713180, -10.08886484896570934, 64.04386393395434141 ) ) ;
#28634=ADVANCED_FACE ( 'NONE', ( #26366 ), #4694, .T. ) ;
#28636=EDGE_LOOP ( 'NONE', ( #1871, #10438 ) ) ;
#28638=DIRECTION ( 'NONE',  ( 2.161108583753623267E-06, 4.147204431722191678E-06, 0.9999999999890650804 ) ) ;
#28643=CARTESIAN_POINT ( 'NONE',  ( -17.72419709140651278, -21.80277058947482516, 58.70553378253836030 ) ) ;
#28644=EDGE_CURVE ( 'NONE', #37610, #566, #30762, .T. ) ;
#28646=CARTESIAN_POINT ( 'NONE',  ( -24.16627971075339332, -12.73851560842801867, 66.18757903754330130 ) ) ;
#28648=CARTESIAN_POINT ( 'NONE',  ( -11.54449245800164903, -11.00967784149594308, 57.49286716219851456 ) ) ;
#28649=ORIENTED_EDGE ( 'NONE', *, *, #37769, .T. ) ;
#28650=VERTEX_POINT ( 'NONE', #45338 ) ;
#28652=CARTESIAN_POINT ( 'NONE',  ( -8.258083856565255232, -9.811588921218147519, 54.49999999999995026 ) ) ;
#28653=CARTESIAN_POINT ( 'NONE',  ( -11.97490362423377164, -10.33561459433851404, 67.78424783647008667 ) ) ;
#28654=EDGE_CURVE ( 'NONE', #39949, #42734, #30811, .T. ) ;
#28655=EDGE_CURVE ( 'NONE', #24440, #43669, #4977, .T. ) ;
#28656=CARTESIAN_POINT ( 'NONE',  ( -14.27319502748954783, -8.558459675072437989, 70.72957628730870283 ) ) ;
#28658=ORIENTED_EDGE ( 'NONE', *, *, #13969, .T. ) ;
#28659=CARTESIAN_POINT ( 'NONE',  ( -14.48548941065489970, -8.400516866317895293, 67.27447142263336843 ) ) ;
#28660=CARTESIAN_POINT ( 'NONE',  ( -21.12749503816145591, -21.27438112535048376, 62.22816062766979428 ) ) ;
#28661=ORIENTED_EDGE ( 'NONE', *, *, #28710, .T. ) ;
#28662=DIRECTION ( 'NONE',  ( 0.1539336739619741601, 0.9880811829098680166, 6.607022902453645889E-08 ) ) ;
#28663=EDGE_CURVE ( 'NONE', #41284, #24527, #27903, .T. ) ;
#28664=LINE ( 'NONE', #42953, #4679 ) ;
#28666=VERTEX_POINT ( 'NONE', #20191 ) ;
#28668=CARTESIAN_POINT ( 'NONE',  ( -12.26902398874117495, -19.54473763108856943, 58.22682373989366766 ) ) ;
#28669=ORIENTED_EDGE ( 'NONE', *, *, #24132, .F. ) ;
#28670=CARTESIAN_POINT ( 'NONE',  ( -13.93897074462874919, -20.93787812888889377, 68.74153005185598886 ) ) ;
#28674=CARTESIAN_POINT ( 'NONE',  ( -24.69675289721077505, -13.19280437224551505, 59.48455129494911375 ) ) ;
#28676=DIRECTION ( 'NONE',  ( -0.8547111024021492032, -0.5191039697695418731, -7.472447831848563370E-08 ) ) ;
#28677=CARTESIAN_POINT ( 'NONE',  ( -19.74200936563729769, -21.46758226568296024, 68.94954551542706156 ) ) ;
#28679=FACE_OUTER_BOUND ( 'NONE', #29895, .T. ) ;
#28680=CARTESIAN_POINT ( 'NONE',  ( -23.19948571119275726, -18.85291137746749968, 65.83861571032234394 ) ) ;
#28681=ORIENTED_EDGE ( 'NONE', *, *, #16145, .T. ) ;
#28682=CARTESIAN_POINT ( 'NONE',  ( -23.57909424710215518, -11.36400449684228775, 73.45373529196413642 ) ) ;
#28683=CARTESIAN_POINT ( 'NONE',  ( -18.53289088300742193, -21.77150771217549874, 72.58510914717624019 ) ) ;
#28684=CARTESIAN_POINT ( 'NONE',  ( -13.29033951192469587, -20.46027514905393119, 58.23577251623645878 ) ) ;
#28685=VERTEX_POINT ( 'NONE', #32005 ) ;
#28686=CARTESIAN_POINT ( 'NONE',  ( -12.27729936708703384, -9.991218733798060470, 60.70918086709614414 ) ) ;
#28687=ADVANCED_FACE ( 'NONE', ( #8883 ), #27339, .T. ) ;
#28688=VERTEX_POINT ( 'NONE', #24385 ) ;
#28689=ORIENTED_EDGE ( 'NONE', *, *, #41055, .F. ) ;
#28690=VERTEX_POINT ( 'NONE', #2202 ) ;
#28691=ADVANCED_FACE ( 'NONE', ( #27824 ), #27291, .T. ) ;
#28692=DIRECTION ( 'NONE',  ( -0.3478314405900309048, -0.9375570856950864451, 0.000000000000000000 ) ) ;
#28695=CARTESIAN_POINT ( 'NONE',  ( -12.63116919492461854, -9.104687665260810192, 70.96270001146038453 ) ) ;
#28696=ORIENTED_EDGE ( 'NONE', *, *, #26794, .F. ) ;
#28701=CARTESIAN_POINT ( 'NONE',  ( -24.87414375265050026, -14.81611830904748395, 59.43574407478276100 ) ) ;
#28702=CARTESIAN_POINT ( 'NONE',  ( -24.07500963186500798, -16.99236413854744399, 73.16870702396911952 ) ) ;
#28703=( BOUNDED_CURVE ( )  B_SPLINE_CURVE ( 3, ( #18748, #11368, #14779, #25901 ),
 .UNSPECIFIED., .F., .F. ) 
 B_SPLINE_CURVE_WITH_KNOTS ( ( 4, 4 ),
 ( 0.5000000000000000000, 0.9074455897393651771 ),
 .UNSPECIFIED. ) 
 CURVE ( )  GEOMETRIC_REPRESENTATION_ITEM ( )  RATIONAL_B_SPLINE_CURVE ( ( 0.9999999999999938938, 0.4567392136813211989, 0.3561768502900304334, 0.6983129098261150469 ) ) 
 REPRESENTATION_ITEM ( '' )  );
#28705=EDGE_CURVE ( 'NONE', #16629, #29740, #35762, .T. ) ;
#28706=EDGE_CURVE ( 'NONE', #10157, #3333, #7467, .T. ) ;
#28710=EDGE_CURVE ( 'NONE', #6805, #43621, #7758, .T. ) ;
#28711=FACE_OUTER_BOUND ( 'NONE', #48174, .T. ) ;
#28713=ORIENTED_EDGE ( 'NONE', *, *, #1013, .F. ) ;
#28714=( BOUNDED_SURFACE ( )  B_SPLINE_SURFACE ( 3, 1, ( 
 ( #4558, #19580 ),
 ( #29687, #44722 ),
 ( #3519, #22001 ),
 ( #33058, #36743 ),
 ( #48101, #14567 ),
 ( #25939, #14332 ),
 ( #29390, #44422 ) ),
 .UNSPECIFIED., .T., .F., .F. ) 
 B_SPLINE_SURFACE_WITH_KNOTS ( ( 4, 3, 4 ),
 ( 2, 2 ),
 ( 0.000000000000000000, 0.5000000000000000000, 1.000000000000000000 ),
 ( 0.000000000000000000, 1.000000000000000000 ),
 .UNSPECIFIED. ) 
 GEOMETRIC_REPRESENTATION_ITEM ( )  RATIONAL_B_SPLINE_SURFACE ( (
 ( 1.000000000000000000, 1.000000000000000000),
 ( 0.3333333333333335369, 0.3333333333333330373),
 ( 0.3333333333333335369, 0.3333333333333330373),
 ( 1.000000000000000000, 1.000000000000000000),
 ( 0.3333333333333333703, 0.3333333333333333703),
 ( 0.3333333333333333703, 0.3333333333333333703),
 ( 1.000000000000000000, 1.000000000000000000) ) ) 
 REPRESENTATION_ITEM ( '' )  SURFACE ( )  );
#28716=( BOUNDED_SURFACE ( )  B_SPLINE_SURFACE ( 3, 1, ( 
 ( #4802, #39501 ),
 ( #35308, #8984 ),
 ( #46159, #27442 ),
 ( #20785, #19826 ),
 ( #34824, #24007 ),
 ( #39009, #20561 ),
 ( #1584, #16593 ) ),
 .UNSPECIFIED., .T., .F., .F. ) 
 B_SPLINE_SURFACE_WITH_KNOTS ( ( 4, 3, 4 ),
 ( 2, 2 ),
 ( 0.000000000000000000, 0.5000000000000000000, 1.000000000000000000 ),
 ( 0.000000000000000000, 1.000000000000000000 ),
 .UNSPECIFIED. ) 
 GEOMETRIC_REPRESENTATION_ITEM ( )  RATIONAL_B_SPLINE_SURFACE ( (
 ( 1.000000000000000000, 1.000000000000000000),
 ( 0.3333333333333335369, 0.3333333333333330373),
 ( 0.3333333333333335369, 0.3333333333333330373),
 ( 1.000000000000000000, 1.000000000000000000),
 ( 0.3333333333333333703, 0.3333333333333333703),
 ( 0.3333333333333333703, 0.3333333333333333703),
 ( 1.000000000000000000, 1.000000000000000000) ) ) 
 REPRESENTATION_ITEM ( '' )  SURFACE ( )  );
#28722=CARTESIAN_POINT ( 'NONE',  ( -20.83700022493355775, -19.12221826660256951, 53.49899999999994549 ) ) ;
#28724=DIRECTION ( 'NONE',  ( 1.061592182633803142E-06, 3.103086874681752273E-06, -0.9999999999946220797 ) ) ;
#28725=ORIENTED_EDGE ( 'NONE', *, *, #5717, .F. ) ;
#28726=CARTESIAN_POINT ( 'NONE',  ( -20.68076794159699006, -21.00564031164944012, 58.94475149674252634 ) ) ;
#28727=CARTESIAN_POINT ( 'NONE',  ( -24.44689184067228638, -14.18710713894228093, 69.93803194250310185 ) ) ;
#28728=( BOUNDED_CURVE ( )  B_SPLINE_CURVE ( 3, ( #44663, #10923, #18790, #7244 ),
 .UNSPECIFIED., .F., .F. ) 
 B_SPLINE_CURVE_WITH_KNOTS ( ( 4, 4 ),
 ( 0.000000000000000000, 0.4074455897393655657 ),
 .UNSPECIFIED. ) 
 CURVE ( )  GEOMETRIC_REPRESENTATION_ITEM ( )  RATIONAL_B_SPLINE_CURVE ( ( 1.000000000000000000, 0.4567392136813335224, 0.3561768502900308775, 0.6983129098260920653 ) ) 
 REPRESENTATION_ITEM ( '' )  );
#28729=ORIENTED_EDGE ( 'NONE', *, *, #18725, .T. ) ;
#28732=CARTESIAN_POINT ( 'NONE',  ( -9.975073501874963000, -14.93475060744560245, 74.84132960708070925 ) ) ;
#28733=VERTEX_POINT ( 'NONE', #13032 ) ;
#28735=DIRECTION ( 'NONE',  ( -0.8083598999316398137, -0.5886886037477750966, -6.671815824719443556E-08 ) ) ;
#28738=CARTESIAN_POINT ( 'NONE',  ( -16.66933960180709917, -7.791706125978248743, 74.11585391104840426 ) ) ;
#28740=ORIENTED_EDGE ( 'NONE', *, *, #38303, .T. ) ;
#28741=CARTESIAN_POINT ( 'NONE',  ( -22.07364850117675914, -9.574309989343213090, 59.91098251635671801 ) ) ;
#28742=CARTESIAN_POINT ( 'NONE',  ( -11.09714801257800865, -11.68115280588511773, 64.30448977214732054 ) ) ;
#28744=ORIENTED_EDGE ( 'NONE', *, *, #31582, .T. ) ;
#28745=CARTESIAN_POINT ( 'NONE',  ( -11.19061673737954088, -18.88921303226083737, 64.84732837536805050 ) ) ;
#28746=CARTESIAN_POINT ( 'NONE',  ( -24.77723895724858494, -16.00713575449774595, 66.24820309305337673 ) ) ;
#28748=VERTEX_POINT ( 'NONE', #32945 ) ;
#28749=CARTESIAN_POINT ( 'NONE',  ( -20.46382095854371030, -21.17433842136345490, 58.94475249639827297 ) ) ;
#28750=CARTESIAN_POINT ( 'NONE',  ( -13.85276489020729507, -20.89200646248024995, 72.22607902822389292 ) ) ;
#28751=CARTESIAN_POINT ( 'NONE',  ( -10.02945380498330508, -15.71617353208280221, 61.23063189029311104 ) ) ;
#28752=B_SPLINE_CURVE_WITH_KNOTS ( 'NONE', 1,
 ( #17293, #48068 ),
 .UNSPECIFIED., .F., .F.,
 ( 2, 2 ),
 ( 0.000000000000000000, 1.000000000000000000 ),
 .UNSPECIFIED. ) ;
#28753=CARTESIAN_POINT ( 'NONE',  ( -13.11945872550529835, -9.225962324091906197, 67.67942785705487552 ) ) ;
#28754=DIRECTION ( 'NONE',  ( -1.590463988637600692E-07, 3.579926724016472968E-07, -0.9999999999999232836 ) ) ;
#28755=CARTESIAN_POINT ( 'NONE',  ( -14.80624636014071172, -8.317144122717282428, 60.61996281969079803 ) ) ;
#28756=CARTESIAN_POINT ( 'NONE',  ( -13.04354001453261525, -9.349206015805425096, 67.60616047355428293 ) ) ;
#28757=CARTESIAN_POINT ( 'NONE',  ( -14.77871938317573353, -21.77373431923335190, 61.73576822224330130 ) ) ;
#28759=ORIENTED_EDGE ( 'NONE', *, *, #9071, .F. ) ;
#28761=CARTESIAN_POINT ( 'NONE',  ( -13.38575581802539993, -9.030060914960570173, 60.72478133471773276 ) ) ;
#28762=CARTESIAN_POINT ( 'NONE',  ( -23.07453839662878181, -9.953611553617093932, 66.66369493676361913 ) ) ;
#28763=CARTESIAN_POINT ( 'NONE',  ( -16.01712585257974908, -7.950755256560901429, 67.21177652078760900 ) ) ;
#28768=EDGE_LOOP ( 'NONE', ( #37346, #25286, #22722, #11758, #47632 ) ) ;
#28771=CARTESIAN_POINT ( 'NONE',  ( -14.97035482569482312, -21.41873484682592377, 61.92128389535452015 ) ) ;
#28773=CARTESIAN_POINT ( 'NONE',  ( -16.45566506110110438, -21.79267588865899086, 62.04095995016087528 ) ) ;
#28774=CARTESIAN_POINT ( 'NONE',  ( -10.53876648713876740, -16.36073154998923229, 68.13334680848100788 ) ) ;
#28776=EDGE_CURVE ( 'NONE', #12811, #12076, #36635, .T. ) ;
#28779=CARTESIAN_POINT ( 'NONE',  ( -19.98473524480838748, -8.236797504970272854, 70.45920369457601851 ) ) ;
#28781=DIRECTION ( 'NONE',  ( 7.110378527815250859E-06, 9.728165319648377852E-06, -0.9999999999274026274 ) ) ;
#28782=EDGE_LOOP ( 'NONE', ( #14664, #27475 ) ) ;
#28783=CARTESIAN_POINT ( 'NONE',  ( -20.98579777188748707, -20.83533835786949950, 65.58453944793343737 ) ) ;
#28784=EDGE_LOOP ( 'NONE', ( #35657, #40264 ) ) ;
#28786=CARTESIAN_POINT ( 'NONE',  ( -19.23357275453091830, -7.582241477678771879, 63.62427554819404207 ) ) ;
#28787=EDGE_LOOP ( 'NONE', ( #41181, #9452, #43438, #28280, #47765 ) ) ;
#28788=CARTESIAN_POINT ( 'NONE',  ( -18.46282339125754746, -21.73182043318683299, 72.58510983671801853 ) ) ;
#28791=ORIENTED_EDGE ( 'NONE', *, *, #4562, .T. ) ;
#28794=CARTESIAN_POINT ( 'NONE',  ( -21.62392673332162119, -8.655692864502302797, 73.77941542331133462 ) ) ;
#28795=ORIENTED_EDGE ( 'NONE', *, *, #40561, .F. ) ;
#28796=CARTESIAN_POINT ( 'NONE',  ( -13.34712228287558844, -20.56097989973784834, 58.05209898279497338 ) ) ;
#28799=AXIS2_PLACEMENT_3D ( 'NONE', #44287, #47489, #6839 ) ;
#28800=B_SPLINE_CURVE_WITH_KNOTS ( 'NONE', 3,
 ( #12039, #27055, #42079, #27539, #19418, #4178, #26825, #15461, #12274, #31235 ),
 .UNSPECIFIED., .F., .F.,
 ( 4, 2, 2, 2, 4 ),
 ( 0.6272669072783476629, 0.7522669073002239415, 0.8772669073221003311, 1.002266907343976721, 1.127266907365852999 ),
 .UNSPECIFIED. ) ;
#28801=DIRECTION ( 'NONE',  ( -0.1571515419521612722, 0.9875744999047173511, -7.433889655140016607E-08 ) ) ;
#28802=FACE_OUTER_BOUND ( 'NONE', #47519, .T. ) ;
#28803=ORIENTED_EDGE ( 'NONE', *, *, #46637, .T. ) ;
#28805=CARTESIAN_POINT ( 'NONE',  ( -11.76184414918852106, -18.92500367160094044, 68.44362863376011319 ) ) ;
#28806=CARTESIAN_POINT ( 'NONE',  ( -10.97862690519434459, -18.54530816898288492, 57.95714592071885107 ) ) ;
#28808=CARTESIAN_POINT ( 'NONE',  ( -20.71686288416324118, -8.126370072314889725, 63.51110291890488213 ) ) ;
#28809=( BOUNDED_CURVE ( )  B_SPLINE_CURVE ( 3, ( #8142, #8624, #27803, #23886 ),
 .UNSPECIFIED., .F., .F. ) 
 B_SPLINE_CURVE_WITH_KNOTS ( ( 4, 4 ),
 ( 0.4074455897393700621, 0.5000000000000000000 ),
 .UNSPECIFIED. ) 
 CURVE ( )  GEOMETRIC_REPRESENTATION_ITEM ( )  RATIONAL_B_SPLINE_CURVE ( ( 0.6983129098261103840, 0.7760317562607019770, 0.8765941196519950740, 0.9999999999999821254 ) ) 
 REPRESENTATION_ITEM ( '' )  );
#28811=CARTESIAN_POINT ( 'NONE',  ( -24.15165104652898620, -11.60707627830156952, 63.13873557927141889 ) ) ;
#28813=CARTESIAN_POINT ( 'NONE',  ( -23.70015292207183322, -18.82353835121273988, 69.47867366044893345 ) ) ;
#28814=ORIENTED_EDGE ( 'NONE', *, *, #2508, .F. ) ;
#28818=ORIENTED_EDGE ( 'NONE', *, *, #13541, .F. ) ;
#28819=ORIENTED_EDGE ( 'NONE', *, *, #2373, .F. ) ;
#28820=EDGE_CURVE ( 'NONE', #6217, #37990, #7337, .T. ) ;
#28821=CARTESIAN_POINT ( 'NONE',  ( -10.86332161679245445, -12.36740429957887955, 57.61240734327432733 ) ) ;
#28824=VERTEX_POINT ( 'NONE', #22143 ) ;
#28825=DIRECTION ( 'NONE',  ( -0.9789991564298998750, -0.2038642972899922245, 4.410747590293501250E-08 ) ) ;
#28828=ORIENTED_EDGE ( 'NONE', *, *, #41668, .T. ) ;
#28829=EDGE_CURVE ( 'NONE', #27130, #383, #44923, .T. ) ;
#28830=CARTESIAN_POINT ( 'NONE',  ( -20.72450927900464634, -21.03929139025762751, 58.93003081252663833 ) ) ;
#28832=EDGE_CURVE ( 'NONE', #260, #15899, #9073, .T. ) ;
#28833=DIRECTION ( 'NONE',  ( -2.209513405570979834E-06, 7.769005115158032304E-07, 0.9999999999972571940 ) ) ;
#28834=ORIENTED_EDGE ( 'NONE', *, *, #11587, .T. ) ;
#28835=CARTESIAN_POINT ( 'NONE',  ( -24.15708772167537077, -12.88964773349922410, 69.84413305346230061 ) ) ;
#28837=B_SPLINE_CURVE_WITH_KNOTS ( 'NONE', 3,
 ( #34623, #24287, #909, #8534, #39536, #39294, #23564, #35589, #13166, #42519 ),
 .UNSPECIFIED., .F., .F.,
 ( 4, 2, 2, 2, 4 ),
 ( 0.1272669073658421190, 0.2522669073463229550, 0.3772669073268037909, 0.5022669073072846269, 0.6272669072877654628 ),
 .UNSPECIFIED. ) ;
#28838=CARTESIAN_POINT ( 'NONE',  ( -26.22630854578367021, -13.51651355179587632, 53.49999999999995026 ) ) ;
#28839=CARTESIAN_POINT ( 'NONE',  ( -22.29619887594318328, -17.36118473213641167, 54.07175714974878389 ) ) ;
#28840=CARTESIAN_POINT ( 'NONE',  ( -19.22579309969192707, -21.57336792462666253, 58.52507384993226225 ) ) ;
#28842=CARTESIAN_POINT ( 'NONE',  ( -21.19385221619855386, -22.41842420181545847, 54.38277594638586976 ) ) ;
#28843=CARTESIAN_POINT ( 'NONE',  ( -10.57136597998982985, -13.11950654315977793, 64.42403173677416817 ) ) ;
#28844=CARTESIAN_POINT ( 'NONE',  ( -17.72634082312590920, -21.85272461445201486, 58.40553378267872375 ) ) ;
#28845=( BOUNDED_SURFACE ( )  B_SPLINE_SURFACE ( 3, 1, ( 
 ( #26146, #18997 ),
 ( #21713, #22446 ),
 ( #37437, #33752 ),
 ( #40424, #34001 ),
 ( #15276, #15032 ),
 ( #25895, #14296 ),
 ( #30094, #45117 ) ),
 .UNSPECIFIED., .T., .F., .F. ) 
 B_SPLINE_SURFACE_WITH_KNOTS ( ( 4, 3, 4 ),
 ( 2, 2 ),
 ( 0.000000000000000000, 0.5000000000000000000, 1.000000000000000000 ),
 ( 0.000000000000000000, 1.000000000000000000 ),
 .UNSPECIFIED. ) 
 GEOMETRIC_REPRESENTATION_ITEM ( )  RATIONAL_B_SPLINE_SURFACE ( (
 ( 1.000000000000000000, 1.000000000000000000),
 ( 0.3333333333333335369, 0.3333333333333330373),
 ( 0.3333333333333335369, 0.3333333333333330373),
 ( 1.000000000000000000, 1.000000000000000000),
 ( 0.3333333333333333703, 0.3333333333333333703),
 ( 0.3333333333333333703, 0.3333333333333333703),
 ( 1.000000000000000000, 1.000000000000000000) ) ) 
 REPRESENTATION_ITEM ( '' )  SURFACE ( )  );
#28846=CARTESIAN_POINT ( 'NONE',  ( -15.47121567594983738, -8.035039782910647688, 74.37985637822782792 ) ) ;
#28847=CARTESIAN_POINT ( 'NONE',  ( -10.45529275995371066, -15.48619407273052495, 61.22716148030291805 ) ) ;
#28848=CARTESIAN_POINT ( 'NONE',  ( -23.00381842360518547, -10.58230771189866104, 59.90203429537245228 ) ) ;
#28850=CARTESIAN_POINT ( 'NONE',  ( -23.49605051889219709, -11.22618518380361152, 73.37665428612797314 ) ) ;
#28851=CARTESIAN_POINT ( 'NONE',  ( -12.23165125622869631, -10.02867215863997608, 67.64329750964374455 ) ) ;
#28854=CARTESIAN_POINT ( 'NONE',  ( -11.46043946983621709, -11.04924301243271678, 57.35903212150709152 ) ) ;
#28856=ORIENTED_EDGE ( 'NONE', *, *, #42286, .F. ) ;
#28857=ORIENTED_EDGE ( 'NONE', *, *, #30849, .T. ) ;
#28858=CARTESIAN_POINT ( 'NONE',  ( -21.18836735823073525, -20.77369112572868914, 65.46965119999302374 ) ) ;
#28859=CARTESIAN_POINT ( 'NONE',  ( -24.39416267077224987, -15.91966209353573802, 73.14736799148198543 ) ) ;
#28860=ORIENTED_EDGE ( 'NONE', *, *, #34986, .F. ) ;
#28861=CARTESIAN_POINT ( 'NONE',  ( -9.975583786612773451, -14.65598763567812313, 71.44287367974872893 ) ) ;
#28862=CARTESIAN_POINT ( 'NONE',  ( -10.62433447910814976, -13.14689714368311257, 67.92935478332734078 ) ) ;
#28863=CARTESIAN_POINT ( 'NONE',  ( -12.50766613833179974, -19.86205114983803810, 64.86674886870797252 ) ) ;
#28864=CARTESIAN_POINT ( 'NONE',  ( -14.48970220490235228, -8.453945278547838171, 63.98082128453373940 ) ) ;
#28865=CARTESIAN_POINT ( 'NONE',  ( -10.61357223164714902, -13.19155561173493219, 71.20828586568362084 ) ) ;
#28866=CARTESIAN_POINT ( 'NONE',  ( -22.22492895683646807, -9.112220634607178127, 59.76525293062090327 ) ) ;
#28867=CARTESIAN_POINT ( 'NONE',  ( -11.45752044641470668, -19.27057170535650954, 71.87181270239314301 ) ) ;
#28870=( BOUNDED_CURVE ( )  B_SPLINE_CURVE ( 3, ( #27260, #20360, #2364, #47433 ),
 .UNSPECIFIED., .F., .F. ) 
 B_SPLINE_CURVE_WITH_KNOTS ( ( 4, 4 ),
 ( 0.4074455897393655657, 0.5000000000000000000 ),
 .UNSPECIFIED. ) 
 CURVE ( )  GEOMETRIC_REPRESENTATION_ITEM ( )  RATIONAL_B_SPLINE_CURVE ( ( 0.6983129098260923984, 0.7760317562606950936, 0.8765941196519969614, 0.9999999999999960032 ) ) 
 REPRESENTATION_ITEM ( '' )  );
#28871=VECTOR ( 'NONE', #12106, 1000.000000000000000 ) ;
#28874=VERTEX_POINT ( 'NONE', #10568 ) ;
#28875=CARTESIAN_POINT ( 'NONE',  ( -20.75354924259569245, -21.52967727414722532, 53.49999999999994316 ) ) ;
#28876=CARTESIAN_POINT ( 'NONE',  ( -11.54877110944083896, -18.61454263387444286, 61.38596758451725321 ) ) ;
#28877=AXIS2_PLACEMENT_3D ( 'NONE', #39443, #2724, #28833 ) ;
#28879=CARTESIAN_POINT ( 'NONE',  ( -24.63461978062257174, -12.93251252767717929, 66.48902111634848211 ) ) ;
#28880=ADVANCED_FACE ( 'NONE', ( #3171 ), #25579, .T. ) ;
#28881=CARTESIAN_POINT ( 'NONE',  ( -13.85547199604887503, -20.83131545695484732, 65.21302117645285534 ) ) ;
#28882=CARTESIAN_POINT ( 'NONE',  ( -19.30271930833434979, -8.014115225907463724, 60.11092997145157568 ) ) ;
#28883=ORIENTED_EDGE ( 'NONE', *, *, #19866, .T. ) ;
#28887=CARTESIAN_POINT ( 'NONE',  ( -11.97490362423377164, -10.33561459433851404, 67.78424783647008667 ) ) ;
#28888=B_SPLINE_CURVE_WITH_KNOTS ( 'NONE', 3,
 ( #33132, #17143, #3109, #24578, #47459, #2142, #43528, #48171, #25293, #10022 ),
 .UNSPECIFIED., .F., .F.,
 ( 4, 2, 2, 2, 4 ),
 ( 0.1272669073658118100, 0.2522669073462989742, 0.3772669073267861939, 0.5022669073072734136, 0.6272669072877605778 ),
 .UNSPECIFIED. ) ;
#28889=CARTESIAN_POINT ( 'NONE',  ( -15.41078985079695940, -7.636351814344855882, 74.27323974507916660 ) ) ;
#28890=EDGE_LOOP ( 'NONE', ( #12229, #33904, #40998, #33673, #8695, #2024, #41089, #1964, #47627, #47779, #44555, #9032, #42606, #45746, #27641, #37167, #7877, #17841, #22418, #11893, #35319, #12329, #3156, #4123, #9557, #15411, #3668, #13524, #22748, #10958, #29325, #2098, #35936 ) ) ;
#28892=CARTESIAN_POINT ( 'NONE',  ( -19.30031737610338993, -22.01920738531545396, 58.70320165633192033 ) ) ;
#28893=LINE ( 'NONE', #48096, #46935 ) ;
#28894=ADVANCED_FACE ( 'NONE', ( #44546 ), #10801, .T. ) ;
#28895=ORIENTED_EDGE ( 'NONE', *, *, #30139, .T. ) ;
#28897=CARTESIAN_POINT ( 'NONE',  ( -14.84927081153347039, -21.37251255130113137, 61.65072491673618771 ) ) ;
#28898=AXIS2_PLACEMENT_3D ( 'NONE', #17892, #40555, #36373 ) ;
#28901=CARTESIAN_POINT ( 'NONE',  ( -23.75972628784533569, -10.79550978475970346, 47.99999999999994316 ) ) ;
#28902=CARTESIAN_POINT ( 'NONE',  ( -19.04042241193164386, -7.536568769452434147, 67.01576393362593365 ) ) ;
#28905=CARTESIAN_POINT ( 'NONE',  ( -20.14548719510382924, -7.874031717564547783, 73.92085388793562117 ) ) ;
#28906=CARTESIAN_POINT ( 'NONE',  ( -24.82750207115152463, -13.97654542584719373, 73.30766806548945169 ) ) ;
#28908=EDGE_CURVE ( 'NONE', #19604, #32745, #17692, .T. ) ;
#28909=LINE ( 'NONE', #36516, #39985 ) ;
#28910=CARTESIAN_POINT ( 'NONE',  ( -22.27985548098255109, -20.46033401586769429, 58.87787560672637710 ) ) ;
#28912=CARTESIAN_POINT ( 'NONE',  ( -22.43638724005049667, -20.32197157274265820, 62.34783858214098728 ) ) ;
#28913=AXIS2_PLACEMENT_3D ( 'NONE', #3048, #18061, #33072 ) ;
#28914=CARTESIAN_POINT ( 'NONE',  ( -11.35825037048775066, -11.21643016533577075, 60.67885780704620657 ) ) ;
#28915=CARTESIAN_POINT ( 'NONE',  ( -15.49416032233947504, -8.028509233753512220, 74.07985659018983426 ) ) ;
#28916=CARTESIAN_POINT ( 'NONE',  ( -17.11594671439511828, -7.315539529225058679, 54.27966884056655061 ) ) ;
#28918=CARTESIAN_POINT ( 'NONE',  ( -16.78341102624552050, -22.23169286577646986, 68.88055947109249644 ) ) ;
#28919=CARTESIAN_POINT ( 'NONE',  ( -24.30112618867181240, -13.25578303422174997, 59.64795780745660636 ) ) ;
#28920=ORIENTED_EDGE ( 'NONE', *, *, #6952, .F. ) ;
#28921=CARTESIAN_POINT ( 'NONE',  ( -10.67753361921853461, -12.94244927161164505, 64.49509439877509465 ) ) ;
#28923=DIRECTION ( 'NONE',  ( -5.731567514496413899E-31, -1.020425574103664789E-16, -1.000000000000000000 ) ) ;
#28925=CARTESIAN_POINT ( 'NONE',  ( -17.00410685006708178, -7.771727545396207582, 73.96018273221115180 ) ) ;
#28926=ORIENTED_EDGE ( 'NONE', *, *, #24588, .T. ) ;
#28927=VERTEX_POINT ( 'NONE', #30022 ) ;
#28928=ORIENTED_EDGE ( 'NONE', *, *, #46385, .T. ) ;
#28929=CARTESIAN_POINT ( 'NONE',  ( -14.04312670088115134, -20.93869291823072132, 72.22607738042698600 ) ) ;
#28932=EDGE_CURVE ( 'NONE', #2764, #21586, #3835, .T. ) ;
#28934=CARTESIAN_POINT ( 'NONE',  ( -12.68532353738824803, -9.060482037740600347, 71.03420644255490402 ) ) ;
#28935=AXIS2_PLACEMENT_3D ( 'NONE', #38048, #38786, #31653 ) ;
#28937=ORIENTED_EDGE ( 'NONE', *, *, #11817, .F. ) ;
#28941=AXIS2_PLACEMENT_3D ( 'NONE', #21951, #44374, #6933 ) ;
#28942=CARTESIAN_POINT ( 'NONE',  ( -11.34764044004908534, -18.38430194568898912, 58.10154788514100943 ) ) ;
#28944=ADVANCED_FACE ( 'NONE', ( #45289 ), #30518, .T. ) ;
#28946=ORIENTED_EDGE ( 'NONE', *, *, #19430, .F. ) ;
#28947=CARTESIAN_POINT ( 'NONE',  ( -23.92465930214516234, -12.07130710318904221, 59.57415707955740203 ) ) ;
#28948=CARTESIAN_POINT ( 'NONE',  ( -24.36028583763659583, -16.11466138999042030, 69.67740616536292464 ) ) ;
#28949=ORIENTED_EDGE ( 'NONE', *, *, #42408, .F. ) ;
#28950=CARTESIAN_POINT ( 'NONE',  ( -17.04413539470110095, -21.84925844046378174, 72.45071136019464575 ) ) ;
#28953=CARTESIAN_POINT ( 'NONE',  ( -14.63112947634313521, -8.332108846598762497, 67.35155072858903225 ) ) ;
#28954=CARTESIAN_POINT ( 'NONE',  ( -11.02440266205174524, -11.97271778485252192, 74.55840233405203321 ) ) ;
#28955=CARTESIAN_POINT ( 'NONE',  ( -13.57213406898786978, -20.71828813759911014, 58.04649799015020761 ) ) ;
#28956=ORIENTED_EDGE ( 'NONE', *, *, #6881, .F. ) ;
#28958=CARTESIAN_POINT ( 'NONE',  ( -19.24025795797341942, -7.996846695050864540, 60.24620885950562865 ) ) ;
#28959=EDGE_CURVE ( 'NONE', #17956, #32730, #39518, .T. ) ;
#28960=VECTOR ( 'NONE', #40431, 1000.000000000000000 ) ;
#28961=CARTESIAN_POINT ( 'NONE',  ( -23.17061082369141900, -10.06671700699632233, 66.72837583070179335 ) ) ;
#28962=CARTESIAN_POINT ( 'NONE',  ( -23.40706900507760224, -18.44293855997280929, 73.06368236814604700 ) ) ;
#28964=CARTESIAN_POINT ( 'NONE',  ( -21.52726120556258849, -9.076273861542912158, 70.28132538914752558 ) ) ;
#28965=AXIS2_PLACEMENT_3D ( 'NONE', #23069, #48415, #11001 ) ;
#28967=CARTESIAN_POINT ( 'NONE',  ( -14.90123591195245112, -21.39555782113924209, 65.52085318447059592 ) ) ;
#28968=B_SPLINE_CURVE_WITH_KNOTS ( 'NONE', 3,
 ( #2318, #24508, #39508, #17566, #32373, #5787, #35560, #39014, #39993, #20794 ),
 .UNSPECIFIED., .F., .F.,
 ( 4, 2, 2, 2, 4 ),
 ( 0.000000000000000000, 0.2500000000000000000, 0.5000000000000000000, 0.7500000000000000000, 1.000000000000000000 ),
 .UNSPECIFIED. ) ;
#28969=ORIENTED_EDGE ( 'NONE', *, *, #43874, .F. ) ;
#28971=CARTESIAN_POINT ( 'NONE',  ( -13.65110163016468015, -21.23324793748626504, 68.57129851394472553 ) ) ;
#28972=CARTESIAN_POINT ( 'NONE',  ( -10.39241571269986331, -17.41794234916963191, 53.49999999999994316 ) ) ;
#28973=CARTESIAN_POINT ( 'NONE',  ( -22.63008543824757979, -10.12971389395683097, 70.01178520543939499 ) ) ;
#28974=ORIENTED_EDGE ( 'NONE', *, *, #10263, .F. ) ;
#28975=CARTESIAN_POINT ( 'NONE',  ( -10.37497030826117417, -14.69804335084345759, 71.32782692816427073 ) ) ;
#28977=CARTESIAN_POINT ( 'NONE',  ( -23.80338573481879294, -11.80731802715296119, 59.76763678108634537 ) ) ;
#28978=CARTESIAN_POINT ( 'NONE',  ( -23.34421923326152992, -18.54457442964731584, 69.57906566121042147 ) ) ;
#28979=EDGE_CURVE ( 'NONE', #6635, #24347, #29160, .T. ) ;
#28982=EDGE_CURVE ( 'NONE', #34596, #37312, #33425, .T. ) ;
#28983=CARTESIAN_POINT ( 'NONE',  ( -10.98557804775572144, -17.68114217416224321, 71.71718193507115302 ) ) ;
#28985=EDGE_CURVE ( 'NONE', #26173, #38482, #33096, .T. ) ;
#28987=ORIENTED_EDGE ( 'NONE', *, *, #32860, .T. ) ;
#28988=CARTESIAN_POINT ( 'NONE',  ( -13.85546777306732480, -20.89347761745142407, 72.01787893532731744 ) ) ;
#28989=CARTESIAN_POINT ( 'NONE',  ( -10.02101610845663870, -15.64516224647144149, 61.16072161825523068 ) ) ;
#28990=CARTESIAN_POINT ( 'NONE',  ( -24.18470913683765389, -12.80901137141652768, 69.78715111652664405 ) ) ;
#28991=CARTESIAN_POINT ( 'NONE',  ( -12.74836358285320159, -20.08597126951521261, 71.82125749157572159 ) ) ;
#28992=( BOUNDED_CURVE ( )  B_SPLINE_CURVE ( 3, ( #17662, #39841, #21136, #10298 ),
 .UNSPECIFIED., .F., .F. ) 
 B_SPLINE_CURVE_WITH_KNOTS ( ( 4, 4 ),
 ( 0.000000000000000000, 0.4074455897393665649 ),
 .UNSPECIFIED. ) 
 CURVE ( )  GEOMETRIC_REPRESENTATION_ITEM ( )  RATIONAL_B_SPLINE_CURVE ( ( 1.000000000000000000, 0.4567392136813214210, 0.3561768502900264366, 0.6983129098261150469 ) ) 
 REPRESENTATION_ITEM ( '' )  );
#28994=CARTESIAN_POINT ( 'NONE',  ( -12.35277413765887999, -20.26681541663451114, 68.45162113748973809 ) ) ;
#28995=CARTESIAN_POINT ( 'NONE',  ( -22.74914502862361587, -19.44157078561079999, 72.79967855327656423 ) ) ;
#28997=ORIENTED_EDGE ( 'NONE', *, *, #28603, .F. ) ;
#28998=FACE_OUTER_BOUND ( 'NONE', #18294, .T. ) ;
#28999=PLANE ( 'NONE',  #24416 ) ;
#29001=CARTESIAN_POINT ( 'NONE',  ( -14.97035482569482312, -21.41873484682592377, 61.92128389535452015 ) ) ;
#29002=CARTESIAN_POINT ( 'NONE',  ( -10.38181936765313473, -14.47839093401252875, 67.85800130414834541 ) ) ;
#29006=( BOUNDED_SURFACE ( )  B_SPLINE_SURFACE ( 3, 1, ( 
 ( #19130, #33901 ),
 ( #22098, #30230 ),
 ( #3373, #4131 ),
 ( #25785, #45491 ),
 ( #194, #40799 ),
 ( #3621, #18381 ),
 ( #18622, #48676 ) ),
 .UNSPECIFIED., .T., .F., .F. ) 
 B_SPLINE_SURFACE_WITH_KNOTS ( ( 4, 3, 4 ),
 ( 2, 2 ),
 ( 0.000000000000000000, 0.5000000000000000000, 1.000000000000000000 ),
 ( 0.000000000000000000, 1.000000000000000000 ),
 .UNSPECIFIED. ) 
 GEOMETRIC_REPRESENTATION_ITEM ( )  RATIONAL_B_SPLINE_SURFACE ( (
 ( 1.000000000000000000, 1.000000000000000000),
 ( 0.3333333333333335369, 0.3333333333333330373),
 ( 0.3333333333333335369, 0.3333333333333330373),
 ( 1.000000000000000000, 1.000000000000000000),
 ( 0.3333333333333333703, 0.3333333333333333703),
 ( 0.3333333333333333703, 0.3333333333333333703),
 ( 1.000000000000000000, 1.000000000000000000) ) ) 
 REPRESENTATION_ITEM ( '' )  SURFACE ( )  );
#29008=ORIENTED_EDGE ( 'NONE', *, *, #15308, .T. ) ;
#29010=DIRECTION ( 'NONE',  ( -2.515467001362780054E-08, -7.569581535656660169E-10, 0.9999999999999996669 ) ) ;
#29012=CARTESIAN_POINT ( 'NONE',  ( -19.30128557755455532, -21.60500301973953086, 58.81035253397666196 ) ) ;
#29013=VERTEX_POINT ( 'NONE', #38348 ) ;
#29014=( BOUNDED_SURFACE ( )  B_SPLINE_SURFACE ( 3, 1, ( 
 ( #36451, #35973 ),
 ( #2729, #17737 ),
 ( #32766, #33981 ),
 ( #25874, #25623 ),
 ( #30321, #278 ),
 ( #18469, #41137 ),
 ( #33230, #22673 ) ),
 .UNSPECIFIED., .T., .F., .F. ) 
 B_SPLINE_SURFACE_WITH_KNOTS ( ( 4, 3, 4 ),
 ( 2, 2 ),
 ( 0.000000000000000000, 0.5000000000000000000, 1.000000000000000000 ),
 ( 0.000000000000000000, 1.000000000000000000 ),
 .UNSPECIFIED. ) 
 GEOMETRIC_REPRESENTATION_ITEM ( )  RATIONAL_B_SPLINE_SURFACE ( (
 ( 1.000000000000000000, 1.000000000000000000),
 ( 0.3333333333333335369, 0.3333333333333330373),
 ( 0.3333333333333335369, 0.3333333333333330373),
 ( 1.000000000000000000, 1.000000000000000000),
 ( 0.3333333333333333703, 0.3333333333333333703),
 ( 0.3333333333333333703, 0.3333333333333333703),
 ( 1.000000000000000000, 1.000000000000000000) ) ) 
 REPRESENTATION_ITEM ( '' )  SURFACE ( )  );
#29015=ADVANCED_FACE ( 'NONE', ( #34175 ), #23353, .T. ) ;
#29016=CARTESIAN_POINT ( 'NONE',  ( -13.53844544295976249, -20.69534049476535031, 65.40117765236396963 ) ) ;
#29019=B_SPLINE_CURVE_WITH_KNOTS ( 'NONE', 3,
 ( #42493, #4566, #30687, #19588, #34597, #12436, #46428, #881, #12683, #24025 ),
 .UNSPECIFIED., .F., .F.,
 ( 4, 2, 2, 2, 4 ),
 ( 0.6272669072877820051, 0.7522669073072913992, 0.8772669073268006823, 1.002266907346310187, 1.127266907365819470 ),
 .UNSPECIFIED. ) ;
#29020=CARTESIAN_POINT ( 'NONE',  ( -16.13263948075386978, -7.878200451182638453, 63.68483172840383588 ) ) ;
#29021=VERTEX_POINT ( 'NONE', #18419 ) ;
#29022=CARTESIAN_POINT ( 'NONE',  ( -19.08517061958907490, -7.953970113302217371, 60.16912824253490299 ) ) ;
#29023=ORIENTED_EDGE ( 'NONE', *, *, #31906, .F. ) ;
#29024=CARTESIAN_POINT ( 'NONE',  ( -24.87269970749685299, -14.66254690463778942, 62.90634777101153219 ) ) ;
#29025=ORIENTED_EDGE ( 'NONE', *, *, #37152, .T. ) ;
#29028=AXIS2_PLACEMENT_3D ( 'NONE', #2753, #20997, #1801 ) ;
#29029=ORIENTED_EDGE ( 'NONE', *, *, #46433, .F. ) ;
#29031=AXIS2_PLACEMENT_3D ( 'NONE', #29301, #44568, #33698 ) ;
#29033=CARTESIAN_POINT ( 'NONE',  ( -21.55883939963115026, -8.611815437115641458, 73.78624134823098757 ) ) ;
#29037=AXIS2_PLACEMENT_3D ( 'NONE', #16791, #28133, #43158 ) ;
#29038=ADVANCED_FACE ( 'NONE', ( #11301 ), #48465, .F. ) ;
#29039=CARTESIAN_POINT ( 'NONE',  ( -17.15293984484763712, -7.364064364366409876, 70.53389935397558475 ) ) ;
#29040=CARTESIAN_POINT ( 'NONE',  ( -24.05420634179087358, -17.20676946999824608, 69.69867738674849988 ) ) ;
#29041=CARTESIAN_POINT ( 'NONE',  ( -23.42631727757699878, -10.39480074052133141, 59.78858809748042091 ) ) ;
#29043=EDGE_CURVE ( 'NONE', #22189, #21219, #12472, .T. ) ;
#29044=ORIENTED_EDGE ( 'NONE', *, *, #13609, .F. ) ;
#29045=ORIENTED_EDGE ( 'NONE', *, *, #5745, .T. ) ;
#29046=CARTESIAN_POINT ( 'NONE',  ( -21.23484681875272884, -20.74088929683185611, 69.33978048267414351 ) ) ;
#29047=ORIENTED_EDGE ( 'NONE', *, *, #19226, .F. ) ;
#29048=CARTESIAN_POINT ( 'NONE',  ( -20.69509153224808173, -8.115601224564374050, 63.49616927690831858 ) ) ;
#29049=VECTOR ( 'NONE', #29781, 1000.000000000000000 ) ;
#29051=CARTESIAN_POINT ( 'NONE',  ( -23.71751471349159601, -11.63122711669449316, 63.23746208799618529 ) ) ;
#29052=CARTESIAN_POINT ( 'NONE',  ( -14.34827028450108344, -21.16170790896200060, 72.08174668229233362 ) ) ;
#29053=CARTESIAN_POINT ( 'NONE',  ( -20.54969731993802995, -8.046573202280342230, 66.98115280391161264 ) ) ;
#29055=ORIENTED_EDGE ( 'NONE', *, *, #40762, .F. ) ;
#29056=ADVANCED_FACE ( 'NONE', ( #27285 ), #10897, .T. ) ;
#29061=ORIENTED_EDGE ( 'NONE', *, *, #38238, .T. ) ;
#29062=B_SPLINE_CURVE_WITH_KNOTS ( 'NONE', 1,
 ( #39068, #34157 ),
 .UNSPECIFIED., .F., .F.,
 ( 2, 2 ),
 ( 0.000000000000000000, 1.000000000000000000 ),
 .UNSPECIFIED. ) ;
#29063=ADVANCED_FACE ( 'NONE', ( #31708 ), #16432, .T. ) ;
#29064=CARTESIAN_POINT ( 'NONE',  ( -17.66159697976433307, -21.85550285805611637, 58.42025434932890704 ) ) ;
#29065=CARTESIAN_POINT ( 'NONE',  ( -23.66688185712976633, -11.64243612726180643, 62.96720739904996833 ) ) ;
#29067=CARTESIAN_POINT ( 'NONE',  ( -23.91639008814848211, -11.15506099060319123, 69.99236505904349315 ) ) ;
#29069=ORIENTED_EDGE ( 'NONE', *, *, #21141, .T. ) ;
#29071=LINE ( 'NONE', #44350, #19558 ) ;
#29072=CARTESIAN_POINT ( 'NONE',  ( -11.40126873537406205, -11.24191379345135999, 60.97885781058090515 ) ) ;
#29073=ADVANCED_FACE ( 'NONE', ( #1669 ), #9558, .T. ) ;
#29074=EDGE_LOOP ( 'NONE', ( #39200, #13013, #33381, #37374, #14503 ) ) ;
#29076=CARTESIAN_POINT ( 'NONE',  ( -17.78490012859682423, -21.80118270052165741, 62.10365751430077808 ) ) ;
#29077=FACE_OUTER_BOUND ( 'NONE', #39633, .T. ) ;
#29078=ORIENTED_EDGE ( 'NONE', *, *, #8427, .T. ) ;
#29079=CARTESIAN_POINT ( 'NONE',  ( -11.97490362423377164, -10.33561459433851404, 67.78424783647008667 ) ) ;
#29080=VERTEX_POINT ( 'NONE', #16674 ) ;
#29081=CARTESIAN_POINT ( 'NONE',  ( -24.31823774515246939, -17.63313259158020685, 66.05861911469568781 ) ) ;
#29082=CARTESIAN_POINT ( 'NONE',  ( -13.52830415862076308, -20.68508020484520671, 61.51646354542308615 ) ) ;
#29083=FACE_BOUND ( 'NONE', #24569, .T. ) ;
#29085=CARTESIAN_POINT ( 'NONE',  ( -21.40357752720559503, -21.10733023442637446, 69.15426546848676992 ) ) ;
#29086=CARTESIAN_POINT ( 'NONE',  ( -10.72572792941078212, -12.60087465324735945, 64.68324854050578665 ) ) ;
#29088=CARTESIAN_POINT ( 'NONE',  ( -10.80019681701181966, -17.07282933688417970, 57.79646546703656895 ) ) ;
#29089=DIRECTION ( 'NONE',  ( 0.05957303659011964347, 0.9982239494779874267, -2.515684304544914870E-08 ) ) ;
#29090=DIRECTION ( 'NONE',  ( -5.408674110437222193E-06, 4.460197095916123975E-06, 0.9999999999754265456 ) ) ;
#29092=CARTESIAN_POINT ( 'NONE',  ( -24.87143190479848798, -14.60822328784750646, 62.81958198222076106 ) ) ;
#29093=CARTESIAN_POINT ( 'NONE',  ( -20.50783493979771421, -8.027295371342848540, 66.96599508560271374 ) ) ;
#29096=CARTESIAN_POINT ( 'NONE',  ( -24.27033112822875438, -13.12649005559073423, 63.13264177271825872 ) ) ;
#29098=ORIENTED_EDGE ( 'NONE', *, *, #29192, .T. ) ;
#29099=ORIENTED_EDGE ( 'NONE', *, *, #2359, .T. ) ;
#29100=AXIS2_PLACEMENT_3D ( 'NONE', #2194, #3160, #29506 ) ;
#29101=CARTESIAN_POINT ( 'NONE',  ( -22.70900583301066433, -10.21894050583236968, 66.55684684265230544 ) ) ;
#29103=ORIENTED_EDGE ( 'NONE', *, *, #38698, .T. ) ;
#29104=CARTESIAN_POINT ( 'NONE',  ( -19.28288283825861527, -21.60990478829091899, 58.81947569273916088 ) ) ;
#29105=CARTESIAN_POINT ( 'NONE',  ( -11.40127056704611519, -11.24191079892443135, 60.67885781060143557 ) ) ;
#29106=CARTESIAN_POINT ( 'NONE',  ( -13.41953676616927460, -9.006914687363744676, 60.73950246439220280 ) ) ;
#29108=CARTESIAN_POINT ( 'NONE',  ( -19.50103315386265024, -8.068942516160735323, 60.37581784757137626 ) ) ;
#29110=CARTESIAN_POINT ( 'NONE',  ( -24.74044779172452024, -16.21442189768792375, 62.63682720862403386 ) ) ;
#29113=CARTESIAN_POINT ( 'NONE',  ( -10.42278038625809700, -14.74509079444783843, 74.90852043434034613 ) ) ;
#29114=EDGE_CURVE ( 'NONE', #33155, #35366, #40698, .T. ) ;
#29115=EDGE_CURVE ( 'NONE', #11354, #42239, #26836, .T. ) ;
#29116=DIRECTION ( 'NONE',  ( -7.166348394334737576E-06, 1.030346079289304524E-05, 0.9999999999212411117 ) ) ;
#29117=VERTEX_POINT ( 'NONE', #5624 ) ;
#29120=ADVANCED_FACE ( 'NONE', ( #46248 ), #2413, .T. ) ;
#29121=AXIS2_PLACEMENT_3D ( 'NONE', #15173, #30231, #34138 ) ;
#29123=CARTESIAN_POINT ( 'NONE',  ( -18.11889358109259973, -21.82488563948435711, 65.64532159284070190 ) ) ;
#29126=CARTESIAN_POINT ( 'NONE',  ( -16.44450580018572339, -21.74194830683597957, 65.41491530808407617 ) ) ;
#29127=ORIENTED_EDGE ( 'NONE', *, *, #17843, .T. ) ;
#29130=VERTEX_POINT ( 'NONE', #17871 ) ;
#29131=EDGE_CURVE ( 'NONE', #29545, #20111, #3114, .T. ) ;
#29132=CARTESIAN_POINT ( 'NONE',  ( -17.34580053807816924, -7.359449399152106608, 67.18072987562666754 ) ) ;
#29133=CARTESIAN_POINT ( 'NONE',  ( -19.12163971562669218, -7.963538243666484107, 67.31560661829935555 ) ) ;
#29134=B_SPLINE_CURVE_WITH_KNOTS ( 'NONE', 3,
 ( #25819, #22884, #7124, #22140, #18417, #22375, #33422, #26311, #11536, #14697 ),
 .UNSPECIFIED., .F., .F.,
 ( 4, 2, 2, 2, 4 ),
 ( 0.6272669072877884444, 0.7522669073072847379, 0.8772669073267809203, 1.002266907346277325, 1.127266907365773507 ),
 .UNSPECIFIED. ) ;
#29135=CARTESIAN_POINT ( 'NONE',  ( -23.41616298382994898, -18.52428493080399008, 72.77840375779385340 ) ) ;
#29136=CARTESIAN_POINT ( 'NONE',  ( -10.37382936219775154, -14.83089353207902050, 74.81251018390587149 ) ) ;
#29137=VERTEX_POINT ( 'NONE', #9795 ) ;
#29139=CARTESIAN_POINT ( 'NONE',  ( -19.29341177869643431, -22.02104676444090359, 58.68653925579838671 ) ) ;
#29140=CARTESIAN_POINT ( 'NONE',  ( -22.04378365035703879, -20.13510231884741231, 62.24911246861644543 ) ) ;
#29141=ORIENTED_EDGE ( 'NONE', *, *, #43150, .F. ) ;
#29145=ORIENTED_EDGE ( 'NONE', *, *, #35597, .T. ) ;
#29146=CARTESIAN_POINT ( 'NONE',  ( -17.72634082312590920, -21.85272461445201486, 58.40553378267873796 ) ) ;
#29147=CARTESIAN_POINT ( 'NONE',  ( -21.48252188606478086, -21.05763224395268196, 69.16794793541382091 ) ) ;
#29148=PLANE ( 'NONE',  #45468 ) ;
#29149=ORIENTED_EDGE ( 'NONE', *, *, #13606, .F. ) ;
#29150=CARTESIAN_POINT ( 'NONE',  ( -20.12289019246589206, -7.865124395032225380, 73.90592041591946781 ) ) ;
#29151=CARTESIAN_POINT ( 'NONE',  ( -24.82750207115152463, -13.97654542584719373, 73.30766806548945169 ) ) ;
#29153=EDGE_CURVE ( 'NONE', #30489, #25477, #25523, .T. ) ;
#29154=CARTESIAN_POINT ( 'NONE',  ( -10.75977711076063414, -17.10919593975601316, 61.15743126648893480 ) ) ;
#29155=CARTESIAN_POINT ( 'NONE',  ( -23.96897392247960923, -17.29205672707886166, 66.05243358630347927 ) ) ;
#29157=B_SPLINE_CURVE_WITH_KNOTS ( 'NONE', 3,
 ( #1250, #14184, #29239, #43302, #39592, #5868, #35879, #2161, #47230, #32452 ),
 .UNSPECIFIED., .F., .F.,
 ( 4, 2, 2, 2, 4 ),
 ( 0.000000000000000000, 0.2500000000000000000, 0.5000000000000000000, 0.7500000000000000000, 1.000000000000000000 ),
 .UNSPECIFIED. ) ;
#29159=CARTESIAN_POINT ( 'NONE',  ( -11.98246295270348050, -15.60836430055780610, 53.49999999999995026 ) ) ;
#29160=( BOUNDED_CURVE ( )  B_SPLINE_CURVE ( 3, ( #37371, #26558, #12030, #4168 ),
 .UNSPECIFIED., .F., .F. ) 
 B_SPLINE_CURVE_WITH_KNOTS ( ( 4, 4 ),
 ( 0.4074455897393628456, 0.5000000000000000000 ),
 .UNSPECIFIED. ) 
 CURVE ( )  GEOMETRIC_REPRESENTATION_ITEM ( )  RATIONAL_B_SPLINE_CURVE ( ( 0.6983129098260804080, 0.7760317562606710018, 0.8765941196519728695, 0.9999999999999741318 ) ) 
 REPRESENTATION_ITEM ( '' )  );
#29161=LINE ( 'NONE', #44208, #19516 ) ;
#29164=VECTOR ( 'NONE', #34041, 1000.000000000000114 ) ;
#29166=CARTESIAN_POINT ( 'NONE',  ( -23.62573085457600541, -18.93877797592854506, 65.93734031310268051 ) ) ;
#29167=ORIENTED_EDGE ( 'NONE', *, *, #8216, .T. ) ;
#29169=CARTESIAN_POINT ( 'NONE',  ( -14.01118748589247964, -10.49619482288619565, 54.07175714974879099 ) ) ;
#29170=CARTESIAN_POINT ( 'NONE',  ( -11.73709015858045035, -9.996482182051650511, 67.67709622917277557 ) ) ;
#29175=ORIENTED_EDGE ( 'NONE', *, *, #15478, .F. ) ;
#29179=CARTESIAN_POINT ( 'NONE',  ( -21.30779305846920479, -20.69320811116774195, 72.53006253430444872 ) ) ;
#29180=ADVANCED_FACE ( 'NONE', ( #5853 ), #14169, .T. ) ;
#29182=DIRECTION ( 'NONE',  ( 0.4599824152910791941, 0.8879280250239793837, 2.250728352126283350E-08 ) ) ;
#29183=FACE_OUTER_BOUND ( 'NONE', #44271, .T. ) ;
#29186=ORIENTED_EDGE ( 'NONE', *, *, #38661, .T. ) ;
#29187=ADVANCED_FACE ( 'NONE', ( #20867 ), #2393, .T. ) ;
#29192=EDGE_CURVE ( 'NONE', #25531, #41086, #35474, .T. ) ;
#29195=LINE ( 'NONE', #33587, #43512 ) ;
#29197=CARTESIAN_POINT ( 'NONE',  ( -24.79781851656146330, -15.87314393256401424, 69.64812203948034153 ) ) ;
#29198=DIRECTION ( 'NONE',  ( 0.6621635203543606574, 0.7493593746073508033, 2.316976118889566110E-08 ) ) ;
#29200=CARTESIAN_POINT ( 'NONE',  ( -18.78767905735283605, -20.13749289187802916, 54.07175714974878389 ) ) ;
#29201=ORIENTED_EDGE ( 'NONE', *, *, #29829, .F. ) ;
#29203=DIRECTION ( 'NONE',  ( 1.522745436688331916E-06, -7.096186242782870827E-06, 0.9999999999736625123 ) ) ;
#29204=CARTESIAN_POINT ( 'NONE',  ( -19.47326719839287890, -21.50389106269314965, 65.53656487971998956 ) ) ;
#29205=CARTESIAN_POINT ( 'NONE',  ( -24.42338697892460075, -14.97596148503881786, 59.47130019869695161 ) ) ;
#29206=CARTESIAN_POINT ( 'NONE',  ( -9.995192866514953423, -14.24820641570412683, 64.49529709569884517 ) ) ;
#29208=ORIENTED_EDGE ( 'NONE', *, *, #29389, .F. ) ;
#29210=ADVANCED_FACE ( 'NONE', ( #32199 ), #40309, .T. ) ;
#29212=LINE ( 'NONE', #43273, #22924 ) ;
#29213=ORIENTED_EDGE ( 'NONE', *, *, #36586, .T. ) ;
#29214=FACE_OUTER_BOUND ( 'NONE', #3360, .T. ) ;
#29215=DIRECTION ( 'NONE',  ( 5.329554274754248866E-07, 1.313503380136696700E-06, 0.9999999999989952482 ) ) ;
#29216=DIRECTION ( 'NONE',  ( -0.9345716196833626643, 0.3557750520798445559, 2.412542607589989711E-09 ) ) ;
#29217=ORIENTED_EDGE ( 'NONE', *, *, #8665, .F. ) ;
#29218=CARTESIAN_POINT ( 'NONE',  ( -14.86359179994916246, -21.80616968373489684, 65.29251951080507865 ) ) ;
#29219=VERTEX_POINT ( 'NONE', #43530 ) ;
#29220=CARTESIAN_POINT ( 'NONE',  ( -10.99582063857411995, -11.91441743271276188, 74.55840195587596497 ) ) ;
#29221=CARTESIAN_POINT ( 'NONE',  ( -13.70160630012599157, -20.73736701164767027, 61.62532223698378431 ) ) ;
#29222=CARTESIAN_POINT ( 'NONE',  ( -24.41778221492472412, -14.51057486539872876, 62.93969914534589094 ) ) ;
#29226=CARTESIAN_POINT ( 'NONE',  ( -24.17899325218984785, -11.66673737571591296, 59.66731058339561855 ) ) ;
#29227=CARTESIAN_POINT ( 'NONE',  ( -23.30282546666849086, -18.60927426030231047, 69.59371984657600763 ) ) ;
#29228=ORIENTED_EDGE ( 'NONE', *, *, #1090, .F. ) ;
#29229=CARTESIAN_POINT ( 'NONE',  ( -9.982647249627337516, -14.45068338159927990, 68.11446040317247252 ) ) ;
#29231=AXIS2_PLACEMENT_3D ( 'NONE', #3466, #29089, #17988 ) ;
#29234=CARTESIAN_POINT ( 'NONE',  ( -15.28965001900414755, -21.53148179447737220, 64.99108044553886998 ) ) ;
#29236=CARTESIAN_POINT ( 'NONE',  ( -13.10977233404386944, -20.39504592733330313, 58.19083229533344337 ) ) ;
#29237=( BOUNDED_CURVE ( )  B_SPLINE_CURVE ( 3, ( #46262, #32213, #43301, #43046 ),
 .UNSPECIFIED., .F., .F. ) 
 B_SPLINE_CURVE_WITH_KNOTS ( ( 4, 4 ),
 ( 0.5000000000000000000, 0.9074455897393632897 ),
 .UNSPECIFIED. ) 
 CURVE ( )  GEOMETRIC_REPRESENTATION_ITEM ( )  RATIONAL_B_SPLINE_CURVE ( ( 0.9999999999999968914, 0.4567392136813324122, 0.3561768502900325428, 0.6983129098260938417 ) ) 
 REPRESENTATION_ITEM ( '' )  );
#29238=FACE_OUTER_BOUND ( 'NONE', #8712, .T. ) ;
#29239=CARTESIAN_POINT ( 'NONE',  ( -19.48861532486628434, -21.49789759945147694, 62.01006052078847119 ) ) ;
#29241=CARTESIAN_POINT ( 'NONE',  ( -11.25989573505624364, -11.38792594226331190, 64.14882039369129529 ) ) ;
#29243=EDGE_LOOP ( 'NONE', ( #22308, #28744 ) ) ;
#29244=ORIENTED_EDGE ( 'NONE', *, *, #33209, .F. ) ;
#29247=CARTESIAN_POINT ( 'NONE',  ( -23.70135487130767515, -11.71146637837649074, 63.25218278684473461 ) ) ;
#29249=CARTESIAN_POINT ( 'NONE',  ( -19.99112905230247961, -8.296885111154901793, 73.72096600045514947 ) ) ;
#29250=CARTESIAN_POINT ( 'NONE',  ( -23.68653687815194786, -11.57061008776568123, 66.43686604568146947 ) ) ;
#29251=CARTESIAN_POINT ( 'NONE',  ( -10.97672180207948145, -17.53854803984884470, 71.63888375208067316 ) ) ;
#29253=CARTESIAN_POINT ( 'NONE',  ( -12.18836193727821460, -19.53083876418623532, 57.94154444592973618 ) ) ;
#29254=EDGE_LOOP ( 'NONE', ( #39808, #10186 ) ) ;
#29257=B_SPLINE_CURVE_WITH_KNOTS ( 'NONE', 1,
 ( #16835, #19578 ),
 .UNSPECIFIED., .F., .F.,
 ( 2, 2 ),
 ( 0.000000000000000000, 1.000000000000000000 ),
 .UNSPECIFIED. ) ;
#29261=CARTESIAN_POINT ( 'NONE',  ( -10.03035355355731006, -15.72374577095404824, 61.22284339518546403 ) ) ;
#29263=ORIENTED_EDGE ( 'NONE', *, *, #32241, .T. ) ;
#29264=ADVANCED_FACE ( 'NONE', ( #38056 ), #25697, .T. ) ;
#29266=EDGE_CURVE ( 'NONE', #42055, #8895, #42970, .T. ) ;
#29267=CARTESIAN_POINT ( 'NONE',  ( -14.54749350918766204, -8.372447261038935551, 64.07506791522041567 ) ) ;
#29269=EDGE_CURVE ( 'NONE', #8530, #31901, #4343, .T. ) ;
#29270=CARTESIAN_POINT ( 'NONE',  ( -14.05371270701021480, -21.00138147690670820, 71.92607703580546286 ) ) ;
#29271=CARTESIAN_POINT ( 'NONE',  ( -24.12044147510846059, -12.60386701182102698, 73.24785355581104795 ) ) ;
#29272=EDGE_LOOP ( 'NONE', ( #2740, #17832, #14684, #34128, #15432 ) ) ;
#29274=VERTEX_POINT ( 'NONE', #33880 ) ;
#29275=FACE_OUTER_BOUND ( 'NONE', #24323, .T. ) ;
#29276=FACE_OUTER_BOUND ( 'NONE', #45554, .T. ) ;
#29277=ORIENTED_EDGE ( 'NONE', *, *, #10924, .T. ) ;
#29278=CARTESIAN_POINT ( 'NONE',  ( -13.71897584585257235, -21.27267513736575566, 68.57812350262666712 ) ) ;
#29279=DIRECTION ( 'NONE',  ( -0.9893521221787096032, 0.1455416721783832079, 6.188545272020285247E-08 ) ) ;
#29280=ORIENTED_EDGE ( 'NONE', *, *, #18242, .T. ) ;
#29281=CARTESIAN_POINT ( 'NONE',  ( -18.84910040211995863, -7.954480482427757515, 70.44238404915014939 ) ) ;
#29282=( BOUNDED_CURVE ( )  B_SPLINE_CURVE ( 3, ( #4570, #23294, #27943, #38279 ),
 .UNSPECIFIED., .F., .F. ) 
 B_SPLINE_CURVE_WITH_KNOTS ( ( 4, 4 ),
 ( 0.4074455897393617909, 0.5000000000000000000 ),
 .UNSPECIFIED. ) 
 CURVE ( )  GEOMETRIC_REPRESENTATION_ITEM ( )  RATIONAL_B_SPLINE_CURVE ( ( 0.6983129098260847378, 0.7760317562606787734, 0.8765941196519803080, 0.9999999999999805711 ) ) 
 REPRESENTATION_ITEM ( '' )  );
#29283=CARTESIAN_POINT ( 'NONE',  ( -11.11225360959527819, -18.76719628086529212, 61.43744160855001013 ) ) ;
#29285=ORIENTED_EDGE ( 'NONE', *, *, #37063, .T. ) ;
#29289=ORIENTED_EDGE ( 'NONE', *, *, #15596, .F. ) ;
#29290=ORIENTED_EDGE ( 'NONE', *, *, #19436, .F. ) ;
#29291=CARTESIAN_POINT ( 'NONE',  ( -23.38871250174943839, -10.34516057075380679, 59.72486561860700505 ) ) ;
#29292=CARTESIAN_POINT ( 'NONE',  ( -16.85710124362929463, -7.832207225656589777, 74.15121474590814898 ) ) ;
#29294=CARTESIAN_POINT ( 'NONE',  ( -22.71334156758821265, -10.13600392596141475, 63.22752948238618842 ) ) ;
#29295=CARTESIAN_POINT ( 'NONE',  ( -13.28240554951661245, -9.100331501070346718, 67.79431631125400770 ) ) ;
#29296=CARTESIAN_POINT ( 'NONE',  ( -23.70782535920394452, -18.81166901052139551, 69.43225427700679120 ) ) ;
#29297=( BOUNDED_CURVE ( )  B_SPLINE_CURVE ( 3, ( #26769, #907, #27482, #34372 ),
 .UNSPECIFIED., .F., .F. ) 
 B_SPLINE_CURVE_WITH_KNOTS ( ( 4, 4 ),
 ( 1.570796326794896780, 1.780235837034217283 ),
 .UNSPECIFIED. ) 
 CURVE ( )  GEOMETRIC_REPRESENTATION_ITEM ( )  RATIONAL_B_SPLINE_CURVE ( ( 1.000000000000000000, 0.9963479302455154896, 0.9963479302455154896, 1.000000000000000000 ) ) 
 REPRESENTATION_ITEM ( '' )  );
#29298=FACE_OUTER_BOUND ( 'NONE', #8293, .T. ) ;
#29300=EDGE_CURVE ( 'NONE', #4669, #35358, #22081, .T. ) ;
#29301=CARTESIAN_POINT ( 'NONE',  ( 0.000000000000000000, 0.000000000000000000, 0.000000000000000000 ) ) ;
#29303=CARTESIAN_POINT ( 'NONE',  ( -11.64902330566212463, -10.02396254413167576, 54.27966884056655061 ) ) ;
#29305=( BOUNDED_SURFACE ( )  B_SPLINE_SURFACE ( 3, 1, ( 
 ( #14742, #48030 ),
 ( #36670, #25386 ),
 ( #41131, #3212 ),
 ( #41365, #10380 ),
 ( #11341, #22181 ),
 ( #32986, #29811 ),
 ( #22415, #44586 ) ),
 .UNSPECIFIED., .T., .F., .F. ) 
 B_SPLINE_SURFACE_WITH_KNOTS ( ( 4, 3, 4 ),
 ( 2, 2 ),
 ( 0.000000000000000000, 0.5000000000000000000, 1.000000000000000000 ),
 ( 0.000000000000000000, 1.000000000000000000 ),
 .UNSPECIFIED. ) 
 GEOMETRIC_REPRESENTATION_ITEM ( )  RATIONAL_B_SPLINE_SURFACE ( (
 ( 1.000000000000000000, 1.000000000000000000),
 ( 0.3333333333333335369, 0.3333333333333330373),
 ( 0.3333333333333335369, 0.3333333333333330373),
 ( 1.000000000000000000, 1.000000000000000000),
 ( 0.3333333333333333703, 0.3333333333333333703),
 ( 0.3333333333333333703, 0.3333333333333333703),
 ( 1.000000000000000000, 1.000000000000000000) ) ) 
 REPRESENTATION_ITEM ( '' )  SURFACE ( )  );
#29306=ORIENTED_EDGE ( 'NONE', *, *, #10569, .F. ) ;
#29308=CARTESIAN_POINT ( 'NONE',  ( -24.46146587544552276, -14.38248120490118787, 66.46820668217904426 ) ) ;
#29309=CARTESIAN_POINT ( 'NONE',  ( -23.92344128327244590, -11.16753467582692672, 69.99936603959443460 ) ) ;
#29310=CARTESIAN_POINT ( 'NONE',  ( -11.63532267033605372, -18.83847007233952908, 72.10174756685907482 ) ) ;
#29312=EDGE_CURVE ( 'NONE', #43753, #43742, #19351, .T. ) ;
#29313=CARTESIAN_POINT ( 'NONE',  ( -18.63018970549565978, -7.457396494496333794, 73.95569010969242640 ) ) ;
#29314=B_SPLINE_CURVE_WITH_KNOTS ( 'NONE', 3,
 ( #25068, #22336, #6595, #48677, #18382, #14421, #11015, #47706, #6352, #6830 ),
 .UNSPECIFIED., .F., .F.,
 ( 4, 2, 2, 2, 4 ),
 ( 0.1272669073658570793, 0.2522669073463325029, 0.3772669073268078987, 0.5022669073072834056, 0.6272669072877588015 ),
 .UNSPECIFIED. ) ;
#29318=EDGE_CURVE ( 'NONE', #14220, #17691, #37200, .T. ) ;
#29320=CARTESIAN_POINT ( 'NONE',  ( -13.65110067086344792, -21.23324738024127356, 68.57129742521463811 ) ) ;
#29321=CARTESIAN_POINT ( 'NONE',  ( -19.69914571794098990, -21.90346627284599634, 65.58769322485436248 ) ) ;
#29322=CARTESIAN_POINT ( 'NONE',  ( -24.76566745545338222, -16.07607805037886450, 66.31970875637813378 ) ) ;
#29323=ORIENTED_EDGE ( 'NONE', *, *, #3535, .T. ) ;
#29325=ORIENTED_EDGE ( 'NONE', *, *, #14607, .T. ) ;
#29326=CARTESIAN_POINT ( 'NONE',  ( -23.81973173699715574, -10.98832876278002502, 73.46919161870800963 ) ) ;
#29327=CARTESIAN_POINT ( 'NONE',  ( -24.38867418725816805, -14.10591363164734524, 69.84378491695960633 ) ) ;
#29328=VERTEX_POINT ( 'NONE', #411 ) ;
#29329=CARTESIAN_POINT ( 'NONE',  ( -24.44689184067228638, -14.18710713894228270, 69.93803194250308763 ) ) ;
#29330=CARTESIAN_POINT ( 'NONE',  ( -24.47354813883760016, -12.39902559715248032, 73.42720875634239519 ) ) ;
#29331=AXIS2_PLACEMENT_3D ( 'NONE', #37528, #32868, #18087 ) ;
#29333=CARTESIAN_POINT ( 'NONE',  ( -18.50162525266306091, -21.72577549820248421, 72.58510940979837756 ) ) ;
#29334=CARTESIAN_POINT ( 'NONE',  ( -23.91010245674826251, -17.57297063409389537, 62.75888927877479517 ) ) ;
#29336=CARTESIAN_POINT ( 'NONE',  ( -23.96075645138428101, -17.45014240273063066, 65.94357239682317129 ) ) ;
#29337=EDGE_LOOP ( 'NONE', ( #6539, #12064, #6619, #38668, #18713 ) ) ;
#29338=CARTESIAN_POINT ( 'NONE',  ( -20.43185948505062299, -8.432683554863363184, 66.79576150497511833 ) ) ;
#29339=CARTESIAN_POINT ( 'NONE',  ( -10.36816553299425792, -14.63937932467125691, 64.54370954096965818 ) ) ;
#29340=CARTESIAN_POINT ( 'NONE',  ( -14.48682561153071902, -7.962540396457996827, 63.91261920127995211 ) ) ;
#29342=CARTESIAN_POINT ( 'NONE',  ( -10.81476099607377961, -12.49952454704760996, 61.02683403436387977 ) ) ;
#29343=CARTESIAN_POINT ( 'NONE',  ( -24.27720304158778575, -16.23785116329529643, 62.87712181919398802 ) ) ;
#29345=ORIENTED_EDGE ( 'NONE', *, *, #7275, .F. ) ;
#29348=CARTESIAN_POINT ( 'NONE',  ( -23.93648101794248362, -17.51022725521227841, 65.95829288617392194 ) ) ;
#29351=CARTESIAN_POINT ( 'NONE',  ( -11.75134375414733334, -18.91116183774077797, 71.97069383046880375 ) ) ;
#29352=FACE_OUTER_BOUND ( 'NONE', #6977, .T. ) ;
#29353=CARTESIAN_POINT ( 'NONE',  ( -10.64854695470030599, -12.86019059820356780, 64.55364013863997741 ) ) ;
#29354=CARTESIAN_POINT ( 'NONE',  ( -12.05615996164320691, -19.97535249625256526, 61.51183308442717390 ) ) ;
#29355=FACE_BOUND ( 'NONE', #20340, .T. ) ;
#29356=CARTESIAN_POINT ( 'NONE',  ( -23.86426273889453498, -17.55550152358811999, 66.01527417605778680 ) ) ;
#29357=CARTESIAN_POINT ( 'NONE',  ( -10.42297872178580853, -14.76125658070002622, 75.02608819853371358 ) ) ;
#29358=DIRECTION ( 'NONE',  ( -8.419732596317119940E-06, 4.907637675873463559E-06, 0.9999999999525115424 ) ) ;
#29359=ORIENTED_EDGE ( 'NONE', *, *, #36195, .T. ) ;
#29360=DIRECTION ( 'NONE',  ( -0.8651630202045381690, 0.5014907262059381532, 5.433021001366390361E-08 ) ) ;
#29362=ADVANCED_FACE ( 'NONE', ( #8776 ), #23548, .T. ) ;
#29363=B_SPLINE_CURVE_WITH_KNOTS ( 'NONE', 3,
 ( #24881, #39894, #6166, #21191, #47763, #13999, #29053, #44100, #41345, #250 ),
 .UNSPECIFIED., .F., .F.,
 ( 4, 2, 2, 2, 4 ),
 ( 0.1272669073658642125, 0.2522669073439609555, 0.3772669073220577540, 0.5022669073001545526, 0.6272669072782512956 ),
 .UNSPECIFIED. ) ;
#29364=CARTESIAN_POINT ( 'NONE',  ( -16.98991503782990975, -22.24662993548692214, 72.35038528954983406 ) ) ;
#29367=CARTESIAN_POINT ( 'NONE',  ( -14.91789657710648598, -21.40191547797545724, 58.05129291223532562 ) ) ;
#29369=ORIENTED_EDGE ( 'NONE', *, *, #4430, .T. ) ;
#29370=ORIENTED_EDGE ( 'NONE', *, *, #18095, .F. ) ;
#29371=B_SPLINE_CURVE_WITH_KNOTS ( 'NONE', 3,
 ( #12652, #38505, #4787, #1313, #16324, #34812, #16084, #46146, #31366, #23991 ),
 .UNSPECIFIED., .F., .F.,
 ( 4, 2, 2, 2, 4 ),
 ( 0.6272669072877984364, 0.7522669073073017243, 0.8772669073268051232, 1.002266907346308411, 1.127266907365811699 ),
 .UNSPECIFIED. ) ;
#29373=ORIENTED_EDGE ( 'NONE', *, *, #16635, .T. ) ;
#29376=CARTESIAN_POINT ( 'NONE',  ( -12.05806040642128707, -10.23620046216302448, 67.51368956197082127 ) ) ;
#29378=EDGE_CURVE ( 'NONE', #33946, #38947, #31658, .T. ) ;
#29379=EDGE_CURVE ( 'NONE', #33854, #19106, #32872, .T. ) ;
#29380=CARTESIAN_POINT ( 'NONE',  ( -15.54494036203377405, -7.599968873926485458, 70.73177050285754319 ) ) ;
#29382=CARTESIAN_POINT ( 'NONE',  ( -13.88833677318074500, -20.91193151007171736, 64.87139997340349851 ) ) ;
#29383=CARTESIAN_POINT ( 'NONE',  ( -12.42993038278122597, -9.833123725877770838, 57.08935529208049076 ) ) ;
#29386=DIRECTION ( 'NONE',  ( -6.919810407550069512E-06, -1.067025350021132924E-05, 0.9999999999191310218 ) ) ;
#29387=VERTEX_POINT ( 'NONE', #46677 ) ;
#29389=EDGE_CURVE ( 'NONE', #38508, #47624, #1651, .T. ) ;
#29390=CARTESIAN_POINT ( 'NONE',  ( -10.93232766038821424, -17.55941949638709687, 68.38249893951126523 ) ) ;
#29391=CARTESIAN_POINT ( 'NONE',  ( -12.14425517392406917, -10.13739710456042964, 64.17914326607970565 ) ) ;
#29392=CARTESIAN_POINT ( 'NONE',  ( -23.00454255336054743, -10.50046069577333263, 59.88731295783226471 ) ) ;
#29394=CARTESIAN_POINT ( 'NONE',  ( -20.18941624216641273, -7.891347737435665977, 73.83601159825586535 ) ) ;
#29395=ADVANCED_FACE ( 'NONE', ( #1609 ), #15892, .F. ) ;
#29397=CARTESIAN_POINT ( 'NONE',  ( -13.85393650630732054, -8.270265118416840977, 74.38450092284953996 ) ) ;
#29398=CARTESIAN_POINT ( 'NONE',  ( -23.91439714532632621, -17.43141235356291574, 65.94357239632037704 ) ) ;
#29401=FACE_OUTER_BOUND ( 'NONE', #39868, .T. ) ;
#29402=CARTESIAN_POINT ( 'NONE',  ( -16.39155704513022016, -21.78318439201321866, 61.75568132354042916 ) ) ;
#29403=CARTESIAN_POINT ( 'NONE',  ( -11.64873123714592396, -10.76074834137913960, 74.32396018297762907 ) ) ;
#29406=VERTEX_POINT ( 'NONE', #892 ) ;
#29407=CARTESIAN_POINT ( 'NONE',  ( -24.19028598586675116, -12.80082241304059210, 62.98831023884616798 ) ) ;
#29409=VERTEX_POINT ( 'NONE', #31406 ) ;
#29412=CARTESIAN_POINT ( 'NONE',  ( -18.69922557824643761, -7.468382084482742655, 74.02719791125277027 ) ) ;
#29413=ORIENTED_EDGE ( 'NONE', *, *, #15162, .T. ) ;
#29416=ORIENTED_EDGE ( 'NONE', *, *, #10402, .F. ) ;
#29417=ORIENTED_EDGE ( 'NONE', *, *, #5545, .F. ) ;
#29419=CARTESIAN_POINT ( 'NONE',  ( -18.81087689773607607, -7.489408793048438540, 70.57079237633290347 ) ) ;
#29421=CARTESIAN_POINT ( 'NONE',  ( -13.38575581802539993, -9.030060914960570173, 60.72478133471773987 ) ) ;
#29422=ORIENTED_EDGE ( 'NONE', *, *, #43293, .F. ) ;
#29423=ORIENTED_EDGE ( 'NONE', *, *, #43427, .T. ) ;
#29425=B_SPLINE_CURVE_WITH_KNOTS ( 'NONE', 1,
 ( #23340, #5115 ),
 .UNSPECIFIED., .F., .F.,
 ( 2, 2 ),
 ( 0.000000000000000000, 1.000000000000000000 ),
 .UNSPECIFIED. ) ;
#29426=CARTESIAN_POINT ( 'NONE',  ( -11.48080861122161167, -10.31672956615889269, 74.60031634573793724 ) ) ;
#29428=( BOUNDED_CURVE ( )  B_SPLINE_CURVE ( 3, ( #40053, #2619, #24795, #32424 ),
 .UNSPECIFIED., .F., .F. ) 
 B_SPLINE_CURVE_WITH_KNOTS ( ( 4, 4 ),
 ( 0.5000000000000000000, 0.9074455897393665094 ),
 .UNSPECIFIED. ) 
 CURVE ( )  GEOMETRIC_REPRESENTATION_ITEM ( )  RATIONAL_B_SPLINE_CURVE ( ( 1.000000000000025757, 0.4567392136813333003, 0.3561768502900126698, 0.6983129098260916212 ) ) 
 REPRESENTATION_ITEM ( '' )  );
#29431=EDGE_CURVE ( 'NONE', #918, #38805, #10788, .T. ) ;
#29434=CARTESIAN_POINT ( 'NONE',  ( -18.50932193227059486, -21.77517953109191140, 72.58510940649487964 ) ) ;
#29435=CARTESIAN_POINT ( 'NONE',  ( -24.41275629217255272, -14.38907661853721542, 69.88105113750283692 ) ) ;
#29436=ORIENTED_EDGE ( 'NONE', *, *, #47131, .F. ) ;
#29438=( BOUNDED_CURVE ( )  B_SPLINE_CURVE ( 3, ( #34991, #16261, #42154, #38438 ),
 .UNSPECIFIED., .F., .F. ) 
 B_SPLINE_CURVE_WITH_KNOTS ( ( 4, 4 ),
 ( 0.4074455897393596260, 0.5000000000000000000 ),
 .UNSPECIFIED. ) 
 CURVE ( )  GEOMETRIC_REPRESENTATION_ITEM ( )  RATIONAL_B_SPLINE_CURVE ( ( 0.6983129098260744128, 0.7760317562606953157, 0.8765941196520076195, 1.000000000000020872 ) ) 
 REPRESENTATION_ITEM ( '' )  );
#29442=DIRECTION ( 'NONE',  ( 0.9753750245375039096, 0.2205528542287732985, 7.244220459260265297E-08 ) ) ;
#29443=CARTESIAN_POINT ( 'NONE',  ( -24.42383174400572088, -14.88139811306343496, 59.24300232022908830 ) ) ;
#29447=CARTESIAN_POINT ( 'NONE',  ( -10.31252162633752079, -12.58677457285831913, 60.91198276946202128 ) ) ;
#29448=CARTESIAN_POINT ( 'NONE',  ( -24.21202825980905615, -11.73864819121529912, 59.60518815382388169 ) ) ;
#29450=CARTESIAN_POINT ( 'NONE',  ( -11.25989573505624364, -11.38792594226331190, 64.14882039369129529 ) ) ;
#29452=VERTEX_POINT ( 'NONE', #42256 ) ;
#29453=DIRECTION ( 'NONE',  ( 0.7915359335728471279, 0.6111226275167354061, 5.146443701300904349E-08 ) ) ;
#29455=CARTESIAN_POINT ( 'NONE',  ( -12.59783444659965390, -19.87951993436981368, 65.15209581050474696 ) ) ;
#29457=FACE_BOUND ( 'NONE', #35225, .T. ) ;
#29458=ORIENTED_EDGE ( 'NONE', *, *, #16884, .F. ) ;
#29459=LINE ( 'NONE', #7805, #37600 ) ;
#29460=LINE ( 'NONE', #2861, #9033 ) ;
#29464=CARTESIAN_POINT ( 'NONE',  ( -10.47191917896302371, -13.98145069646090022, 60.98991602035415838 ) ) ;
#29465=VERTEX_POINT ( 'NONE', #4576 ) ;
#29466=CARTESIAN_POINT ( 'NONE',  ( -16.81468282041412010, -21.83654306051557015, 65.22564162490351691 ) ) ;
#29467=CARTESIAN_POINT ( 'NONE',  ( -23.68653687815194786, -11.57061008776568123, 66.43686604568146947 ) ) ;
#29473=ORIENTED_EDGE ( 'NONE', *, *, #48207, .T. ) ;
#29474=ORIENTED_EDGE ( 'NONE', *, *, #5632, .T. ) ;
#29475=CARTESIAN_POINT ( 'NONE',  ( -15.62301844010884899, -8.044815583578751372, 70.89524431202903543 ) ) ;
#29476=CARTESIAN_POINT ( 'NONE',  ( -20.50783594841701785, -8.027295835816985914, 66.96599399791791996 ) ) ;
#29478=CARTESIAN_POINT ( 'NONE',  ( -16.57395829291861844, -22.21062093300318807, 65.26918445414273151 ) ) ;
#29479=CARTESIAN_POINT ( 'NONE',  ( -12.37644160373227287, -19.65923220176213349, 61.69678630681026732 ) ) ;
#29480=CARTESIAN_POINT ( 'NONE',  ( -16.13263948075386978, -7.878200451182638453, 63.68483172840383588 ) ) ;
#29481=CARTESIAN_POINT ( 'NONE',  ( -22.83095763869631512, -19.93459457198476770, 72.82895875648904394 ) ) ;
#29483=EDGE_LOOP ( 'NONE', ( #46493, #3215, #5883, #4979, #15386 ) ) ;
#29484=CARTESIAN_POINT ( 'NONE',  ( -13.25302027261275484, -9.121009434035636687, 60.64769990268487732 ) ) ;
#29485=CARTESIAN_POINT ( 'NONE',  ( -23.09419775198653468, -9.976756388841243606, 66.64158628164071274 ) ) ;
#29488=CARTESIAN_POINT ( 'NONE',  ( -24.30048628764226137, -16.36411057843138650, 59.27332431757403697 ) ) ;
#29489=EDGE_LOOP ( 'NONE', ( #18693, #43998, #9428, #42950, #34738 ) ) ;
#29490=EDGE_CURVE ( 'NONE', #32198, #11365, #26988, .T. ) ;
#29492=ORIENTED_EDGE ( 'NONE', *, *, #23693, .F. ) ;
#29494=CARTESIAN_POINT ( 'NONE',  ( -12.09300774956044755, -19.42703681131052562, 58.34171032836335513 ) ) ;
#29495=CARTESIAN_POINT ( 'NONE',  ( -10.73412848974934874, -11.53077067998621175, 71.20365450754333381 ) ) ;
#29496=ORIENTED_EDGE ( 'NONE', *, *, #34772, .F. ) ;
#29498=CARTESIAN_POINT ( 'NONE',  ( -23.34092575347512266, -10.28207967581048088, 59.78698817202694471 ) ) ;
#29500=EDGE_CURVE ( 'NONE', #22230, #36064, #29542, .T. ) ;
#29501=ORIENTED_EDGE ( 'NONE', *, *, #12060, .F. ) ;
#29502=CARTESIAN_POINT ( 'NONE',  ( -16.97946044980448121, -21.84517136462328324, 72.31543221430108304 ) ) ;
#29503=EDGE_CURVE ( 'NONE', #39013, #773, #21965, .T. ) ;
#29504=CARTESIAN_POINT ( 'NONE',  ( -10.11977905767481900, -16.27558856157159539, 71.55476250049129305 ) ) ;
#29505=ORIENTED_EDGE ( 'NONE', *, *, #11881, .F. ) ;
#29506=DIRECTION ( 'NONE',  ( 0.9375570856950865561, -0.3478314405900308492, 0.000000000000000000 ) ) ;
#29508=CARTESIAN_POINT ( 'NONE',  ( -23.87460028475566887, -17.65420844160683700, 62.47360984062320455 ) ) ;
#29512=VERTEX_POINT ( 'NONE', #13642 ) ;
#29513=CARTESIAN_POINT ( 'NONE',  ( -23.97789761167216938, -17.40771579525701895, 66.23797482430366301 ) ) ;
#29517=( BOUNDED_SURFACE ( )  B_SPLINE_SURFACE ( 3, 1, ( 
 ( #32451, #21128 ),
 ( #2646, #6347 ),
 ( #25063, #39832 ),
 ( #47477, #25534 ),
 ( #43782, #21844 ),
 ( #17655, #10290 ),
 ( #18134, #33385 ) ),
 .UNSPECIFIED., .T., .F., .F. ) 
 B_SPLINE_SURFACE_WITH_KNOTS ( ( 4, 3, 4 ),
 ( 2, 2 ),
 ( 0.000000000000000000, 0.5000000000000000000, 1.000000000000000000 ),
 ( 0.000000000000000000, 1.000000000000000000 ),
 .UNSPECIFIED. ) 
 GEOMETRIC_REPRESENTATION_ITEM ( )  RATIONAL_B_SPLINE_SURFACE ( (
 ( 1.000000000000000000, 1.000000000000000000),
 ( 0.3333333333333335369, 0.3333333333333330373),
 ( 0.3333333333333335369, 0.3333333333333330373),
 ( 1.000000000000000000, 1.000000000000000000),
 ( 0.3333333333333333703, 0.3333333333333333703),
 ( 0.3333333333333333703, 0.3333333333333333703),
 ( 1.000000000000000000, 1.000000000000000000) ) ) 
 REPRESENTATION_ITEM ( '' )  SURFACE ( )  );
#29518=ADVANCED_FACE ( 'NONE', ( #6030 ), #21054, .T. ) ;
#29519=CARTESIAN_POINT ( 'NONE',  ( -11.07866493849470579, -18.71282305161091486, 61.37736592674749403 ) ) ;
#29520=CARTESIAN_POINT ( 'NONE',  ( -23.46013293835336100, -11.16077341686890989, 69.77721965307074470 ) ) ;
#29522=CARTESIAN_POINT ( 'NONE',  ( -24.61605457543312525, -12.86511826566283290, 66.41751344402152313 ) ) ;
#29524=B_SPLINE_CURVE_WITH_KNOTS ( 'NONE', 3,
 ( #32362, #35305, #17062, #42945, #42717, #36024, #39252, #47132, #5533, #20554 ),
 .UNSPECIFIED., .F., .F.,
 ( 4, 2, 2, 2, 4 ),
 ( 0.000000000000000000, 0.2500000000000000000, 0.5000000000000000000, 0.7500000000000000000, 1.000000000000000000 ),
 .UNSPECIFIED. ) ;
#29525=CARTESIAN_POINT ( 'NONE',  ( -24.03992722153932959, -17.24514946215870381, 69.71339794702862491 ) ) ;
#29529=CARTESIAN_POINT ( 'NONE',  ( -23.39264018726221650, -10.35034530683095078, 59.76349971690503082 ) ) ;
#29530=CARTESIAN_POINT ( 'NONE',  ( -11.88369906670657628, -10.53078588752935651, 71.25427731142369225 ) ) ;
#29531=CARTESIAN_POINT ( 'NONE',  ( -10.81170448216924740, -12.36318809540519048, 57.34329390664808557 ) ) ;
#29533=CARTESIAN_POINT ( 'NONE',  ( -15.81235419205221504, -7.945607373518417837, 67.42535135806457447 ) ) ;
#29534=CARTESIAN_POINT ( 'NONE',  ( -13.87299615820197296, -20.90301826156740717, 72.34096506744559463 ) ) ;
#29535=CARTESIAN_POINT ( 'NONE',  ( -19.04853579327176760, -7.948602568230340282, 63.71617106789811658 ) ) ;
#29536=CARTESIAN_POINT ( 'NONE',  ( -14.66287647794328386, -8.376693760123846033, 64.08978834288900828 ) ) ;
#29539=CARTESIAN_POINT ( 'NONE',  ( -24.31986544270498030, -13.34244042609839198, 59.36267955695507226 ) ) ;
#29542=B_SPLINE_CURVE_WITH_KNOTS ( 'NONE', 3,
 ( #5075, #20082, #35088, #12693, #42744, #21775, #28921, #40012, #36761, #47162 ),
 .UNSPECIFIED., .F., .F.,
 ( 4, 2, 2, 2, 4 ),
 ( 0.000000000000000000, 0.2500000000000000000, 0.5000000000000000000, 0.7500000000000000000, 1.000000000000000000 ),
 .UNSPECIFIED. ) ;
#29543=EDGE_CURVE ( 'NONE', #47790, #30264, #19613, .T. ) ;
#29545=VERTEX_POINT ( 'NONE', #39524 ) ;
#29546=CARTESIAN_POINT ( 'NONE',  ( -22.75539019595754908, -10.19575032747719412, 66.82710158566565894 ) ) ;
#29549=CARTESIAN_POINT ( 'NONE',  ( -13.43921408130402817, -8.993432070331126127, 60.73950277491898930 ) ) ;
#29551=EDGE_CURVE ( 'NONE', #23975, #45444, #34247, .T. ) ;
#29552=CARTESIAN_POINT ( 'NONE',  ( -24.48935351541090455, -12.44598921085947119, 73.34251321892850228 ) ) ;
#29553=CARTESIAN_POINT ( 'NONE',  ( -11.35974425695043699, -11.20802616635808313, 64.56370858977317084 ) ) ;
#29555=FACE_OUTER_BOUND ( 'NONE', #47000, .T. ) ;
#29557=( BOUNDED_CURVE ( )  B_SPLINE_CURVE ( 3, ( #31477, #8594, #46021, #16923 ),
 .UNSPECIFIED., .F., .F. ) 
 B_SPLINE_CURVE_WITH_KNOTS ( ( 4, 4 ),
 ( 0.000000000000000000, 0.4074455897393656767 ),
 .UNSPECIFIED. ) 
 CURVE ( )  GEOMETRIC_REPRESENTATION_ITEM ( )  RATIONAL_B_SPLINE_CURVE ( ( 1.000000000000000000, 0.4567392136813333003, 0.3561768502900307665, 0.6983129098260923984 ) ) 
 REPRESENTATION_ITEM ( '' )  );
#29558=FACE_OUTER_BOUND ( 'NONE', #22027, .T. ) ;
#29559=ORIENTED_EDGE ( 'NONE', *, *, #1190, .F. ) ;
#29560=CARTESIAN_POINT ( 'NONE',  ( -11.87166626389854329, -10.45903512182793982, 67.70716783823823448 ) ) ;
#29563=CARTESIAN_POINT ( 'NONE',  ( -23.79882860864043082, -10.95363794417970738, 73.46169666061963710 ) ) ;
#29565=CARTESIAN_POINT ( 'NONE',  ( -19.67760665824181388, -21.48965406232008490, 65.75014118398131302 ) ) ;
#29567=CARTESIAN_POINT ( 'NONE',  ( -21.38142803800936420, -21.12127404432104072, 69.15475944846217260 ) ) ;
#29568=CARTESIAN_POINT ( 'NONE',  ( -19.38509533341928659, -21.58113884793795378, 62.00063448590932325 ) ) ;
#29572=EDGE_CURVE ( 'NONE', #34971, #6268, #2690, .T. ) ;
#29573=CARTESIAN_POINT ( 'NONE',  ( -24.23700366861210753, -17.82382531738836562, 62.73006892227505915 ) ) ;
#29575=CARTESIAN_POINT ( 'NONE',  ( -10.42496409221358178, -14.69883174549087279, 71.32782692796889989 ) ) ;
#29576=EDGE_LOOP ( 'NONE', ( #30096, #15335, #29933, #24801, #43674 ) ) ;
#29577=( BOUNDED_CURVE ( )  B_SPLINE_CURVE ( 3, ( #37443, #3736, #6944, #40429 ),
 .UNSPECIFIED., .F., .F. ) 
 B_SPLINE_CURVE_WITH_KNOTS ( ( 4, 4 ),
 ( 0.9074455897393668424, 1.000000000000000000 ),
 .UNSPECIFIED. ) 
 CURVE ( )  GEOMETRIC_REPRESENTATION_ITEM ( )  RATIONAL_B_SPLINE_CURVE ( ( 0.6983129098260837386, 0.7760317562606902086, 0.8765941196519956291, 1.000000000000000000 ) ) 
 REPRESENTATION_ITEM ( '' )  );
#29579=CARTESIAN_POINT ( 'NONE',  ( -16.13432406759100601, -21.74052631579560568, 58.30057715624173653 ) ) ;
#29580=CARTESIAN_POINT ( 'NONE',  ( -14.47196271362616748, -7.969019419113326563, 63.98317130198068270 ) ) ;
#29585=ORIENTED_EDGE ( 'NONE', *, *, #34543, .F. ) ;
#29586=CARTESIAN_POINT ( 'NONE',  ( -16.98261326800368209, -21.79527086262147861, 72.16543221550985265 ) ) ;
#29587=CARTESIAN_POINT ( 'NONE',  ( -9.975810198805103113, -14.64163036238288740, 71.46749302621661570 ) ) ;
#29589=CARTESIAN_POINT ( 'NONE',  ( -23.99312320239454976, -11.29471777418100231, 66.60709819448160829 ) ) ;
#29590=CARTESIAN_POINT ( 'NONE',  ( -11.70868095541711540, -18.85353058150503713, 71.79759075073991426 ) ) ;
#29591=CARTESIAN_POINT ( 'NONE',  ( -13.38575581802539993, -9.030060914960570173, 60.72478133471773276 ) ) ;
#29592=CARTESIAN_POINT ( 'NONE',  ( -11.57425499491753307, -18.65360305739656610, 64.74707076836355668 ) ) ;
#29595=CARTESIAN_POINT ( 'NONE',  ( -11.21150076820731378, -18.14943614556009166, 57.89894789413084197 ) ) ;
#29596=CARTESIAN_POINT ( 'NONE',  ( -17.65006842549283306, -20.30456235612523841, 54.07175714974878389 ) ) ;
#29597=EDGE_CURVE ( 'NONE', #8440, #17754, #28428, .T. ) ;
#29599=( BOUNDED_CURVE ( )  B_SPLINE_CURVE ( 3, ( #2272, #27651, #2030, #20265 ),
 .UNSPECIFIED., .F., .F. ) 
 B_SPLINE_CURVE_WITH_KNOTS ( ( 4, 4 ),
 ( 0.4074455897393683412, 0.5000000000000000000 ),
 .UNSPECIFIED. ) 
 CURVE ( )  GEOMETRIC_REPRESENTATION_ITEM ( )  RATIONAL_B_SPLINE_CURVE ( ( 0.6983129098260890677, 0.7760317562606889874, 0.8765941196519907441, 0.9999999999999906741 ) ) 
 REPRESENTATION_ITEM ( '' )  );
#29600=CARTESIAN_POINT ( 'NONE',  ( -18.34560609025200861, -9.386954687716537293, 53.49999999999995026 ) ) ;
#29601=EDGE_CURVE ( 'NONE', #31901, #23884, #6086, .T. ) ;
#29603=VERTEX_POINT ( 'NONE', #8000 ) ;
#29604=DIRECTION ( 'NONE',  ( -1.078386540356568435E-05, 7.293043936188563530E-06, -0.9999999999152598962 ) ) ;
#29605=CARTESIAN_POINT ( 'NONE',  ( -10.19958527806322302, -12.98708191879287455, 67.85176988805619658 ) ) ;
#29606=CARTESIAN_POINT ( 'NONE',  ( -24.69984158949002406, -13.20708760842489582, 59.55542051466775888 ) ) ;
#29609=CARTESIAN_POINT ( 'NONE',  ( -14.67242798431547968, -21.73322265534233111, 58.27962637798393786 ) ) ;
#29610=CARTESIAN_POINT ( 'NONE',  ( -23.85974590284097374, -11.05473623917629844, 73.54848671873985211 ) ) ;
#29615=EDGE_LOOP ( 'NONE', ( #42748, #31884 ) ) ;
#29616=CARTESIAN_POINT ( 'NONE',  ( -17.11779890868097809, -21.80256347443895848, 72.39216574764959944 ) ) ;
#29617=CARTESIAN_POINT ( 'NONE',  ( -12.14849447404118088, -10.12808629081546563, 67.91385578414299573 ) ) ;
#29618=CARTESIAN_POINT ( 'NONE',  ( -24.60351398785051558, -12.81959416700296117, 66.50235511976165981 ) ) ;
#29619=EDGE_CURVE ( 'NONE', #34569, #4804, #14863, .T. ) ;
#29620=LINE ( 'NONE', #33528, #37971 ) ;
#29621=ORIENTED_EDGE ( 'NONE', *, *, #31798, .T. ) ;
#29624=VERTEX_POINT ( 'NONE', #22022 ) ;
#29626=CARTESIAN_POINT ( 'NONE',  ( -15.02898246956647910, -5.450173255943768780, 54.50428052266513390 ) ) ;
#29627=ORIENTED_EDGE ( 'NONE', *, *, #27266, .F. ) ;
#29628=CARTESIAN_POINT ( 'NONE',  ( -17.84735443592641602, -7.371153788697909270, 60.19565345827741965 ) ) ;
#29632=VERTEX_POINT ( 'NONE', #7002 ) ;
#29633=LINE ( 'NONE', #14820, #12053 ) ;
#29634=CARTESIAN_POINT ( 'NONE',  ( -15.87557863975121641, -7.931372594209569193, 67.14007279017359053 ) ) ;
#29635=B_SPLINE_CURVE_WITH_KNOTS ( 'NONE', 3,
 ( #21260, #2543, #17544, #13834, #28876, #43921, #48555, #33509, #3495, #18507 ),
 .UNSPECIFIED., .F., .F.,
 ( 4, 2, 2, 2, 4 ),
 ( 0.000000000000000000, 0.2500000000000000000, 0.5000000000000000000, 0.7500000000000000000, 1.000000000000000000 ),
 .UNSPECIFIED. ) ;
#29636=B_SPLINE_CURVE_WITH_KNOTS ( 'NONE', 3,
 ( #15503, #41636, #8159, #1001, #4446, #19719, #4217, #11110, #26132, #38163 ),
 .UNSPECIFIED., .F., .F.,
 ( 4, 2, 2, 2, 4 ),
 ( 0.000000000000000000, 0.2500000000000000000, 0.5000000000000000000, 0.7500000000000000000, 1.000000000000000000 ),
 .UNSPECIFIED. ) ;
#29637=CARTESIAN_POINT ( 'NONE',  ( -11.90659230680199165, -10.41482083560927485, 74.53065494142421699 ) ) ;
#29638=DIRECTION ( 'NONE',  ( -5.731567514496413899E-31, -1.020425574103664789E-16, -1.000000000000000000 ) ) ;
#29640=CARTESIAN_POINT ( 'NONE',  ( -10.67448150008226904, -11.65383075329928886, 74.74495363721690921 ) ) ;
#29642=CARTESIAN_POINT ( 'NONE',  ( -14.05371385056185574, -21.00138210837564401, 72.07607703579976999 ) ) ;
#29646=FACE_OUTER_BOUND ( 'NONE', #15304, .T. ) ;
#29647=ORIENTED_EDGE ( 'NONE', *, *, #19074, .F. ) ;
#29648=CARTESIAN_POINT ( 'NONE',  ( -24.31477923169101629, -16.30090137217950996, 59.40860294853779777 ) ) ;
#29649=VERTEX_POINT ( 'NONE', #25710 ) ;
#29652=CARTESIAN_POINT ( 'NONE',  ( -21.65914559189701194, -18.31838547852702703, 53.49899999999994549 ) ) ;
#29653=CARTESIAN_POINT ( 'NONE',  ( -24.34138250757121469, -16.17068267630804357, 62.89328676667766871 ) ) ;
#29654=ORIENTED_EDGE ( 'NONE', *, *, #7330, .T. ) ;
#29655=CARTESIAN_POINT ( 'NONE',  ( -10.05508844999486939, -15.90482974550872974, 64.70760360623624763 ) ) ;
#29656=CYLINDRICAL_SURFACE ( 'NONE', #18853, 0.1500000000000020484 ) ;
#29657=ADVANCED_FACE ( 'NONE', ( #44686 ), #45413, .T. ) ;
#29658=EDGE_CURVE ( 'NONE', #17650, #45493, #38963, .T. ) ;
#29660=ORIENTED_EDGE ( 'NONE', *, *, #2796, .F. ) ;
#29662=DIRECTION ( 'NONE',  ( 0.7029450532227031756, 0.7112441579020041260, -7.405715380709556396E-09 ) ) ;
#29663=CARTESIAN_POINT ( 'NONE',  ( -13.76436681951595098, -7.422085961289871747, 53.49999999999995026 ) ) ;
#29666=ORIENTED_EDGE ( 'NONE', *, *, #4670, .F. ) ;
#29667=EDGE_LOOP ( 'NONE', ( #22132, #22894, #3703, #35617, #26136 ) ) ;
#29669=EDGE_CURVE ( 'NONE', #34964, #4399, #46136, .T. ) ;
#29674=B_SPLINE_CURVE_WITH_KNOTS ( 'NONE', 3,
 ( #3877, #41788, #11744, #30470, #45487, #29722, #41287, #34371, #37329, #7571 ),
 .UNSPECIFIED., .F., .F.,
 ( 4, 2, 2, 2, 4 ),
 ( 0.000000000000000000, 0.2500000000000000000, 0.5000000000000000000, 0.7500000000000000000, 1.000000000000000000 ),
 .UNSPECIFIED. ) ;
#29675=B_SPLINE_CURVE_WITH_KNOTS ( 'NONE', 3,
 ( #45910, #8242, #27425, #1081, #8731, #43922, #20769, #21262, #28156, #20538 ),
 .UNSPECIFIED., .F., .F.,
 ( 4, 2, 2, 2, 4 ),
 ( 0.1272669073657700656, 0.2522669073462741052, 0.3772669073267782003, 0.5022669073072822954, 0.6272669072877863350 ),
 .UNSPECIFIED. ) ;
#29677=ORIENTED_EDGE ( 'NONE', *, *, #47039, .T. ) ;
#29681=CARTESIAN_POINT ( 'NONE',  ( -11.21783104652298846, -18.93062367394879431, 64.93202350587574756 ) ) ;
#29684=VERTEX_POINT ( 'NONE', #22264 ) ;
#29685=CARTESIAN_POINT ( 'NONE',  ( -22.66103498339474953, -20.10797505100955718, 69.32417989821951210 ) ) ;
#29686=CARTESIAN_POINT ( 'NONE',  ( -19.45790305330666925, -21.50891704259349169, 65.65413287592375013 ) ) ;
#29687=CARTESIAN_POINT ( 'NONE',  ( -11.03557423443333008, -17.80950410671109196, 68.25289248663547426 ) ) ;
#29688=CARTESIAN_POINT ( 'NONE',  ( -20.84119928492007645, -20.97572016636869918, 62.41471400470057773 ) ) ;
#29690=CARTESIAN_POINT ( 'NONE',  ( -11.09534973027204074, -10.87830236297815745, 57.36936532087455021 ) ) ;
#29693=CARTESIAN_POINT ( 'NONE',  ( -22.63560516303400050, -20.13310814558360917, 69.28922553891734992 ) ) ;
#29695=CARTESIAN_POINT ( 'NONE',  ( -22.68321696279682342, -10.11402890775583074, 70.01178527271520124 ) ) ;
#29696=FACE_OUTER_BOUND ( 'NONE', #34304, .T. ) ;
#29700=ORIENTED_EDGE ( 'NONE', *, *, #30628, .F. ) ;
#29701=CARTESIAN_POINT ( 'NONE',  ( -21.37101582717423298, -20.65516655669274826, 69.26269923806351869 ) ) ;
#29702=CARTESIAN_POINT ( 'NONE',  ( -24.38756562526642213, -15.91227465074931935, 66.34852784166324113 ) ) ;
#29703=CARTESIAN_POINT ( 'NONE',  ( -18.72680718162379065, -7.880610904852765053, 70.67068030199192208 ) ) ;
#29704=VECTOR ( 'NONE', #34530, 1000.000000000000114 ) ;
#29706=EDGE_LOOP ( 'NONE', ( #16971, #13907, #4363, #42852, #3243 ) ) ;
#29707=CARTESIAN_POINT ( 'NONE',  ( -14.27672825910291365, -8.496605361553417168, 74.49954621647665931 ) ) ;
#29708=VERTEX_POINT ( 'NONE', #33074 ) ;
#29709=( BOUNDED_SURFACE ( )  B_SPLINE_SURFACE ( 3, 1, ( 
 ( #39893, #11808 ),
 ( #723, #45795 ),
 ( #27454, #11318 ),
 ( #38364, #34686 ),
 ( #4657, #15227 ),
 ( #34191, #33956 ),
 ( #22642, #7882 ) ),
 .UNSPECIFIED., .T., .F., .F. ) 
 B_SPLINE_SURFACE_WITH_KNOTS ( ( 4, 3, 4 ),
 ( 2, 2 ),
 ( 0.000000000000000000, 0.5000000000000000000, 1.000000000000000000 ),
 ( 0.000000000000000000, 1.000000000000000000 ),
 .UNSPECIFIED. ) 
 GEOMETRIC_REPRESENTATION_ITEM ( )  RATIONAL_B_SPLINE_SURFACE ( (
 ( 1.000000000000000000, 1.000000000000000000),
 ( 0.3333333333333335369, 0.3333333333333330373),
 ( 0.3333333333333335369, 0.3333333333333330373),
 ( 1.000000000000000000, 1.000000000000000000),
 ( 0.3333333333333333703, 0.3333333333333333703),
 ( 0.3333333333333333703, 0.3333333333333333703),
 ( 1.000000000000000000, 1.000000000000000000) ) ) 
 REPRESENTATION_ITEM ( '' )  SURFACE ( )  );
#29710=CARTESIAN_POINT ( 'NONE',  ( -12.68532267716109985, -9.060482739934947460, 71.03420753023118550 ) ) ;
#29711=CARTESIAN_POINT ( 'NONE',  ( -20.72450927900464634, -21.03929139025762751, 58.93003081252663833 ) ) ;
#29712=ORIENTED_EDGE ( 'NONE', *, *, #26217, .T. ) ;
#29713=AXIS2_PLACEMENT_3D ( 'NONE', #42090, #254, #38133 ) ;
#29718=ORIENTED_EDGE ( 'NONE', *, *, #22919, .T. ) ;
#29719=CARTESIAN_POINT ( 'NONE',  ( -15.65720112442257950, -8.035743057838505621, 70.90989791475803372 ) ) ;
#29720=CYLINDRICAL_SURFACE ( 'NONE', #13132, 0.1500000000000056566 ) ;
#29722=CARTESIAN_POINT ( 'NONE',  ( -21.27974070113173255, -20.65163647771647604, 69.24553270363776392 ) ) ;
#29723=DIRECTION ( 'NONE',  ( -0.8651630202045381690, 0.5014907262059381532, 5.433021001366390361E-08 ) ) ;
#29724=( BOUNDED_CURVE ( )  B_SPLINE_CURVE ( 3, ( #15712, #15222, #15462, #34921 ),
 .UNSPECIFIED., .F., .F. ) 
 B_SPLINE_CURVE_WITH_KNOTS ( ( 4, 4 ),
 ( 0.5000000000000000000, 0.9074455897393653991 ),
 .UNSPECIFIED. ) 
 CURVE ( )  GEOMETRIC_REPRESENTATION_ITEM ( )  RATIONAL_B_SPLINE_CURVE ( ( 1.000000000000008660, 0.4567392136813321346, 0.3561768502900242162, 0.6983129098260942857 ) ) 
 REPRESENTATION_ITEM ( '' )  );
#29725=CARTESIAN_POINT ( 'NONE',  ( -13.22529448846758982, -9.145569705956512863, 64.19474388871357462 ) ) ;
#29726=FACE_OUTER_BOUND ( 'NONE', #16559, .T. ) ;
#29731=EDGE_CURVE ( 'NONE', #45314, #33165, #17199, .T. ) ;
#29733=CARTESIAN_POINT ( 'NONE',  ( -12.13084389729548640, -10.22855792347674786, 64.04416791493218852 ) ) ;
#29735=CARTESIAN_POINT ( 'NONE',  ( -21.36489355414517632, -8.963473290115421932, 73.90128753234840531 ) ) ;
#29737=CARTESIAN_POINT ( 'NONE',  ( -10.97013630564127773, -17.52378418614773281, 71.67791182052884835 ) ) ;
#29738=CARTESIAN_POINT ( 'NONE',  ( -15.15660932275500272, -21.48492473237050859, 65.39124617759186719 ) ) ;
#29739=ADVANCED_FACE ( 'NONE', ( #12636 ), #23490, .T. ) ;
#29740=VERTEX_POINT ( 'NONE', #12872 ) ;
#29742=( BOUNDED_CURVE ( )  B_SPLINE_CURVE ( 3, ( #14094, #47623, #43697, #13854 ),
 .UNSPECIFIED., .F., .F. ) 
 B_SPLINE_CURVE_WITH_KNOTS ( ( 4, 4 ),
 ( 0.000000000000000000, 0.4074455897393665649 ),
 .UNSPECIFIED. ) 
 CURVE ( )  GEOMETRIC_REPRESENTATION_ITEM ( )  RATIONAL_B_SPLINE_CURVE ( ( 1.000000000000000000, 0.4567392136813314685, 0.3561768502900301003, 0.6983129098260959511 ) ) 
 REPRESENTATION_ITEM ( '' )  );
#29743=ORIENTED_EDGE ( 'NONE', *, *, #43174, .T. ) ;
#29745=ADVANCED_FACE ( 'NONE', ( #5020 ), #5253, .T. ) ;
#29749=VERTEX_POINT ( 'NONE', #23976 ) ;
#29750=CARTESIAN_POINT ( 'NONE',  ( -22.50276953350645925, -9.919252841961412770, 73.77601325438966740 ) ) ;
#29751=VECTOR ( 'NONE', #27649, 1000.000000000000000 ) ;
#29753=FACE_OUTER_BOUND ( 'NONE', #40506, .T. ) ;
#29754=CARTESIAN_POINT ( 'NONE',  ( -27.41460927708051898, -13.34199974102237896, 54.54971261817296835 ) ) ;
#29757=CYLINDRICAL_SURFACE ( 'NONE', #39125, 0.1500000000000022427 ) ;
#29760=CARTESIAN_POINT ( 'NONE',  ( -24.67963342063540466, -16.50099095021179352, 59.28478976814308510 ) ) ;
#29763=CARTESIAN_POINT ( 'NONE',  ( -17.59145722722324479, -7.361077857161463456, 63.75045814445680037 ) ) ;
#29766=CARTESIAN_POINT ( 'NONE',  ( -16.52316554273587101, -21.80170452179945073, 65.24036514508233608 ) ) ;
#29768=CARTESIAN_POINT ( 'NONE',  ( -21.44204676556661582, -20.54122665395610525, 72.71549499130021843 ) ) ;
#29770=CARTESIAN_POINT ( 'NONE',  ( -11.10470791607724550, -18.75498134223953883, 61.46206221440264983 ) ) ;
#29772=B_SPLINE_CURVE_WITH_KNOTS ( 'NONE', 3,
 ( #36690, #29340, #33246, #48286, #14517, #29580, #7192, #18482, #33487, #14766 ),
 .UNSPECIFIED., .F., .F.,
 ( 4, 2, 2, 2, 4 ),
 ( 0.1272669073658055372, 0.2522669073462952549, 0.3772669073267849171, 0.5022669073072746349, 0.6272669072877643526 ),
 .UNSPECIFIED. ) ;
#29773=B_SPLINE_CURVE_WITH_KNOTS ( 'NONE', 1,
 ( #20862, #42792 ),
 .UNSPECIFIED., .F., .F.,
 ( 2, 2 ),
 ( 0.000000000000000000, 1.000000000000000000 ),
 .UNSPECIFIED. ) ;
#29775=CARTESIAN_POINT ( 'NONE',  ( -13.36507556264098717, -20.57353123648257665, 58.04650106771609330 ) ) ;
#29776=CARTESIAN_POINT ( 'NONE',  ( -14.92957361138602579, -21.82925975653312278, 65.22101252026929785 ) ) ;
#29778=EDGE_CURVE ( 'NONE', #27147, #6936, #17492, .T. ) ;
#29780=ORIENTED_EDGE ( 'NONE', *, *, #32346, .F. ) ;
#29781=DIRECTION ( 'NONE',  ( 0.9926276493613465091, 0.06323820549166281335, 0.1033986416233891870 ) ) ;
#29782=CARTESIAN_POINT ( 'NONE',  ( -16.96571475693685116, -7.824107681210383802, 74.26018256191720468 ) ) ;
#29783=VECTOR ( 'NONE', #20743, 1000.000000000000227 ) ;
#29786=CARTESIAN_POINT ( 'NONE',  ( -23.30132152709437676, -10.22970227413176580, 63.25841351925517841 ) ) ;
#29787=CARTESIAN_POINT ( 'NONE',  ( -13.17078218117215549, -9.186392337449538203, 67.39414915108072535 ) ) ;
#29788=CARTESIAN_POINT ( 'NONE',  ( -23.98503169607928953, -17.39005800936845603, 66.22885190747201989 ) ) ;
#29791=CARTESIAN_POINT ( 'NONE',  ( -14.62687819956926027, -8.392386103536567887, 64.08978840643771946 ) ) ;
#29792=ORIENTED_EDGE ( 'NONE', *, *, #38290, .F. ) ;
#29793=CARTESIAN_POINT ( 'NONE',  ( -24.12071557656922494, -11.54438865435207795, 63.06722852297808402 ) ) ;
#29795=VECTOR ( 'NONE', #1339, 1000.000000000000114 ) ;
#29798=EDGE_CURVE ( 'NONE', #37103, #9885, #31112, .T. ) ;
#29799=EDGE_LOOP ( 'NONE', ( #10851, #16520, #12465, #6381, #22877 ) ) ;
#29804=CARTESIAN_POINT ( 'NONE',  ( -11.72771377538897042, -10.00769167454747688, 67.60622713944691498 ) ) ;
#29805=CARTESIAN_POINT ( 'NONE',  ( -10.18203091723714770, -13.06113264623505721, 71.40166907525704687 ) ) ;
#29808=CARTESIAN_POINT ( 'NONE',  ( -24.50475423537784536, -17.33693471837318612, 54.02312124697527906 ) ) ;
#29809=DIRECTION ( 'NONE',  ( 0.3163880819683246304, 0.8528035521334702551, 0.4154812667942326954 ) ) ;
#29810=VERTEX_POINT ( 'NONE', #23743 ) ;
#29811=CARTESIAN_POINT ( 'NONE',  ( -22.33161753753789469, -20.41455022152800325, 62.49085083065315160 ) ) ;
#29813=( BOUNDED_SURFACE ( )  B_SPLINE_SURFACE ( 3, 1, ( 
 ( #25031, #36094 ),
 ( #2618, #24564 ),
 ( #24315, #25277 ),
 ( #28489, #28245 ),
 ( #43014, #40051 ),
 ( #40293, #47676 ),
 ( #28958, #20850 ) ),
 .UNSPECIFIED., .T., .F., .F. ) 
 B_SPLINE_SURFACE_WITH_KNOTS ( ( 4, 3, 4 ),
 ( 2, 2 ),
 ( 0.000000000000000000, 0.5000000000000000000, 1.000000000000000000 ),
 ( 0.000000000000000000, 1.000000000000000000 ),
 .UNSPECIFIED. ) 
 GEOMETRIC_REPRESENTATION_ITEM ( )  RATIONAL_B_SPLINE_SURFACE ( (
 ( 1.000000000000000000, 1.000000000000000000),
 ( 0.3333333333333335369, 0.3333333333333330373),
 ( 0.3333333333333335369, 0.3333333333333330373),
 ( 1.000000000000000000, 1.000000000000000000),
 ( 0.3333333333333333703, 0.3333333333333333703),
 ( 0.3333333333333333703, 0.3333333333333333703),
 ( 1.000000000000000000, 1.000000000000000000) ) ) 
 REPRESENTATION_ITEM ( '' )  SURFACE ( )  );
#29816=CARTESIAN_POINT ( 'NONE',  ( -10.85423598487861874, -17.22645666615770921, 64.91122787125294735 ) ) ;
#29817=ORIENTED_EDGE ( 'NONE', *, *, #37788, .F. ) ;
#29821=CARTESIAN_POINT ( 'NONE',  ( -19.49109506855409180, -21.54969648977046148, 62.28031529404344013 ) ) ;
#29822=CARTESIAN_POINT ( 'NONE',  ( -24.39570712928462370, -14.17877393659436080, 69.66777723616006313 ) ) ;
#29823=ORIENTED_EDGE ( 'NONE', *, *, #18187, .F. ) ;
#29825=CYLINDRICAL_SURFACE ( 'NONE', #36741, 0.1499999999999973577 ) ;
#29827=CARTESIAN_POINT ( 'NONE',  ( -16.16748626245079379, -22.20318634978239203, 53.49999999999994316 ) ) ;
#29829=EDGE_CURVE ( 'NONE', #45965, #16929, #44551, .T. ) ;
#29832=CYLINDRICAL_SURFACE ( 'NONE', #13232, 0.1500000000000061007 ) ;
#29833=ORIENTED_EDGE ( 'NONE', *, *, #16982, .F. ) ;
#29834=CARTESIAN_POINT ( 'NONE',  ( -16.91855014848012928, -22.24212009645463439, 72.28047803099305213 ) ) ;
#29836=CARTESIAN_POINT ( 'NONE',  ( -22.75923595801102550, -10.27751167601812909, 66.54182257657851096 ) ) ;
#29838=CARTESIAN_POINT ( 'NONE',  ( -10.78527719640413451, -12.58937423537859424, 60.79853578751971099 ) ) ;
#29839=CARTESIAN_POINT ( 'NONE',  ( -23.80628931054383202, -18.65249568317075202, 72.95642365399113771 ) ) ;
#29840=ORIENTED_EDGE ( 'NONE', *, *, #43642, .T. ) ;
#29843=CARTESIAN_POINT ( 'NONE',  ( -14.95042968149815188, -8.260718009457519884, 56.84999999999994458 ) ) ;
#29845=CARTESIAN_POINT ( 'NONE',  ( -23.68653687815194786, -11.57061008776567945, 66.43686604568146947 ) ) ;
#29846=LINE ( 'NONE', #26384, #9203 ) ;
#29847=CARTESIAN_POINT ( 'NONE',  ( -24.21255584207132827, -13.09477218448524027, 66.41319906622749158 ) ) ;
#29848=CARTESIAN_POINT ( 'NONE',  ( -20.70278685264619867, -8.119407593049823291, 63.41783206474445223 ) ) ;
#29849=DIRECTION ( 'NONE',  ( -5.731567514496413899E-31, -1.020425574103664789E-16, -1.000000000000000000 ) ) ;
#29850=CARTESIAN_POINT ( 'NONE',  ( -24.27661814142333796, -16.49973396376381984, 62.73761853866894711 ) ) ;
#29851=CARTESIAN_POINT ( 'NONE',  ( -11.45752044641470668, -19.27057170535650954, 71.87181270239314301 ) ) ;
#29853=B_SPLINE_CURVE_WITH_KNOTS ( 'NONE', 3,
 ( #20347, #20595, #31910, #24289, #35356, #35104, #1869, #16392, #8794, #46927 ),
 .UNSPECIFIED., .F., .F.,
 ( 4, 2, 2, 2, 4 ),
 ( 0.000000000000000000, 0.2500000000000000000, 0.5000000000000000000, 0.7500000000000000000, 1.000000000000000000 ),
 .UNSPECIFIED. ) ;
#29855=ORIENTED_EDGE ( 'NONE', *, *, #30870, .F. ) ;
#29856=CARTESIAN_POINT ( 'NONE',  ( -21.68499601416157674, -9.192516039336663169, 66.66149992327366647 ) ) ;
#29857=EDGE_CURVE ( 'NONE', #47871, #39323, #4294, .T. ) ;
#29859=CARTESIAN_POINT ( 'NONE',  ( -12.11599782822167271, -20.03693337884723391, 61.55712024599606025 ) ) ;
#29861=CARTESIAN_POINT ( 'NONE',  ( -24.23813412381375088, -12.99935709875259704, 66.31718868320673721 ) ) ;
#29862=CARTESIAN_POINT ( 'NONE',  ( -20.75918756122348441, -8.147305293919229641, 63.42626095967343502 ) ) ;
#29866=EDGE_CURVE ( 'NONE', #28685, #5757, #24298, .T. ) ;
#29867=ORIENTED_EDGE ( 'NONE', *, *, #466, .F. ) ;
#29868=CARTESIAN_POINT ( 'NONE',  ( -17.11743416019711361, -21.80254600073977045, 72.23831284135304998 ) ) ;
#29871=ADVANCED_FACE ( 'NONE', ( #46627 ), #34300, .T. ) ;
#29872=( BOUNDED_SURFACE ( )  B_SPLINE_SURFACE ( 3, 1, ( 
 ( #9884, #36925 ),
 ( #17727, #40394 ),
 ( #6183, #18216 ),
 ( #33221, #48260 ),
 ( #14497, #44584 ),
 ( #39914, #36208 ),
 ( #11092, #45321 ) ),
 .UNSPECIFIED., .T., .F., .F. ) 
 B_SPLINE_SURFACE_WITH_KNOTS ( ( 4, 3, 4 ),
 ( 2, 2 ),
 ( 0.000000000000000000, 0.5000000000000000000, 1.000000000000000000 ),
 ( 0.000000000000000000, 1.000000000000000000 ),
 .UNSPECIFIED. ) 
 GEOMETRIC_REPRESENTATION_ITEM ( )  RATIONAL_B_SPLINE_SURFACE ( (
 ( 1.000000000000000000, 1.000000000000000000),
 ( 0.3333333333333335369, 0.3333333333333330373),
 ( 0.3333333333333335369, 0.3333333333333330373),
 ( 1.000000000000000000, 1.000000000000000000),
 ( 0.3333333333333333703, 0.3333333333333333703),
 ( 0.3333333333333333703, 0.3333333333333333703),
 ( 1.000000000000000000, 1.000000000000000000) ) ) 
 REPRESENTATION_ITEM ( '' )  SURFACE ( )  );
#29873=LINE ( 'NONE', #3277, #13497 ) ;
#29875=EDGE_LOOP ( 'NONE', ( #11987, #9837, #32052, #43821, #21319 ) ) ;
#29876=CARTESIAN_POINT ( 'NONE',  ( -23.07906183844443859, -9.958936969296642516, 66.72677665813928627 ) ) ;
#29878=EDGE_LOOP ( 'NONE', ( #33420, #26312, #28401, #14362, #21487 ) ) ;
#29879=CARTESIAN_POINT ( 'NONE',  ( -17.19811928533322387, -9.313850733363548073, 53.49999999999995026 ) ) ;
#29880=ADVANCED_FACE ( 'NONE', ( #8233 ), #36047, .T. ) ;
#29881=( BOUNDED_CURVE ( )  B_SPLINE_CURVE ( 3, ( #23687, #16979, #23432, #19740 ),
 .UNSPECIFIED., .F., .F. ) 
 B_SPLINE_CURVE_WITH_KNOTS ( ( 4, 4 ),
 ( 0.4074455897393668979, 0.5000000000000000000 ),
 .UNSPECIFIED. ) 
 CURVE ( )  GEOMETRIC_REPRESENTATION_ITEM ( )  RATIONAL_B_SPLINE_CURVE ( ( 0.6983129098261043888, 0.7760317562607172981, 0.8765941196520187217, 1.000000000000014877 ) ) 
 REPRESENTATION_ITEM ( '' )  );
#29883=VERTEX_POINT ( 'NONE', #13820 ) ;
#29884=CARTESIAN_POINT ( 'NONE',  ( -17.95184243766222565, -21.84304804239566522, 58.61373395300507383 ) ) ;
#29885=CARTESIAN_POINT ( 'NONE',  ( -11.10300301615976259, -11.79817525417081292, 74.66913066534023358 ) ) ;
#29886=CARTESIAN_POINT ( 'NONE',  ( -14.42683414290149635, -8.428067600363895906, 67.25975083869262505 ) ) ;
#29887=EDGE_CURVE ( 'NONE', #30487, #39013, #181, .T. ) ;
#29889=FACE_OUTER_BOUND ( 'NONE', #22825, .T. ) ;
#29890=CARTESIAN_POINT ( 'NONE',  ( -11.77326604373719476, -19.03093417793677133, 68.21689334798529103 ) ) ;
#29892=VECTOR ( 'NONE', #24741, 1000.000000000000114 ) ;
#29893=CARTESIAN_POINT ( 'NONE',  ( -15.07489245205697159, -21.40335507889944111, 65.40596683994178306 ) ) ;
#29894=CARTESIAN_POINT ( 'NONE',  ( -10.88286923018596575, -17.43962093083235843, 68.11193994895104709 ) ) ;
#29895=EDGE_LOOP ( 'NONE', ( #41990, #14991, #14648, #22972, #42158 ) ) ;
#29896=CARTESIAN_POINT ( 'NONE',  ( -11.45656716003344933, -19.26928393672501727, 71.73039932227760573 ) ) ;
#29898=AXIS2_PLACEMENT_3D ( 'NONE', #24823, #14185, #44040 ) ;
#29902=ORIENTED_EDGE ( 'NONE', *, *, #19647, .T. ) ;
#29903=CARTESIAN_POINT ( 'NONE',  ( -17.69342360693616456, -22.25450524205111691, 58.54519988936747410 ) ) ;
#29904=CARTESIAN_POINT ( 'NONE',  ( -24.71300512064630794, -13.26796065199660113, 59.61913874400077873 ) ) ;
#29909=ORIENTED_EDGE ( 'NONE', *, *, #2776, .T. ) ;
#29910=DIRECTION ( 'NONE',  ( -0.7700094066334552956, -0.6380325334150243055, -2.326497556385353503E-17 ) ) ;
#29911=CARTESIAN_POINT ( 'NONE',  ( -23.47627603871685409, -18.32658462313428060, 72.99041477383734389 ) ) ;
#29915=CARTESIAN_POINT ( 'NONE',  ( -12.84690951644825851, -8.931012861620404308, 67.56438176077992352 ) ) ;
#29916=DIRECTION ( 'NONE',  ( -2.201155566701781786E-06, -7.355553121729402965E-06, -0.9999999999705254661 ) ) ;
#29918=CARTESIAN_POINT ( 'NONE',  ( -19.37616851487812752, -21.99900361761337919, 58.71002773933979313 ) ) ;
#29919=ORIENTED_EDGE ( 'NONE', *, *, #3322, .F. ) ;
#29920=ORIENTED_EDGE ( 'NONE', *, *, #41515, .F. ) ;
#29922=EDGE_CURVE ( 'NONE', #15790, #34971, #22537, .T. ) ;
#29925=CARTESIAN_POINT ( 'NONE',  ( -23.52949419687348964, -11.28347464189849525, 70.17738639980606763 ) ) ;
#29928=EDGE_LOOP ( 'NONE', ( #34155, #46337, #8111, #45959, #5252 ) ) ;
#29930=CARTESIAN_POINT ( 'NONE',  ( -10.48480550552488744, -16.05393363305330823, 68.27767801788075985 ) ) ;
#29931=AXIS2_PLACEMENT_3D ( 'NONE', #21560, #36312, #44700 ) ;
#29932=CARTESIAN_POINT ( 'NONE',  ( -11.41947236009895228, -18.50911967460687535, 65.16195962094886340 ) ) ;
#29933=ORIENTED_EDGE ( 'NONE', *, *, #34707, .T. ) ;
#29937=B_SPLINE_CURVE_WITH_KNOTS ( 'NONE', 3,
 ( #11426, #7760, #363, #3805, #44692, #30407, #10949, #2643, #41720, #8008 ),
 .UNSPECIFIED., .F., .F.,
 ( 4, 2, 2, 2, 4 ),
 ( 0.6272669072877923302, 0.7522669073072929535, 0.8772669073267936879, 1.002266907346294422, 1.127266907365795046 ),
 .UNSPECIFIED. ) ;
#29938=CYLINDRICAL_SURFACE ( 'NONE', #26060, 0.1499999999999991063 ) ;
#29942=ADVANCED_FACE ( 'NONE', ( #43166 ), #27577, .T. ) ;
#29943=CARTESIAN_POINT ( 'NONE',  ( -9.989595930756898667, -14.32624556671389549, 64.54837224505392612 ) ) ;
#29945=EDGE_LOOP ( 'NONE', ( #38862, #44514, #8683, #29045, #37024 ) ) ;
#29946=CARTESIAN_POINT ( 'NONE',  ( -10.40174226954351866, -17.29724918936392442, 61.34238429002267878 ) ) ;
#29947=CARTESIAN_POINT ( 'NONE',  ( -16.50454536406711981, -22.20232556258728351, 65.34068991928313608 ) ) ;
#29948=DIRECTION ( 'NONE',  ( 0.5088156898428700670, 0.8608754809899751281, 5.922709712265243479E-08 ) ) ;
#29949=CARTESIAN_POINT ( 'NONE',  ( -10.07931644449276476, -16.05763419655898616, 68.15580616013423310 ) ) ;
#29951=CARTESIAN_POINT ( 'NONE',  ( -10.37497031247464463, -14.69804315800203298, 71.62782692816419683 ) ) ;
#29952=CARTESIAN_POINT ( 'NONE',  ( -17.15992076746773876, -7.363842158706400021, 70.59697549560173968 ) ) ;
#29953=CARTESIAN_POINT ( 'NONE',  ( -18.76558392140857023, -7.480892851696864021, 70.55563303198719893 ) ) ;
#29954=FACE_BOUND ( 'NONE', #30978, .T. ) ;
#29956=CARTESIAN_POINT ( 'NONE',  ( -13.11455056595802660, -20.88644485624005398, 58.20796624012236720 ) ) ;
#29957=CARTESIAN_POINT ( 'NONE',  ( -10.53944148391707891, -16.08179225747893071, 71.67580357262283997 ) ) ;
#29958=CARTESIAN_POINT ( 'NONE',  ( -16.09584876169039802, -7.477806291315723719, 63.85666425603482566 ) ) ;
#29959=ORIENTED_EDGE ( 'NONE', *, *, #42149, .F. ) ;
#29962=DIRECTION ( 'NONE',  ( -0.9529680021988312655, 0.3030709269876716294, 3.918663088761644638E-08 ) ) ;
#29964=CARTESIAN_POINT ( 'NONE',  ( -14.07539642552819359, -8.605278304397881328, 74.19954655214911554 ) ) ;
#29965=EDGE_LOOP ( 'NONE', ( #19115, #35092 ) ) ;
#29966=FACE_OUTER_BOUND ( 'NONE', #26789, .T. ) ;
#29968=CARTESIAN_POINT ( 'NONE',  ( -11.00648394673626562, -17.60476015118163673, 68.17010079748926898 ) ) ;
#29970=EDGE_CURVE ( 'NONE', #9317, #41086, #24703, .T. ) ;
#29972=ORIENTED_EDGE ( 'NONE', *, *, #24708, .T. ) ;
#29973=CARTESIAN_POINT ( 'NONE',  ( -15.79261328423922706, -21.67602794760135154, 72.20142491214876657 ) ) ;
#29974=CARTESIAN_POINT ( 'NONE',  ( -22.34470957656571599, -19.78791530553215949, 69.47417989488683077 ) ) ;
#29976=CARTESIAN_POINT ( 'NONE',  ( -12.45502217426375680, -20.36096218193827667, 71.99308960123012469 ) ) ;
#29977=CARTESIAN_POINT ( 'NONE',  ( -10.57110082969170683, -13.38215148069720861, 74.67817647591368768 ) ) ;
#29978=CARTESIAN_POINT ( 'NONE',  ( -10.40174263535760524, -17.29725023780839166, 61.34238537770443855 ) ) ;
#29980=CARTESIAN_POINT ( 'NONE',  ( -10.39241571269986331, -17.41794234916963191, 54.27966884056652219 ) ) ;
#29981=VERTEX_POINT ( 'NONE', #39470 ) ;
#29982=ORIENTED_EDGE ( 'NONE', *, *, #25791, .T. ) ;
#29983=CARTESIAN_POINT ( 'NONE',  ( -16.46477641927899782, -7.821750181629138154, 60.61517342399707076 ) ) ;
#29984=VECTOR ( 'NONE', #10011, 1000.000000000000000 ) ;
#29985=ADVANCED_FACE ( 'NONE', ( #5752 ), #20755, .T. ) ;
#29986=PLANE ( 'NONE',  #30718 ) ;
#29987=CARTESIAN_POINT ( 'NONE',  ( -11.89178972046640936, -10.43929686452144878, 71.11893105542935700 ) ) ;
#29988=CYLINDRICAL_SURFACE ( 'NONE', #33871, 0.1500000000000028255 ) ;
#29989=ORIENTED_EDGE ( 'NONE', *, *, #38306, .T. ) ;
#29991=ORIENTED_EDGE ( 'NONE', *, *, #38582, .T. ) ;
#29994=CARTESIAN_POINT ( 'NONE',  ( -11.96073139429061527, -19.87431630704028152, 57.97036459255868124 ) ) ;
#29997=ORIENTED_EDGE ( 'NONE', *, *, #36988, .T. ) ;
#29999=AXIS2_PLACEMENT_3D ( 'NONE', #7907, #5834, #13186 ) ;
#30000=CYLINDRICAL_SURFACE ( 'NONE', #18049, 0.1500000000000061007 ) ;
#30001=CARTESIAN_POINT ( 'NONE',  ( -14.80624607021532135, -8.317144234858641738, 60.31996281969095719 ) ) ;
#30002=ADVANCED_FACE ( 'NONE', ( #18841 ), #33206, .T. ) ;
#30006=( BOUNDED_CURVE ( )  B_SPLINE_CURVE ( 3, ( #37760, #34065, #356, #22025 ),
 .UNSPECIFIED., .F., .F. ) 
 B_SPLINE_CURVE_WITH_KNOTS ( ( 4, 4 ),
 ( 0.5000000000000000000, 0.9074455897393618464 ),
 .UNSPECIFIED. ) 
 CURVE ( )  GEOMETRIC_REPRESENTATION_ITEM ( )  RATIONAL_B_SPLINE_CURVE ( ( 1.000000000000016653, 0.4567392136813336334, 0.3561768502900192201, 0.6983129098260912881 ) ) 
 REPRESENTATION_ITEM ( '' )  );
#30007=CARTESIAN_POINT ( 'NONE',  ( -10.05862335131466700, -15.92885902279982524, 64.69266873560974318 ) ) ;
#30008=CARTESIAN_POINT ( 'NONE',  ( -24.03783269458455862, -17.25936868619852760, 65.82868649746481537 ) ) ;
#30010=DIRECTION ( 'NONE',  ( -0.4433615477241707459, 0.8963428685495451465, -2.661652803430156647E-08 ) ) ;
#30012=FACE_OUTER_BOUND ( 'NONE', #36210, .T. ) ;
#30013=EDGE_CURVE ( 'NONE', #45327, #28927, #8413, .T. ) ;
#30015=CARTESIAN_POINT ( 'NONE',  ( -24.87290000513101873, -14.67112934921935974, 62.82801050733710468 ) ) ;
#30016=VERTEX_POINT ( 'NONE', #14982 ) ;
#30017=CARTESIAN_POINT ( 'NONE',  ( -22.09234465700630423, -20.09219189623108548, 62.23439162498055310 ) ) ;
#30019=EDGE_CURVE ( 'NONE', #44359, #45444, #34823, .T. ) ;
#30020=CARTESIAN_POINT ( 'NONE',  ( -20.60788153932096023, -8.518722016582882972, 63.32593600985608617 ) ) ;
#30021=ORIENTED_EDGE ( 'NONE', *, *, #3076, .T. ) ;
#30022=CARTESIAN_POINT ( 'NONE',  ( -14.62687819956926027, -8.392386103536567887, 64.08978840643771946 ) ) ;
#30023=ADVANCED_FACE ( 'NONE', ( #29298 ), #25595, .T. ) ;
#30024=DIRECTION ( 'NONE',  ( 0.7111926860893301727, -0.6953514824629924984, 0.1033986416233890065 ) ) ;
#30025=( BOUNDED_CURVE ( )  B_SPLINE_CURVE ( 3, ( #38976, #6467, #20520, #42922 ),
 .UNSPECIFIED., .F., .F. ) 
 B_SPLINE_CURVE_WITH_KNOTS ( ( 4, 4 ),
 ( 0.5000000000000000000, 0.9074455897393682857 ),
 .UNSPECIFIED. ) 
 CURVE ( )  GEOMETRIC_REPRESENTATION_ITEM ( )  RATIONAL_B_SPLINE_CURVE ( ( 0.9999999999999892308, 0.4567392136813265835, 0.3561768502900357625, 0.6983129098261049439 ) ) 
 REPRESENTATION_ITEM ( '' )  );
#30027=ORIENTED_EDGE ( 'NONE', *, *, #1216, .T. ) ;
#30028=( BOUNDED_SURFACE ( )  B_SPLINE_SURFACE ( 3, 1, ( 
 ( #27319, #5165 ),
 ( #27568, #42607 ),
 ( #4675, #9105 ),
 ( #42349, #23647 ),
 ( #38645, #19940 ),
 ( #46288, #20173 ),
 ( #1454, #23388 ) ),
 .UNSPECIFIED., .T., .F., .F. ) 
 B_SPLINE_SURFACE_WITH_KNOTS ( ( 4, 3, 4 ),
 ( 2, 2 ),
 ( 0.000000000000000000, 0.5000000000000000000, 1.000000000000000000 ),
 ( 0.000000000000000000, 1.000000000000000000 ),
 .UNSPECIFIED. ) 
 GEOMETRIC_REPRESENTATION_ITEM ( )  RATIONAL_B_SPLINE_SURFACE ( (
 ( 1.000000000000000000, 1.000000000000000000),
 ( 0.3333333333333335369, 0.3333333333333330373),
 ( 0.3333333333333335369, 0.3333333333333330373),
 ( 1.000000000000000000, 1.000000000000000000),
 ( 0.3333333333333333703, 0.3333333333333333703),
 ( 0.3333333333333333703, 0.3333333333333333703),
 ( 1.000000000000000000, 1.000000000000000000) ) ) 
 REPRESENTATION_ITEM ( '' )  SURFACE ( )  );
#30029=CARTESIAN_POINT ( 'NONE',  ( -12.15399223456666178, -9.543296633619027247, 57.20440205305690995 ) ) ;
#30030=B_SPLINE_CURVE_WITH_KNOTS ( 'NONE', 3,
 ( #32008, #39146, #43591, #39398, #31277, #28562, #16964, #43089, #9369, #28325 ),
 .UNSPECIFIED., .F., .F.,
 ( 4, 2, 2, 2, 4 ),
 ( 0.000000000000000000, 0.2500000000000000000, 0.5000000000000000000, 0.7500000000000000000, 1.000000000000000000 ),
 .UNSPECIFIED. ) ;
#30031=CARTESIAN_POINT ( 'NONE',  ( -13.33151401730585306, -20.55006798877650454, 58.06122216312902395 ) ) ;
#30035=ORIENTED_EDGE ( 'NONE', *, *, #2760, .F. ) ;
#30037=AXIS2_PLACEMENT_3D ( 'NONE', #14478, #6649, #2937 ) ;
#30038=CARTESIAN_POINT ( 'NONE',  ( -24.26595340233995302, -13.32969406988797623, 59.36267925071750540 ) ) ;
#30039=CARTESIAN_POINT ( 'NONE',  ( -24.25510706449861686, -16.56479617024167084, 59.53821300994621168 ) ) ;
#30040=FACE_OUTER_BOUND ( 'NONE', #41546, .T. ) ;
#30043=FACE_OUTER_BOUND ( 'NONE', #24566, .T. ) ;
#30044=CARTESIAN_POINT ( 'NONE',  ( -12.15935936027619668, -9.537873432754242486, 57.21218613097342143 ) ) ;
#30045=FACE_OUTER_BOUND ( 'NONE', #38173, .T. ) ;
#30046=( BOUNDED_CURVE ( )  B_SPLINE_CURVE ( 3, ( #26491, #41025, #7798, #22815 ),
 .UNSPECIFIED., .F., .F. ) 
 B_SPLINE_CURVE_WITH_KNOTS ( ( 4, 4 ),
 ( 0.5000000000000000000, 0.9074455897393733927 ),
 .UNSPECIFIED. ) 
 CURVE ( )  GEOMETRIC_REPRESENTATION_ITEM ( )  RATIONAL_B_SPLINE_CURVE ( ( 0.9999999999999990008, 0.4567392136813159809, 0.3561768502900249933, 0.6983129098261249279 ) ) 
 REPRESENTATION_ITEM ( '' )  );
#30047=CARTESIAN_POINT ( 'NONE',  ( -16.50454536406711981, -22.20232556258728351, 65.34068991928313608 ) ) ;
#30048=ORIENTED_EDGE ( 'NONE', *, *, #28979, .T. ) ;
#30050=B_SPLINE_CURVE_WITH_KNOTS ( 'NONE', 1,
 ( #29253, #10540 ),
 .UNSPECIFIED., .F., .F.,
 ( 2, 2 ),
 ( 0.000000000000000000, 1.000000000000000000 ),
 .UNSPECIFIED. ) ;
#30052=CARTESIAN_POINT ( 'NONE',  ( -19.92776479198160189, -21.39998277484045275, 72.41950795000725805 ) ) ;
#30054=EDGE_LOOP ( 'NONE', ( #14587, #9740, #46539, #511, #46685 ) ) ;
#30055=EDGE_LOOP ( 'NONE', ( #9976, #1901, #5168, #4101, #5051 ) ) ;
#30056=CARTESIAN_POINT ( 'NONE',  ( -17.70250950100762566, -21.85374724789173584, 58.40553377166283866 ) ) ;
#30058=CARTESIAN_POINT ( 'NONE',  ( -22.06352460594304787, -8.980016202103444201, 63.37649054182217867 ) ) ;
#30059=PLANE ( 'NONE',  #22513 ) ;
#30060=EDGE_CURVE ( 'NONE', #43790, #35496, #25997, .T. ) ;
#30061=ORIENTED_EDGE ( 'NONE', *, *, #38030, .T. ) ;
#30062=CARTESIAN_POINT ( 'NONE',  ( -22.72031779163844689, -16.29245029320677673, 53.49999999999995026 ) ) ;
#30063=CARTESIAN_POINT ( 'NONE',  ( -23.00441852451001523, -19.11762575345012749, 58.88410642058938294 ) ) ;
#30066=AXIS2_PLACEMENT_3D ( 'NONE', #37773, #30170, #3316 ) ;
#30069=CARTESIAN_POINT ( 'NONE',  ( -10.83447761903821061, -17.17455418348055218, 64.69909585894313864 ) ) ;
#30070=ORIENTED_EDGE ( 'NONE', *, *, #6068, .T. ) ;
#30071=CARTESIAN_POINT ( 'NONE',  ( -21.71715435735689326, -9.279671086701025473, 66.94533469040406715 ) ) ;
#30073=CARTESIAN_POINT ( 'NONE',  ( -19.57546054543010783, -21.94189796748987575, 62.03857704761023939 ) ) ;
#30077=CARTESIAN_POINT ( 'NONE',  ( -10.29385348138020539, -12.64970417265235803, 64.38340698725603772 ) ) ;
#30080=CARTESIAN_POINT ( 'NONE',  ( -10.70532053225239366, -12.67267096592666675, 61.08381491717225487 ) ) ;
#30081=EDGE_CURVE ( 'NONE', #35856, #508, #47707, .T. ) ;
#30082=CARTESIAN_POINT ( 'NONE',  ( -23.96654618570108042, -17.44381333609114648, 62.35872369075587329 ) ) ;
#30083=DIRECTION ( 'NONE',  ( 6.312331213287273068E-07, 6.220915576652692866E-06, 0.9999999999804508599 ) ) ;
#30084=CARTESIAN_POINT ( 'NONE',  ( -17.20472057461396176, -21.85940646863547343, 72.37363138342533375 ) ) ;
#30085=ORIENTED_EDGE ( 'NONE', *, *, #24068, .T. ) ;
#30086=CARTESIAN_POINT ( 'NONE',  ( -10.43291801062321866, -14.45783718407127694, 64.49689883712670735 ) ) ;
#30089=CARTESIAN_POINT ( 'NONE',  ( -12.54046192938994153, -19.89396152535205076, 65.16115129690373919 ) ) ;
#30090=CYLINDRICAL_SURFACE ( 'NONE', #27460, 2.500000000000001332 ) ;
#30091=CARTESIAN_POINT ( 'NONE',  ( -24.18432332345330948, -12.99280965528459930, 63.02367257271272649 ) ) ;
#30093=ORIENTED_EDGE ( 'NONE', *, *, #35779, .F. ) ;
#30094=CARTESIAN_POINT ( 'NONE',  ( -23.62594491300536959, -11.45603751788689095, 66.70742424642772050 ) ) ;
#30095=CARTESIAN_POINT ( 'NONE',  ( -10.47550909334574598, -13.59594187864236581, 74.67817481325579365 ) ) ;
#30096=ORIENTED_EDGE ( 'NONE', *, *, #5872, .T. ) ;
#30097=CARTESIAN_POINT ( 'NONE',  ( -24.03794070092309454, -17.10236419872843783, 73.18336037747248213 ) ) ;
#30098=CARTESIAN_POINT ( 'NONE',  ( -24.20826260513847217, -13.07918714609906452, 66.37417080772955558 ) ) ;
#30099=CARTESIAN_POINT ( 'NONE',  ( -12.50376665500426654, -9.829597046481099554, 57.10552118696781321 ) ) ;
#30100=DIRECTION ( 'NONE',  ( -0.5729733056696844073, 0.8195740302071247152, 7.403245352187747277E-08 ) ) ;
#30101=EDGE_CURVE ( 'NONE', #33816, #46437, #42589, .T. ) ;
#30102=CARTESIAN_POINT ( 'NONE',  ( -23.38410589725464916, -10.33907962427212190, 59.71708035543083071 ) ) ;
#30104=CARTESIAN_POINT ( 'NONE',  ( -14.06267692155865312, -8.668962760654556732, 74.49954661250710330 ) ) ;
#30109=DIRECTION ( 'NONE',  ( 9.880513543698878618E-06, 1.241746734295183170E-06, -0.9999999999504167736 ) ) ;
#30110=DIRECTION ( 'NONE',  ( -0.6538427738826437796, -0.7566304428460742804, 5.916677973164435741E-08 ) ) ;
#30111=CARTESIAN_POINT ( 'NONE',  ( -12.10599200002982556, -20.02663609087960239, 61.58174067880212021 ) ) ;
#30113=FACE_OUTER_BOUND ( 'NONE', #42163, .T. ) ;
#30114=CARTESIAN_POINT ( 'NONE',  ( -11.81178328723415660, -10.62567094834893311, 74.73885052262691886 ) ) ;
#30115=CARTESIAN_POINT ( 'NONE',  ( -18.05316936118225968, -22.23335149483498085, 65.53187476518867527 ) ) ;
#30116=VERTEX_POINT ( 'NONE', #37898 ) ;
#30119=VERTEX_POINT ( 'NONE', #46025 ) ;
#30122=( BOUNDED_CURVE ( )  B_SPLINE_CURVE ( 3, ( #48277, #32770, #36223, #6919 ),
 .UNSPECIFIED., .F., .F. ) 
 B_SPLINE_CURVE_WITH_KNOTS ( ( 4, 4 ),
 ( 0.000000000000000000, 0.4074455897393698955 ),
 .UNSPECIFIED. ) 
 CURVE ( )  GEOMETRIC_REPRESENTATION_ITEM ( )  RATIONAL_B_SPLINE_CURVE ( ( 1.000000000000000000, 0.4567392136813278603, 0.3561768502900287681, 0.6983129098261027234 ) ) 
 REPRESENTATION_ITEM ( '' )  );
#30124=CARTESIAN_POINT ( 'NONE',  ( -11.30361205576526196, -11.41219277671509147, 64.44882039656690154 ) ) ;
#30125=CARTESIAN_POINT ( 'NONE',  ( -16.16379340615718618, -22.15191857530921382, 58.47080845268740035 ) ) ;
#30127=ORIENTED_EDGE ( 'NONE', *, *, #38941, .T. ) ;
#30129=CARTESIAN_POINT ( 'NONE',  ( -24.20371252810814866, -12.87440185077122834, 66.58774614429587757 ) ) ;
#30130=ORIENTED_EDGE ( 'NONE', *, *, #41302, .F. ) ;
#30133=ORIENTED_EDGE ( 'NONE', *, *, #19406, .T. ) ;
#30134=CARTESIAN_POINT ( 'NONE',  ( -23.38417127501956116, -19.28035200660907122, 62.54062256979923973 ) ) ;
#30136=CARTESIAN_POINT ( 'NONE',  ( -22.07022430586338402, -11.86582892075562334, 54.07175714974878389 ) ) ;
#30137=ORIENTED_EDGE ( 'NONE', *, *, #12533, .T. ) ;
#30138=CARTESIAN_POINT ( 'NONE',  ( -10.89280197141400919, -11.22507430941316642, 64.33377434530349603 ) ) ;
#30139=EDGE_CURVE ( 'NONE', #34661, #575, #7289, .T. ) ;
#30141=EDGE_CURVE ( 'NONE', #12343, #1510, #23372, .T. ) ;
#30143=CARTESIAN_POINT ( 'NONE',  ( -23.96382046939319821, -17.30576672235113378, 66.01645378202925940 ) ) ;
#30144=VERTEX_POINT ( 'NONE', #30776 ) ;
#30146=CARTESIAN_POINT ( 'NONE',  ( -10.92750425249182022, -11.16255029878774252, 64.26386639478288032 ) ) ;
#30147=CARTESIAN_POINT ( 'NONE',  ( -10.39074299160501980, -14.27365074699323522, 68.15800167629423356 ) ) ;
#30148=CARTESIAN_POINT ( 'NONE',  ( -20.94708704702029323, -20.85805098747363928, 62.22357391611139832 ) ) ;
#30149=EDGE_CURVE ( 'NONE', #1086, #42645, #41095, .T. ) ;
#30152=EDGE_LOOP ( 'NONE', ( #20205, #13097, #34198, #17220, #34067 ) ) ;
#30153=FACE_OUTER_BOUND ( 'NONE', #20959, .T. ) ;
#30158=CARTESIAN_POINT ( 'NONE',  ( -22.55199058362584452, -10.04362098402029346, 73.49777690555987419 ) ) ;
#30159=FACE_OUTER_BOUND ( 'NONE', #27352, .T. ) ;
#30162=CARTESIAN_POINT ( 'NONE',  ( -14.72744631621160494, -8.295007313424175521, 60.60524229057013201 ) ) ;
#30163=PLANE ( 'NONE',  #48503 ) ;
#30164=B_SPLINE_CURVE_WITH_KNOTS ( 'NONE', 3,
 ( #5998, #39493, #5039, #35547, #47127, #1822, #17060, #5773, #27683, #12412 ),
 .UNSPECIFIED., .F., .F.,
 ( 4, 2, 2, 2, 4 ),
 ( 0.1272669073658617700, 0.2522669073463401634, 0.3772669073268185014, 0.5022669073072968393, 0.6272669072877752328 ),
 .UNSPECIFIED. ) ;
#30166=EDGE_LOOP ( 'NONE', ( #1816, #7869, #5888, #45334 ) ) ;
#30169=CARTESIAN_POINT ( 'NONE',  ( -12.84137621205286628, -8.935279004184852880, 67.50130000652654871 ) ) ;
#30170=DIRECTION ( 'NONE',  ( -0.5881408891789771110, -0.8087584895849666555, 7.565907428972492613E-08 ) ) ;
#30171=( BOUNDED_SURFACE ( )  B_SPLINE_SURFACE ( 3, 1, ( 
 ( #38835, #20375 ),
 ( #30976, #30742 ),
 ( #42053, #15932 ),
 ( #23835, #934 ),
 ( #9294, #8327 ),
 ( #45769, #1161 ),
 ( #16661, #24316 ) ),
 .UNSPECIFIED., .T., .F., .F. ) 
 B_SPLINE_SURFACE_WITH_KNOTS ( ( 4, 3, 4 ),
 ( 2, 2 ),
 ( 0.000000000000000000, 0.5000000000000000000, 1.000000000000000000 ),
 ( 0.000000000000000000, 1.000000000000000000 ),
 .UNSPECIFIED. ) 
 GEOMETRIC_REPRESENTATION_ITEM ( )  RATIONAL_B_SPLINE_SURFACE ( (
 ( 1.000000000000000000, 1.000000000000000000),
 ( 0.3333333333333335369, 0.3333333333333330373),
 ( 0.3333333333333335369, 0.3333333333333330373),
 ( 1.000000000000000000, 1.000000000000000000),
 ( 0.3333333333333333703, 0.3333333333333333703),
 ( 0.3333333333333333703, 0.3333333333333333703),
 ( 1.000000000000000000, 1.000000000000000000) ) ) 
 REPRESENTATION_ITEM ( '' )  SURFACE ( )  );
#30172=CARTESIAN_POINT ( 'NONE',  ( -24.85419441251774941, -14.26332397151243647, 69.77558371844806118 ) ) ;
#30174=EDGE_CURVE ( 'NONE', #45761, #936, #34180, .T. ) ;
#30180=EDGE_CURVE ( 'NONE', #15909, #2586, #26646, .T. ) ;
#30182=( BOUNDED_CURVE ( )  B_SPLINE_CURVE ( 3, ( #40290, #6559, #44723, #33350 ),
 .UNSPECIFIED., .F., .F. ) 
 B_SPLINE_CURVE_WITH_KNOTS ( ( 4, 4 ),
 ( 0.4074455897393631787, 0.5000000000000000000 ),
 .UNSPECIFIED. ) 
 CURVE ( )  GEOMETRIC_REPRESENTATION_ITEM ( )  RATIONAL_B_SPLINE_CURVE ( ( 0.6983129098261022794, 0.7760317562607047526, 0.8765941196520036227, 0.9999999999999977796 ) ) 
 REPRESENTATION_ITEM ( '' )  );
#30183=CARTESIAN_POINT ( 'NONE',  ( -10.80190757246176325, -17.07816907218938951, 61.45743131804429282 ) ) ;
#30184=CARTESIAN_POINT ( 'NONE',  ( -20.42942694929465119, -8.423054519096806914, 59.99692253513481432 ) ) ;
#30186=CARTESIAN_POINT ( 'NONE',  ( -23.78373255665641750, -17.85216390223663652, 59.00938192581773478 ) ) ;
#30188=CARTESIAN_POINT ( 'NONE',  ( -12.36794899618824140, -19.72224014812425708, 61.69678633597966666 ) ) ;
#30189=EDGE_CURVE ( 'NONE', #27648, #44379, #4008, .T. ) ;
#30190=VERTEX_POINT ( 'NONE', #34927 ) ;
#30191=CARTESIAN_POINT ( 'NONE',  ( -10.41569439578338496, -15.57669382292980131, 61.05261153187079515 ) ) ;
#30192=CARTESIAN_POINT ( 'NONE',  ( -18.17450402892199790, -21.77015454618090473, 68.88685014060939693 ) ) ;
#30193=CARTESIAN_POINT ( 'NONE',  ( -24.42140808089354920, -17.36692438891622103, 69.53527060154695505 ) ) ;
#30194=CARTESIAN_POINT ( 'NONE',  ( -22.07022430586338402, -11.86582892075562157, 53.49999999999995026 ) ) ;
#30195=AXIS2_PLACEMENT_3D ( 'NONE', #11181, #44930, #33068 ) ;
#30196=ORIENTED_EDGE ( 'NONE', *, *, #2436, .F. ) ;
#30197=CARTESIAN_POINT ( 'NONE',  ( -10.78898398081525301, -17.19290454168847404, 61.44271037915215317 ) ) ;
#30198=CARTESIAN_POINT ( 'NONE',  ( -24.17899278864585355, -11.66673636667039027, 59.66731167108189737 ) ) ;
#30199=B_SPLINE_CURVE_WITH_KNOTS ( 'NONE', 3,
 ( #17698, #40849, #3177, #32953, #17468, #36171, #22148, #32727, #47998, #18184 ),
 .UNSPECIFIED., .F., .F.,
 ( 4, 2, 2, 2, 4 ),
 ( 0.000000000000000000, 0.2500000000000000000, 0.5000000000000000000, 0.7500000000000000000, 1.000000000000000000 ),
 .UNSPECIFIED. ) ;
#30201=CARTESIAN_POINT ( 'NONE',  ( -24.32102769702319378, -16.00663948712615081, 66.06324977198688941 ) ) ;
#30203=CARTESIAN_POINT ( 'NONE',  ( -10.53260261225980621, -17.63940775673892603, 68.19747689442833405 ) ) ;
#30204=CARTESIAN_POINT ( 'NONE',  ( -17.14435614197124025, -7.364337588275183144, 70.61223108419747518 ) ) ;
#30205=CARTESIAN_POINT ( 'NONE',  ( -12.59809028756154525, -19.87976139299041023, 64.88177373049498442 ) ) ;
#30206=FACE_BOUND ( 'NONE', #43041, .T. ) ;
#30207=VERTEX_POINT ( 'NONE', #484 ) ;
#30208=ADVANCED_FACE ( 'NONE', ( #15470 ), #39230, .T. ) ;
#30209=CARTESIAN_POINT ( 'NONE',  ( -13.16483405634261850, -20.92159860622343004, 58.24638845815591992 ) ) ;
#30210=CARTESIAN_POINT ( 'NONE',  ( -10.83536383905390998, -17.31742040078651357, 64.62739380450889826 ) ) ;
#30212=EDGE_CURVE ( 'NONE', #37972, #5768, #9327, .T. ) ;
#30213=CARTESIAN_POINT ( 'NONE',  ( -24.31823732957325745, -17.63313362019280106, 66.05861802595141796 ) ) ;
#30214=ORIENTED_EDGE ( 'NONE', *, *, #11660, .F. ) ;
#30217=CARTESIAN_POINT ( 'NONE',  ( -10.29385348138020539, -12.64970417265235803, 64.38340698725603772 ) ) ;
#30218=CARTESIAN_POINT ( 'NONE',  ( -16.97420703900234074, -7.769956100637374519, 70.69855872207435254 ) ) ;
#30220=ORIENTED_EDGE ( 'NONE', *, *, #23033, .F. ) ;
#30222=ORIENTED_EDGE ( 'NONE', *, *, #42471, .T. ) ;
#30224=ORIENTED_EDGE ( 'NONE', *, *, #22639, .T. ) ;
#30225=CARTESIAN_POINT ( 'NONE',  ( -15.32672178808326535, -21.95796145784420261, 72.30221390644346968 ) ) ;
#30226=CARTESIAN_POINT ( 'NONE',  ( -20.57133303063786300, -8.056536552513840377, 67.03749994897439990 ) ) ;
#30227=CARTESIAN_POINT ( 'NONE',  ( -19.39004244333994720, -21.99530814555272329, 58.68540713731352554 ) ) ;
#30230=CARTESIAN_POINT ( 'NONE',  ( -13.97628689860590079, -8.204186434626230096, 70.84302338899487950 ) ) ;
#30231=DIRECTION ( 'NONE',  ( -5.731567514496413899E-31, -1.020425574103664789E-16, -1.000000000000000000 ) ) ;
#30232=EDGE_CURVE ( 'NONE', #5757, #31902, #8979, .T. ) ;
#30234=ORIENTED_EDGE ( 'NONE', *, *, #20786, .F. ) ;
#30235=( BOUNDED_SURFACE ( )  B_SPLINE_SURFACE ( 3, 1, ( 
 ( #41690, #4499 ),
 ( #42428, #37980 ),
 ( #34281, #20735 ),
 ( #24441, #6194 ),
 ( #35254, #47079 ),
 ( #27638, #35499 ),
 ( #24189, #13560 ) ),
 .UNSPECIFIED., .T., .F., .F. ) 
 B_SPLINE_SURFACE_WITH_KNOTS ( ( 4, 3, 4 ),
 ( 2, 2 ),
 ( 0.000000000000000000, 0.5000000000000000000, 1.000000000000000000 ),
 ( 0.000000000000000000, 1.000000000000000000 ),
 .UNSPECIFIED. ) 
 GEOMETRIC_REPRESENTATION_ITEM ( )  RATIONAL_B_SPLINE_SURFACE ( (
 ( 1.000000000000000000, 1.000000000000000000),
 ( 0.3333333333333335369, 0.3333333333333330373),
 ( 0.3333333333333335369, 0.3333333333333330373),
 ( 1.000000000000000000, 1.000000000000000000),
 ( 0.3333333333333333703, 0.3333333333333333703),
 ( 0.3333333333333333703, 0.3333333333333333703),
 ( 1.000000000000000000, 1.000000000000000000) ) ) 
 REPRESENTATION_ITEM ( '' )  SURFACE ( )  );
#30236=CARTESIAN_POINT ( 'NONE',  ( -19.36683724782897897, -21.58655468785150688, 62.00975759738177118 ) ) ;
#30237=EDGE_CURVE ( 'NONE', #26502, #3283, #31349, .T. ) ;
#30238=EDGE_CURVE ( 'NONE', #5029, #24134, #42527, .T. ) ;
#30239=VECTOR ( 'NONE', #17575, 1000.000000000000341 ) ;
#30240=CARTESIAN_POINT ( 'NONE',  ( -13.90930827832509387, -8.240377080047705860, 74.39292945093751541 ) ) ;
#30241=CARTESIAN_POINT ( 'NONE',  ( -10.05341976060008058, -15.89348643430029462, 64.65771587268669407 ) ) ;
#30243=ORIENTED_EDGE ( 'NONE', *, *, #38381, .F. ) ;
#30245=EDGE_LOOP ( 'NONE', ( #13649, #29840, #27614, #2473, #17615 ) ) ;
#30246=CARTESIAN_POINT ( 'NONE',  ( -9.993180735906239676, -14.27626192956519269, 64.53803862179867679 ) ) ;
#30248=DIRECTION ( 'NONE',  ( 0.5327540375067997269, 0.8462701315302331162, 7.203825861310633201E-08 ) ) ;
#30249=ORIENTED_EDGE ( 'NONE', *, *, #24078, .T. ) ;
#30250=CARTESIAN_POINT ( 'NONE',  ( -20.38868793477728403, -7.974332091099226361, 70.42913073863570617 ) ) ;
#30251=B_SPLINE_CURVE_WITH_KNOTS ( 'NONE', 3,
 ( #17367, #32408, #41001, #29426, #22045, #48374, #18569, #33579, #7027, #37038 ),
 .UNSPECIFIED., .F., .F.,
 ( 4, 2, 2, 2, 4 ),
 ( 0.1272669073658565242, 0.2522669073463414957, 0.3772669073268264395, 0.5022669073073113832, 0.6272669072877963270 ),
 .UNSPECIFIED. ) ;
#30255=CARTESIAN_POINT ( 'NONE',  ( -10.38618466708840415, -14.33732170831495978, 60.91821109628303788 ) ) ;
#30256=CARTESIAN_POINT ( 'NONE',  ( -14.63795604342543655, -7.899797297607364044, 60.46996282252440835 ) ) ;
#30257=DIRECTION ( 'NONE',  ( -0.3478314405900309603, -0.9375570856950864451, 0.000000000000000000 ) ) ;
#30258=ORIENTED_EDGE ( 'NONE', *, *, #5232, .F. ) ;
#30259=CARTESIAN_POINT ( 'NONE',  ( -24.69316504521514233, -16.44114857855330669, 59.32321200223080382 ) ) ;
#30261=VECTOR ( 'NONE', #10274, 1000.000000000000000 ) ;
#30262=DIRECTION ( 'NONE',  ( 6.471065204144449778E-06, 1.909039588689591427E-06, -0.9999999999772404280 ) ) ;
#30264=VERTEX_POINT ( 'NONE', #24346 ) ;
#30265=FACE_OUTER_BOUND ( 'NONE', #34701, .T. ) ;
#30266=CARTESIAN_POINT ( 'NONE',  ( -24.06765785688162751, -12.42634649716644013, 69.92810001462744651 ) ) ;
#30267=VECTOR ( 'NONE', #34914, 1000.000000000000000 ) ;
#30269=ADVANCED_FACE ( 'NONE', ( #1691 ), #45859, .T. ) ;
#30270=ORIENTED_EDGE ( 'NONE', *, *, #30788, .F. ) ;
#30271=CARTESIAN_POINT ( 'NONE',  ( -21.42950876998643750, -20.55006782965317669, 72.59734371715153145 ) ) ;
#30272=CARTESIAN_POINT ( 'NONE',  ( -16.34730751551633077, -7.892078375978933913, 60.48411973959233734 ) ) ;
#30273=B_SPLINE_CURVE_WITH_KNOTS ( 'NONE', 3,
 ( #11716, #3850, #30445, #10987, #37300, #18858, #45459, #33866, #4102, #19101 ),
 .UNSPECIFIED., .F., .F.,
 ( 4, 2, 2, 2, 4 ),
 ( 0.1272669073657819172, 0.2522669073462828759, 0.3772669073267839179, 0.5022669073072848489, 0.6272669072877858909 ),
 .UNSPECIFIED. ) ;
#30275=ORIENTED_EDGE ( 'NONE', *, *, #28089, .T. ) ;
#30276=CARTESIAN_POINT ( 'NONE',  ( -19.09948850906665285, -8.012659424734943414, 63.73089235424028942 ) ) ;
#30277=CARTESIAN_POINT ( 'NONE',  ( -21.73098984888145679, -8.730191469543168381, 70.31627926275058371 ) ) ;
#30280=DIRECTION ( 'NONE',  ( -0.2573866790907600177, -0.9663084897829604669, -6.714855467380868574E-08 ) ) ;
#30281=CARTESIAN_POINT ( 'NONE',  ( -15.02405691534179688, -8.340062653448301333, 47.99999999999994316 ) ) ;
#30285=CARTESIAN_POINT ( 'NONE',  ( -12.45784128279547431, -19.74247851094704487, 61.41181112604091652 ) ) ;
#30286=B_SPLINE_CURVE_WITH_KNOTS ( 'NONE', 3,
 ( #47809, #9679, #44151, #24695, #48052, #40419, #5966, #21708, #35993, #36691 ),
 .UNSPECIFIED., .F., .F.,
 ( 4, 2, 2, 2, 4 ),
 ( 0.6272669072877788965, 0.7522669073072940638, 0.8772669073268093420, 1.002266907346324398, 1.127266907365839677 ),
 .UNSPECIFIED. ) ;
#30287=CARTESIAN_POINT ( 'NONE',  ( -12.15399301493812878, -9.543295845094297292, 57.20440096431307353 ) ) ;
#30290=ORIENTED_EDGE ( 'NONE', *, *, #11053, .T. ) ;
#30293=EDGE_CURVE ( 'NONE', #20123, #48485, #32611, .T. ) ;
#30294=B_SPLINE_CURVE_WITH_KNOTS ( 'NONE', 1,
 ( #47528, #20701 ),
 .UNSPECIFIED., .F., .F.,
 ( 2, 2 ),
 ( 0.000000000000000000, 1.000000000000000000 ),
 .UNSPECIFIED. ) ;
#30297=VERTEX_POINT ( 'NONE', #37029 ) ;
#30298=VECTOR ( 'NONE', #3741, 1000.000000000000114 ) ;
#30299=EDGE_CURVE ( 'NONE', #15104, #26867, #17191, .T. ) ;
#30300=EDGE_CURVE ( 'NONE', #32895, #32695, #22482, .T. ) ;
#30302=CARTESIAN_POINT ( 'NONE',  ( -19.89748337530321365, -21.35767964923046236, 68.98863364564390110 ) ) ;
#30303=AXIS2_PLACEMENT_3D ( 'NONE', #16975, #12817, #12579 ) ;
#30304=CARTESIAN_POINT ( 'NONE',  ( -17.01596769717176372, -7.370308014455987156, 74.07522855441366971 ) ) ;
#30305=CARTESIAN_POINT ( 'NONE',  ( -13.31969252371020929, -21.02664138888986756, 61.71657530956684212 ) ) ;
#30306=FACE_OUTER_BOUND ( 'NONE', #4284, .T. ) ;
#30307=( BOUNDED_CURVE ( )  B_SPLINE_CURVE ( 3, ( #3361, #7559, #7321, #647 ),
 .UNSPECIFIED., .F., .F. ) 
 B_SPLINE_CURVE_WITH_KNOTS ( ( 4, 4 ),
 ( 0.4074455897393696735, 0.5000000000000000000 ),
 .UNSPECIFIED. ) 
 CURVE ( )  GEOMETRIC_REPRESENTATION_ITEM ( )  RATIONAL_B_SPLINE_CURVE ( ( 0.6983129098261152690, 0.7760317562607143005, 0.8765941196520082856, 0.9999999999999950040 ) ) 
 REPRESENTATION_ITEM ( '' )  );
#30309=CARTESIAN_POINT ( 'NONE',  ( -13.53325622885376944, -21.16256470055228789, 65.17124264509627096 ) ) ;
#30311=EDGE_CURVE ( 'NONE', #40297, #16415, #26117, .T. ) ;
#30312=ORIENTED_EDGE ( 'NONE', *, *, #39279, .F. ) ;
#30313=CARTESIAN_POINT ( 'NONE',  ( -10.37871274698333046, -17.23124524545501046, 61.41389037703014964 ) ) ;
#30314=CARTESIAN_POINT ( 'NONE',  ( -11.10300763040008398, -10.86615618544839457, 57.39398486019972268 ) ) ;
#30316=( BOUNDED_SURFACE ( )  B_SPLINE_SURFACE ( 3, 1, ( 
 ( #10096, #25119 ),
 ( #12814, #16502 ),
 ( #5691, #9630 ),
 ( #9859, #35938 ),
 ( #24646, #2213 ),
 ( #35690, #24874 ),
 ( #29046, #40139 ) ),
 .UNSPECIFIED., .T., .F., .F. ) 
 B_SPLINE_SURFACE_WITH_KNOTS ( ( 4, 3, 4 ),
 ( 2, 2 ),
 ( 0.000000000000000000, 0.5000000000000000000, 1.000000000000000000 ),
 ( 0.000000000000000000, 1.000000000000000000 ),
 .UNSPECIFIED. ) 
 GEOMETRIC_REPRESENTATION_ITEM ( )  RATIONAL_B_SPLINE_SURFACE ( (
 ( 1.000000000000000000, 1.000000000000000000),
 ( 0.3333333333333335369, 0.3333333333333330373),
 ( 0.3333333333333335369, 0.3333333333333330373),
 ( 1.000000000000000000, 1.000000000000000000),
 ( 0.3333333333333333703, 0.3333333333333333703),
 ( 0.3333333333333333703, 0.3333333333333333703),
 ( 1.000000000000000000, 1.000000000000000000) ) ) 
 REPRESENTATION_ITEM ( '' )  SURFACE ( )  );
#30317=ORIENTED_EDGE ( 'NONE', *, *, #7685, .T. ) ;
#30318=( BOUNDED_CURVE ( )  B_SPLINE_CURVE ( 3, ( #2043, #17041, #6230, #32090 ),
 .UNSPECIFIED., .F., .F. ) 
 B_SPLINE_CURVE_WITH_KNOTS ( ( 4, 4 ),
 ( 0.9074455897393708392, 1.000000000000000000 ),
 .UNSPECIFIED. ) 
 CURVE ( )  GEOMETRIC_REPRESENTATION_ITEM ( )  RATIONAL_B_SPLINE_CURVE ( ( 0.6983129098261174894, 0.7760317562607192965, 0.8765941196520135037, 1.000000000000000000 ) ) 
 REPRESENTATION_ITEM ( '' )  );
#30321=CARTESIAN_POINT ( 'NONE',  ( -22.28538024775887294, -19.92612572838908491, 72.78833238834644703 ) ) ;
#30324=CARTESIAN_POINT ( 'NONE',  ( -13.65684165595416921, -8.849801312179289781, 56.98439896120441261 ) ) ;
#30327=CARTESIAN_POINT ( 'NONE',  ( -10.78967749848787427, -12.41559940729129785, 61.21342246320382685 ) ) ;
#30328=CARTESIAN_POINT ( 'NONE',  ( -10.63109664364847440, -11.75017249117723317, 74.70840197822751350 ) ) ;
#30331=VERTEX_POINT ( 'NONE', #33832 ) ;
#30332=DIRECTION ( 'NONE',  ( -1.149299189161336899E-05, 1.849289878362067349E-06, -0.9999999999322456423 ) ) ;
#30333=( BOUNDED_SURFACE ( )  B_SPLINE_SURFACE ( 3, 1, ( 
 ( #38107, #45283 ),
 ( #19402, #15204 ),
 ( #34406, #38601 ),
 ( #4885, #11530 ),
 ( #41575, #45774 ),
 ( #1167, #38341 ),
 ( #31213, #7858 ) ),
 .UNSPECIFIED., .T., .F., .F. ) 
 B_SPLINE_SURFACE_WITH_KNOTS ( ( 4, 3, 4 ),
 ( 2, 2 ),
 ( 0.000000000000000000, 0.5000000000000000000, 1.000000000000000000 ),
 ( 0.000000000000000000, 1.000000000000000000 ),
 .UNSPECIFIED. ) 
 GEOMETRIC_REPRESENTATION_ITEM ( )  RATIONAL_B_SPLINE_SURFACE ( (
 ( 1.000000000000000000, 1.000000000000000000),
 ( 0.3333333333333335369, 0.3333333333333330373),
 ( 0.3333333333333335369, 0.3333333333333330373),
 ( 1.000000000000000000, 1.000000000000000000),
 ( 0.3333333333333333703, 0.3333333333333333703),
 ( 0.3333333333333333703, 0.3333333333333333703),
 ( 1.000000000000000000, 1.000000000000000000) ) ) 
 REPRESENTATION_ITEM ( '' )  SURFACE ( )  );
#30334=CARTESIAN_POINT ( 'NONE',  ( -13.24203256135214346, -20.97556893053616989, 58.15994682967826179 ) ) ;
#30336=B_SPLINE_CURVE_WITH_KNOTS ( 'NONE', 1,
 ( #11782, #18920 ),
 .UNSPECIFIED., .F., .F.,
 ( 2, 2 ),
 ( 0.000000000000000000, 1.000000000000000000 ),
 .UNSPECIFIED. ) ;
#30337=CARTESIAN_POINT ( 'NONE',  ( -11.89179040387956832, -10.43929601004734486, 70.96893105543333036 ) ) ;
#30338=DIRECTION ( 'NONE',  ( -0.1738928961406289164, 0.9847645711904029486, 7.871847295470929299E-08 ) ) ;
#30339=CARTESIAN_POINT ( 'NONE',  ( -22.79478857039302042, -9.645877667282650947, 73.60348353842616120 ) ) ;
#30340=ORIENTED_EDGE ( 'NONE', *, *, #16268, .T. ) ;
#30341=ORIENTED_EDGE ( 'NONE', *, *, #18126, .F. ) ;
#30342=CARTESIAN_POINT ( 'NONE',  ( -21.46132321166677315, -9.088779937831205302, 73.79055940392021284 ) ) ;
#30343=CARTESIAN_POINT ( 'NONE',  ( -14.67111461712440601, -7.886426496449994161, 60.43500955848998757 ) ) ;
#30345=CARTESIAN_POINT ( 'NONE',  ( -10.01391823204708231, -15.58571177677185915, 57.68137499724732464 ) ) ;
#30347=CARTESIAN_POINT ( 'NONE',  ( -12.55420361774382698, -9.778633124847853964, 57.27862503956445295 ) ) ;
#30349=CARTESIAN_POINT ( 'NONE',  ( -24.39228817134714689, -14.13808901473641377, 73.40654960426921605 ) ) ;
#30350=CARTESIAN_POINT ( 'NONE',  ( -23.59429156608431200, -18.98457121427007976, 65.98422751227842298 ) ) ;
#30352=CARTESIAN_POINT ( 'NONE',  ( -24.39634131874377587, -15.43191468712751302, 73.11189705367094405 ) ) ;
#30354=CARTESIAN_POINT ( 'NONE',  ( -24.10946622006557760, -11.52159296043784309, 63.15229477024898586 ) ) ;
#30355=CARTESIAN_POINT ( 'NONE',  ( -19.59054105953293856, -21.52187752522791442, 69.02662522961304603 ) ) ;
#30356=CARTESIAN_POINT ( 'NONE',  ( -11.35719102664687874, -18.40077844947705188, 58.09242476654641507 ) ) ;
#30359=ORIENTED_EDGE ( 'NONE', *, *, #38038, .T. ) ;
#30360=ORIENTED_EDGE ( 'NONE', *, *, #32394, .F. ) ;
#30361=PLANE ( 'NONE',  #15527 ) ;
#30362=EDGE_CURVE ( 'NONE', #2842, #1538, #13652, .T. ) ;
#30363=VERTEX_POINT ( 'NONE', #30660 ) ;
#30369=CARTESIAN_POINT ( 'NONE',  ( -13.39714536113074139, -8.541322072920136677, 57.06993516337580274 ) ) ;
#30372=DIRECTION ( 'NONE',  ( 8.563106566420985232E-06, -6.519503004583679708E-06, 0.9999999999420846608 ) ) ;
#30373=CARTESIAN_POINT ( 'NONE',  ( -18.80072161947576603, -7.487499411268177418, 70.52068027036284548 ) ) ;
#30376=CARTESIAN_POINT ( 'NONE',  ( -23.93808071853957031, -17.37550477255097903, 69.48509980817377141 ) ) ;
#30377=EDGE_LOOP ( 'NONE', ( #41814, #20072, #46338, #12906, #7511 ) ) ;
#30380=CARTESIAN_POINT ( 'NONE',  ( -12.56172001024846452, -20.45377019276184427, 71.99149100736865137 ) ) ;
#30382=CARTESIAN_POINT ( 'NONE',  ( -10.73229864388703625, -12.57879810080903482, 64.56836243396730879 ) ) ;
#30383=CARTESIAN_POINT ( 'NONE',  ( -10.28365401573067039, -12.68397276782584449, 64.41836109611280392 ) ) ;
#30384=CARTESIAN_POINT ( 'NONE',  ( -11.55100916664023103, -10.22540270530303275, 71.14609986067189595 ) ) ;
#30386=ORIENTED_EDGE ( 'NONE', *, *, #11905, .F. ) ;
#30387=CARTESIAN_POINT ( 'NONE',  ( -24.25510706449861686, -16.56479617024167084, 59.53821300994621168 ) ) ;
#30388=DIRECTION ( 'NONE',  ( -0.6562885720885138774, 0.7545099801500438907, 1.193821363054685294E-08 ) ) ;
#30389=FACE_OUTER_BOUND ( 'NONE', #2929, .T. ) ;
#30390=CARTESIAN_POINT ( 'NONE',  ( -23.45651108574825372, -18.46362474097727002, 69.17883092557275404 ) ) ;
#30391=FACE_OUTER_BOUND ( 'NONE', #46986, .T. ) ;
#30392=CARTESIAN_POINT ( 'NONE',  ( -10.90759852523040507, -17.49952041063523822, 68.09721944423129969 ) ) ;
#30394=EDGE_LOOP ( 'NONE', ( #21659, #18213 ) ) ;
#30395=CARTESIAN_POINT ( 'NONE',  ( -24.63355139826557760, -12.92841318297298692, 62.94608782021682458 ) ) ;
#30397=ORIENTED_EDGE ( 'NONE', *, *, #39745, .F. ) ;
#30400=CARTESIAN_POINT ( 'NONE',  ( -10.40181215838624240, -12.32098906055858478, 57.37211424251319158 ) ) ;
#30401=ADVANCED_FACE ( 'NONE', ( #3557 ), #45678, .T. ) ;
#30403=B_SPLINE_CURVE_WITH_KNOTS ( 'NONE', 3,
 ( #21479, #40652, #33008, #32780, #13809, #6210, #47576, #44862, #17749, #6690 ),
 .UNSPECIFIED., .F., .F.,
 ( 4, 2, 2, 2, 4 ),
 ( 0.6272669072977357096, 0.7522669073147704166, 0.8772669073318051236, 1.002266907348839720, 1.127266907365874538 ),
 .UNSPECIFIED. ) ;
#30404=CARTESIAN_POINT ( 'NONE',  ( -18.51768661843271602, -21.77690966467453393, 68.70025907080108141 ) ) ;
#30405=AXIS2_PLACEMENT_3D ( 'NONE', #2911, #228, #41322 ) ;
#30407=CARTESIAN_POINT ( 'NONE',  ( -18.39099673902470045, -22.19624494031300088, 68.92176384159974134 ) ) ;
#30408=B_SPLINE_CURVE_WITH_KNOTS ( 'NONE', 1,
 ( #42957, #46168 ),
 .UNSPECIFIED., .F., .F.,
 ( 2, 2 ),
 ( 0.000000000000000000, 1.000000000000000000 ),
 .UNSPECIFIED. ) ;
#30411=( BOUNDED_SURFACE ( )  B_SPLINE_SURFACE ( 3, 1, ( 
 ( #35452, #27589 ),
 ( #46315, #20694 ),
 ( #5684, #8889 ),
 ( #43351, #35684 ),
 ( #31770, #1737 ),
 ( #12324, #24145 ),
 ( #39401, #28066 ) ),
 .UNSPECIFIED., .T., .F., .F. ) 
 B_SPLINE_SURFACE_WITH_KNOTS ( ( 4, 3, 4 ),
 ( 2, 2 ),
 ( 0.000000000000000000, 0.5000000000000000000, 1.000000000000000000 ),
 ( 0.000000000000000000, 1.000000000000000000 ),
 .UNSPECIFIED. ) 
 GEOMETRIC_REPRESENTATION_ITEM ( )  RATIONAL_B_SPLINE_SURFACE ( (
 ( 1.000000000000000000, 1.000000000000000000),
 ( 0.3333333333333335369, 0.3333333333333330373),
 ( 0.3333333333333335369, 0.3333333333333330373),
 ( 1.000000000000000000, 1.000000000000000000),
 ( 0.3333333333333333703, 0.3333333333333333703),
 ( 0.3333333333333333703, 0.3333333333333333703),
 ( 1.000000000000000000, 1.000000000000000000) ) ) 
 REPRESENTATION_ITEM ( '' )  SURFACE ( )  );
#30417=ORIENTED_EDGE ( 'NONE', *, *, #11564, .F. ) ;
#30419=EDGE_CURVE ( 'NONE', #27633, #35167, #19067, .T. ) ;
#30421=CARTESIAN_POINT ( 'NONE',  ( -19.61601346313181082, -21.50980264518277707, 65.46486213821818012 ) ) ;
#30422=ADVANCED_FACE ( 'NONE', ( #33570 ), #22520, .T. ) ;
#30424=B_SPLINE_CURVE_WITH_KNOTS ( 'NONE', 3,
 ( #5500, #17183, #3150, #24844, #18157, #35900, #2180, #36863, #47725, #36385 ),
 .UNSPECIFIED., .F., .F.,
 ( 4, 2, 2, 2, 4 ),
 ( 0.6272669072878305219, 0.7522669073073273704, 0.8772669073268243300, 1.002266907346321290, 1.127266907365818138 ),
 .UNSPECIFIED. ) ;
#30426=CARTESIAN_POINT ( 'NONE',  ( -21.12516169987187098, -20.80993955427394582, 69.06922321213187388 ) ) ;
#30427=CARTESIAN_POINT ( 'NONE',  ( -10.59656512619885227, -13.05092609425065220, 68.02360230423869325 ) ) ;
#30428=CARTESIAN_POINT ( 'NONE',  ( -18.90996118681096405, -7.968724231816139536, 67.20071784163268092 ) ) ;
#30429=DIRECTION ( 'NONE',  ( -0.8459089628457130416, -0.5333273165489313961, 7.771812504399801304E-08 ) ) ;
#30436=CARTESIAN_POINT ( 'NONE',  ( -20.22859725435685618, -8.395501029963087447, 67.00777471169989497 ) ) ;
#30437=CARTESIAN_POINT ( 'NONE',  ( -12.51505295934874518, -9.205071670917405413, 74.47956342064293267 ) ) ;
#30438=CARTESIAN_POINT ( 'NONE',  ( -24.27033112822875438, -13.12649005559073068, 63.13264177271826583 ) ) ;
#30440=CARTESIAN_POINT ( 'NONE',  ( -18.12717186014929283, -21.82707771419581633, 61.76047256604253732 ) ) ;
#30441=CARTESIAN_POINT ( 'NONE',  ( -14.67759629421408718, -7.883812837594224021, 60.49809014262143592 ) ) ;
#30442=VECTOR ( 'NONE', #46712, 1000.000000000000000 ) ;
#30443=CARTESIAN_POINT ( 'NONE',  ( -19.39738106961548425, -7.625280727630859623, 60.06069365028482565 ) ) ;
#30444=ORIENTED_EDGE ( 'NONE', *, *, #4998, .F. ) ;
#30445=CARTESIAN_POINT ( 'NONE',  ( -19.49467501587391638, -21.96586113430295484, 62.13470298284286031 ) ) ;
#30446=CARTESIAN_POINT ( 'NONE',  ( -20.81921389985186721, -21.44071754855728784, 58.75979745677555854 ) ) ;
#30448=FACE_BOUND ( 'NONE', #36338, .T. ) ;
#30450=CARTESIAN_POINT ( 'NONE',  ( -18.08967161758600994, -21.83134672834333045, 68.90694883545079108 ) ) ;
#30452=CARTESIAN_POINT ( 'NONE',  ( -24.16575376147897813, -12.74704232990201547, 69.77243002240838621 ) ) ;
#30453=CARTESIAN_POINT ( 'NONE',  ( -21.53550107051403018, -9.078485192726875042, 74.01617645989524874 ) ) ;
#30455=CARTESIAN_POINT ( 'NONE',  ( -22.66727051383977809, -10.09628829486277546, 70.31178520457007153 ) ) ;
#30456=ORIENTED_EDGE ( 'NONE', *, *, #30963, .T. ) ;
#30457=CARTESIAN_POINT ( 'NONE',  ( -19.86569447268031041, -19.73755174630646891, 53.49999999999995026 ) ) ;
#30458=LINE ( 'NONE', #11734, #28278 ) ;
#30459=( BOUNDED_CURVE ( )  B_SPLINE_CURVE ( 3, ( #6377, #35911, #21637, #21407 ),
 .UNSPECIFIED., .F., .F. ) 
 B_SPLINE_CURVE_WITH_KNOTS ( ( 4, 4 ),
 ( 0.5000000000000000000, 0.9074455897393683967 ),
 .UNSPECIFIED. ) 
 CURVE ( )  GEOMETRIC_REPRESENTATION_ITEM ( )  RATIONAL_B_SPLINE_CURVE ( ( 1.000000000000004663, 0.4567392136813338555, 0.3561768502900276023, 0.6983129098260909551 ) ) 
 REPRESENTATION_ITEM ( '' )  );
#30461=CARTESIAN_POINT ( 'NONE',  ( -13.91686280105865947, -8.236299372188803147, 74.31459218752463869 ) ) ;
#30463=B_SPLINE_CURVE_WITH_KNOTS ( 'NONE', 3,
 ( #23721, #42899, #20242, #38711, #31813, #39193, #5481, #35249, #1527, #16533 ),
 .UNSPECIFIED., .F., .F.,
 ( 4, 2, 2, 2, 4 ),
 ( 0.6272669072976988502, 0.7522669073147150165, 0.8772669073317311828, 1.002266907348747349, 1.127266907365763515 ),
 .UNSPECIFIED. ) ;
#30467=ORIENTED_EDGE ( 'NONE', *, *, #89, .F. ) ;
#30470=CARTESIAN_POINT ( 'NONE',  ( -21.26695983349702246, -20.66012254167596041, 69.12738141313978701 ) ) ;
#30471=DIRECTION ( 'NONE',  ( -4.436160455182634911E-06, -7.761523761658527715E-06, 0.9999999999600395206 ) ) ;
#30472=DIRECTION ( 'NONE',  ( 0.8705373987491421550, -0.4921022631314296847, 4.758021987246392719E-08 ) ) ;
#30475=CARTESIAN_POINT ( 'NONE',  ( -19.43397188950632781, -8.102277950761333614, 60.15020107494644463 ) ) ;
#30476=( BOUNDED_SURFACE ( )  B_SPLINE_SURFACE ( 3, 1, ( 
 ( #16366, #8508 ),
 ( #27462, #883 ),
 ( #4568, #23785 ),
 ( #26746, #19591 ),
 ( #401, #12685 ),
 ( #12201, #20075 ),
 ( #11719, #34599 ) ),
 .UNSPECIFIED., .T., .F., .F. ) 
 B_SPLINE_SURFACE_WITH_KNOTS ( ( 4, 3, 4 ),
 ( 2, 2 ),
 ( 0.000000000000000000, 0.5000000000000000000, 1.000000000000000000 ),
 ( 0.000000000000000000, 1.000000000000000000 ),
 .UNSPECIFIED. ) 
 GEOMETRIC_REPRESENTATION_ITEM ( )  RATIONAL_B_SPLINE_SURFACE ( (
 ( 1.000000000000000000, 1.000000000000000000),
 ( 0.3333333333333335369, 0.3333333333333330373),
 ( 0.3333333333333335369, 0.3333333333333330373),
 ( 1.000000000000000000, 1.000000000000000000),
 ( 0.3333333333333333703, 0.3333333333333333703),
 ( 0.3333333333333333703, 0.3333333333333333703),
 ( 1.000000000000000000, 1.000000000000000000) ) ) 
 REPRESENTATION_ITEM ( '' )  SURFACE ( )  );
#30477=VECTOR ( 'NONE', #20823, 1000.000000000000114 ) ;
#30478=VECTOR ( 'NONE', #4153, 1000.000000000000114 ) ;
#30480=ORIENTED_EDGE ( 'NONE', *, *, #20532, .T. ) ;
#30481=CARTESIAN_POINT ( 'NONE',  ( -16.09168231696496676, -7.478562553351938647, 60.31373090009974902 ) ) ;
#30483=CARTESIAN_POINT ( 'NONE',  ( -9.995738364564658696, -14.24060042610175358, 64.50308557176904856 ) ) ;
#30484=CARTESIAN_POINT ( 'NONE',  ( -10.50393342808087560, -15.87404512457899664, 68.08841022104337526 ) ) ;
#30486=CARTESIAN_POINT ( 'NONE',  ( -23.73810165963432084, -18.76483127932742789, 69.40716580542252245 ) ) ;
#30487=VERTEX_POINT ( 'NONE', #8474 ) ;
#30489=VERTEX_POINT ( 'NONE', #12887 ) ;
#30490=EDGE_CURVE ( 'NONE', #5443, #19021, #37627, .T. ) ;
#30491=CARTESIAN_POINT ( 'NONE',  ( -11.62161759534551919, -18.81995649556354877, 71.98686160459075722 ) ) ;
#30492=CARTESIAN_POINT ( 'NONE',  ( -19.04853579327176760, -7.948602568230340282, 63.71617106789811658 ) ) ;
#30493=CARTESIAN_POINT ( 'NONE',  ( -15.29809733969474195, -21.47854975192407778, 68.87592918283094434 ) ) ;
#30494=EDGE_CURVE ( 'NONE', #36010, #486, #26952, .T. ) ;
#30498=CARTESIAN_POINT ( 'NONE',  ( -12.36756753426621813, -9.896138138887707214, 57.37463480816234096 ) ) ;
#30499=EDGE_LOOP ( 'NONE', ( #18862, #7325 ) ) ;
#30503=CARTESIAN_POINT ( 'NONE',  ( -23.83512934130040861, -17.76108582422602922, 66.08789927488301430 ) ) ;
#30505=DIRECTION ( 'NONE',  ( -0.9862050927915950727, -0.1655279884246635413, -7.765682857010803534E-08 ) ) ;
#30510=CARTESIAN_POINT ( 'NONE',  ( -10.54994933093899867, -13.24305344519376959, 71.49356453765415154 ) ) ;
#30512=ORIENTED_EDGE ( 'NONE', *, *, #36711, .F. ) ;
#30513=EDGE_CURVE ( 'NONE', #9257, #1174, #42698, .T. ) ;
#30515=CARTESIAN_POINT ( 'NONE',  ( -23.81768792596037798, -11.95822681598703063, 59.76619129867536628 ) ) ;
#30516=FACE_OUTER_BOUND ( 'NONE', #23773, .T. ) ;
#30517=ORIENTED_EDGE ( 'NONE', *, *, #17708, .T. ) ;
#30518=PLANE ( 'NONE',  #14206 ) ;
#30519=CARTESIAN_POINT ( 'NONE',  ( -10.90063107880032867, -21.18736481497725421, 54.44843099904677075 ) ) ;
#30520=CARTESIAN_POINT ( 'NONE',  ( -11.39216336840796373, -18.45920852072106300, 61.29182966166492719 ) ) ;
#30523=CARTESIAN_POINT ( 'NONE',  ( -21.57995947450667984, -9.113990939708571659, 70.14604673427196246 ) ) ;
#30524=EDGE_LOOP ( 'NONE', ( #36584, #13778, #25471, #11688, #42712 ) ) ;
#30525=VERTEX_POINT ( 'NONE', #5032 ) ;
#30533=CARTESIAN_POINT ( 'NONE',  ( -10.79572441526863180, -11.40795732096215254, 67.80359905390240272 ) ) ;
#30534=VERTEX_POINT ( 'NONE', #9210 ) ;
#30535=DIRECTION ( 'NONE',  ( -0.9918916210775229336, -0.1270866320121812332, 6.503929234589265847E-08 ) ) ;
#30537=CARTESIAN_POINT ( 'NONE',  ( -17.06879511326789256, -7.767867012253359071, 73.97490359703523666 ) ) ;
#30538=FACE_OUTER_BOUND ( 'NONE', #40349, .T. ) ;
#30540=AXIS2_PLACEMENT_3D ( 'NONE', #13870, #2086, #21300 ) ;
#30541=ORIENTED_EDGE ( 'NONE', *, *, #26815, .T. ) ;
#30542=VECTOR ( 'NONE', #20620, 1000.000000000000114 ) ;
#30543=ORIENTED_EDGE ( 'NONE', *, *, #9071, .T. ) ;
#30544=EDGE_CURVE ( 'NONE', #44170, #22485, #11907, .T. ) ;
#30546=CARTESIAN_POINT ( 'NONE',  ( -12.79725838692604434, -20.12850099319811292, 71.80653676770127447 ) ) ;
#30547=CARTESIAN_POINT ( 'NONE',  ( -21.89130958583942288, -9.354787850460871468, 63.20625856529903075 ) ) ;
#30548=CARTESIAN_POINT ( 'NONE',  ( -10.05862351292959467, -15.92886012141397245, 64.69266982328383619 ) ) ;
#30550=ORIENTED_EDGE ( 'NONE', *, *, #12337, .T. ) ;
#30551=DIRECTION ( 'NONE',  ( -5.935091885548698876E-07, -2.117535313761473712E-07, 0.9999999999998014921 ) ) ;
#30552=CARTESIAN_POINT ( 'NONE',  ( -13.27770465421436619, -9.107456272842560097, 64.20946529204060482 ) ) ;
#30556=ORIENTED_EDGE ( 'NONE', *, *, #4349, .F. ) ;
#30558=ADVANCED_FACE ( 'NONE', ( #46873 ), #14318, .T. ) ;
#30559=ORIENTED_EDGE ( 'NONE', *, *, #37606, .F. ) ;
#30560=CARTESIAN_POINT ( 'NONE',  ( -22.51726263819124441, -19.68384825699994423, 72.79400547081151274 ) ) ;
#30561=CARTESIAN_POINT ( 'NONE',  ( -20.39214861733253770, -8.469596852450818503, 63.50224710712079457 ) ) ;
#30562=ORIENTED_EDGE ( 'NONE', *, *, #27895, .T. ) ;
#30563=CARTESIAN_POINT ( 'NONE',  ( -9.982716954774490503, -14.44908413001617298, 67.97304700561097945 ) ) ;
#30566=DIRECTION ( 'NONE',  ( -1.066846703571655765E-06, 9.113387012630844478E-06, 0.9999999999579040066 ) ) ;
#30568=CARTESIAN_POINT ( 'NONE',  ( -12.87522519725752268, -8.909181681006783649, 67.52942783090081491 ) ) ;
#30570=CARTESIAN_POINT ( 'NONE',  ( -18.91168463870544869, -7.914867951563272719, 63.31600393140114136 ) ) ;
#30571=CARTESIAN_POINT ( 'NONE',  ( -10.66703363856100317, -12.79807828486586807, 64.26836111018113229 ) ) ;
#30573=CARTESIAN_POINT ( 'NONE',  ( -19.18784625403669963, -21.58347547587811377, 58.52507428381958476 ) ) ;
#30576=CARTESIAN_POINT ( 'NONE',  ( -13.43773910423563400, -20.62433115109003268, 58.33177939114180788 ) ) ;
#30578=CARTESIAN_POINT ( 'NONE',  ( -24.84449963183508459, -13.71944596863515464, 53.49999999999994316 ) ) ;
#30579=CARTESIAN_POINT ( 'NONE',  ( -17.06648941491218707, -7.818287007874094030, 70.56323971375660165 ) ) ;
#30582=DIRECTION ( 'NONE',  ( 0.4251432040024066827, 0.9051260995521939190, 1.185120001106693976E-09 ) ) ;
#30583=LINE ( 'NONE', #11859, #27370 ) ;
#30584=ORIENTED_EDGE ( 'NONE', *, *, #35114, .F. ) ;
#30585=CARTESIAN_POINT ( 'NONE',  ( -23.22909885928854834, -6.086929677699679075, 53.49999999999995026 ) ) ;
#30586=CARTESIAN_POINT ( 'NONE',  ( -15.74539340629102924, -7.550670488425484272, 67.31724133890321582 ) ) ;
#30589=FACE_OUTER_BOUND ( 'NONE', #46097, .T. ) ;
#30590=CARTESIAN_POINT ( 'NONE',  ( -14.22441598498101989, -8.081217260141077219, 67.44470407312981308 ) ) ;
#30591=CARTESIAN_POINT ( 'NONE',  ( -24.29039363205059843, -16.40874438636378230, 59.12892251125953891 ) ) ;
#30594=EDGE_CURVE ( 'NONE', #47031, #2695, #22449, .T. ) ;
#30596=CARTESIAN_POINT ( 'NONE',  ( -12.11086159817483932, -20.03164753588056257, 61.51865900489719508 ) ) ;
#30597=CARTESIAN_POINT ( 'NONE',  ( -13.79232328012607312, -20.79486899771962172, 68.68455086219127281 ) ) ;
#30598=CARTESIAN_POINT ( 'NONE',  ( -19.77787797429642325, -21.45850311741518368, 72.49658723834933483 ) ) ;
#30599=( BOUNDED_SURFACE ( )  B_SPLINE_SURFACE ( 3, 1, ( 
 ( #24986, #2331 ),
 ( #28196, #2577 ),
 ( #36294, #17577 ),
 ( #5798, #17338 ),
 ( #21540, #16849 ),
 ( #31889, #39756 ),
 ( #39277, #39519 ) ),
 .UNSPECIFIED., .T., .F., .F. ) 
 B_SPLINE_SURFACE_WITH_KNOTS ( ( 4, 3, 4 ),
 ( 2, 2 ),
 ( 0.000000000000000000, 0.5000000000000000000, 1.000000000000000000 ),
 ( 0.000000000000000000, 1.000000000000000000 ),
 .UNSPECIFIED. ) 
 GEOMETRIC_REPRESENTATION_ITEM ( )  RATIONAL_B_SPLINE_SURFACE ( (
 ( 1.000000000000000000, 1.000000000000000000),
 ( 0.3333333333333335369, 0.3333333333333330373),
 ( 0.3333333333333335369, 0.3333333333333330373),
 ( 1.000000000000000000, 1.000000000000000000),
 ( 0.3333333333333333703, 0.3333333333333333703),
 ( 0.3333333333333333703, 0.3333333333333333703),
 ( 1.000000000000000000, 1.000000000000000000) ) ) 
 REPRESENTATION_ITEM ( '' )  SURFACE ( )  );
#30600=CARTESIAN_POINT ( 'NONE',  ( -18.45262242793555885, -21.79183460504582470, 65.50099240037707204 ) ) ;
#30601=ORIENTED_EDGE ( 'NONE', *, *, #44739, .T. ) ;
#30603=CARTESIAN_POINT ( 'NONE',  ( -20.23203131230217267, -21.71059417314907591, 72.51823477531823414 ) ) ;
#30604=ORIENTED_EDGE ( 'NONE', *, *, #44209, .T. ) ;
#30607=B_SPLINE_CURVE_WITH_KNOTS ( 'NONE', 1,
 ( #24039, #1360 ),
 .UNSPECIFIED., .F., .F.,
 ( 2, 2 ),
 ( 0.000000000000000000, 1.000000000000000000 ),
 .UNSPECIFIED. ) ;
#30608=CARTESIAN_POINT ( 'NONE',  ( -22.78151503426583702, -19.98625364524674097, 72.75905110386234753 ) ) ;
#30609=( BOUNDED_SURFACE ( )  B_SPLINE_SURFACE ( 3, 1, ( 
 ( #47233, #43785 ),
 ( #21131, #21381 ),
 ( #13477, #10046 ),
 ( #2649, #28994 ),
 ( #17658, #32685 ),
 ( #47705, #40323 ),
 ( #15409, #26771 ) ),
 .UNSPECIFIED., .T., .F., .F. ) 
 B_SPLINE_SURFACE_WITH_KNOTS ( ( 4, 3, 4 ),
 ( 2, 2 ),
 ( 0.000000000000000000, 0.5000000000000000000, 1.000000000000000000 ),
 ( 0.000000000000000000, 1.000000000000000000 ),
 .UNSPECIFIED. ) 
 GEOMETRIC_REPRESENTATION_ITEM ( )  RATIONAL_B_SPLINE_SURFACE ( (
 ( 1.000000000000000000, 1.000000000000000000),
 ( 0.3333333333333335369, 0.3333333333333330373),
 ( 0.3333333333333335369, 0.3333333333333330373),
 ( 1.000000000000000000, 1.000000000000000000),
 ( 0.3333333333333333703, 0.3333333333333333703),
 ( 0.3333333333333333703, 0.3333333333333333703),
 ( 1.000000000000000000, 1.000000000000000000) ) ) 
 REPRESENTATION_ITEM ( '' )  SURFACE ( )  );
#30610=VECTOR ( 'NONE', #9453, 1000.000000000000114 ) ;
#30611=VECTOR ( 'NONE', #28825, 1000.000000000000114 ) ;
#30612=CARTESIAN_POINT ( 'NONE',  ( -16.00544582274271477, -7.903112417841744453, 63.95538887075813506 ) ) ;
#30613=CARTESIAN_POINT ( 'NONE',  ( -16.11840895131430429, -22.14390444347510822, 58.48596779410638646 ) ) ;
#30615=CARTESIAN_POINT ( 'NONE',  ( -15.95021555058110607, -7.506329832067567764, 63.79198235507756465 ) ) ;
#30616=AXIS2_PLACEMENT_3D ( 'NONE', #37557, #26254, #7555 ) ;
#30617=FACE_OUTER_BOUND ( 'NONE', #40955, .T. ) ;
#30618=ORIENTED_EDGE ( 'NONE', *, *, #7572, .F. ) ;
#30619=CARTESIAN_POINT ( 'NONE',  ( -10.79220951835107023, -12.56890123353462307, 57.55530741402424155 ) ) ;
#30620=FACE_OUTER_BOUND ( 'NONE', #33727, .T. ) ;
#30621=( BOUNDED_SURFACE ( )  B_SPLINE_SURFACE ( 3, 1, ( 
 ( #48344, #45399 ),
 ( #7496, #40968 ),
 ( #45170, #22496 ),
 ( #7741, #26434 ),
 ( #7252, #29640 ),
 ( #41702, #2625 ),
 ( #18542, #37493 ) ),
 .UNSPECIFIED., .T., .F., .F. ) 
 B_SPLINE_SURFACE_WITH_KNOTS ( ( 4, 3, 4 ),
 ( 2, 2 ),
 ( 0.000000000000000000, 0.5000000000000000000, 1.000000000000000000 ),
 ( 0.000000000000000000, 1.000000000000000000 ),
 .UNSPECIFIED. ) 
 GEOMETRIC_REPRESENTATION_ITEM ( )  RATIONAL_B_SPLINE_SURFACE ( (
 ( 1.000000000000000000, 1.000000000000000000),
 ( 0.3333333333333335369, 0.3333333333333330373),
 ( 0.3333333333333335369, 0.3333333333333330373),
 ( 1.000000000000000000, 1.000000000000000000),
 ( 0.3333333333333333703, 0.3333333333333333703),
 ( 0.3333333333333333703, 0.3333333333333333703),
 ( 1.000000000000000000, 1.000000000000000000) ) ) 
 REPRESENTATION_ITEM ( '' )  SURFACE ( )  );
#30624=CARTESIAN_POINT ( 'NONE',  ( -16.78341102624552050, -22.23169286577646986, 68.88055947109249644 ) ) ;
#30625=CARTESIAN_POINT ( 'NONE',  ( -22.58065782673598321, -12.89613362149922438, 53.49999999999995026 ) ) ;
#30626=ORIENTED_EDGE ( 'NONE', *, *, #43652, .F. ) ;
#30628=EDGE_CURVE ( 'NONE', #18626, #1976, #12771, .T. ) ;
#30629=FACE_OUTER_BOUND ( 'NONE', #27498, .T. ) ;
#30631=ORIENTED_EDGE ( 'NONE', *, *, #12545, .F. ) ;
#30633=DIRECTION ( 'NONE',  ( -0.1186632576870824130, 0.9929345553837299887, 6.051931679537041823E-08 ) ) ;
#30634=CARTESIAN_POINT ( 'NONE',  ( -20.85321405943728834, -20.91189875045330737, 62.41471372066478551 ) ) ;
#30636=ADVANCED_FACE ( 'NONE', ( #40216 ), #40801, .T. ) ;
#30637=CARTESIAN_POINT ( 'NONE',  ( -22.33376602745314798, -19.86903051493497685, 69.18890041286789483 ) ) ;
#30639=ORIENTED_EDGE ( 'NONE', *, *, #43012, .F. ) ;
#30640=EDGE_CURVE ( 'NONE', #29387, #17516, #34204, .T. ) ;
#30642=CARTESIAN_POINT ( 'NONE',  ( -24.10584592916820057, -12.56049825913868645, 73.24225570139947195 ) ) ;
#30645=DIRECTION ( 'NONE',  ( -1.148482744091818979E-06, 2.957121237693701878E-08, 0.9999999999993399724 ) ) ;
#30646=EDGE_CURVE ( 'NONE', #35257, #10902, #9555, .T. ) ;
#30648=CARTESIAN_POINT ( 'NONE',  ( -13.11946000997128436, -9.225961346166455357, 67.52942785706356688 ) ) ;
#30649=ORIENTED_EDGE ( 'NONE', *, *, #46117, .F. ) ;
#30650=CARTESIAN_POINT ( 'NONE',  ( -21.24554616535955631, -21.20453920045676810, 65.76949338751086316 ) ) ;
#30653=CARTESIAN_POINT ( 'NONE',  ( -24.42340526462838923, -14.70674901051565975, 59.46973661257310084 ) ) ;
#30654=CARTESIAN_POINT ( 'NONE',  ( -23.48373383537063930, -18.31359856532379737, 72.95471315433937320 ) ) ;
#30655=EDGE_CURVE ( 'NONE', #39625, #46585, #19381, .T. ) ;
#30656=VERTEX_POINT ( 'NONE', #13598 ) ;
#30660=CARTESIAN_POINT ( 'NONE',  ( -21.80947544975385810, -9.353161466788067813, 63.19153755920122251 ) ) ;
#30663=VERTEX_POINT ( 'NONE', #45134 ) ;
#30664=ORIENTED_EDGE ( 'NONE', *, *, #3386, .T. ) ;
#30666=CARTESIAN_POINT ( 'NONE',  ( -16.94458633259734270, -7.374567983260779336, 74.14513688882354359 ) ) ;
#30667=CARTESIAN_POINT ( 'NONE',  ( -18.98390459359973548, -7.933620001262258192, 66.91543923465640376 ) ) ;
#30669=CARTESIAN_POINT ( 'NONE',  ( -15.32672178808326535, -21.95796145784420261, 72.30221390644346968 ) ) ;
#30670=CARTESIAN_POINT ( 'NONE',  ( -20.05785487306503256, -7.839488668639425839, 73.83441365354759967 ) ) ;
#30671=CARTESIAN_POINT ( 'NONE',  ( -24.77723877343947478, -16.00713684962007122, 66.24820200538215431 ) ) ;
#30674=FACE_OUTER_BOUND ( 'NONE', #34387, .T. ) ;
#30676=ORIENTED_EDGE ( 'NONE', *, *, #4562, .F. ) ;
#30678=CARTESIAN_POINT ( 'NONE',  ( -24.39403702774331606, -17.44049340399234893, 69.52844358061491903 ) ) ;
#30680=ADVANCED_FACE ( 'NONE', ( #22465 ), #15618, .T. ) ;
#30681=ORIENTED_EDGE ( 'NONE', *, *, #1877, .F. ) ;
#30682=CARTESIAN_POINT ( 'NONE',  ( -10.33431758219403207, -12.52035302217920254, 60.98348881056122650 ) ) ;
#30683=CARTESIAN_POINT ( 'NONE',  ( -14.68422391818051587, -7.881140326852841937, 60.48142765572568180 ) ) ;
#30684=CARTESIAN_POINT ( 'NONE',  ( -23.30282330091471366, -18.60927750845715067, 69.29371984660140527 ) ) ;
#30685=CARTESIAN_POINT ( 'NONE',  ( -24.46506320217640962, -17.24406362331221132, 72.99840605271779737 ) ) ;
#30686=ORIENTED_EDGE ( 'NONE', *, *, #37842, .F. ) ;
#30687=CARTESIAN_POINT ( 'NONE',  ( -10.33966868199281386, -17.11483672006214718, 57.84793901998011023 ) ) ;
#30692=VERTEX_POINT ( 'NONE', #18764 ) ;
#30693=CARTESIAN_POINT ( 'NONE',  ( -20.87011516470288797, -20.96386168028406871, 58.64475080180090316 ) ) ;
#30694=DIRECTION ( 'NONE',  ( 0.2393415023380396356, -0.9709354485539014590, 6.438601123316498798E-08 ) ) ;
#30696=FACE_OUTER_BOUND ( 'NONE', #40967, .T. ) ;
#30699=ORIENTED_EDGE ( 'NONE', *, *, #43521, .F. ) ;
#30700=CARTESIAN_POINT ( 'NONE',  ( -10.10423179225323054, -16.19963241119870645, 71.63405780323361682 ) ) ;
#30702=EDGE_LOOP ( 'NONE', ( #47333, #5164, #41881, #37299, #44572 ) ) ;
#30703=CARTESIAN_POINT ( 'NONE',  ( -7.334870405450504727, -11.98365049024292972, 53.49999999999995026 ) ) ;
#30704=LINE ( 'NONE', #27715, #28238 ) ;
#30708=EDGE_LOOP ( 'NONE', ( #36307, #37597, #11922, #24556, #29416 ) ) ;
#30709=ORIENTED_EDGE ( 'NONE', *, *, #9149, .F. ) ;
#30710=ORIENTED_EDGE ( 'NONE', *, *, #41183, .T. ) ;
#30712=AXIS2_PLACEMENT_3D ( 'NONE', #37672, #21933, #10849 ) ;
#30713=CARTESIAN_POINT ( 'NONE',  ( -13.71293426195967413, -21.26916566922604801, 68.64120525947689089 ) ) ;
#30714=DIRECTION ( 'NONE',  ( 0.9811758422909349076, 0.1931164583992469319, 7.863147543881890502E-08 ) ) ;
#30715=ADVANCED_FACE ( 'NONE', ( #30113 ), #7464, .T. ) ;
#30716=CARTESIAN_POINT ( 'NONE',  ( -24.17271849214968071, -12.95015691860989371, 66.60246741689840633 ) ) ;
#30717=CARTESIAN_POINT ( 'NONE',  ( -11.81163076501576015, -9.909691595435425882, 64.16767832365785296 ) ) ;
#30718=AXIS2_PLACEMENT_3D ( 'NONE', #26283, #3627, #15668 ) ;
#30719=VERTEX_POINT ( 'NONE', #37715 ) ;
#30721=CARTESIAN_POINT ( 'NONE',  ( -24.83263366448169762, -15.59490076022755112, 73.18799035805197661 ) ) ;
#30722=CARTESIAN_POINT ( 'NONE',  ( -10.37743716876973643, -14.51010320183636715, 64.27315137562472103 ) ) ;
#30723=CARTESIAN_POINT ( 'NONE',  ( -24.14992822999210276, -18.01341164000503525, 59.11882993461590274 ) ) ;
#30724=VECTOR ( 'NONE', #24483, 1000.000000000000227 ) ;
#30725=CARTESIAN_POINT ( 'NONE',  ( -11.42622084110231029, -18.51434063454203738, 61.27710833181470917 ) ) ;
#30726=VERTEX_POINT ( 'NONE', #11622 ) ;
#30727=B_SPLINE_CURVE_WITH_KNOTS ( 'NONE', 3,
 ( #34248, #38183, #534, #45357, #15777, #33761, #19480, #45614, #46078, #22710 ),
 .UNSPECIFIED., .F., .F.,
 ( 4, 2, 2, 2, 4 ),
 ( 0.1272669073658455330, 0.2522669073463257861, 0.3772669073268060114, 0.5022669073072862922, 0.6272669072877665730 ),
 .UNSPECIFIED. ) ;
#30729=VERTEX_POINT ( 'NONE', #22969 ) ;
#30730=CARTESIAN_POINT ( 'NONE',  ( -10.01440787728688520, -14.03439562150409969, 61.03325889150411143 ) ) ;
#30732=FACE_OUTER_BOUND ( 'NONE', #4662, .T. ) ;
#30734=ORIENTED_EDGE ( 'NONE', *, *, #28511, .T. ) ;
#30735=CARTESIAN_POINT ( 'NONE',  ( -22.53429313110963506, -9.952421254863264011, 73.78161091678163075 ) ) ;
#30736=CARTESIAN_POINT ( 'NONE',  ( -10.47425521701617157, -17.49314416303823450, 64.81234701634230078 ) ) ;
#30737=CARTESIAN_POINT ( 'NONE',  ( -24.19967835704668246, -11.71176484350101354, 59.58261478314079795 ) ) ;
#30739=VERTEX_POINT ( 'NONE', #22224 ) ;
#30740=CARTESIAN_POINT ( 'NONE',  ( -10.39215600595210631, -14.30487551902977650, 64.38803863383273551 ) ) ;
#30742=CARTESIAN_POINT ( 'NONE',  ( -17.29025345054776963, -7.359659516233258536, 67.13384346071842401 ) ) ;
#30744=EDGE_LOOP ( 'NONE', ( #6834, #42805, #41589, #10206, #20730 ) ) ;
#30745=CARTESIAN_POINT ( 'NONE',  ( -24.45201639769885205, -14.25170802724723451, 69.80275273439818307 ) ) ;
#30746=AXIS2_PLACEMENT_3D ( 'NONE', #44715, #34092, #14616 ) ;
#30747=ORIENTED_EDGE ( 'NONE', *, *, #5265, .F. ) ;
#30748=CARTESIAN_POINT ( 'NONE',  ( -18.66311988809301425, -7.868636481342422329, 70.65595886192740238 ) ) ;
#30749=ORIENTED_EDGE ( 'NONE', *, *, #30419, .T. ) ;
#30750=CARTESIAN_POINT ( 'NONE',  ( -22.16045306466799403, -20.56002303229518446, 58.92589421280841577 ) ) ;
#30751=LINE ( 'NONE', #45777, #16091 ) ;
#30752=CARTESIAN_POINT ( 'NONE',  ( -11.61908885153752813, -23.53148341178916425, 53.49999999999995026 ) ) ;
#30753=ADVANCED_FACE ( 'NONE', ( #40680 ), #12187, .T. ) ;
#30755=CARTESIAN_POINT ( 'NONE',  ( -17.92193035392797285, -21.84160718002658541, 61.87535923543196503 ) ) ;
#30758=CARTESIAN_POINT ( 'NONE',  ( -10.13055098088643646, -13.29041361134464516, 74.82817645606137091 ) ) ;
#30759=CARTESIAN_POINT ( 'NONE',  ( -11.17827002090033339, -11.53132166989810337, 71.38860948999864320 ) ) ;
#30761=CARTESIAN_POINT ( 'NONE',  ( -12.10369346210734243, -9.594120923840563364, 57.27430859790474926 ) ) ;
#30762=( BOUNDED_CURVE ( )  B_SPLINE_CURVE ( 3, ( #23172, #762, #15756, #26618 ),
 .UNSPECIFIED., .F., .F. ) 
 B_SPLINE_CURVE_WITH_KNOTS ( ( 4, 4 ),
 ( 0.9074455897393695070, 1.000000000000000000 ),
 .UNSPECIFIED. ) 
 CURVE ( )  GEOMETRIC_REPRESENTATION_ITEM ( )  RATIONAL_B_SPLINE_CURVE ( ( 0.6983129098261110501, 0.7760317562607137454, 0.8765941196520100620, 1.000000000000000000 ) ) 
 REPRESENTATION_ITEM ( '' )  );
#30763=EDGE_CURVE ( 'NONE', #26171, #42055, #24429, .T. ) ;
#30764=CARTESIAN_POINT ( 'NONE',  ( -12.64139926011484505, -9.624549101048229360, 74.31922783352578676 ) ) ;
#30766=ORIENTED_EDGE ( 'NONE', *, *, #23237, .T. ) ;
#30769=CARTESIAN_POINT ( 'NONE',  ( -13.71339271347209987, -20.80363700974685059, 65.28628881287177421 ) ) ;
#30773=CARTESIAN_POINT ( 'NONE',  ( -20.31649760022732565, -7.943510736669368910, 70.43595667626200907 ) ) ;
#30774=CARTESIAN_POINT ( 'NONE',  ( -12.49855684652675514, -19.85736664535339813, 68.75146050727752822 ) ) ;
#30775=CARTESIAN_POINT ( 'NONE',  ( -23.30282546666849086, -18.60927426030231047, 69.59371984657600763 ) ) ;
#30776=CARTESIAN_POINT ( 'NONE',  ( -20.37299750454370439, -8.405577324698720432, 66.78104082189589974 ) ) ;
#30777=VERTEX_POINT ( 'NONE', #34755 ) ;
#30778=AXIS2_PLACEMENT_3D ( 'NONE', #43559, #9820, #39113 ) ;
#30779=CARTESIAN_POINT ( 'NONE',  ( -22.62394951084894146, -10.04809318868971424, 70.29706442286226320 ) ) ;
#30781=CARTESIAN_POINT ( 'NONE',  ( -10.02907021082448225, -13.90480008044668381, 57.57012250139395348 ) ) ;
#30782=CARTESIAN_POINT ( 'NONE',  ( -21.95939004544374740, -9.477125498926222136, 59.72171213236985921 ) ) ;
#30783=EDGE_CURVE ( 'NONE', #35674, #38958, #27162, .T. ) ;
#30786=EDGE_CURVE ( 'NONE', #21625, #30729, #138, .T. ) ;
#30787=VERTEX_POINT ( 'NONE', #27613 ) ;
#30788=EDGE_CURVE ( 'NONE', #26955, #17516, #16517, .T. ) ;
#30790=CARTESIAN_POINT ( 'NONE',  ( -23.12302657392458016, -18.95946740514217765, 62.35406880581414413 ) ) ;
#30791=CARTESIAN_POINT ( 'NONE',  ( -15.49415775405465823, -8.028509947901662613, 74.37985659017797957 ) ) ;
#30792=CARTESIAN_POINT ( 'NONE',  ( -16.78411603780843464, -21.83009879966275690, 68.84560651669730191 ) ) ;
#30793=EDGE_LOOP ( 'NONE', ( #22623, #16500, #10671, #4025, #42172 ) ) ;
#30794=CARTESIAN_POINT ( 'NONE',  ( -13.02800473326296782, -9.361643555834115560, 70.84925385331725067 ) ) ;
#30797=CARTESIAN_POINT ( 'NONE',  ( -11.49500183448703083, -10.99442376238782337, 57.22375354680192316 ) ) ;
#30799=ORIENTED_EDGE ( 'NONE', *, *, #27890, .T. ) ;
#30801=ORIENTED_EDGE ( 'NONE', *, *, #9875, .F. ) ;
#30802=DIRECTION ( 'NONE',  ( 0.2479245821708770392, 0.9687793358424796608, -9.885672099568309358E-17 ) ) ;
#30805=B_SPLINE_CURVE_WITH_KNOTS ( 'NONE', 3,
 ( #25672, #37223, #18772, #29868, #21986, #44182, #29616, #36727, #18517, #3015 ),
 .UNSPECIFIED., .F., .F.,
 ( 4, 2, 2, 2, 4 ),
 ( 0.000000000000000000, 0.2500000000000000000, 0.5000000000000000000, 0.7500000000000000000, 1.000000000000000000 ),
 .UNSPECIFIED. ) ;
#30806=ORIENTED_EDGE ( 'NONE', *, *, #45577, .T. ) ;
#30807=CARTESIAN_POINT ( 'NONE',  ( -24.42608592195226080, -15.63182493645487803, 73.00863554951556011 ) ) ;
#30810=VECTOR ( 'NONE', #8517, 1000.000000000000114 ) ;
#30811=LINE ( 'NONE', #34228, #2390 ) ;
#30812=B_SPLINE_CURVE_WITH_KNOTS ( 'NONE', 1,
 ( #29353, #36703 ),
 .UNSPECIFIED., .F., .F.,
 ( 2, 2 ),
 ( 0.000000000000000000, 1.000000000000000000 ),
 .UNSPECIFIED. ) ;
#30814=FACE_OUTER_BOUND ( 'NONE', #35467, .T. ) ;
#30815=ORIENTED_EDGE ( 'NONE', *, *, #30870, .T. ) ;
#30816=CARTESIAN_POINT ( 'NONE',  ( -23.74619244455239198, -11.68933966055485207, 63.25218278636740621 ) ) ;
#30819=EDGE_CURVE ( 'NONE', #27387, #11362, #29438, .T. ) ;
#30820=DIRECTION ( 'NONE',  ( -0.3478314405900307382, -0.9375570856950865561, 0.000000000000000000 ) ) ;
#30821=PLANE ( 'NONE',  #21635 ) ;
#30823=VERTEX_POINT ( 'NONE', #8416 ) ;
#30824=EDGE_CURVE ( 'NONE', #26563, #4162, #43661, .T. ) ;
#30825=CARTESIAN_POINT ( 'NONE',  ( -21.44791994599160034, -9.079744384496041931, 73.67299128577275269 ) ) ;
#30826=CARTESIAN_POINT ( 'NONE',  ( -10.36101939589240573, -12.43898124111679948, 60.96000069308703928 ) ) ;
#30827=ORIENTED_EDGE ( 'NONE', *, *, #35148, .F. ) ;
#30828=CARTESIAN_POINT ( 'NONE',  ( -20.99769161626881697, -21.34631032816609064, 62.29284164739992491 ) ) ;
#30830=CARTESIAN_POINT ( 'NONE',  ( -16.29760673242258306, -22.17363489859456038, 61.87072740723333197 ) ) ;
#30833=CARTESIAN_POINT ( 'NONE',  ( -14.28913779072144230, -8.050817036395716997, 67.37479760520351135 ) ) ;
#30834=CARTESIAN_POINT ( 'NONE',  ( -11.32173637914110742, -11.26291225165672927, 67.76297573134488061 ) ) ;
#30837=CARTESIAN_POINT ( 'NONE',  ( -24.39508262754368317, -15.44650746503438654, 73.07591740786084245 ) ) ;
#30839=CARTESIAN_POINT ( 'NONE',  ( -22.86572475812252847, -14.01004878893095196, 54.07175714974878389 ) ) ;
#30841=CARTESIAN_POINT ( 'NONE',  ( -21.03507683653377924, -21.32559370058661585, 62.26471398792010348 ) ) ;
#30842=CARTESIAN_POINT ( 'NONE',  ( -12.36648897341435749, -9.886239853951966694, 64.17347106801278755 ) ) ;
#30843=CARTESIAN_POINT ( 'NONE',  ( -14.80261111872947133, -21.30118156454888734, 61.70770622945212125 ) ) ;
#30844=EDGE_CURVE ( 'NONE', #31661, #37124, #42882, .T. ) ;
#30846=ORIENTED_EDGE ( 'NONE', *, *, #5904, .F. ) ;
#30848=ORIENTED_EDGE ( 'NONE', *, *, #48070, .F. ) ;
#30849=EDGE_CURVE ( 'NONE', #40867, #23333, #17780, .T. ) ;
#30856=CARTESIAN_POINT ( 'NONE',  ( -16.23868518553448936, -7.453991501053678803, 60.32311612641502307 ) ) ;
#30857=CARTESIAN_POINT ( 'NONE',  ( -13.70631631145106155, -20.74045196213498343, 64.98628931290484445 ) ) ;
#30858=CARTESIAN_POINT ( 'NONE',  ( -17.18480517372767125, -21.85814792571105514, 72.05054515682328997 ) ) ;
#30860=CARTESIAN_POINT ( 'NONE',  ( -23.16117746674104438, -18.90708040007733359, 62.63934749780565880 ) ) ;
#30861=CARTESIAN_POINT ( 'NONE',  ( -24.22092373047179947, -12.93688097883364208, 66.30246741375938768 ) ) ;
#30864=CARTESIAN_POINT ( 'NONE',  ( -12.20856039377037128, -20.12912213554072238, 64.97400716046928437 ) ) ;
#30865=EDGE_LOOP ( 'NONE', ( #11520, #10473 ) ) ;
#30866=LINE ( 'NONE', #1051, #29164 ) ;
#30867=CARTESIAN_POINT ( 'NONE',  ( -24.01421620325079331, -12.44888360987459741, 73.31513625682875102 ) ) ;
#30868=ORIENTED_EDGE ( 'NONE', *, *, #8780, .T. ) ;
#30869=CARTESIAN_POINT ( 'NONE',  ( -23.24383905832493014, -10.15805014756499070, 63.17211752265900060 ) ) ;
#30870=EDGE_CURVE ( 'NONE', #7306, #27306, #47136, .T. ) ;
#30872=FACE_OUTER_BOUND ( 'NONE', #34690, .T. ) ;
#30873=CARTESIAN_POINT ( 'NONE',  ( -24.36630790243135181, -13.91161852910999031, 73.23157508594482579 ) ) ;
#30874=CARTESIAN_POINT ( 'NONE',  ( -11.29134393598116937, -11.33126488396075260, 64.16354160640879911 ) ) ;
#30882=CARTESIAN_POINT ( 'NONE',  ( -10.47696978178682414, -17.50027494739433820, 64.80456292574326937 ) ) ;
#30884=DIRECTION ( 'NONE',  ( -0.3303050442826436783, 0.9438742382973703826, 3.829623549872328964E-09 ) ) ;
#30885=CARTESIAN_POINT ( 'NONE',  ( -10.62494255334146231, -17.85455924901271629, 71.76706980444858175 ) ) ;
#30887=CARTESIAN_POINT ( 'NONE',  ( -13.47245400663725690, -21.12492667118925382, 65.10133491818508844 ) ) ;
#30888=( BOUNDED_CURVE ( )  B_SPLINE_CURVE ( 3, ( #44224, #2347, #25250, #17357 ),
 .UNSPECIFIED., .F., .F. ) 
 B_SPLINE_CURVE_WITH_KNOTS ( ( 4, 4 ),
 ( 0.4074455897393634562, 0.5000000000000000000 ),
 .UNSPECIFIED. ) 
 CURVE ( )  GEOMETRIC_REPRESENTATION_ITEM ( )  RATIONAL_B_SPLINE_CURVE ( ( 0.6983129098261030565, 0.7760317562607105257, 0.8765941196520107281, 1.000000000000005995 ) ) 
 REPRESENTATION_ITEM ( '' )  );
#30889=EDGE_LOOP ( 'NONE', ( #45044, #26998 ) ) ;
#30890=FACE_OUTER_BOUND ( 'NONE', #27184, .T. ) ;
#30891=CARTESIAN_POINT ( 'NONE',  ( -11.96084906401204506, -9.743958800322932490, 60.74413413563605957 ) ) ;
#30892=ORIENTED_EDGE ( 'NONE', *, *, #4007, .F. ) ;
#30893=CARTESIAN_POINT ( 'NONE',  ( -24.17899325218984785, -11.66673737571591296, 59.66731058339561855 ) ) ;
#30895=B_SPLINE_CURVE_WITH_KNOTS ( 'NONE', 1,
 ( #29766, #40838 ),
 .UNSPECIFIED., .F., .F.,
 ( 2, 2 ),
 ( 0.000000000000000000, 1.000000000000000000 ),
 .UNSPECIFIED. ) ;
#30898=( BOUNDED_CURVE ( )  B_SPLINE_CURVE ( 3, ( #26647, #41908, #34254, #41662 ),
 .UNSPECIFIED., .F., .F. ) 
 B_SPLINE_CURVE_WITH_KNOTS ( ( 4, 4 ),
 ( 0.000000000000000000, 0.4074455897393689519 ),
 .UNSPECIFIED. ) 
 CURVE ( )  GEOMETRIC_REPRESENTATION_ITEM ( )  RATIONAL_B_SPLINE_CURVE ( ( 1.000000000000000000, 0.4567392136813275272, 0.3561768502900286570, 0.6983129098261033896 ) ) 
 REPRESENTATION_ITEM ( '' )  );
#30899=VERTEX_POINT ( 'NONE', #13540 ) ;
#30900=ORIENTED_EDGE ( 'NONE', *, *, #28571, .F. ) ;
#30906=CARTESIAN_POINT ( 'NONE',  ( -20.50783493979771421, -8.027295371342848540, 66.96599508560271374 ) ) ;
#30907=( BOUNDED_SURFACE ( )  B_SPLINE_SURFACE ( 3, 1, ( 
 ( #3337, #11456 ),
 ( #34335, #41014 ),
 ( #33596, #15133 ),
 ( #387, #22057 ),
 ( #37290, #41495 ),
 ( #33347, #26479 ),
 ( #623, #7296 ) ),
 .UNSPECIFIED., .T., .F., .F. ) 
 B_SPLINE_SURFACE_WITH_KNOTS ( ( 4, 3, 4 ),
 ( 2, 2 ),
 ( 0.000000000000000000, 0.5000000000000000000, 1.000000000000000000 ),
 ( 0.000000000000000000, 1.000000000000000000 ),
 .UNSPECIFIED. ) 
 GEOMETRIC_REPRESENTATION_ITEM ( )  RATIONAL_B_SPLINE_SURFACE ( (
 ( 1.000000000000000000, 1.000000000000000000),
 ( 0.3333333333333335369, 0.3333333333333330373),
 ( 0.3333333333333335369, 0.3333333333333330373),
 ( 1.000000000000000000, 1.000000000000000000),
 ( 0.3333333333333333703, 0.3333333333333333703),
 ( 0.3333333333333333703, 0.3333333333333333703),
 ( 1.000000000000000000, 1.000000000000000000) ) ) 
 REPRESENTATION_ITEM ( '' )  SURFACE ( )  );
#30908=EDGE_CURVE ( 'NONE', #37344, #21796, #3695, .T. ) ;
#30910=DIRECTION ( 'NONE',  ( 0.9986807914369957295, -0.05134858142905001505, 1.286972170232539807E-09 ) ) ;
#30911=FACE_OUTER_BOUND ( 'NONE', #19702, .T. ) ;
#30912=CARTESIAN_POINT ( 'NONE',  ( -20.06975372951847447, -8.274133229585533655, 73.73568642813194174 ) ) ;
#30914=ORIENTED_EDGE ( 'NONE', *, *, #15800, .F. ) ;
#30915=CARTESIAN_POINT ( 'NONE',  ( -22.34470984022960138, -19.78791505225649416, 69.17417989488706098 ) ) ;
#30916=CARTESIAN_POINT ( 'NONE',  ( -24.26646706006808429, -13.09550643046007679, 59.36267627158827764 ) ) ;
#30917=VERTEX_POINT ( 'NONE', #39660 ) ;
#30920=ORIENTED_EDGE ( 'NONE', *, *, #41119, .T. ) ;
#30921=CARTESIAN_POINT ( 'NONE',  ( -12.40538999107997498, -20.31523868419091272, 68.52152871938794476 ) ) ;
#30922=EDGE_CURVE ( 'NONE', #545, #13505, #43612, .T. ) ;
#30924=CARTESIAN_POINT ( 'NONE',  ( -18.25645571269274825, -21.81792545032241293, 62.03103110229211836 ) ) ;
#30925=CARTESIAN_POINT ( 'NONE',  ( -20.17268404433175633, -8.371407854712250796, 70.55100341248845552 ) ) ;
#30926=CARTESIAN_POINT ( 'NONE',  ( -20.86898800509773011, -8.203323387673732370, 59.97978722081754199 ) ) ;
#30927=ORIENTED_EDGE ( 'NONE', *, *, #25971, .F. ) ;
#30932=PRODUCT_CONTEXT ( 'NONE', #8652, 'mechanical' ) ;
#30933=CARTESIAN_POINT ( 'NONE',  ( -22.11655536972627090, -20.00359415806959618, 62.51973814734046186 ) ) ;
#30934=CARTESIAN_POINT ( 'NONE',  ( -10.55057756800719737, -16.13619752454317791, 71.46367081720265446 ) ) ;
#30936=DIRECTION ( 'NONE',  ( -2.515467001362780054E-08, -7.569581535656660169E-10, 0.9999999999999996669 ) ) ;
#30939=ORIENTED_EDGE ( 'NONE', *, *, #19621, .F. ) ;
#30940=FACE_OUTER_BOUND ( 'NONE', #8886, .T. ) ;
#30941=CARTESIAN_POINT ( 'NONE',  ( -22.93319280244040570, -10.48995202115733605, 63.35569470095123279 ) ) ;
#30944=FACE_BOUND ( 'NONE', #33424, .T. ) ;
#30945=ORIENTED_EDGE ( 'NONE', *, *, #24625, .F. ) ;
#30946=ORIENTED_EDGE ( 'NONE', *, *, #14278, .T. ) ;
#30948=CARTESIAN_POINT ( 'NONE',  ( -17.98584054083101691, -22.23808389992613499, 62.06031238270200845 ) ) ;
#30949=LINE ( 'NONE', #19864, #27426 ) ;
#30951=CARTESIAN_POINT ( 'NONE',  ( -14.48363552191318604, -8.456628570761285602, 67.25975083097569041 ) ) ;
#30952=CARTESIAN_POINT ( 'NONE',  ( -11.86838291625971742, -9.845553222893467904, 64.14418898700822069 ) ) ;
#30953=CARTESIAN_POINT ( 'NONE',  ( -19.36486170040678090, -8.083171235113246311, 60.24476463208835497 ) ) ;
#30958=CARTESIAN_POINT ( 'NONE',  ( -11.86269392149798207, -9.851982632420845931, 64.22252622837828540 ) ) ;
#30959=DIRECTION ( 'NONE',  ( 0.2664710960620865210, -0.9638429098994647504, 4.833213314675751572E-08 ) ) ;
#30960=CARTESIAN_POINT ( 'NONE',  ( -20.60788153932096023, -8.518722016582882972, 63.32593600985608617 ) ) ;
#30963=EDGE_CURVE ( 'NONE', #16796, #41098, #20478, .T. ) ;
#30964=ORIENTED_EDGE ( 'NONE', *, *, #44965, .F. ) ;
#30965=FACE_OUTER_BOUND ( 'NONE', #34396, .T. ) ;
#30967=EDGE_CURVE ( 'NONE', #45444, #44359, #4843, .T. ) ;
#30968=DIRECTION ( 'NONE',  ( -5.731567514496413899E-31, -1.020425574103664789E-16, -1.000000000000000000 ) ) ;
#30970=ORIENTED_EDGE ( 'NONE', *, *, #25020, .F. ) ;
#30972=CARTESIAN_POINT ( 'NONE',  ( -10.42773860147015519, -14.58150043490377179, 67.87302585467796234 ) ) ;
#30975=CARTESIAN_POINT ( 'NONE',  ( -15.15107538838304002, -21.43001499838511847, 65.40596678908117667 ) ) ;
#30976=CARTESIAN_POINT ( 'NONE',  ( -17.06206538396918404, -7.760525543569854356, 67.17606901500077754 ) ) ;
#30977=CARTESIAN_POINT ( 'NONE',  ( -11.39842353126723218, -18.37420439508194647, 61.50540784843255437 ) ) ;
#30978=EDGE_LOOP ( 'NONE', ( #36556, #10389 ) ) ;
#30979=FACE_OUTER_BOUND ( 'NONE', #33129, .T. ) ;
#30981=CARTESIAN_POINT ( 'NONE',  ( -19.18081468460184524, -7.569236297829234239, 63.53750910235358873 ) ) ;
#30982=CARTESIAN_POINT ( 'NONE',  ( -15.28630342961327138, -8.082779564739171363, 56.99432743296591042 ) ) ;
#30983=ORIENTED_EDGE ( 'NONE', *, *, #48669, .F. ) ;
#30984=CARTESIAN_POINT ( 'NONE',  ( -10.90759836534377492, -17.49952001658422063, 68.39721944423101263 ) ) ;
#30986=CARTESIAN_POINT ( 'NONE',  ( -14.23218538299976643, -8.077567926792571740, 67.36636790937856745 ) ) ;
#30987=ORIENTED_EDGE ( 'NONE', *, *, #46542, .F. ) ;
#30989=CARTESIAN_POINT ( 'NONE',  ( -20.96474559848019226, -20.91483931500396309, 58.80042297414523489 ) ) ;
#30990=CARTESIAN_POINT ( 'NONE',  ( -14.01118748589247964, -10.49619482288619565, 53.49899999999994549 ) ) ;
#30991=CARTESIAN_POINT ( 'NONE',  ( -11.95607289622835978, -9.749060919267328984, 60.68105355187064021 ) ) ;
#30992=VERTEX_POINT ( 'NONE', #3685 ) ;
#30993=CARTESIAN_POINT ( 'NONE',  ( -11.43875873011815258, -18.53463696397233207, 61.57710806188755015 ) ) ;
#30995=ORIENTED_EDGE ( 'NONE', *, *, #26264, .F. ) ;
#30996=ORIENTED_EDGE ( 'NONE', *, *, #46225, .F. ) ;
#30997=CARTESIAN_POINT ( 'NONE',  ( -22.78465755717926555, -10.30744034590000346, 66.84182281441593432 ) ) ;
#30998=CARTESIAN_POINT ( 'NONE',  ( -10.54994933093899867, -13.24305344519376959, 71.49356453765415154 ) ) ;
#31002=EDGE_CURVE ( 'NONE', #48717, #31810, #3074, .T. ) ;
#31003=CARTESIAN_POINT ( 'NONE',  ( -11.89178903705324863, -10.43929771899554737, 71.26893105542536944 ) ) ;
#31005=CARTESIAN_POINT ( 'NONE',  ( -10.53028993777715883, -16.28642212234895226, 71.73278239416407587 ) ) ;
#31006=VERTEX_POINT ( 'NONE', #21911 ) ;
#31007=ORIENTED_EDGE ( 'NONE', *, *, #10375, .T. ) ;
#31008=CARTESIAN_POINT ( 'NONE',  ( -22.98758735661991892, -9.854289139077749837, 70.26824437992965500 ) ) ;
#31010=CARTESIAN_POINT ( 'NONE',  ( -14.54176669294802693, -21.67913874359843973, 58.28122557424108408 ) ) ;
#31012=CARTESIAN_POINT ( 'NONE',  ( -18.83428564917659287, -7.493810079819247072, 70.62713979963420741 ) ) ;
#31016=CARTESIAN_POINT ( 'NONE',  ( -10.53692143227921818, -11.79390935372226323, 53.76227901944321985 ) ) ;
#31017=EDGE_CURVE ( 'NONE', #32391, #37778, #46535, .T. ) ;
#31018=CARTESIAN_POINT ( 'NONE',  ( -14.92237289681681034, -21.82673989507453882, 65.22879770143127587 ) ) ;
#31019=DIRECTION ( 'NONE',  ( -0.9796876409582463419, 0.2005296141562636081, 7.890952370353029293E-08 ) ) ;
#31020=ADVANCED_FACE ( 'NONE', ( #257 ), #33212, .T. ) ;
#31021=( BOUNDED_CURVE ( )  B_SPLINE_CURVE ( 3, ( #25278, #20852, #1894, #35851 ),
 .UNSPECIFIED., .F., .F. ) 
 B_SPLINE_CURVE_WITH_KNOTS ( ( 4, 4 ),
 ( 0.9074455897393649551, 1.000000000000000000 ),
 .UNSPECIFIED. ) 
 CURVE ( )  GEOMETRIC_REPRESENTATION_ITEM ( )  RATIONAL_B_SPLINE_CURVE ( ( 0.6983129098260929535, 0.7760317562606982023, 0.8765941196520005141, 1.000000000000000000 ) ) 
 REPRESENTATION_ITEM ( '' )  );
#31022=ORIENTED_EDGE ( 'NONE', *, *, #16207, .F. ) ;
#31023=CARTESIAN_POINT ( 'NONE',  ( -10.55755145186731880, -16.16957250319292072, 68.16870912284423412 ) ) ;
#31025=EDGE_CURVE ( 'NONE', #18851, #48127, #9041, .T. ) ;
#31028=ORIENTED_EDGE ( 'NONE', *, *, #30212, .T. ) ;
#31029=FACE_OUTER_BOUND ( 'NONE', #39264, .T. ) ;
#31031=CARTESIAN_POINT ( 'NONE',  ( -13.89433361489564156, -8.703010632355098863, 74.08466061421664506 ) ) ;
#31033=CARTESIAN_POINT ( 'NONE',  ( -23.65353884516659733, -18.89565076926976062, 69.43338659176652072 ) ) ;
#31034=ADVANCED_FACE ( 'NONE', ( #48017 ), #37149, .T. ) ;
#31035=( BOUNDED_SURFACE ( )  B_SPLINE_SURFACE ( 3, 1, ( 
 ( #23378, #31249 ),
 ( #19688, #1444 ),
 ( #26838, #34699 ),
 ( #42337, #8858 ),
 ( #973, #46033 ),
 ( #38879, #31012 ),
 ( #15969, #12290 ) ),
 .UNSPECIFIED., .T., .F., .F. ) 
 B_SPLINE_SURFACE_WITH_KNOTS ( ( 4, 3, 4 ),
 ( 2, 2 ),
 ( 0.000000000000000000, 0.5000000000000000000, 1.000000000000000000 ),
 ( 0.000000000000000000, 1.000000000000000000 ),
 .UNSPECIFIED. ) 
 GEOMETRIC_REPRESENTATION_ITEM ( )  RATIONAL_B_SPLINE_SURFACE ( (
 ( 1.000000000000000000, 1.000000000000000000),
 ( 0.3333333333333335369, 0.3333333333333330373),
 ( 0.3333333333333335369, 0.3333333333333330373),
 ( 1.000000000000000000, 1.000000000000000000),
 ( 0.3333333333333333703, 0.3333333333333333703),
 ( 0.3333333333333333703, 0.3333333333333333703),
 ( 1.000000000000000000, 1.000000000000000000) ) ) 
 REPRESENTATION_ITEM ( '' )  SURFACE ( )  );
#31037=FACE_OUTER_BOUND ( 'NONE', #6746, .T. ) ;
#31039=VERTEX_POINT ( 'NONE', #3437 ) ;
#31040=CARTESIAN_POINT ( 'NONE',  ( -24.01844669341070926, -17.32505205508840262, 62.62928254837112974 ) ) ;
#31043=CARTESIAN_POINT ( 'NONE',  ( -21.38436113231072966, -21.11942757641454094, 69.25461391254337684 ) ) ;
#31044=CARTESIAN_POINT ( 'NONE',  ( -22.21294348278119912, -9.102026181049186704, 59.86024708057400545 ) ) ;
#31045=CARTESIAN_POINT ( 'NONE',  ( -21.73662441638723308, -9.231682010981758779, 66.67622112302015580 ) ) ;
#31046=ORIENTED_EDGE ( 'NONE', *, *, #11857, .F. ) ;
#31047=DIRECTION ( 'NONE',  ( 0.8810891847886932471, 0.4615090133018354690, 0.1033986416233890065 ) ) ;
#31050=CARTESIAN_POINT ( 'NONE',  ( -24.76413943691219899, -16.08518182373101624, 66.18608065020819708 ) ) ;
#31053=LINE ( 'NONE', #42636, #45595 ) ;
#31054=CARTESIAN_POINT ( 'NONE',  ( -24.33896800083871526, -16.20181617365279791, 66.36325218972963569 ) ) ;
#31055=VERTEX_POINT ( 'NONE', #18205 ) ;
#31058=CARTESIAN_POINT ( 'NONE',  ( -10.28759036655602976, -12.67074725465185203, 64.36861864226402474 ) ) ;
#31059=CARTESIAN_POINT ( 'NONE',  ( -18.72681101482837818, -7.880611649715417499, 70.37068030201731972 ) ) ;
#31060=EDGE_CURVE ( 'NONE', #11637, #29328, #15918, .T. ) ;
#31061=FACE_OUTER_BOUND ( 'NONE', #33964, .T. ) ;
#31062=CARTESIAN_POINT ( 'NONE',  ( -15.82706267189338689, -7.992506172297358269, 70.83819797924105899 ) ) ;
#31066=CARTESIAN_POINT ( 'NONE',  ( -22.48562329102781021, -19.71690596984645438, 72.64960304871698327 ) ) ;
#31068=CARTESIAN_POINT ( 'NONE',  ( -14.11566384109317873, -8.583543149139638118, 74.20514413324690395 ) ) ;
#31070=ORIENTED_EDGE ( 'NONE', *, *, #15183, .T. ) ;
#31071=EDGE_LOOP ( 'NONE', ( #7175, #8346, #15840, #20562, #3377 ) ) ;
#31072=B_SPLINE_CURVE_WITH_KNOTS ( 'NONE', 3,
 ( #15410, #22845, #42273, #431, #37838, #4132, #8537, #23566, #22583, #19869 ),
 .UNSPECIFIED., .F., .F.,
 ( 4, 2, 2, 2, 4 ),
 ( 0.1272669073658287964, 0.2522669073463161826, 0.3772669073268035689, 0.5022669073072909551, 0.6272669072877783414 ),
 .UNSPECIFIED. ) ;
#31074=CARTESIAN_POINT ( 'NONE',  ( -11.14016733508048240, -18.81244675540447631, 64.93362470803228348 ) ) ;
#31075=VERTEX_POINT ( 'NONE', #25601 ) ;
#31076=CARTESIAN_POINT ( 'NONE',  ( -10.43244321615298809, -14.46516663507775213, 68.15800133269522121 ) ) ;
#31078=DIRECTION ( 'NONE',  ( -0.3478314405900310158, -0.9375570856950865561, 1.977132801529374134E-16 ) ) ;
#31079=ORIENTED_EDGE ( 'NONE', *, *, #24296, .F. ) ;
#31081=CARTESIAN_POINT ( 'NONE',  ( -13.83108396514174565, -21.33561889020367630, 72.04112409899799729 ) ) ;
#31082=EDGE_CURVE ( 'NONE', #39506, #17461, #27861, .T. ) ;
#31083=CARTESIAN_POINT ( 'NONE',  ( -21.63336539757928634, -9.153348366551478321, 66.94677872351418557 ) ) ;
#31086=B_SPLINE_CURVE_WITH_KNOTS ( 'NONE', 3,
 ( #45945, #12205, #27226, #5308, #42252, #8512, #27466, #42498, #4339, #23544 ),
 .UNSPECIFIED., .F., .F.,
 ( 4, 2, 2, 2, 4 ),
 ( 0.000000000000000000, 0.2500000000000000000, 0.5000000000000000000, 0.7500000000000000000, 1.000000000000000000 ),
 .UNSPECIFIED. ) ;
#31087=VECTOR ( 'NONE', #43490, 1000.000000000000000 ) ;
#31088=ORIENTED_EDGE ( 'NONE', *, *, #20495, .F. ) ;
#31089=CARTESIAN_POINT ( 'NONE',  ( -24.53780051168580911, -12.59584816521350348, 69.95738404390658616 ) ) ;
#31090=CARTESIAN_POINT ( 'NONE',  ( -17.17561717955991085, -7.363342535065456218, 70.69024626294222458 ) ) ;
#31091=EDGE_LOOP ( 'NONE', ( #11969, #31446, #6907, #19398, #39399 ) ) ;
#31092=CARTESIAN_POINT ( 'NONE',  ( -10.43125849979191955, -13.91324152291312188, 57.74825034919034294 ) ) ;
#31096=CARTESIAN_POINT ( 'NONE',  ( -11.60006209888454443, -10.16330164164447325, 71.08397698276321819 ) ) ;
#31097=CARTESIAN_POINT ( 'NONE',  ( -20.95545100651803594, -20.91135505560678709, 65.59926067308570907 ) ) ;
#31100=EDGE_CURVE ( 'NONE', #15096, #4739, #23877, .T. ) ;
#31101=CARTESIAN_POINT ( 'NONE',  ( -14.37682202087475680, -19.38786730597468022, 54.07175714974878389 ) ) ;
#31102=DIRECTION ( 'NONE',  ( 2.671295499615842957E-06, 1.272698189891367967E-05, 0.9999999999154439712 ) ) ;
#31103=CARTESIAN_POINT ( 'NONE',  ( -21.01123855637963089, -20.87838213191899683, 65.58453944497207999 ) ) ;
#31104=EDGE_CURVE ( 'NONE', #43248, #47012, #20961, .T. ) ;
#31105=EDGE_CURVE ( 'NONE', #8440, #14865, #840, .T. ) ;
#31107=ORIENTED_EDGE ( 'NONE', *, *, #18273, .T. ) ;
#31108=CARTESIAN_POINT ( 'NONE',  ( -21.66487278515026915, -9.172785956992999701, 63.39973619028431528 ) ) ;
#31109=CARTESIAN_POINT ( 'NONE',  ( -10.45152819156127144, -17.43344342502064848, 64.73465214939118084 ) ) ;
#31111=B_SPLINE_CURVE_WITH_KNOTS ( 'NONE', 3,
 ( #20035, #9694, #24711, #12396, #19803, #16074, #34805, #1075, #24475, #5259 ),
 .UNSPECIFIED., .F., .F.,
 ( 4, 2, 2, 2, 4 ),
 ( 0.000000000000000000, 0.2500000000000000000, 0.5000000000000000000, 0.7500000000000000000, 1.000000000000000000 ),
 .UNSPECIFIED. ) ;
#31112=LINE ( 'NONE', #24213, #14240 ) ;
#31113=CARTESIAN_POINT ( 'NONE',  ( -21.59804090337381410, -20.98026344205569771, 72.70941702861115630 ) ) ;
#31114=CARTESIAN_POINT ( 'NONE',  ( -23.26195008415477972, -10.18062560903149638, 63.24998768291849416 ) ) ;
#31116=VERTEX_POINT ( 'NONE', #35173 ) ;
#31117=CARTESIAN_POINT ( 'NONE',  ( -23.76773515637538736, -11.84597937754909935, 63.06291311429629332 ) ) ;
#31118=B_SPLINE_CURVE_WITH_KNOTS ( 'NONE', 3,
 ( #39363, #20419, #17171, #27555, #31247, #42595, #31972, #8856, #46989, #39842 ),
 .UNSPECIFIED., .F., .F.,
 ( 4, 2, 2, 2, 4 ),
 ( 0.000000000000000000, 0.2500000000000000000, 0.5000000000000000000, 0.7500000000000000000, 1.000000000000000000 ),
 .UNSPECIFIED. ) ;
#31119=CARTESIAN_POINT ( 'NONE',  ( -23.99312268326606201, -11.29471679256767125, 66.60709928216182618 ) ) ;
#31121=CARTESIAN_POINT ( 'NONE',  ( -17.13503149044196405, -7.764836982087095052, 70.77563787455143540 ) ) ;
#31123=CARTESIAN_POINT ( 'NONE',  ( -10.00731251637046881, -14.10555026099538978, 61.10316585833331260 ) ) ;
#31125=VERTEX_POINT ( 'NONE', #22911 ) ;
#31126=EDGE_LOOP ( 'NONE', ( #42745, #46753, #34279, #38086, #24920 ) ) ;
#31128=ADVANCED_FACE ( 'NONE', ( #27310 ), #31035, .T. ) ;
#31129=CARTESIAN_POINT ( 'NONE',  ( -22.99825578621637590, -9.866157890886050552, 70.15145146949444666 ) ) ;
#31130=CARTESIAN_POINT ( 'NONE',  ( -15.48628188820593543, -7.614865071177022493, 74.26641013817956605 ) ) ;
#31133=CARTESIAN_POINT ( 'NONE',  ( -20.47364665458772848, -8.506973655552112490, 67.00933899976185160 ) ) ;
#31134=ADVANCED_FACE ( 'NONE', ( #8131 ), #19929, .T. ) ;
#31135=CARTESIAN_POINT ( 'NONE',  ( -18.85724798917316392, -7.906108138700305155, 67.18599644112759961 ) ) ;
#31136=CARTESIAN_POINT ( 'NONE',  ( -24.39403741458288266, -17.44049236422942784, 69.52844466935830781 ) ) ;
#31137=ORIENTED_EDGE ( 'NONE', *, *, #3796, .T. ) ;
#31138=CARTESIAN_POINT ( 'NONE',  ( -21.25294243521737059, -20.66975681891597816, 72.80829934587789865 ) ) ;
#31139=CARTESIAN_POINT ( 'NONE',  ( -24.31482381427648676, -13.31912605980313735, 59.36267924676594987 ) ) ;
#31141=CARTESIAN_POINT ( 'NONE',  ( -13.31679730094617575, -21.02473588039183028, 61.61672084944926553 ) ) ;
#31142=CARTESIAN_POINT ( 'NONE',  ( -24.25171796977671335, -16.35308120058899206, 59.42332432118549690 ) ) ;
#31143=ORIENTED_EDGE ( 'NONE', *, *, #33585, .F. ) ;
#31144=CARTESIAN_POINT ( 'NONE',  ( -15.39536932222403287, -19.92137602241599836, 53.49899999999994549 ) ) ;
#31146=( BOUNDED_CURVE ( )  B_SPLINE_CURVE ( 3, ( #35781, #31861, #46881, #39248 ),
 .UNSPECIFIED., .F., .F. ) 
 B_SPLINE_CURVE_WITH_KNOTS ( ( 4, 4 ),
 ( 1.570796326794896780, 1.675516081914553590 ),
 .UNSPECIFIED. ) 
 CURVE ( )  GEOMETRIC_REPRESENTATION_ITEM ( )  RATIONAL_B_SPLINE_CURVE ( ( 1.000000000000000000, 0.9990863565030492222, 0.9990863565030492222, 1.000000000000000000 ) ) 
 REPRESENTATION_ITEM ( '' )  );
#31147=CARTESIAN_POINT ( 'NONE',  ( -10.33213862838506891, -12.52699322434005680, 60.92040820086095465 ) ) ;
#31148=CARTESIAN_POINT ( 'NONE',  ( -10.43125849979191955, -13.91324152291312366, 57.74825034919034294 ) ) ;
#31151=CARTESIAN_POINT ( 'NONE',  ( -20.87508512492161472, -21.41177400750635229, 58.75136860439389608 ) ) ;
#31152=CARTESIAN_POINT ( 'NONE',  ( -10.89696847888502163, -11.21756741187531681, 64.25543717716909953 ) ) ;
#31153=EDGE_CURVE ( 'NONE', #25531, #41086, #27767, .T. ) ;
#31156=FACE_BOUND ( 'NONE', #43535, .T. ) ;
#31159=ADVANCED_FACE ( 'NONE', ( #30538 ), #20680, .T. ) ;
#31161=CARTESIAN_POINT ( 'NONE',  ( -11.40126873537406205, -11.24191379345135999, 60.97885781058090515 ) ) ;
#31162=B_SPLINE_CURVE_WITH_KNOTS ( 'NONE', 1,
 ( #26535, #7841 ),
 .UNSPECIFIED., .F., .F.,
 ( 2, 2 ),
 ( 0.000000000000000000, 1.000000000000000000 ),
 .UNSPECIFIED. ) ;
#31169=ORIENTED_EDGE ( 'NONE', *, *, #23059, .F. ) ;
#31170=( BOUNDED_SURFACE ( )  B_SPLINE_SURFACE ( 3, 1, ( 
 ( #41898, #4233 ),
 ( #19974, #37947 ),
 ( #12099, #34975 ),
 ( #11862, #34491 ),
 ( #302, #23429 ),
 ( #778, #15774 ),
 ( #19242, #15521 ) ),
 .UNSPECIFIED., .T., .F., .F. ) 
 B_SPLINE_SURFACE_WITH_KNOTS ( ( 4, 3, 4 ),
 ( 2, 2 ),
 ( 0.000000000000000000, 0.5000000000000000000, 1.000000000000000000 ),
 ( 0.000000000000000000, 1.000000000000000000 ),
 .UNSPECIFIED. ) 
 GEOMETRIC_REPRESENTATION_ITEM ( )  RATIONAL_B_SPLINE_SURFACE ( (
 ( 1.000000000000000000, 1.000000000000000000),
 ( 0.3333333333333335369, 0.3333333333333330373),
 ( 0.3333333333333335369, 0.3333333333333330373),
 ( 1.000000000000000000, 1.000000000000000000),
 ( 0.3333333333333333703, 0.3333333333333333703),
 ( 0.3333333333333333703, 0.3333333333333333703),
 ( 1.000000000000000000, 1.000000000000000000) ) ) 
 REPRESENTATION_ITEM ( '' )  SURFACE ( )  );
#31172=ADVANCED_FACE ( 'NONE', ( #39366 ), #1934, .T. ) ;
#31173=EDGE_CURVE ( 'NONE', #10695, #19831, #16592, .T. ) ;
#31174=FACE_BOUND ( 'NONE', #18934, .T. ) ;
#31177=EDGE_LOOP ( 'NONE', ( #34044, #20138, #23307, #931 ) ) ;
#31178=CARTESIAN_POINT ( 'NONE',  ( -17.91451304303208403, -22.24313331792350112, 61.99040607801043734 ) ) ;
#31179=SURFACE_STYLE_FILL_AREA ( #32350 ) ;
#31181=CARTESIAN_POINT ( 'NONE',  ( -22.71059208588729561, -10.14448404190931186, 70.02650598627910483 ) ) ;
#31182=CARTESIAN_POINT ( 'NONE',  ( -10.72572792941078212, -12.60087465324735945, 64.68324854050578665 ) ) ;
#31183=CARTESIAN_POINT ( 'NONE',  ( -16.36834455927873222, -22.18410795223847387, 61.94063518049016182 ) ) ;
#31184=( BOUNDED_CURVE ( )  B_SPLINE_CURVE ( 3, ( #24554, #3081, #39788, #32869 ),
 .UNSPECIFIED., .F., .F. ) 
 B_SPLINE_CURVE_WITH_KNOTS ( ( 4, 4 ),
 ( 0.9074455897393642889, 1.000000000000000000 ),
 .UNSPECIFIED. ) 
 CURVE ( )  GEOMETRIC_REPRESENTATION_ITEM ( )  RATIONAL_B_SPLINE_CURVE ( ( 0.6983129098261030565, 0.7760317562607068620, 0.8765941196520058432, 1.000000000000000000 ) ) 
 REPRESENTATION_ITEM ( '' )  );
#31186=ORIENTED_EDGE ( 'NONE', *, *, #32917, .T. ) ;
#31188=EDGE_CURVE ( 'NONE', #19518, #18739, #5397, .T. ) ;
#31189=CARTESIAN_POINT ( 'NONE',  ( -21.06713455244400635, -20.85430592508659586, 72.66879606033384675 ) ) ;
#31192=EDGE_LOOP ( 'NONE', ( #13958, #36348, #45262, #18870 ) ) ;
#31196=VERTEX_POINT ( 'NONE', #6360 ) ;
#31198=CARTESIAN_POINT ( 'NONE',  ( -24.46260454045723520, -17.25128545673921465, 73.00619124008264293 ) ) ;
#31200=EDGE_LOOP ( 'NONE', ( #45752, #27852 ) ) ;
#31201=CYLINDRICAL_SURFACE ( 'NONE', #18590, 0.1500000000000057676 ) ;
#31202=FACE_OUTER_BOUND ( 'NONE', #8505, .T. ) ;
#31203=DIRECTION ( 'NONE',  ( -0.09855345062332551698, -0.9951317587989214619, -3.188559572103130227E-08 ) ) ;
#31204=CARTESIAN_POINT ( 'NONE',  ( -22.83095840648717711, -19.93459376977450859, 72.82895984417613988 ) ) ;
#31207=CARTESIAN_POINT ( 'NONE',  ( -22.91699213338677055, -19.14904519381134307, 58.90027305065820684 ) ) ;
#31208=CARTESIAN_POINT ( 'NONE',  ( -12.38818700662999994, -20.29940648439967887, 68.43633818813384551 ) ) ;
#31209=ORIENTED_EDGE ( 'NONE', *, *, #44602, .T. ) ;
#31210=CARTESIAN_POINT ( 'NONE',  ( -10.37560970945560967, -14.44337087574636769, 61.07388280500082800 ) ) ;
#31212=CARTESIAN_POINT ( 'NONE',  ( -9.974233412304723601, -14.74161775280529341, 71.46636207693717324 ) ) ;
#31213=CARTESIAN_POINT ( 'NONE',  ( -24.35389707626741185, -16.10709931453381216, 62.87856533165624029 ) ) ;
#31214=ORIENTED_EDGE ( 'NONE', *, *, #14832, .T. ) ;
#31216=CARTESIAN_POINT ( 'NONE',  ( -16.45566506110110083, -21.79267588865899086, 62.04095995016087528 ) ) ;
#31217=CARTESIAN_POINT ( 'NONE',  ( -24.64841560034816936, -12.98888891688536695, 63.00981035192142343 ) ) ;
#31219=DIRECTION ( 'NONE',  ( 0.7171836970970659753, -0.6968841687240311389, 4.479616660400600567E-09 ) ) ;
#31220=ORIENTED_EDGE ( 'NONE', *, *, #3038, .F. ) ;
#31221=CARTESIAN_POINT ( 'NONE',  ( -9.991168605297003680, -14.30431744343353628, 64.58078014788073062 ) ) ;
#31223=CARTESIAN_POINT ( 'NONE',  ( -20.66207843469866745, -8.601311859664747317, 63.42194587956323204 ) ) ;
#31224=CARTESIAN_POINT ( 'NONE',  ( -23.58616457878146377, -18.99640866789479432, 66.00884704819274873 ) ) ;
#31226=VERTEX_POINT ( 'NONE', #36378 ) ;
#31227=AXIS2_PLACEMENT_3D ( 'NONE', #19745, #46083, #18756 ) ;
#31230=ADVANCED_FACE ( 'NONE', ( #28534 ), #2660, .T. ) ;
#31231=CARTESIAN_POINT ( 'NONE',  ( -24.72547442936383888, -16.29049779397720243, 62.71611815716154581 ) ) ;
#31232=ORIENTED_EDGE ( 'NONE', *, *, #42356, .F. ) ;
#31235=CARTESIAN_POINT ( 'NONE',  ( -24.85359113602694237, -14.25571898851532460, 69.76779851910008290 ) ) ;
#31236=CARTESIAN_POINT ( 'NONE',  ( -10.15133553508400510, -13.19036488398009510, 71.32173201719281508 ) ) ;
#31240=CARTESIAN_POINT ( 'NONE',  ( -11.08714103679422713, -19.29340435200039394, 54.49999999999995026 ) ) ;
#31241=CARTESIAN_POINT ( 'NONE',  ( -19.75213962495824305, -21.88613070990731302, 65.56462585307971835 ) ) ;
#31242=ORIENTED_EDGE ( 'NONE', *, *, #11483, .F. ) ;
#31243=ORIENTED_EDGE ( 'NONE', *, *, #7788, .F. ) ;
#31244=CARTESIAN_POINT ( 'NONE',  ( -12.39977816794586829, -20.31007402754922353, 68.52931606572398948 ) ) ;
#31245=EDGE_CURVE ( 'NONE', #38697, #8171, #24836, .T. ) ;
#31247=CARTESIAN_POINT ( 'NONE',  ( -23.68216657795769109, -11.66929788463824202, 66.53287594076890343 ) ) ;
#31249=CARTESIAN_POINT ( 'NONE',  ( -18.76558392140857023, -7.480892851696864021, 70.55563303198719893 ) ) ;
#31252=CARTESIAN_POINT ( 'NONE',  ( -24.09792882696954663, -17.08130396874204138, 73.03336032035906555 ) ) ;
#31253=CARTESIAN_POINT ( 'NONE',  ( -15.48424252676649182, -21.53505049348036948, 72.34575460973682937 ) ) ;
#31255=ORIENTED_EDGE ( 'NONE', *, *, #47868, .F. ) ;
#31259=ORIENTED_EDGE ( 'NONE', *, *, #45484, .F. ) ;
#31260=AXIS2_PLACEMENT_3D ( 'NONE', #32063, #47798, #14039 ) ;
#31261=CARTESIAN_POINT ( 'NONE',  ( -14.72778360411233045, -21.32322305517535099, 58.31617885012778402 ) ) ;
#31262=CARTESIAN_POINT ( 'NONE',  ( -24.21863450226962300, -16.49938964532870145, 59.23405620101143398 ) ) ;
#31263=EDGE_CURVE ( 'NONE', #18577, #9916, #38207, .T. ) ;
#31264=ORIENTED_EDGE ( 'NONE', *, *, #31742, .T. ) ;
#31265=FACE_BOUND ( 'NONE', #33275, .T. ) ;
#31266=AXIS2_PLACEMENT_3D ( 'NONE', #42689, #8956, #27410 ) ;
#31268=CARTESIAN_POINT ( 'NONE',  ( -15.68503146357154776, -7.977064754671971514, 70.75989839959960648 ) ) ;
#31269=FACE_OUTER_BOUND ( 'NONE', #16068, .T. ) ;
#31271=CARTESIAN_POINT ( 'NONE',  ( -23.91010245674826251, -17.57297063409389537, 62.75888927877479517 ) ) ;
#31273=LINE ( 'NONE', #16230, #1405 ) ;
#31276=CARTESIAN_POINT ( 'NONE',  ( -19.31122959855452237, -8.013358182787271744, 63.84578077065769719 ) ) ;
#31277=CARTESIAN_POINT ( 'NONE',  ( -10.93683055674727633, -17.43892421286904337, 64.73625468762544699 ) ) ;
#31280=CARTESIAN_POINT ( 'NONE',  ( -11.63680200852674496, -10.77675165258979284, 74.64704609179688077 ) ) ;
#31281=CARTESIAN_POINT ( 'NONE',  ( -24.59520773924778325, -12.78944134693112744, 66.42433958033493013 ) ) ;
#31284=ORIENTED_EDGE ( 'NONE', *, *, #39573, .T. ) ;
#31285=ADVANCED_FACE ( 'NONE', ( #25548 ), #29988, .T. ) ;
#31286=CARTESIAN_POINT ( 'NONE',  ( -11.16720068213728467, -11.56054720508597455, 67.76864607954532005 ) ) ;
#31287=CARTESIAN_POINT ( 'NONE',  ( -24.36611147337434957, -16.04009697885371111, 66.07797069094537790 ) ) ;
#31288=VERTEX_POINT ( 'NONE', #2891 ) ;
#31291=FACE_OUTER_BOUND ( 'NONE', #21134, .T. ) ;
#31294=CARTESIAN_POINT ( 'NONE',  ( -24.41419987208840325, -15.75358948762744760, 66.27144644829634501 ) ) ;
#31298=CARTESIAN_POINT ( 'NONE',  ( -23.72641715273374530, -11.63183476396761407, 70.03643756225406491 ) ) ;
#31299=VECTOR ( 'NONE', #13799, 1000.000000000000000 ) ;
#31300=EDGE_LOOP ( 'NONE', ( #46734, #38564 ) ) ;
#31301=EDGE_CURVE ( 'NONE', #7468, #26935, #2972, .T. ) ;
#31302=CARTESIAN_POINT ( 'NONE',  ( -22.23351441301664622, -19.96811234597608120, 69.58906588434240348 ) ) ;
#31304=CARTESIAN_POINT ( 'NONE',  ( -12.86353962931362283, -9.432586330540292607, 74.33395128836551180 ) ) ;
#31305=VECTOR ( 'NONE', #40533, 999.9999999999998863 ) ;
#31306=CARTESIAN_POINT ( 'NONE',  ( -17.63137589695670471, -7.812166007416677438, 63.85057029281470875 ) ) ;
#31307=CARTESIAN_POINT ( 'NONE',  ( -21.37553466301574190, -9.031134576986278972, 70.24018460668924035 ) ) ;
#31309=( BOUNDED_CURVE ( )  B_SPLINE_CURVE ( 3, ( #19467, #41642, #30089, #7193 ),
 .UNSPECIFIED., .F., .F. ) 
 B_SPLINE_CURVE_WITH_KNOTS ( ( 4, 4 ),
 ( 0.9074455897393561843, 1.000000000000000000 ),
 .UNSPECIFIED. ) 
 CURVE ( )  GEOMETRIC_REPRESENTATION_ITEM ( )  RATIONAL_B_SPLINE_CURVE ( ( 0.6983129098260747458, 0.7760317562606824371, 0.8765941196519908551, 1.000000000000000000 ) ) 
 REPRESENTATION_ITEM ( '' )  );
#31310=AXIS2_PLACEMENT_3D ( 'NONE', #17757, #9915, #39221 ) ;
#31313=VERTEX_POINT ( 'NONE', #33911 ) ;
#31314=CARTESIAN_POINT ( 'NONE',  ( -11.00364514860770271, -18.58846920323082585, 57.94568058987277936 ) ) ;
#31316=( BOUNDED_CURVE ( )  B_SPLINE_CURVE ( 3, ( #19228, #34474, #22685, #31045 ),
 .UNSPECIFIED., .F., .F. ) 
 B_SPLINE_CURVE_WITH_KNOTS ( ( 4, 4 ),
 ( 0.4074455897393665094, 0.5000000000000000000 ),
 .UNSPECIFIED. ) 
 CURVE ( )  GEOMETRIC_REPRESENTATION_ITEM ( )  RATIONAL_B_SPLINE_CURVE ( ( 0.6983129098260970613, 0.7760317562606922071, 0.8765941196519905221, 0.9999999999999851230 ) ) 
 REPRESENTATION_ITEM ( '' )  );
#31318=CARTESIAN_POINT ( 'NONE',  ( -17.56322643164902431, -15.18422937902243142, 56.49999999999994316 ) ) ;
#31319=EDGE_LOOP ( 'NONE', ( #43228, #10378 ) ) ;
#31320=VECTOR ( 'NONE', #7547, 1000.000000000000114 ) ;
#31321=CARTESIAN_POINT ( 'NONE',  ( -10.46488639952936950, -14.05403152202256223, 57.67498297385893125 ) ) ;
#31322=VECTOR ( 'NONE', #20648, 1000.000000000000227 ) ;
#31323=ORIENTED_EDGE ( 'NONE', *, *, #27445, .T. ) ;
#31324=CARTESIAN_POINT ( 'NONE',  ( -20.03744868119640898, -21.78660147720172802, 69.04827188316701836 ) ) ;
#31326=CARTESIAN_POINT ( 'NONE',  ( -17.56947109021050224, -7.760665246103527259, 63.85057029441095011 ) ) ;
#31329=FACE_OUTER_BOUND ( 'NONE', #36742, .T. ) ;
#31330=CARTESIAN_POINT ( 'NONE',  ( -16.64258257546838138, -22.21885596081591174, 68.88215988439684168 ) ) ;
#31331=CARTESIAN_POINT ( 'NONE',  ( -10.41342670640989176, -14.06412934096922562, 60.92381095562976867 ) ) ;
#31336=CARTESIAN_POINT ( 'NONE',  ( -18.33724152424255394, -21.79985958048214556, 69.11514682450841462 ) ) ;
#31337=CARTESIAN_POINT ( 'NONE',  ( -10.77962265614084814, -17.18953632050836333, 68.24154640182683806 ) ) ;
#31338=CARTESIAN_POINT ( 'NONE',  ( -14.91112529534803066, -8.221969756899694559, 57.13527940342243028 ) ) ;
#31339=CARTESIAN_POINT ( 'NONE',  ( -17.51497182922874174, -7.809736700347588823, 63.56559502915499849 ) ) ;
#31341=CARTESIAN_POINT ( 'NONE',  ( -10.76763535483202539, -17.13171813241336494, 61.30743118825921556 ) ) ;
#31345=EDGE_CURVE ( 'NONE', #15104, #28108, #37922, .T. ) ;
#31348=VERTEX_POINT ( 'NONE', #48436 ) ;
#31349=B_SPLINE_CURVE_WITH_KNOTS ( 'NONE', 3,
 ( #13714, #5873, #13478, #9813, #28279, #24599, #24827, #28526, #20888, #35412 ),
 .UNSPECIFIED., .F., .F.,
 ( 4, 2, 2, 2, 4 ),
 ( 0.1272669073658556915, 0.2522669073488191804, 0.3772669073317826971, 0.5022669073147462138, 0.6272669072977097304 ),
 .UNSPECIFIED. ) ;
#31350=CARTESIAN_POINT ( 'NONE',  ( -13.89389072038462025, -21.36980434119256600, 72.11103101793651149 ) ) ;
#31351=CARTESIAN_POINT ( 'NONE',  ( -14.66630222544868900, -8.320656262913127321, 63.80450889863892172 ) ) ;
#31352=CARTESIAN_POINT ( 'NONE',  ( -24.23636277187043220, -17.82529184948975498, 62.58865552117998021 ) ) ;
#31353=CARTESIAN_POINT ( 'NONE',  ( -12.68381401182790569, -19.95991009262169413, 68.33657438305763776 ) ) ;
#31354=CARTESIAN_POINT ( 'NONE',  ( -14.71062220868414805, -21.26200545334448222, 58.16617879205879404 ) ) ;
#31355=VERTEX_POINT ( 'NONE', #45022 ) ;
#31356=CARTESIAN_POINT ( 'NONE',  ( -23.73600461991442501, -11.78168063161743362, 62.96834887429472616 ) ) ;
#31357=CARTESIAN_POINT ( 'NONE',  ( -19.86569447268030686, -19.73755174630646536, 53.49899999999994549 ) ) ;
#31359=CARTESIAN_POINT ( 'NONE',  ( -19.09949158415725634, -8.012660229328147921, 63.43089235425713923 ) ) ;
#31361=CYLINDRICAL_SURFACE ( 'NONE', #14031, 0.1500000000000004385 ) ;
#31363=EDGE_CURVE ( 'NONE', #17355, #23884, #37586, .T. ) ;
#31365=VECTOR ( 'NONE', #36126, 1000.000000000000227 ) ;
#31366=CARTESIAN_POINT ( 'NONE',  ( -21.78293781325145773, -8.767371536720848013, 70.23858402064847439 ) ) ;
#31369=AXIS2_PLACEMENT_3D ( 'NONE', #26932, #15826, #34294 ) ;
#31370=ORIENTED_EDGE ( 'NONE', *, *, #45560, .F. ) ;
#31373=DIRECTION ( 'NONE',  ( 3.549360974554993999E-17, -6.371834667797928663E-18, -1.000000000000000000 ) ) ;
#31374=CARTESIAN_POINT ( 'NONE',  ( -15.35181094580836358, -7.653138554841501850, 74.12339718037890179 ) ) ;
#31376=ADVANCED_FACE ( 'NONE', ( #33161 ), #3629, .F. ) ;
#31378=CARTESIAN_POINT ( 'NONE',  ( -14.27319436148695431, -8.558459998996717388, 71.02957628730779049 ) ) ;
#31379=EDGE_CURVE ( 'NONE', #33892, #1223, #18231, .T. ) ;
#31381=CARTESIAN_POINT ( 'NONE',  ( -9.979603264230430426, -14.52052340097724148, 68.04295441848455539 ) ) ;
#31382=CARTESIAN_POINT ( 'NONE',  ( -24.26194381736407735, -17.76675604995504543, 62.66635152724034441 ) ) ;
#31383=ORIENTED_EDGE ( 'NONE', *, *, #48514, .F. ) ;
#31386=CARTESIAN_POINT ( 'NONE',  ( -10.13784000599894597, -13.25541019000276499, 74.79322239981686948 ) ) ;
#31387=CARTESIAN_POINT ( 'NONE',  ( -9.974321184477874525, -14.87343388147542100, 74.99117216852748413 ) ) ;
#31389=CYLINDRICAL_SURFACE ( 'NONE', #41923, 0.1500000000000031863 ) ;
#31390=FACE_OUTER_BOUND ( 'NONE', #34003, .T. ) ;
#31392=( BOUNDED_CURVE ( )  B_SPLINE_CURVE ( 3, ( #43369, #32283, #21195, #5456 ),
 .UNSPECIFIED., .F., .F. ) 
 B_SPLINE_CURVE_WITH_KNOTS ( ( 4, 4 ),
 ( 0.4074455897393643444, 0.5000000000000000000 ),
 .UNSPECIFIED. ) 
 CURVE ( )  GEOMETRIC_REPRESENTATION_ITEM ( )  RATIONAL_B_SPLINE_CURVE ( ( 0.6983129098261118273, 0.7760317562607139674, 0.8765941196520097289, 0.9999999999999991118 ) ) 
 REPRESENTATION_ITEM ( '' )  );
#31396=CARTESIAN_POINT ( 'NONE',  ( -18.57335281209669375, -21.76520412651811043, 72.57038810541313012 ) ) ;
#31397=DIRECTION ( 'NONE',  ( -0.4182840851231335866, 0.9083162577718750796, -8.112345261760041810E-09 ) ) ;
#31400=DIRECTION ( 'NONE',  ( -6.291559624462811924E-07, 1.530398240482465057E-06, -0.9999999999986309840 ) ) ;
#31401=FACE_BOUND ( 'NONE', #16915, .T. ) ;
#31402=CARTESIAN_POINT ( 'NONE',  ( -20.72450927900464634, -21.03929139025762751, 58.93003081252663833 ) ) ;
#31403=CARTESIAN_POINT ( 'NONE',  ( -17.46222794319647775, -7.759011850482251837, 67.03511641684839617 ) ) ;
#31404=CARTESIAN_POINT ( 'NONE',  ( -22.57893663749957369, -9.999394138389961384, 73.49633153340955971 ) ) ;
#31406=CARTESIAN_POINT ( 'NONE',  ( -21.84079957929829874, -9.314189696129256291, 63.19153755727188582 ) ) ;
#31409=DIRECTION ( 'NONE',  ( -5.731567514496413899E-31, -1.020425574103664789E-16, -1.000000000000000000 ) ) ;
#31410=DIRECTION ( 'NONE',  ( 0.02400335114476204526, -0.9997118780597843424, -1.529429985666831130E-10 ) ) ;
#31411=ORIENTED_EDGE ( 'NONE', *, *, #16234, .F. ) ;
#31413=CARTESIAN_POINT ( 'NONE',  ( -11.60006209888454443, -10.16330164164447325, 71.08397698276321819 ) ) ;
#31414=EDGE_CURVE ( 'NONE', #3376, #48249, #17352, .T. ) ;
#31415=VERTEX_POINT ( 'NONE', #33645 ) ;
#31418=EDGE_CURVE ( 'NONE', #23554, #45950, #20619, .T. ) ;
#31419=CARTESIAN_POINT ( 'NONE',  ( -10.41569439578338496, -15.57669382292980131, 61.05261153187079515 ) ) ;
#31420=CYLINDRICAL_SURFACE ( 'NONE', #7521, 0.1500000000000042133 ) ;
#31423=ORIENTED_EDGE ( 'NONE', *, *, #16898, .T. ) ;
#31425=CARTESIAN_POINT ( 'NONE',  ( -22.68532657142340980, -20.08396690885253477, 69.21772085510332317 ) ) ;
#31431=EDGE_CURVE ( 'NONE', #25227, #23300, #30050, .T. ) ;
#31433=EDGE_CURVE ( 'NONE', #30016, #37344, #21856, .T. ) ;
#31434=EDGE_CURVE ( 'NONE', #39530, #35725, #24128, .T. ) ;
#31435=CARTESIAN_POINT ( 'NONE',  ( -14.72662834380375685, -21.75384922062382032, 61.75883521239082086 ) ) ;
#31436=EDGE_CURVE ( 'NONE', #8033, #35067, #19138, .T. ) ;
#31437=CARTESIAN_POINT ( 'NONE',  ( -15.33756252250768881, -21.49113013396807403, 68.57592903490986203 ) ) ;
#31438=CARTESIAN_POINT ( 'NONE',  ( -17.32080883166002039, -7.809907297400525472, 67.30574285593853290 ) ) ;
#31439=AXIS2_PLACEMENT_3D ( 'NONE', #6856, #13504, #28548 ) ;
#31440=( BOUNDED_CURVE ( )  B_SPLINE_CURVE ( 3, ( #44576, #18211, #35959, #33217 ),
 .UNSPECIFIED., .F., .F. ) 
 B_SPLINE_CURVE_WITH_KNOTS ( ( 4, 4 ),
 ( 0.9074455897393632897, 1.000000000000000000 ),
 .UNSPECIFIED. ) 
 CURVE ( )  GEOMETRIC_REPRESENTATION_ITEM ( )  RATIONAL_B_SPLINE_CURVE ( ( 0.6983129098260834056, 0.7760317562606898756, 0.8765941196519954071, 1.000000000000000000 ) ) 
 REPRESENTATION_ITEM ( '' )  );
#31441=ORIENTED_EDGE ( 'NONE', *, *, #15946, .T. ) ;
#31442=CARTESIAN_POINT ( 'NONE',  ( -11.68335768792166185, -18.81469630946190819, 68.51689631952916670 ) ) ;
#31443=CARTESIAN_POINT ( 'NONE',  ( -10.83541799943766293, -17.32598710976732903, 61.04254427365582103 ) ) ;
#31445=CARTESIAN_POINT ( 'NONE',  ( -24.17309265654468931, -11.65389292077413685, 59.62089248282786969 ) ) ;
#31446=ORIENTED_EDGE ( 'NONE', *, *, #41539, .T. ) ;
#31449=CARTESIAN_POINT ( 'NONE',  ( -11.39842260918292638, -18.37420288192462792, 61.34881185081356847 ) ) ;
#31450=VERTEX_POINT ( 'NONE', #42281 ) ;
#31451=CARTESIAN_POINT ( 'NONE',  ( -16.01882192674287708, -7.492892668753452945, 63.86349355235967806 ) ) ;
#31452=( BOUNDED_CURVE ( )  B_SPLINE_CURVE ( 3, ( #32442, #47465, #13700, #15837 ),
 .UNSPECIFIED., .F., .F. ) 
 B_SPLINE_CURVE_WITH_KNOTS ( ( 4, 4 ),
 ( 0.000000000000000000, 0.4074455897393696180 ),
 .UNSPECIFIED. ) 
 CURVE ( )  GEOMETRIC_REPRESENTATION_ITEM ( )  RATIONAL_B_SPLINE_CURVE ( ( 1.000000000000000000, 0.4567392136813263059, 0.3561768502900282130, 0.6983129098261057210 ) ) 
 REPRESENTATION_ITEM ( '' )  );
#31454=CARTESIAN_POINT ( 'NONE',  ( -21.47456293661849713, -9.038556783377254433, 70.41660404402310292 ) ) ;
#31455=CARTESIAN_POINT ( 'NONE',  ( -10.37714865501246564, -15.10143083228766159, 74.68290095780284332 ) ) ;
#31457=CARTESIAN_POINT ( 'NONE',  ( -22.16028090469329825, -20.56016676735646698, 58.90409545820185144 ) ) ;
#31458=FACE_OUTER_BOUND ( 'NONE', #22652, .T. ) ;
#31460=CARTESIAN_POINT ( 'NONE',  ( -24.22177711603362482, -13.13842781680106420, 62.83264177645653348 ) ) ;
#31462=DIRECTION ( 'NONE',  ( -0.8810891847886966888, -0.4615090133018290852, 0.1033986416233891037 ) ) ;
#31463=VERTEX_POINT ( 'NONE', #12001 ) ;
#31465=AXIS2_PLACEMENT_3D ( 'NONE', #45096, #41373, #26125 ) ;
#31466=CARTESIAN_POINT ( 'NONE',  ( -10.89280251029460622, -11.22507333849785027, 64.33377325762776877 ) ) ;
#31467=CARTESIAN_POINT ( 'NONE',  ( -22.24221110980738558, -9.126920263178931236, 59.92159993762222570 ) ) ;
#31469=CARTESIAN_POINT ( 'NONE',  ( -15.75283698213507755, -7.548994588147243334, 67.32502552484606895 ) ) ;
#31471=( BOUNDED_SURFACE ( )  B_SPLINE_SURFACE ( 3, 1, ( 
 ( #4545, #27441 ),
 ( #8983, #41985 ),
 ( #31632, #20301 ),
 ( #38257, #20058 ),
 ( #39255, #1325 ),
 ( #27200, #34328 ),
 ( #862, #31381 ) ),
 .UNSPECIFIED., .T., .F., .F. ) 
 B_SPLINE_SURFACE_WITH_KNOTS ( ( 4, 3, 4 ),
 ( 2, 2 ),
 ( 0.000000000000000000, 0.5000000000000000000, 1.000000000000000000 ),
 ( 0.000000000000000000, 1.000000000000000000 ),
 .UNSPECIFIED. ) 
 GEOMETRIC_REPRESENTATION_ITEM ( )  RATIONAL_B_SPLINE_SURFACE ( (
 ( 1.000000000000000000, 1.000000000000000000),
 ( 0.3333333333333335369, 0.3333333333333330373),
 ( 0.3333333333333335369, 0.3333333333333330373),
 ( 1.000000000000000000, 1.000000000000000000),
 ( 0.3333333333333333703, 0.3333333333333333703),
 ( 0.3333333333333333703, 0.3333333333333333703),
 ( 1.000000000000000000, 1.000000000000000000) ) ) 
 REPRESENTATION_ITEM ( '' )  SURFACE ( )  );
#31473=EDGE_LOOP ( 'NONE', ( #1074, #11849 ) ) ;
#31474=CARTESIAN_POINT ( 'NONE',  ( -10.44881481234349252, -17.42631575494719698, 64.74243950200344955 ) ) ;
#31475=CARTESIAN_POINT ( 'NONE',  ( -13.01353397724842154, -8.804979801064929390, 64.09441804368185558 ) ) ;
#31476=ADVANCED_FACE ( 'NONE', ( #4858, #917 ), #41550, .T. ) ;
#31477=CARTESIAN_POINT ( 'NONE',  ( -10.37541943412130863, -14.96049300415475614, 75.08306784598362071 ) ) ;
#31481=B_SPLINE_CURVE_WITH_KNOTS ( 'NONE', 3,
 ( #15987, #39385, #31033, #5666, #46049, #20679, #27329, #1219, #16222, #27576 ),
 .UNSPECIFIED., .F., .F.,
 ( 4, 2, 2, 2, 4 ),
 ( 0.1272669073658583838, 0.2522669073439522958, 0.3772669073220461522, 0.5022669073001400086, 0.6272669072782339761 ),
 .UNSPECIFIED. ) ;
#31482=CARTESIAN_POINT ( 'NONE',  ( -23.41616298382994898, -18.52428493080399363, 72.77840375779385340 ) ) ;
#31483=CARTESIAN_POINT ( 'NONE',  ( -23.26031807999110157, -18.67503349580112015, 69.30988682986618699 ) ) ;
#31484=CARTESIAN_POINT ( 'NONE',  ( -11.13733870171179596, -11.61806121328042174, 67.90392505421056057 ) ) ;
#31485=VERTEX_POINT ( 'NONE', #27497 ) ;
#31486=ORIENTED_EDGE ( 'NONE', *, *, #30141, .F. ) ;
#31487=CARTESIAN_POINT ( 'NONE',  ( -11.18734459328334907, -11.50497870355291319, 60.83452645039198359 ) ) ;
#31490=CARTESIAN_POINT ( 'NONE',  ( -13.18362795047878144, -8.683667697493742565, 60.62445659250467145 ) ) ;
#31491=CARTESIAN_POINT ( 'NONE',  ( -21.85574357498200015, -9.390598081573159561, 59.79459286646363836 ) ) ;
#31492=B_SPLINE_CURVE_WITH_KNOTS ( 'NONE', 3,
 ( #46785, #43083, #24383, #39393, #20687, #44544, #48462, #10799, #37876, #21882 ),
 .UNSPECIFIED., .F., .F.,
 ( 4, 2, 2, 2, 4 ),
 ( 0.6272669072877963270, 0.7522669073073113832, 0.8772669073268264395, 1.002266907346341496, 1.127266907365856552 ),
 .UNSPECIFIED. ) ;
#31493=ORIENTED_EDGE ( 'NONE', *, *, #46729, .F. ) ;
#31494=EDGE_CURVE ( 'NONE', #47561, #32087, #24728, .T. ) ;
#31496=LINE ( 'NONE', #5653, #20964 ) ;
#31497=CARTESIAN_POINT ( 'NONE',  ( -24.48201381491371009, -14.78211897600973934, 66.32725479646262556 ) ) ;
#31499=CARTESIAN_POINT ( 'NONE',  ( -14.92957361138602579, -21.82925975653312278, 65.22101252026929785 ) ) ;
#31501=ORIENTED_EDGE ( 'NONE', *, *, #13014, .F. ) ;
#31503=CARTESIAN_POINT ( 'NONE',  ( -10.55452786565646228, -16.15453179965403763, 68.05055783647944168 ) ) ;
#31504=EDGE_CURVE ( 'NONE', #26563, #4162, #28295, .T. ) ;
#31505=EDGE_CURVE ( 'NONE', #30656, #23723, #26780, .T. ) ;
#31506=CARTESIAN_POINT ( 'NONE',  ( -24.03160980685186843, -17.26750534774173929, 69.41339792588560442 ) ) ;
#31507=ORIENTED_EDGE ( 'NONE', *, *, #18933, .T. ) ;
#31509=AXIS2_PLACEMENT_3D ( 'NONE', #441, #18897, #23572 ) ;
#31511=CARTESIAN_POINT ( 'NONE',  ( -24.24305604114050539, -16.39138756491875171, 59.12332478929949531 ) ) ;
#31512=EDGE_LOOP ( 'NONE', ( #38544, #2009 ) ) ;
#31516=CARTESIAN_POINT ( 'NONE',  ( -18.71262049920375503, -21.74350751539899562, 72.17022092985547488 ) ) ;
#31517=ORIENTED_EDGE ( 'NONE', *, *, #27895, .F. ) ;
#31518=DIRECTION ( 'NONE',  ( 0.8467008005855412023, -0.3141239757129647425, -0.4294460177601887585 ) ) ;
#31519=DIRECTION ( 'NONE',  ( 0.5881408891789771110, 0.8087584895849666555, -7.565907429265703656E-08 ) ) ;
#31520=ADVANCED_FACE ( 'NONE', ( #7833 ), #44281, .T. ) ;
#31523=ORIENTED_EDGE ( 'NONE', *, *, #32376, .T. ) ;
#31524=CARTESIAN_POINT ( 'NONE',  ( -14.80072874354800305, -7.836285926156586257, 56.89354091526551116 ) ) ;
#31525=CARTESIAN_POINT ( 'NONE',  ( -24.45577199812615632, -12.20047074031916168, 47.99999999999994316 ) ) ;
#31527=CARTESIAN_POINT ( 'NONE',  ( -16.13676401591364140, -7.928535094101303748, 60.42701728694442664 ) ) ;
#31528=CARTESIAN_POINT ( 'NONE',  ( -11.64873123714592396, -10.76074834137913960, 74.32396018297762907 ) ) ;
#31531=VECTOR ( 'NONE', #15179, 1000.000000000000000 ) ;
#31532=CARTESIAN_POINT ( 'NONE',  ( -12.25319814409069252, -20.17255476956438542, 64.91028984507975963 ) ) ;
#31533=ORIENTED_EDGE ( 'NONE', *, *, #32715, .T. ) ;
#31534=ORIENTED_EDGE ( 'NONE', *, *, #39126, .F. ) ;
#31535=AXIS2_PLACEMENT_3D ( 'NONE', #1120, #16854, #1355 ) ;
#31537=CARTESIAN_POINT ( 'NONE',  ( -24.31724253335826447, -16.02795960786995977, 62.82001908927701805 ) ) ;
#31540=CARTESIAN_POINT ( 'NONE',  ( -19.41474841345058522, -21.52018966427049307, 62.29503644830997189 ) ) ;
#31541=CARTESIAN_POINT ( 'NONE',  ( -23.01604236747990839, -10.51564102213499474, 59.89643612291379071 ) ) ;
#31542=LINE ( 'NONE', #42870, #4578 ) ;
#31546=CARTESIAN_POINT ( 'NONE',  ( -16.92050523043788957, -21.84918965566402704, 65.38131313066115524 ) ) ;
#31547=CARTESIAN_POINT ( 'NONE',  ( -19.17247957453286844, -7.567181637230756763, 63.61584517348745038 ) ) ;
#31549=CARTESIAN_POINT ( 'NONE',  ( -12.58002213166789041, -9.148928514680237711, 74.43427606957253317 ) ) ;
#31550=CARTESIAN_POINT ( 'NONE',  ( -12.57881008754452345, -9.149975892475048056, 74.57568945445216002 ) ) ;
#31551=CARTESIAN_POINT ( 'NONE',  ( -21.18000576974785787, -20.77541348745421246, 69.35450184739246993 ) ) ;
#31552=EDGE_CURVE ( 'NONE', #27678, #9892, #22856, .T. ) ;
#31553=ORIENTED_EDGE ( 'NONE', *, *, #2167, .F. ) ;
#31554=VERTEX_POINT ( 'NONE', #17114 ) ;
#31556=EDGE_CURVE ( 'NONE', #6043, #33004, #24548, .T. ) ;
#31557=CARTESIAN_POINT ( 'NONE',  ( -17.79901357976508791, -7.766176623049141803, 63.96545652844361740 ) ) ;
#31559=CARTESIAN_POINT ( 'NONE',  ( -20.01035006975242680, -21.36773898636727509, 72.70478738042278621 ) ) ;
#31561=CARTESIAN_POINT ( 'NONE',  ( -21.73662441638722953, -9.231682010981758779, 66.67622112302015580 ) ) ;
#31563=ORIENTED_EDGE ( 'NONE', *, *, #21097, .F. ) ;
#31564=EDGE_CURVE ( 'NONE', #47492, #24829, #9465, .T. ) ;
#31566=CARTESIAN_POINT ( 'NONE',  ( -10.63133999448158384, -17.86890150755132822, 71.67379904062892138 ) ) ;
#31567=CARTESIAN_POINT ( 'NONE',  ( -19.30128557755455176, -21.60500301973953086, 58.81035253397666196 ) ) ;
#31572=CARTESIAN_POINT ( 'NONE',  ( -10.58054468882281363, -13.33752895606068201, 71.31714512707709730 ) ) ;
#31573=ORIENTED_EDGE ( 'NONE', *, *, #41350, .T. ) ;
#31575=CARTESIAN_POINT ( 'NONE',  ( -22.47381490279794036, -20.28691852675989793, 65.84388348312960204 ) ) ;
#31577=ORIENTED_EDGE ( 'NONE', *, *, #8386, .T. ) ;
#31580=CARTESIAN_POINT ( 'NONE',  ( -22.17253171379126897, -20.54993857985014216, 59.02088830234949057 ) ) ;
#31582=EDGE_CURVE ( 'NONE', #2353, #41372, #16504, .T. ) ;
#31583=( BOUNDED_CURVE ( )  B_SPLINE_CURVE ( 3, ( #27957, #4836, #11985, #16382 ),
 .UNSPECIFIED., .F., .F. ) 
 B_SPLINE_CURVE_WITH_KNOTS ( ( 4, 4 ),
 ( 0.000000000000000000, 0.4074455897393663428 ),
 .UNSPECIFIED. ) 
 CURVE ( )  GEOMETRIC_REPRESENTATION_ITEM ( )  RATIONAL_B_SPLINE_CURVE ( ( 1.000000000000000000, 0.4567392136813290815, 0.3561768502900292122, 0.6983129098261003920 ) ) 
 REPRESENTATION_ITEM ( '' )  );
#31584=CARTESIAN_POINT ( 'NONE',  ( -15.62101046192594289, -7.580605815997546237, 70.72494447658496597 ) ) ;
#31585=DIRECTION ( 'NONE',  ( -6.258914682829359833E-07, 5.777405174637831559E-07, 0.9999999999996371791 ) ) ;
#31586=CARTESIAN_POINT ( 'NONE',  ( -20.60910058366379616, -21.04276686425195919, 58.94475179565701950 ) ) ;
#31587=EDGE_LOOP ( 'NONE', ( #29492, #26636, #46942, #36564, #11386 ) ) ;
#31590=CARTESIAN_POINT ( 'NONE',  ( -16.20950590255762691, -7.458868724970470154, 60.30054238772634534 ) ) ;
#31591=B_SPLINE_CURVE_WITH_KNOTS ( 'NONE', 3,
 ( #24542, #20098, #20828, #47174, #5582, #46205, #42991, #42521, #16868, #31183 ),
 .UNSPECIFIED., .F., .F.,
 ( 4, 2, 2, 2, 4 ),
 ( 0.1272669073658357908, 0.2522669073463156275, 0.3772669073267955198, 0.5022669073072754120, 0.6272669072877552487 ),
 .UNSPECIFIED. ) ;
#31592=DIRECTION ( 'NONE',  ( -0.1464579420318390945, 0.9892168979631277281, 7.284849527811297202E-08 ) ) ;
#31593=CARTESIAN_POINT ( 'NONE',  ( -14.14556133858745390, -20.99403164004895217, 71.94110109989711077 ) ) ;
#31597=EDGE_LOOP ( 'NONE', ( #19494, #21735, #16528, #44980, #20692 ) ) ;
#31599=FACE_OUTER_BOUND ( 'NONE', #45169, .T. ) ;
#31600=ORIENTED_EDGE ( 'NONE', *, *, #38960, .F. ) ;
#31601=CARTESIAN_POINT ( 'NONE',  ( -24.37683887807358474, -15.97618392648307584, 66.36324926629207255 ) ) ;
#31602=CARTESIAN_POINT ( 'NONE',  ( -15.49415775405465645, -8.028509947901662613, 74.37985659017799378 ) ) ;
#31603=CARTESIAN_POINT ( 'NONE',  ( -12.74071780128996423, -9.015264284427722430, 70.96430057504635158 ) ) ;
#31604=CARTESIAN_POINT ( 'NONE',  ( -11.03124120290388532, -17.66077365132053956, 71.86718193465377169 ) ) ;
#31605=FACE_OUTER_BOUND ( 'NONE', #34941, .T. ) ;
#31606=( BOUNDED_SURFACE ( )  B_SPLINE_SURFACE ( 3, 1, ( 
 ( #18710, #37667 ),
 ( #11098, #41133 ),
 ( #22417, #44590 ),
 ( #33721, #10845 ),
 ( #7664, #25867 ),
 ( #37411, #29322 ),
 ( #40884, #7415 ) ),
 .UNSPECIFIED., .T., .F., .F. ) 
 B_SPLINE_SURFACE_WITH_KNOTS ( ( 4, 3, 4 ),
 ( 2, 2 ),
 ( 0.000000000000000000, 0.5000000000000000000, 1.000000000000000000 ),
 ( 0.000000000000000000, 1.000000000000000000 ),
 .UNSPECIFIED. ) 
 GEOMETRIC_REPRESENTATION_ITEM ( )  RATIONAL_B_SPLINE_SURFACE ( (
 ( 1.000000000000000000, 1.000000000000000000),
 ( 0.3333333333333335369, 0.3333333333333330373),
 ( 0.3333333333333335369, 0.3333333333333330373),
 ( 1.000000000000000000, 1.000000000000000000),
 ( 0.3333333333333333703, 0.3333333333333333703),
 ( 0.3333333333333333703, 0.3333333333333333703),
 ( 1.000000000000000000, 1.000000000000000000) ) ) 
 REPRESENTATION_ITEM ( '' )  SURFACE ( )  );
#31607=ORIENTED_EDGE ( 'NONE', *, *, #31025, .T. ) ;
#31608=( BOUNDED_CURVE ( )  B_SPLINE_CURVE ( 3, ( #8469, #23750, #19804, #41719 ),
 .UNSPECIFIED., .F., .F. ) 
 B_SPLINE_CURVE_WITH_KNOTS ( ( 4, 4 ),
 ( 0.4074455897393575166, 0.5000000000000000000 ),
 .UNSPECIFIED. ) 
 CURVE ( )  GEOMETRIC_REPRESENTATION_ITEM ( )  RATIONAL_B_SPLINE_CURVE ( ( 0.6983129098260714152, 0.7760317562606667829, 0.8765941196519724254, 0.9999999999999796829 ) ) 
 REPRESENTATION_ITEM ( '' )  );
#31609=CARTESIAN_POINT ( 'NONE',  ( -24.47401588645412573, -14.84236399432835540, 59.39300237059229914 ) ) ;
#31610=CARTESIAN_POINT ( 'NONE',  ( -10.85841931818429629, -17.37798394237198707, 64.91267318220633342 ) ) ;
#31612=CARTESIAN_POINT ( 'NONE',  ( -18.96810653497118437, -7.981552352277012652, 63.50377208636563608 ) ) ;
#31614=CARTESIAN_POINT ( 'NONE',  ( -18.58222256244375714, -22.16864733340743143, 72.48499710573040034 ) ) ;
#31616=CARTESIAN_POINT ( 'NONE',  ( -13.42842659190323751, -9.059672259974458797, 64.09873707138190468 ) ) ;
#31618=ADVANCED_FACE ( 'NONE', ( #35833 ), #35113, .T. ) ;
#31619=CARTESIAN_POINT ( 'NONE',  ( -15.55171241031346696, -7.598245096497682205, 70.79485117658632021 ) ) ;
#31620=B_SPLINE_CURVE_WITH_KNOTS ( 'NONE', 3,
 ( #18802, #108, #15093, #11413, #20986, #43649, #27887, #31590, #17022, #1542 ),
 .UNSPECIFIED., .F., .F.,
 ( 4, 2, 2, 2, 4 ),
 ( 0.6272669072877363750, 0.7522669073072645318, 0.8772669073267927997, 1.002266907346321068, 1.127266907365849224 ),
 .UNSPECIFIED. ) ;
#31622=( BOUNDED_CURVE ( )  B_SPLINE_CURVE ( 3, ( #11656, #34051, #16297, #5009 ),
 .UNSPECIFIED., .F., .F. ) 
 B_SPLINE_CURVE_WITH_KNOTS ( ( 4, 4 ),
 ( 0.9074455897393666204, 1.000000000000000000 ),
 .UNSPECIFIED. ) 
 CURVE ( )  GEOMETRIC_REPRESENTATION_ITEM ( )  RATIONAL_B_SPLINE_CURVE ( ( 0.6983129098260977274, 0.7760317562607021991, 0.8765941196520029566, 1.000000000000000000 ) ) 
 REPRESENTATION_ITEM ( '' )  );
#31624=ORIENTED_EDGE ( 'NONE', *, *, #3993, .F. ) ;
#31626=CARTESIAN_POINT ( 'NONE',  ( -19.15588758283814386, -7.975065456818123621, 63.43649048405502811 ) ) ;
#31627=CARTESIAN_POINT ( 'NONE',  ( -11.76425449931685030, -10.60075661872682140, 70.85404331479517737 ) ) ;
#31629=CARTESIAN_POINT ( 'NONE',  ( -24.31294276048392078, -17.64623836558455494, 66.10503720318618548 ) ) ;
#31631=B_SPLINE_CURVE_WITH_KNOTS ( 'NONE', 3,
 ( #48556, #20827, #2108, #22222, #25913, #21068 ),
 .UNSPECIFIED., .F., .F.,
 ( 4, 2, 4 ),
 ( 0.2909959651135547443, 0.4999962229283157478, 0.7089964807430767513 ),
 .UNSPECIFIED. ) ;
#31632=CARTESIAN_POINT ( 'NONE',  ( -10.37182134788606369, -14.70778158825885207, 67.74311464738552502 ) ) ;
#31633=CARTESIAN_POINT ( 'NONE',  ( -24.41897112398753933, -17.37347453850100720, 69.59835118672229726 ) ) ;
#31634=ADVANCED_FACE ( 'NONE', ( #46701 ), #16646, .T. ) ;
#31635=EDGE_LOOP ( 'NONE', ( #11582, #31707 ) ) ;
#31636=CARTESIAN_POINT ( 'NONE',  ( -24.15060978519040091, -18.01196315242050261, 59.26024333157867119 ) ) ;
#31637=CARTESIAN_POINT ( 'NONE',  ( -17.04628442466378502, -7.819299381639010171, 74.26018289601994127 ) ) ;
#31638=B_SPLINE_CURVE_WITH_KNOTS ( 'NONE', 3,
 ( #45497, #202, #4137, #4603, #7343, #22342, #11754, #33643, #11270, #7582 ),
 .UNSPECIFIED., .F., .F.,
 ( 4, 2, 2, 2, 4 ),
 ( 0.6272669072877816721, 0.7522669073072908441, 0.8772669073268000162, 1.002266907346309299, 1.127266907365818360 ),
 .UNSPECIFIED. ) ;
#31639=ORIENTED_EDGE ( 'NONE', *, *, #4077, .F. ) ;
#31640=ADVANCED_FACE ( 'NONE', ( #35363 ), #12946, .T. ) ;
#31641=CARTESIAN_POINT ( 'NONE',  ( -10.44916082259176093, -15.83527127794237543, 64.80771589743309846 ) ) ;
#31642=ORIENTED_EDGE ( 'NONE', *, *, #21287, .F. ) ;
#31643=CARTESIAN_POINT ( 'NONE',  ( -17.70936732686351789, -22.25382107568847800, 58.66199285276312025 ) ) ;
#31644=CARTESIAN_POINT ( 'NONE',  ( -10.00315453233114305, -15.46673966334550521, 57.66818560559547535 ) ) ;
#31645=EDGE_CURVE ( 'NONE', #7173, #40988, #34462, .T. ) ;
#31646=CARTESIAN_POINT ( 'NONE',  ( -10.34160677812053208, -12.49813974654896320, 60.89829944146450913 ) ) ;
#31647=CARTESIAN_POINT ( 'NONE',  ( -13.99679447977218061, -20.97040113148658591, 71.94079819673058296 ) ) ;
#31648=VERTEX_POINT ( 'NONE', #1875 ) ;
#31651=ADVANCED_FACE ( 'NONE', ( #10244 ), #25259, .T. ) ;
#31652=CARTESIAN_POINT ( 'NONE',  ( -17.04413539470110095, -21.84925844046378174, 72.45071136019464575 ) ) ;
#31653=DIRECTION ( 'NONE',  ( -9.941263206155103325E-06, -7.040377910290660294E-06, 0.9999999999258021299 ) ) ;
#31656=CARTESIAN_POINT ( 'NONE',  ( -23.80321479583337307, -17.81075880182941873, 59.30378417737343710 ) ) ;
#31658=LINE ( 'NONE', #38545, #8741 ) ;
#31659=CARTESIAN_POINT ( 'NONE',  ( -11.55820670847359821, -18.73429759261662397, 71.83119032172525920 ) ) ;
#31661=VERTEX_POINT ( 'NONE', #22284 ) ;
#31662=CARTESIAN_POINT ( 'NONE',  ( -19.92776479198160189, -21.39998277484045275, 72.41950795000725805 ) ) ;
#31663=FACE_BOUND ( 'NONE', #13716, .T. ) ;
#31665=ORIENTED_EDGE ( 'NONE', *, *, #13065, .T. ) ;
#31666=VERTEX_POINT ( 'NONE', #3077 ) ;
#31668=LINE ( 'NONE', #43242, #20857 ) ;
#31669=EDGE_CURVE ( 'NONE', #36512, #11228, #2831, .T. ) ;
#31671=CARTESIAN_POINT ( 'NONE',  ( -12.62620107223973243, -19.90688791973824578, 68.62040837454712516 ) ) ;
#31672=ORIENTED_EDGE ( 'NONE', *, *, #9153, .T. ) ;
#31674=B_SPLINE_CURVE_WITH_KNOTS ( 'NONE', 3,
 ( #8755, #39743, #32370, #39505, #16832, #47388, #8988, #47141, #9721, #39012 ),
 .UNSPECIFIED., .F., .F.,
 ( 4, 2, 2, 2, 4 ),
 ( 0.000000000000000000, 0.2500000000000000000, 0.5000000000000000000, 0.7500000000000000000, 1.000000000000000000 ),
 .UNSPECIFIED. ) ;
#31676=CARTESIAN_POINT ( 'NONE',  ( -21.39967327233876659, -20.63170314183283693, 72.80974286114339122 ) ) ;
#31677=CARTESIAN_POINT ( 'NONE',  ( -24.87377682536729750, -14.89413262103416002, 59.40446719508604190 ) ) ;
#31678=CARTESIAN_POINT ( 'NONE',  ( -23.27832888692776336, -18.64690537560570860, 65.93275336871789705 ) ) ;
#31681=ORIENTED_EDGE ( 'NONE', *, *, #21206, .T. ) ;
#31684=CARTESIAN_POINT ( 'NONE',  ( -17.35617175722243744, -7.809413396383948935, 67.32039598645116030 ) ) ;
#31685=( BOUNDED_CURVE ( )  B_SPLINE_CURVE ( 3, ( #47988, #14226, #21880, #36880 ),
 .UNSPECIFIED., .F., .F. ) 
 B_SPLINE_CURVE_WITH_KNOTS ( ( 4, 4 ),
 ( 0.9074455897393720605, 1.000000000000000000 ),
 .UNSPECIFIED. ) 
 CURVE ( )  GEOMETRIC_REPRESENTATION_ITEM ( )  RATIONAL_B_SPLINE_CURVE ( ( 0.6983129098261073864, 0.7760317562607105257, 0.8765941196520080636, 1.000000000000000000 ) ) 
 REPRESENTATION_ITEM ( '' )  );
#31687=LINE ( 'NONE', #5833, #30442 ) ;
#31689=CARTESIAN_POINT ( 'NONE',  ( -10.37172597770583415, -14.90377323363781414, 71.21294082064301278 ) ) ;
#31690=CARTESIAN_POINT ( 'NONE',  ( -18.71951286714620011, -7.876189896296080128, 66.78582905748461940 ) ) ;
#31692=EDGE_CURVE ( 'NONE', #12494, #35872, #18866, .T. ) ;
#31694=CARTESIAN_POINT ( 'NONE',  ( -14.84764829735760827, -8.246537290690364230, 60.33468334944129197 ) ) ;
#31695=CARTESIAN_POINT ( 'NONE',  ( -22.88305391114024800, -19.19300254727433597, 59.11240555529296614 ) ) ;
#31696=CARTESIAN_POINT ( 'NONE',  ( -11.44812231001245095, -18.45465661085254538, 61.57710877958685103 ) ) ;
#31698=FACE_OUTER_BOUND ( 'NONE', #40146, .T. ) ;
#31699=ORIENTED_EDGE ( 'NONE', *, *, #13124, .T. ) ;
#31700=CARTESIAN_POINT ( 'NONE',  ( -24.42398663107514523, -15.65075326911586906, 73.01775867260030850 ) ) ;
#31702=EDGE_LOOP ( 'NONE', ( #21083, #39885, #32268, #6010, #10830 ) ) ;
#31703=CARTESIAN_POINT ( 'NONE',  ( -22.17130234749883044, -20.55096496926394778, 58.87947491310501391 ) ) ;
#31705=CARTESIAN_POINT ( 'NONE',  ( -17.06879511326789611, -7.767867012253359071, 73.97490359703523666 ) ) ;
#31707=ORIENTED_EDGE ( 'NONE', *, *, #39968, .T. ) ;
#31708=FACE_OUTER_BOUND ( 'NONE', #39033, .T. ) ;
#31711=CARTESIAN_POINT ( 'NONE',  ( -23.41687109752707840, -19.23545012094337991, 62.49373545795776863 ) ) ;
#31712=EDGE_CURVE ( 'NONE', #17470, #891, #6544, .T. ) ;
#31714=CARTESIAN_POINT ( 'NONE',  ( -15.81235419205221859, -7.945607373518419614, 67.42535135806457447 ) ) ;
#31717=EDGE_CURVE ( 'NONE', #11465, #39185, #37040, .T. ) ;
#31718=EDGE_CURVE ( 'NONE', #5083, #46221, #544, .T. ) ;
#31720=VERTEX_POINT ( 'NONE', #11214 ) ;
#31722=CARTESIAN_POINT ( 'NONE',  ( -14.25195992805637246, -21.10928659929985685, 72.13427513627219412 ) ) ;
#31724=FACE_OUTER_BOUND ( 'NONE', #30166, .T. ) ;
#31725=B_SPLINE_CURVE_WITH_KNOTS ( 'NONE', 3,
 ( #43108, #27604, #5698, #16510, #1982, #12340, #1022, #38430, #27359, #4718 ),
 .UNSPECIFIED., .F., .F.,
 ( 4, 2, 2, 2, 4 ),
 ( 0.000000000000000000, 0.2500000000000000000, 0.5000000000000000000, 0.7500000000000000000, 1.000000000000000000 ),
 .UNSPECIFIED. ) ;
#31727=CARTESIAN_POINT ( 'NONE',  ( -16.19813999035177332, -21.75179513556690480, 58.28585572029250983 ) ) ;
#31730=CARTESIAN_POINT ( 'NONE',  ( -22.79947183316497217, -19.38307604245925475, 59.02843669344121480 ) ) ;
#31733=FACE_OUTER_BOUND ( 'NONE', #17781, .T. ) ;
#31737=CARTESIAN_POINT ( 'NONE',  ( -19.70791841144649581, -21.90059652173849969, 65.72132139802793915 ) ) ;
#31739=CARTESIAN_POINT ( 'NONE',  ( -20.60942684424193772, -21.09890871138989965, 58.65947248567252359 ) ) ;
#31740=( BOUNDED_CURVE ( )  B_SPLINE_CURVE ( 3, ( #1513, #31559, #12836, #13063 ),
 .UNSPECIFIED., .F., .F. ) 
 B_SPLINE_CURVE_WITH_KNOTS ( ( 4, 4 ),
 ( 0.9074455897393626236, 1.000000000000000000 ),
 .UNSPECIFIED. ) 
 CURVE ( )  GEOMETRIC_REPRESENTATION_ITEM ( )  RATIONAL_B_SPLINE_CURVE ( ( 0.6983129098260858481, 0.7760317562606919850, 0.8765941196519967393, 1.000000000000000000 ) ) 
 REPRESENTATION_ITEM ( '' )  );
#31742=EDGE_CURVE ( 'NONE', #21230, #44055, #10602, .T. ) ;
#31743=CARTESIAN_POINT ( 'NONE',  ( -15.06802786744574085, -21.40078853851168716, 61.74486554635382163 ) ) ;
#31744=CARTESIAN_POINT ( 'NONE',  ( -24.00405284133622175, -11.31538449050870021, 66.52190887339411063 ) ) ;
#31745=CARTESIAN_POINT ( 'NONE',  ( -14.92297820767285543, -21.82695172143102624, 65.28409420478728009 ) ) ;
#31746=CARTESIAN_POINT ( 'NONE',  ( -24.48810873059073856, -17.17637193698283582, 73.06831349224263761 ) ) ;
#31748=( BOUNDED_CURVE ( )  B_SPLINE_CURVE ( 3, ( #43411, #38968, #16789, #8946 ),
 .UNSPECIFIED., .F., .F. ) 
 B_SPLINE_CURVE_WITH_KNOTS ( ( 4, 4 ),
 ( 0.000000000000000000, 0.4074455897393660653 ),
 .UNSPECIFIED. ) 
 CURVE ( )  GEOMETRIC_REPRESENTATION_ITEM ( )  RATIONAL_B_SPLINE_CURVE ( ( 1.000000000000000000, 0.4567392136813301917, 0.3561768502900296562, 0.6983129098260982826 ) ) 
 REPRESENTATION_ITEM ( '' )  );
#31749=CARTESIAN_POINT ( 'NONE',  ( -24.40836465796088106, -14.33371513455089641, 69.66891893576270434 ) ) ;
#31750=CARTESIAN_POINT ( 'NONE',  ( -24.79803955827340545, -15.87155823828966561, 69.78953433284350183 ) ) ;
#31751=EDGE_CURVE ( 'NONE', #29409, #30363, #40503, .T. ) ;
#31752=CARTESIAN_POINT ( 'NONE',  ( -10.15209110106313695, -13.18697342404853146, 74.86472985364514443 ) ) ;
#31753=FACE_OUTER_BOUND ( 'NONE', #40193, .T. ) ;
#31755=VERTEX_POINT ( 'NONE', #41003 ) ;
#31756=CARTESIAN_POINT ( 'NONE',  ( -14.91112529534803066, -8.221969756899694559, 57.13527940342243028 ) ) ;
#31758=CARTESIAN_POINT ( 'NONE',  ( -10.01516485041080884, -14.02680443569644098, 61.04104412929918055 ) ) ;
#31759=CARTESIAN_POINT ( 'NONE',  ( -10.42420408449255476, -14.84849159528415541, 71.43668796657122755 ) ) ;
#31760=VERTEX_POINT ( 'NONE', #25729 ) ;
#31765=DIRECTION ( 'NONE',  ( 0.9986807914369958405, -0.05134858142905002198, 1.286972170232540014E-09 ) ) ;
#31766=CARTESIAN_POINT ( 'NONE',  ( -14.91112529534803066, -8.221969756899694559, 57.13527940342243028 ) ) ;
#31767=CARTESIAN_POINT ( 'NONE',  ( -13.62794895237762027, -8.864113615554126469, 60.73950575333512347 ) ) ;
#31769=CARTESIAN_POINT ( 'NONE',  ( -16.27008067537174796, -7.904986561263926959, 60.50028479261354875 ) ) ;
#31770=CARTESIAN_POINT ( 'NONE',  ( -10.71605034603323148, -17.00400043661996108, 64.77172137060364321 ) ) ;
#31771=B_SPLINE_CURVE_WITH_KNOTS ( 'NONE', 1,
 ( #33071, #352 ),
 .UNSPECIFIED., .F., .F.,
 ( 2, 2 ),
 ( 0.000000000000000000, 1.000000000000000000 ),
 .UNSPECIFIED. ) ;
#31772=CARTESIAN_POINT ( 'NONE',  ( -12.94748490290780829, -9.362827855744063399, 71.14925333309587074 ) ) ;
#31773=ADVANCED_FACE ( 'NONE', ( #7028 ), #22046, .T. ) ;
#31774=EDGE_CURVE ( 'NONE', #15165, #47561, #8483, .T. ) ;
#31777=CARTESIAN_POINT ( 'NONE',  ( -17.59331747086620368, -7.761237804118463757, 63.85057029381062677 ) ) ;
#31778=CARTESIAN_POINT ( 'NONE',  ( -13.09267315849321456, -9.242013884934323187, 63.90946244383246011 ) ) ;
#31779=EDGE_LOOP ( 'NONE', ( #26754, #11124, #31672, #765, #2254 ) ) ;
#31783=CARTESIAN_POINT ( 'NONE',  ( -13.07701721570114373, -8.758813871092014480, 64.08759315826752356 ) ) ;
#31785=DIRECTION ( 'NONE',  ( -1.069388061899112173E-05, 2.778940573026428581E-06, 0.9999999999389591609 ) ) ;
#31788=EDGE_CURVE ( 'NONE', #41843, #42966, #31801, .T. ) ;
#31790=CARTESIAN_POINT ( 'NONE',  ( -13.00736322368352305, -8.809467263174131091, 64.08663386113011029 ) ) ;
#31791=CARTESIAN_POINT ( 'NONE',  ( -10.45263246496396370, -15.85887054471568014, 64.80771565453923699 ) ) ;
#31792=CARTESIAN_POINT ( 'NONE',  ( -23.71751471349159601, -11.63122711669449494, 63.23746208799618529 ) ) ;
#31793=CARTESIAN_POINT ( 'NONE',  ( -10.79968008669509594, -11.40033872506984203, 67.72526294861705765 ) ) ;
#31794=VERTEX_POINT ( 'NONE', #12177 ) ;
#31795=VERTEX_POINT ( 'NONE', #41480 ) ;
#31796=AXIS2_PLACEMENT_3D ( 'NONE', #31609, #27666, #28151 ) ;
#31797=VERTEX_POINT ( 'NONE', #15610 ) ;
#31798=EDGE_CURVE ( 'NONE', #38648, #24162, #23589, .T. ) ;
#31799=CARTESIAN_POINT ( 'NONE',  ( -20.37299732318518508, -8.405577239842552117, 66.93104082189577753 ) ) ;
#31801=LINE ( 'NONE', #34573, #39436 ) ;
#31802=CARTESIAN_POINT ( 'NONE',  ( -24.11794058161805054, -12.76166764465371628, 69.77243002474142486 ) ) ;
#31803=ORIENTED_EDGE ( 'NONE', *, *, #27340, .T. ) ;
#31804=CARTESIAN_POINT ( 'NONE',  ( -22.01092588021961660, -8.937695967300268052, 66.84805351483468883 ) ) ;
#31805=CARTESIAN_POINT ( 'NONE',  ( -10.00117635412376593, -15.44487469174752903, 57.68297500625912733 ) ) ;
#31809=CARTESIAN_POINT ( 'NONE',  ( -18.91460061187875397, -21.70800071742875303, 58.66940498489888256 ) ) ;
#31810=VERTEX_POINT ( 'NONE', #37783 ) ;
#31811=FACE_OUTER_BOUND ( 'NONE', #12798, .T. ) ;
#31812=VERTEX_POINT ( 'NONE', #19566 ) ;
#31813=CARTESIAN_POINT ( 'NONE',  ( -10.12183752415379168, -13.33225746603075024, 74.80004878148187686 ) ) ;
#31814=ORIENTED_EDGE ( 'NONE', *, *, #24281, .F. ) ;
#31817=CARTESIAN_POINT ( 'NONE',  ( -19.30128557755455532, -21.60500301973953086, 58.81035253397666196 ) ) ;
#31818=EDGE_LOOP ( 'NONE', ( #1490, #36402, #30340, #9014, #36798 ) ) ;
#31820=CARTESIAN_POINT ( 'NONE',  ( -24.70020460095737391, -16.41001677332389619, 59.30049291089687102 ) ) ;
#31821=CARTESIAN_POINT ( 'NONE',  ( -20.18941624216641273, -7.891347737435665977, 73.83601159825586535 ) ) ;
#31822=CARTESIAN_POINT ( 'NONE',  ( -13.66248979885904724, -8.905658713984221819, 56.96967804944289071 ) ) ;
#31823=CARTESIAN_POINT ( 'NONE',  ( -17.79108452803360763, -21.84994637594637368, 58.69081321602850920 ) ) ;
#31824=CARTESIAN_POINT ( 'NONE',  ( -14.97188219925329378, -8.199429090594037461, 57.14999999999994884 ) ) ;
#31827=CARTESIAN_POINT ( 'NONE',  ( -24.66897215040500768, -13.07252427436380238, 63.01076963004065590 ) ) ;
#31828=DIRECTION ( 'NONE',  ( -1.420801289120338746E-06, -1.008342286982562053E-05, 0.9999999999481529178 ) ) ;
#31830=CARTESIAN_POINT ( 'NONE',  ( -14.39999285742539392, -8.436745619719848932, 63.99798883827455143 ) ) ;
#31833=EDGE_CURVE ( 'NONE', #41418, #15882, #3599, .T. ) ;
#31836=CARTESIAN_POINT ( 'NONE',  ( -16.32575768948312600, -7.844986739114469643, 60.21500614002425777 ) ) ;
#31837=CARTESIAN_POINT ( 'NONE',  ( -20.88147576600584543, -8.209942340109883219, 60.02620652709861560 ) ) ;
#31838=ORIENTED_EDGE ( 'NONE', *, *, #14219, .T. ) ;
#31840=CARTESIAN_POINT ( 'NONE',  ( -10.64211600630794585, -13.07553005057556739, 68.02366961159727055 ) ) ;
#31841=CARTESIAN_POINT ( 'NONE',  ( -12.68656345882633296, -9.059469911947932275, 70.89279414395181789 ) ) ;
#31842=CARTESIAN_POINT ( 'NONE',  ( -12.79725860806972904, -20.12850118792689358, 71.95653676770096752 ) ) ;
#31843=CARTESIAN_POINT ( 'NONE',  ( -21.17518949801557682, -8.835587824813147861, 73.60128454375318086 ) ) ;
#31845=CARTESIAN_POINT ( 'NONE',  ( -24.80874383141511430, -15.79476513899138368, 69.71024349780060447 ) ) ;
#31846=CARTESIAN_POINT ( 'NONE',  ( -17.01436944207222624, -7.370403393205478437, 74.21664194825545735 ) ) ;
#31848=CARTESIAN_POINT ( 'NONE',  ( -23.69410989900737263, -17.92519740713284548, 59.19305441470095985 ) ) ;
#31851=EDGE_CURVE ( 'NONE', #25517, #14949, #2119, .T. ) ;
#31853=CARTESIAN_POINT ( 'NONE',  ( -24.56291696005103375, -12.67795903866814733, 69.91209651719337614 ) ) ;
#31856=VERTEX_POINT ( 'NONE', #8023 ) ;
#31857=ORIENTED_EDGE ( 'NONE', *, *, #9886, .T. ) ;
#31859=EDGE_CURVE ( 'NONE', #43190, #11955, #608, .T. ) ;
#31860=CARTESIAN_POINT ( 'NONE',  ( -16.91478550490786859, -21.84108428878278119, 72.18015306840750611 ) ) ;
#31861=CARTESIAN_POINT ( 'NONE',  ( -15.31091769494271837, -7.608297704863611344, 53.63095954094025331 ) ) ;
#31862=CARTESIAN_POINT ( 'NONE',  ( -11.85162103594838001, -10.49015045520576983, 71.25420998615621215 ) ) ;
#31864=LINE ( 'NONE', #13614, #16632 ) ;
#31865=CARTESIAN_POINT ( 'NONE',  ( -14.25068793291388225, -8.513811817964199946, 71.02957628655769895 ) ) ;
#31866=AXIS2_PLACEMENT_3D ( 'NONE', #9855, #32954, #17699 ) ;
#31867=VERTEX_POINT ( 'NONE', #22527 ) ;
#31868=FACE_OUTER_BOUND ( 'NONE', #21430, .T. ) ;
#31869=CARTESIAN_POINT ( 'NONE',  ( -24.84449963183508459, -13.71944596863515464, 53.49999999999994316 ) ) ;
#31870=( BOUNDED_SURFACE ( )  B_SPLINE_SURFACE ( 3, 1, ( 
 ( #28618, #5964 ),
 ( #43648, #36232 ),
 ( #24204, #46618 ),
 ( #10147, #42914 ),
 ( #28851, #35743 ),
 ( #2515, #17519 ),
 ( #12861, #25167 ) ),
 .UNSPECIFIED., .T., .F., .F. ) 
 B_SPLINE_SURFACE_WITH_KNOTS ( ( 4, 3, 4 ),
 ( 2, 2 ),
 ( 0.000000000000000000, 0.5000000000000000000, 1.000000000000000000 ),
 ( 0.000000000000000000, 1.000000000000000000 ),
 .UNSPECIFIED. ) 
 GEOMETRIC_REPRESENTATION_ITEM ( )  RATIONAL_B_SPLINE_SURFACE ( (
 ( 1.000000000000000000, 1.000000000000000000),
 ( 0.3333333333333335369, 0.3333333333333330373),
 ( 0.3333333333333335369, 0.3333333333333330373),
 ( 1.000000000000000000, 1.000000000000000000),
 ( 0.3333333333333333703, 0.3333333333333333703),
 ( 0.3333333333333333703, 0.3333333333333333703),
 ( 1.000000000000000000, 1.000000000000000000) ) ) 
 REPRESENTATION_ITEM ( '' )  SURFACE ( )  );
#31874=EDGE_LOOP ( 'NONE', ( #2894, #34434, #19082, #28154, #46728 ) ) ;
#31875=CARTESIAN_POINT ( 'NONE',  ( -23.29918339618657086, -19.39037464299967439, 58.99915238703562181 ) ) ;
#31876=FACE_OUTER_BOUND ( 'NONE', #47165, .T. ) ;
#31878=CARTESIAN_POINT ( 'NONE',  ( -18.06139463723319949, -21.83834701327926808, 58.56120650458878174 ) ) ;
#31881=( BOUNDED_CURVE ( )  B_SPLINE_CURVE ( 3, ( #47621, #47139, #10442, #13853 ),
 .UNSPECIFIED., .F., .F. ) 
 B_SPLINE_CURVE_WITH_KNOTS ( ( 4, 4 ),
 ( 0.5000000000000000000, 0.9074455897393649551 ),
 .UNSPECIFIED. ) 
 CURVE ( )  GEOMETRIC_REPRESENTATION_ITEM ( )  RATIONAL_B_SPLINE_CURVE ( ( 0.9999999999999747979, 0.4567392136813269166, 0.3561768502900459210, 0.6983129098261047218 ) ) 
 REPRESENTATION_ITEM ( '' )  );
#31883=DIRECTION ( 'NONE',  ( 0.9477661110324760996, -0.3189661404888857188, 2.738326501554841424E-08 ) ) ;
#31884=ORIENTED_EDGE ( 'NONE', *, *, #16620, .T. ) ;
#31885=CARTESIAN_POINT ( 'NONE',  ( -10.66137368835686416, -12.80659570974005668, 60.68364890423993785 ) ) ;
#31887=( BOUNDED_CURVE ( )  B_SPLINE_CURVE ( 3, ( #14946, #19153, #30255, #3397 ),
 .UNSPECIFIED., .F., .F. ) 
 B_SPLINE_CURVE_WITH_KNOTS ( ( 4, 4 ),
 ( 0.000000000000000000, 0.4074455897393697290 ),
 .UNSPECIFIED. ) 
 CURVE ( )  GEOMETRIC_REPRESENTATION_ITEM ( )  RATIONAL_B_SPLINE_CURVE ( ( 1.000000000000000000, 0.4567392136813214210, 0.3561768502900264366, 0.6983129098261150469 ) ) 
 REPRESENTATION_ITEM ( '' )  );
#31888=CARTESIAN_POINT ( 'NONE',  ( -24.14679772577363437, -12.68507108172156883, 70.05770892828130059 ) ) ;
#31889=CARTESIAN_POINT ( 'NONE',  ( -12.09300774956044755, -19.42703681131052562, 58.34171032836335513 ) ) ;
#31890=B_SPLINE_CURVE_WITH_KNOTS ( 'NONE', 1,
 ( #24843, #43565 ),
 .UNSPECIFIED., .F., .F.,
 ( 2, 2 ),
 ( 0.000000000000000000, 1.000000000000000000 ),
 .UNSPECIFIED. ) ;
#31891=CARTESIAN_POINT ( 'NONE',  ( -17.36015951656348832, -7.359395083792595216, 67.20534920880687935 ) ) ;
#31895=CARTESIAN_POINT ( 'NONE',  ( -11.14403518423954509, -11.71714199058991568, 67.72750603396154645 ) ) ;
#31896=CARTESIAN_POINT ( 'NONE',  ( -24.09024125277505490, -17.10388469556238533, 72.88336035478459962 ) ) ;
#31899=( BOUNDED_CURVE ( )  B_SPLINE_CURVE ( 3, ( #4553, #12426, #30916, #31139 ),
 .UNSPECIFIED., .F., .F. ) 
 B_SPLINE_CURVE_WITH_KNOTS ( ( 4, 4 ),
 ( 0.000000000000000000, 0.4074455897393652881 ),
 .UNSPECIFIED. ) 
 CURVE ( )  GEOMETRIC_REPRESENTATION_ITEM ( )  RATIONAL_B_SPLINE_CURVE ( ( 1.000000000000000000, 0.4567392136813347991, 0.3561768502900313216, 0.6983129098260896228 ) ) 
 REPRESENTATION_ITEM ( '' )  );
#31901=VERTEX_POINT ( 'NONE', #45919 ) ;
#31902=VERTEX_POINT ( 'NONE', #27197 ) ;
#31905=CARTESIAN_POINT ( 'NONE',  ( -14.04312441377786946, -20.93869165529285681, 71.92607738043835752 ) ) ;
#31906=EDGE_CURVE ( 'NONE', #47012, #39245, #7161, .T. ) ;
#31907=CARTESIAN_POINT ( 'NONE',  ( -11.46028008028683942, -18.56947564720590194, 61.56238700194530367 ) ) ;
#31908=CARTESIAN_POINT ( 'NONE',  ( -21.21137848157293249, -8.922231491198125752, 73.79231820712855949 ) ) ;
#31910=CARTESIAN_POINT ( 'NONE',  ( -13.40403435948632094, -9.078590645922671953, 60.45452650781103898 ) ) ;
#31911=ORIENTED_EDGE ( 'NONE', *, *, #11267, .F. ) ;
#31914=CARTESIAN_POINT ( 'NONE',  ( -10.74573065459234478, -12.54952415110468422, 60.81325645027152405 ) ) ;
#31916=CARTESIAN_POINT ( 'NONE',  ( -21.06494968540953749, -21.30903997076690359, 62.15825466738357363 ) ) ;
#31917=CARTESIAN_POINT ( 'NONE',  ( -23.66220297886838964, -18.88224728823589160, 69.55017934013164904 ) ) ;
#31918=EDGE_CURVE ( 'NONE', #13753, #14422, #41102, .T. ) ;
#31920=ORIENTED_EDGE ( 'NONE', *, *, #26076, .T. ) ;
#31921=CYLINDRICAL_SURFACE ( 'NONE', #47735, 0.1499999999999975242 ) ;
#31923=CARTESIAN_POINT ( 'NONE',  ( -12.51438907681678536, -19.79882988928595822, 64.86674880260875398 ) ) ;
#31925=DIRECTION ( 'NONE',  ( 1.011289380940303784E-05, -7.260693215641691253E-06, 0.9999999999225058778 ) ) ;
#31926=AXIS2_PLACEMENT_3D ( 'NONE', #22977, #45374, #46341 ) ;
#31927=CARTESIAN_POINT ( 'NONE',  ( -10.37394849890712401, -14.76283852923608464, 71.61310637325181006 ) ) ;
#31928=CARTESIAN_POINT ( 'NONE',  ( -16.35517392334946152, -21.72711159609176690, 58.47688641158507039 ) ) ;
#31929=CARTESIAN_POINT ( 'NONE',  ( -14.47284097950645432, -7.968636565268744754, 63.89704670002799247 ) ) ;
#31931=FACE_OUTER_BOUND ( 'NONE', #39553, .T. ) ;
#31932=EDGE_CURVE ( 'NONE', #31812, #30116, #40388, .T. ) ;
#31933=B_SPLINE_CURVE_WITH_KNOTS ( 'NONE', 1,
 ( #4762, #12144 ),
 .UNSPECIFIED., .F., .F.,
 ( 2, 2 ),
 ( 0.000000000000000000, 1.000000000000000000 ),
 .UNSPECIFIED. ) ;
#31934=CARTESIAN_POINT ( 'NONE',  ( -23.07906255732286738, -9.958937815627702861, 66.72677557046061736 ) ) ;
#31935=CARTESIAN_POINT ( 'NONE',  ( -10.48067351556794158, -16.03044098841782628, 68.27767830705533925 ) ) ;
#31941=VERTEX_POINT ( 'NONE', #39432 ) ;
#31942=DIRECTION ( 'NONE',  ( 1.069446452691264255E-06, -1.103879811633194674E-06, 0.9999999999988189447 ) ) ;
#31943=CARTESIAN_POINT ( 'NONE',  ( -21.80761170843182128, -20.26838994411330219, 58.99272793439983076 ) ) ;
#31944=CARTESIAN_POINT ( 'NONE',  ( -24.07704370891653767, -17.14264987453632827, 72.89808101046212130 ) ) ;
#31947=CARTESIAN_POINT ( 'NONE',  ( -17.42409385541300892, -14.80920654474439679, 56.49999999999994316 ) ) ;
#31948=CYLINDRICAL_SURFACE ( 'NONE', #33693, 0.1500000000000015488 ) ;
#31951=EDGE_CURVE ( 'NONE', #22984, #44794, #22257, .T. ) ;
#31952=CARTESIAN_POINT ( 'NONE',  ( -17.39742543611924575, -7.759256981132187647, 67.32039592192056432 ) ) ;
#31953=CARTESIAN_POINT ( 'NONE',  ( -24.43112999227502868, -15.58634490091467129, 73.00303748142292193 ) ) ;
#31954=ORIENTED_EDGE ( 'NONE', *, *, #8265, .T. ) ;
#31957=CARTESIAN_POINT ( 'NONE',  ( -20.09559670342926552, -21.27944071986311414, 72.63152148437504252 ) ) ;
#31958=EDGE_CURVE ( 'NONE', #24336, #15165, #10031, .T. ) ;
#31959=CARTESIAN_POINT ( 'NONE',  ( -10.99655682251556144, -18.57624055219563175, 57.99209882808910521 ) ) ;
#31961=CARTESIAN_POINT ( 'NONE',  ( -11.74997710522658600, -10.61883180769318535, 70.96892938659537720 ) ) ;
#31963=CARTESIAN_POINT ( 'NONE',  ( -12.25434508901797770, -20.17367074759813406, 65.05170324716399932 ) ) ;
#31964=CARTESIAN_POINT ( 'NONE',  ( -18.94863228570505598, -7.922318267881538922, 70.46248317377518333 ) ) ;
#31966=ORIENTED_EDGE ( 'NONE', *, *, #26807, .F. ) ;
#31967=ORIENTED_EDGE ( 'NONE', *, *, #47856, .T. ) ;
#31968=EDGE_CURVE ( 'NONE', #42734, #43742, #25235, .T. ) ;
#31972=CARTESIAN_POINT ( 'NONE',  ( -23.67460871249246068, -11.65500680865467054, 66.65044377215316729 ) ) ;
#31973=CARTESIAN_POINT ( 'NONE',  ( -14.78750812280958726, -21.29541618567930072, 61.74673429867123531 ) ) ;
#31974=CARTESIAN_POINT ( 'NONE',  ( -24.54031182138101741, -12.60405816868659912, 69.87904686005836652 ) ) ;
#31975=( BOUNDED_CURVE ( )  B_SPLINE_CURVE ( 3, ( #12394, #27415, #34066, #42450 ),
 .UNSPECIFIED., .F., .F. ) 
 B_SPLINE_CURVE_WITH_KNOTS ( ( 4, 4 ),
 ( 0.4074455897393611248, 0.5000000000000000000 ),
 .UNSPECIFIED. ) 
 CURVE ( )  GEOMETRIC_REPRESENTATION_ITEM ( )  RATIONAL_B_SPLINE_CURVE ( ( 0.6983129098260971723, 0.7760317562606624531, 0.8765941196519518863, 0.9999999999999374944 ) ) 
 REPRESENTATION_ITEM ( '' )  );
#31976=EDGE_CURVE ( 'NONE', #40331, #23337, #33967, .T. ) ;
#31978=B_SPLINE_CURVE_WITH_KNOTS ( 'NONE', 3,
 ( #9043, #31435, #39310, #16881, #1387, #27740, #24551, #16402, #43260, #12477 ),
 .UNSPECIFIED., .F., .F.,
 ( 4, 2, 2, 2, 4 ),
 ( 0.1272669073658265759, 0.2522669073439348653, 0.3772669073220431546, 0.5022669073001514439, 0.6272669072782597333 ),
 .UNSPECIFIED. ) ;
#31982=CARTESIAN_POINT ( 'NONE',  ( -11.77169895589660698, -10.59578386207264700, 74.43885051664024388 ) ) ;
#31983=CARTESIAN_POINT ( 'NONE',  ( -24.11881394502254849, -17.01995806294775448, 73.16863963025599560 ) ) ;
#31985=VERTEX_POINT ( 'NONE', #30304 ) ;
#31987=CARTESIAN_POINT ( 'NONE',  ( -21.34511485531846020, -8.950139844736156647, 73.90128722075769474 ) ) ;
#31989=CARTESIAN_POINT ( 'NONE',  ( -10.58203424369019174, -16.28808381980452324, 71.73284965287206205 ) ) ;
#31990=ADVANCED_FACE ( 'NONE', ( #10597 ), #22173, .T. ) ;
#31992=CARTESIAN_POINT ( 'NONE',  ( -18.67229701437506506, -7.919758800372044050, 74.02991576449618094 ) ) ;
#31993=CARTESIAN_POINT ( 'NONE',  ( -15.53265176333180619, -21.60105060138385014, 72.33103357390284316 ) ) ;
#31994=CARTESIAN_POINT ( 'NONE',  ( -23.51785719624223958, -11.36449344406884343, 70.19210750610864125 ) ) ;
#31995=ORIENTED_EDGE ( 'NONE', *, *, #31414, .T. ) ;
#31996=CARTESIAN_POINT ( 'NONE',  ( -10.37599212182869124, -14.63324797960940593, 71.34254748307667171 ) ) ;
#31999=ORIENTED_EDGE ( 'NONE', *, *, #26397, .F. ) ;
#32000=PLANE ( 'NONE',  #39025 ) ;
#32001=EDGE_LOOP ( 'NONE', ( #1335, #35156, #17426, #20005, #26774 ) ) ;
#32002=CARTESIAN_POINT ( 'NONE',  ( -18.32857756213031664, -22.20418371868804996, 68.93019407337365578 ) ) ;
#32004=EDGE_LOOP ( 'NONE', ( #44449, #37044, #4599, #46595, #46508 ) ) ;
#32005=CARTESIAN_POINT ( 'NONE',  ( -14.11063322135152909, -21.03236308526469855, 72.21135587486895702 ) ) ;
#32007=CARTESIAN_POINT ( 'NONE',  ( -10.64864687305616009, -11.71119991730035181, 74.73652894950812708 ) ) ;
#32008=CARTESIAN_POINT ( 'NONE',  ( -10.88209242003807908, -17.29963164818252608, 64.62739380462950578 ) ) ;
#32009=ORIENTED_EDGE ( 'NONE', *, *, #36866, .F. ) ;
#32010=CARTESIAN_POINT ( 'NONE',  ( -16.12274100365893048, -7.931235850141636234, 60.30914399322803376 ) ) ;
#32012=CARTESIAN_POINT ( 'NONE',  ( -24.60327268654570432, -12.81871823346896022, 66.40223105660061265 ) ) ;
#32013=B_SPLINE_CURVE_WITH_KNOTS ( 'NONE', 1,
 ( #42714, #30666 ),
 .UNSPECIFIED., .F., .F.,
 ( 2, 2 ),
 ( 0.000000000000000000, 1.000000000000000000 ),
 .UNSPECIFIED. ) ;
#32015=ORIENTED_EDGE ( 'NONE', *, *, #47009, .F. ) ;
#32016=ORIENTED_EDGE ( 'NONE', *, *, #32517, .T. ) ;
#32017=CARTESIAN_POINT ( 'NONE',  ( -23.80579133695118443, -18.65331559044849641, 72.87029906539265767 ) ) ;
#32018=CARTESIAN_POINT ( 'NONE',  ( -24.86242983737997747, -14.39095285025967286, 66.36788159907001727 ) ) ;
#32019=EDGE_LOOP ( 'NONE', ( #15196, #40845 ) ) ;
#32020=CARTESIAN_POINT ( 'NONE',  ( -11.46043843694620357, -11.04924462883820802, 57.50903212149482613 ) ) ;
#32024=( BOUNDED_CURVE ( )  B_SPLINE_CURVE ( 3, ( #39829, #5383, #35638, #6095 ),
 .UNSPECIFIED., .F., .F. ) 
 B_SPLINE_CURVE_WITH_KNOTS ( ( 4, 4 ),
 ( 0.000000000000000000, 0.4074455897393618464 ),
 .UNSPECIFIED. ) 
 CURVE ( )  GEOMETRIC_REPRESENTATION_ITEM ( )  RATIONAL_B_SPLINE_CURVE ( ( 1.000000000000000000, 0.4567392136813371861, 0.3561768502900322653, 0.6983129098260852929 ) ) 
 REPRESENTATION_ITEM ( '' )  );
#32025=CARTESIAN_POINT ( 'NONE',  ( -24.59706333651279664, -12.79617740830267891, 66.48742133194130588 ) ) ;
#32026=CARTESIAN_POINT ( 'NONE',  ( -15.69736699998981422, -8.025519224215527103, 70.60989840319118116 ) ) ;
#32027=VERTEX_POINT ( 'NONE', #33216 ) ;
#32028=ADVANCED_FACE ( 'NONE', ( #4195 ), #45317, .T. ) ;
#32029=CARTESIAN_POINT ( 'NONE',  ( -20.77150381139373536, -8.660956599501332676, 60.12508712995069260 ) ) ;
#32030=CARTESIAN_POINT ( 'NONE',  ( -22.85367851456767596, -9.707840327915473466, 73.65973829363548475 ) ) ;
#32031=CARTESIAN_POINT ( 'NONE',  ( -10.78921115435649369, -11.42050183187454770, 67.75718084852192646 ) ) ;
#32032=( BOUNDED_CURVE ( )  B_SPLINE_CURVE ( 3, ( #20013, #35976, #17266, #9177 ),
 .UNSPECIFIED., .F., .F. ) 
 B_SPLINE_CURVE_WITH_KNOTS ( ( 4, 4 ),
 ( 0.000000000000000000, 0.4074455897393650106 ),
 .UNSPECIFIED. ) 
 CURVE ( )  GEOMETRIC_REPRESENTATION_ITEM ( )  RATIONAL_B_SPLINE_CURVE ( ( 1.000000000000000000, 0.4567392136813301362, 0.3561768502900296562, 0.6983129098260983936 ) ) 
 REPRESENTATION_ITEM ( '' )  );
#32036=VECTOR ( 'NONE', #46484, 1000.000000000000000 ) ;
#32037=ORIENTED_EDGE ( 'NONE', *, *, #32122, .T. ) ;
#32038=B_SPLINE_CURVE_WITH_KNOTS ( 'NONE', 1,
 ( #4422, #45568 ),
 .UNSPECIFIED., .F., .F.,
 ( 2, 2 ),
 ( 0.000000000000000000, 1.000000000000000000 ),
 .UNSPECIFIED. ) ;
#32040=CARTESIAN_POINT ( 'NONE',  ( -22.57823294519915436, -10.07257407465379551, 70.02680971841948576 ) ) ;
#32042=EDGE_LOOP ( 'NONE', ( #11334, #26497, #28740, #41875, #7331 ) ) ;
#32043=EDGE_CURVE ( 'NONE', #26823, #17855, #22657, .T. ) ;
#32047=EDGE_CURVE ( 'NONE', #16726, #21204, #1152, .T. ) ;
#32050=DIRECTION ( 'NONE',  ( -0.06306825763707681054, 0.9980092158285026605, 2.415158932891090200E-08 ) ) ;
#32051=CARTESIAN_POINT ( 'NONE',  ( -19.37462041217285957, -21.99941596162432589, 58.56861435762115775 ) ) ;
#32052=ORIENTED_EDGE ( 'NONE', *, *, #12934, .F. ) ;
#32053=CARTESIAN_POINT ( 'NONE',  ( -15.74091245749827195, -8.014583633770426374, 67.24893180729357312 ) ) ;
#32055=DIRECTION ( 'NONE',  ( -0.7670373483544790094, -0.6416024518573233415, 2.496223344567222537E-08 ) ) ;
#32057=CARTESIAN_POINT ( 'NONE',  ( -16.27095827323975996, -7.851109476482911909, 64.08499918177189159 ) ) ;
#32058=LINE ( 'NONE', #24442, #25982 ) ;
#32060=ORIENTED_EDGE ( 'NONE', *, *, #35644, .F. ) ;
#32061=CARTESIAN_POINT ( 'NONE',  ( -24.26499789074519597, -17.75976756996305639, 62.65856417960095825 ) ) ;
#32063=CARTESIAN_POINT ( 'NONE',  ( -23.65624089557865872, -11.51332380282628343, 66.57214514605458078 ) ) ;
#32064=VECTOR ( 'NONE', #43751, 1000.000000000000000 ) ;
#32073=CARTESIAN_POINT ( 'NONE',  ( -12.07950851572364748, -19.41234162675539920, 58.01862405632531505 ) ) ;
#32074=CARTESIAN_POINT ( 'NONE',  ( -19.98515930221110892, -21.80534510432024575, 69.09515851530258601 ) ) ;
#32075=CARTESIAN_POINT ( 'NONE',  ( -12.40380818233537141, -19.68739593843253033, 61.69678633575567517 ) ) ;
#32076=ADVANCED_FACE ( 'NONE', ( #19197 ), #15043, .T. ) ;
#32078=FACE_OUTER_BOUND ( 'NONE', #31779, .T. ) ;
#32079=CARTESIAN_POINT ( 'NONE',  ( -24.31482301288783532, -13.31912224170856618, 59.66267924674055934 ) ) ;
#32080=ORIENTED_EDGE ( 'NONE', *, *, #27664, .T. ) ;
#32081=CARTESIAN_POINT ( 'NONE',  ( -11.25385002771267473, -18.98553936430136702, 68.40345028533118921 ) ) ;
#32083=CARTESIAN_POINT ( 'NONE',  ( -23.07906255732286738, -9.958937815627702861, 66.72677557046061736 ) ) ;
#32085=CARTESIAN_POINT ( 'NONE',  ( -22.34470984022960138, -19.78791505225649416, 69.17417989488706098 ) ) ;
#32086=CARTESIAN_POINT ( 'NONE',  ( -16.92616160843403961, -22.24260109534890262, 72.27269065110013457 ) ) ;
#32087=VERTEX_POINT ( 'NONE', #8365 ) ;
#32090=CARTESIAN_POINT ( 'NONE',  ( -20.89788161767221197, -20.94431024770144489, 62.39999296070408974 ) ) ;
#32091=CARTESIAN_POINT ( 'NONE',  ( -23.72463725732412954, -17.86031838844568043, 59.28761838504880899 ) ) ;
#32093=DIRECTION ( 'NONE',  ( -9.009793368474262471E-08, 1.813722298394044057E-06, -0.9999999999983512078 ) ) ;
#32094=CARTESIAN_POINT ( 'NONE',  ( -9.979603215878100286, -14.52052451035377345, 68.04295550616701860 ) ) ;
#32096=CARTESIAN_POINT ( 'NONE',  ( -13.42842738616806209, -9.059671689720946830, 64.02019725504824521 ) ) ;
#32098=CARTESIAN_POINT ( 'NONE',  ( -24.03287018854308954, -12.34366040360348471, 73.24225467054047556 ) ) ;
#32099=FACE_OUTER_BOUND ( 'NONE', #47268, .T. ) ;
#32101=VERTEX_POINT ( 'NONE', #30790 ) ;
#32103=CARTESIAN_POINT ( 'NONE',  ( -11.49688049385020960, -18.62690763749001732, 64.76179218520603342 ) ) ;
#32105=CARTESIAN_POINT ( 'NONE',  ( -17.74514309872235884, -7.766371812394021745, 60.37500991003656736 ) ) ;
#32106=AXIS2_PLACEMENT_3D ( 'NONE', #10817, #37141, #3428 ) ;
#32107=VECTOR ( 'NONE', #9431, 1000.000000000000000 ) ;
#32109=DIRECTION ( 'NONE',  ( -0.2196488028684550620, -0.9755790093059855117, 7.835600157697873389E-08 ) ) ;
#32110=EDGE_CURVE ( 'NONE', #32931, #784, #44095, .T. ) ;
#32112=ORIENTED_EDGE ( 'NONE', *, *, #8949, .F. ) ;
#32113=CARTESIAN_POINT ( 'NONE',  ( -11.33492925930432804, -11.25580429380516456, 60.97325962342065253 ) ) ;
#32115=CARTESIAN_POINT ( 'NONE',  ( -18.90996479553717791, -7.968725069611966916, 66.90071784165556323 ) ) ;
#32116=B_SPLINE_CURVE_WITH_KNOTS ( 'NONE', 1,
 ( #30236, #42032 ),
 .UNSPECIFIED., .F., .F.,
 ( 2, 2 ),
 ( 0.000000000000000000, 1.000000000000000000 ),
 .UNSPECIFIED. ) ;
#32118=CARTESIAN_POINT ( 'NONE',  ( -16.78411497196904278, -21.83009869597353259, 68.69560651670111895 ) ) ;
#32120=ORIENTED_EDGE ( 'NONE', *, *, #27405, .T. ) ;
#32122=EDGE_CURVE ( 'NONE', #33156, #44748, #13738, .T. ) ;
#32123=CARTESIAN_POINT ( 'NONE',  ( -10.31413044408767554, -17.03453498993188475, 57.94406477676061229 ) ) ;
#32126=ADVANCED_FACE ( 'NONE', ( #45566 ), #32340, .T. ) ;
#32128=EDGE_CURVE ( 'NONE', #13240, #32374, #33903, .T. ) ;
#32130=LINE ( 'NONE', #43955, #19759 ) ;
#32131=VERTEX_POINT ( 'NONE', #24113 ) ;
#32132=CARTESIAN_POINT ( 'NONE',  ( -22.10219206297270489, -9.524287713326932803, 63.33586711951718229 ) ) ;
#32135=FACE_OUTER_BOUND ( 'NONE', #16769, .T. ) ;
#32137=CARTESIAN_POINT ( 'NONE',  ( -20.05785487306503256, -7.839488668639425839, 73.83441365354759967 ) ) ;
#32138=CARTESIAN_POINT ( 'NONE',  ( -17.36175868705992897, -7.359389033274929659, 67.06393689457253515 ) ) ;
#32141=FACE_OUTER_BOUND ( 'NONE', #33213, .T. ) ;
#32143=DIRECTION ( 'NONE',  ( -4.615129100576721730E-07, 1.699487034244351503E-08, -0.9999999999998933076 ) ) ;
#32145=CARTESIAN_POINT ( 'NONE',  ( -14.26613035333006785, -8.061623769020160424, 67.45986280861907858 ) ) ;
#32146=CARTESIAN_POINT ( 'NONE',  ( -24.29719970949782137, -16.39516428949632854, 62.89328972680635843 ) ) ;
#32147=ORIENTED_EDGE ( 'NONE', *, *, #14060, .F. ) ;
#32148=CARTESIAN_POINT ( 'NONE',  ( -23.88415222675040539, -17.63235122089636775, 62.47360984996718969 ) ) ;
#32151=EDGE_LOOP ( 'NONE', ( #18359, #6234 ) ) ;
#32152=ORIENTED_EDGE ( 'NONE', *, *, #16204, .T. ) ;
#32153=ORIENTED_EDGE ( 'NONE', *, *, #13355, .T. ) ;
#32154=CARTESIAN_POINT ( 'NONE',  ( -14.00884526327672397, -20.92003366206770210, 71.94224368477696885 ) ) ;
#32156=CARTESIAN_POINT ( 'NONE',  ( -23.72751372599721620, -11.76491108559917720, 59.55523859581371937 ) ) ;
#32157=DIRECTION ( 'NONE',  ( -0.9118114225829224706, -0.4106092176842892627, -5.589476761700638069E-08 ) ) ;
#32158=CARTESIAN_POINT ( 'NONE',  ( -12.05483347687720475, -10.31798811457585963, 67.79896870046731294 ) ) ;
#32159=CARTESIAN_POINT ( 'NONE',  ( -10.72958667791015763, -16.85608332250551200, 57.70377195876292120 ) ) ;
#32163=CARTESIAN_POINT ( 'NONE',  ( -21.02116742812006223, -20.87599269455877860, 61.99982634431184181 ) ) ;
#32165=( BOUNDED_SURFACE ( )  B_SPLINE_SURFACE ( 3, 1, ( 
 ( #26990, #46441 ),
 ( #45951, #42258 ),
 ( #38292, #1611 ),
 ( #9015, #16622 ),
 ( #31659, #16376 ),
 ( #27714, #27473 ),
 ( #24036, #42015 ) ),
 .UNSPECIFIED., .T., .F., .F. ) 
 B_SPLINE_SURFACE_WITH_KNOTS ( ( 4, 3, 4 ),
 ( 2, 2 ),
 ( 0.000000000000000000, 0.5000000000000000000, 1.000000000000000000 ),
 ( 0.000000000000000000, 1.000000000000000000 ),
 .UNSPECIFIED. ) 
 GEOMETRIC_REPRESENTATION_ITEM ( )  RATIONAL_B_SPLINE_SURFACE ( (
 ( 1.000000000000000000, 1.000000000000000000),
 ( 0.3333333333333335369, 0.3333333333333330373),
 ( 0.3333333333333335369, 0.3333333333333330373),
 ( 1.000000000000000000, 1.000000000000000000),
 ( 0.3333333333333333703, 0.3333333333333333703),
 ( 0.3333333333333333703, 0.3333333333333333703),
 ( 1.000000000000000000, 1.000000000000000000) ) ) 
 REPRESENTATION_ITEM ( '' )  SURFACE ( )  );
#32166=EDGE_CURVE ( 'NONE', #3873, #8865, #4672, .T. ) ;
#32168=ORIENTED_EDGE ( 'NONE', *, *, #28098, .T. ) ;
#32169=ADVANCED_FACE ( 'NONE', ( #980 ), #11821, .T. ) ;
#32172=CARTESIAN_POINT ( 'NONE',  ( -24.80746943141735983, -15.80390768895026987, 69.57661537956182940 ) ) ;
#32174=( BOUNDED_SURFACE ( )  B_SPLINE_SURFACE ( 3, 1, ( 
 ( #34289, #42185 ),
 ( #8445, #4759 ),
 ( #23479, #16056 ),
 ( #31097, #46119 ),
 ( #5007, #16296 ),
 ( #5240, #24451 ),
 ( #5962, #1536 ) ),
 .UNSPECIFIED., .T., .F., .F. ) 
 B_SPLINE_SURFACE_WITH_KNOTS ( ( 4, 3, 4 ),
 ( 2, 2 ),
 ( 0.000000000000000000, 0.5000000000000000000, 1.000000000000000000 ),
 ( 0.000000000000000000, 1.000000000000000000 ),
 .UNSPECIFIED. ) 
 GEOMETRIC_REPRESENTATION_ITEM ( )  RATIONAL_B_SPLINE_SURFACE ( (
 ( 1.000000000000000000, 1.000000000000000000),
 ( 0.3333333333333335369, 0.3333333333333330373),
 ( 0.3333333333333335369, 0.3333333333333330373),
 ( 1.000000000000000000, 1.000000000000000000),
 ( 0.3333333333333333703, 0.3333333333333333703),
 ( 0.3333333333333333703, 0.3333333333333333703),
 ( 1.000000000000000000, 1.000000000000000000) ) ) 
 REPRESENTATION_ITEM ( '' )  SURFACE ( )  );
#32176=( BOUNDED_SURFACE ( )  B_SPLINE_SURFACE ( 3, 1, ( 
 ( #35591, #24541 ),
 ( #37211, #39537 ),
 ( #2350, #5817 ),
 ( #47173, #18014 ),
 ( #48077, #21975 ),
 ( #3259, #14313 ),
 ( #18263, #29364 ) ),
 .UNSPECIFIED., .T., .F., .F. ) 
 B_SPLINE_SURFACE_WITH_KNOTS ( ( 4, 3, 4 ),
 ( 2, 2 ),
 ( 0.000000000000000000, 0.5000000000000000000, 1.000000000000000000 ),
 ( 0.000000000000000000, 1.000000000000000000 ),
 .UNSPECIFIED. ) 
 GEOMETRIC_REPRESENTATION_ITEM ( )  RATIONAL_B_SPLINE_SURFACE ( (
 ( 1.000000000000000000, 1.000000000000000000),
 ( 0.3333333333333335369, 0.3333333333333330373),
 ( 0.3333333333333335369, 0.3333333333333330373),
 ( 1.000000000000000000, 1.000000000000000000),
 ( 0.3333333333333333703, 0.3333333333333333703),
 ( 0.3333333333333333703, 0.3333333333333333703),
 ( 1.000000000000000000, 1.000000000000000000) ) ) 
 REPRESENTATION_ITEM ( '' )  SURFACE ( )  );
#32177=AXIS2_PLACEMENT_3D ( 'NONE', #24947, #47601, #13833 ) ;
#32179=CARTESIAN_POINT ( 'NONE',  ( -11.67943375510494697, -18.89645239624664441, 68.50217487844219022 ) ) ;
#32180=CARTESIAN_POINT ( 'NONE',  ( -22.53538519471304369, -20.22938801946909138, 65.74775819791243237 ) ) ;
#32181=ADVANCED_FACE ( 'NONE', ( #12536 ), #27561, .T. ) ;
#32182=ORIENTED_EDGE ( 'NONE', *, *, #13355, .F. ) ;
#32183=VECTOR ( 'NONE', #8774, 1000.000000000000114 ) ;
#32185=CARTESIAN_POINT ( 'NONE',  ( -22.58023486647882550, -9.989541079992143580, 66.69749311060769514 ) ) ;
#32186=CARTESIAN_POINT ( 'NONE',  ( -21.01124108229941001, -20.87838065962769463, 65.88453944495783787 ) ) ;
#32188=CARTESIAN_POINT ( 'NONE',  ( -20.68074900106244840, -21.00565013100700895, 58.64475149681948807 ) ) ;
#32189=( BOUNDED_CURVE ( )  B_SPLINE_CURVE ( 3, ( #10551, #45272, #3905, #29267 ),
 .UNSPECIFIED., .F., .F. ) 
 B_SPLINE_CURVE_WITH_KNOTS ( ( 4, 4 ),
 ( 0.9074455897393650661, 1.000000000000000000 ),
 .UNSPECIFIED. ) 
 CURVE ( )  GEOMETRIC_REPRESENTATION_ITEM ( )  RATIONAL_B_SPLINE_CURVE ( ( 0.6983129098260953960, 0.7760317562607003117, 0.8765941196520018464, 1.000000000000000000 ) ) 
 REPRESENTATION_ITEM ( '' )  );
#32190=ORIENTED_EDGE ( 'NONE', *, *, #39878, .T. ) ;
#32191=CARTESIAN_POINT ( 'NONE',  ( -16.16748626245079379, -22.20318634978239203, 54.27966884056655061 ) ) ;
#32192=CARTESIAN_POINT ( 'NONE',  ( -10.37541943412130863, -14.96049300415475436, 75.08306784598362071 ) ) ;
#32193=ORIENTED_EDGE ( 'NONE', *, *, #47721, .F. ) ;
#32194=CARTESIAN_POINT ( 'NONE',  ( -19.19784432118828121, -7.503115221654976352, 54.02312124697527196 ) ) ;
#32196=CARTESIAN_POINT ( 'NONE',  ( -24.51063837352987207, -17.11019555850099039, 72.99680753360935626 ) ) ;
#32197=CARTESIAN_POINT ( 'NONE',  ( -23.23616409499838653, -18.79948708312782557, 65.82389430043846801 ) ) ;
#32198=VERTEX_POINT ( 'NONE', #24361 ) ;
#32199=FACE_OUTER_BOUND ( 'NONE', #38967, .T. ) ;
#32201=CARTESIAN_POINT ( 'NONE',  ( -23.69044173319201363, -11.56146079933792237, 59.63803016077844177 ) ) ;
#32202=CARTESIAN_POINT ( 'NONE',  ( -23.79253477450064835, -17.84199475294676063, 62.77360976034447759 ) ) ;
#32203=ORIENTED_EDGE ( 'NONE', *, *, #47185, .T. ) ;
#32204=CARTESIAN_POINT ( 'NONE',  ( -23.73493062035036871, -11.65830449210876552, 59.48235750863023696 ) ) ;
#32206=ORIENTED_EDGE ( 'NONE', *, *, #15457, .F. ) ;
#32208=CARTESIAN_POINT ( 'NONE',  ( -24.15165104652898620, -11.60707627830156952, 63.13873557927141889 ) ) ;
#32210=VECTOR ( 'NONE', #32055, 1000.000000000000114 ) ;
#32211=CARTESIAN_POINT ( 'NONE',  ( -10.02191625022346955, -15.65273779443635327, 61.15293638507743168 ) ) ;
#32213=CARTESIAN_POINT ( 'NONE',  ( -12.29382548908870909, -9.968360400451484082, 64.12094344831615444 ) ) ;
#32214=CARTESIAN_POINT ( 'NONE',  ( -11.81178328723415660, -10.62567094834893311, 74.73885052262691886 ) ) ;
#32216=CARTESIAN_POINT ( 'NONE',  ( -12.01648201532752935, -10.28590752825076926, 67.64896869922044687 ) ) ;
#32217=AXIS2_PLACEMENT_3D ( 'NONE', #44553, #28801, #25584 ) ;
#32218=CARTESIAN_POINT ( 'NONE',  ( -23.04402284766838349, -19.06632961612601918, 59.16938527523783620 ) ) ;
#32219=EDGE_LOOP ( 'NONE', ( #14695, #35310, #32785, #13133, #44941 ) ) ;
#32221=CARTESIAN_POINT ( 'NONE',  ( -24.45381059137804058, -15.38184444469599299, 72.88814935371863157 ) ) ;
#32223=CARTESIAN_POINT ( 'NONE',  ( -10.63483715323753565, -17.87674169505483235, 71.75213630217804450 ) ) ;
#32224=CARTESIAN_POINT ( 'NONE',  ( -15.92486819940615916, -7.971526783001416483, 67.44007330037176473 ) ) ;
#32225=AXIS2_PLACEMENT_3D ( 'NONE', #26885, #12095, #34740 ) ;
#32226=CARTESIAN_POINT ( 'NONE',  ( -22.38860277241858654, -19.74596283091575089, 72.87230326346423226 ) ) ;
#32227=CARTESIAN_POINT ( 'NONE',  ( -20.75714322117456945, -21.47287265741918461, 58.83130466214971221 ) ) ;
#32228=EDGE_CURVE ( 'NONE', #28368, #40867, #20099, .T. ) ;
#32231=CARTESIAN_POINT ( 'NONE',  ( -21.89264518680100835, -20.26253109894388160, 58.77915004610761684 ) ) ;
#32232=CARTESIAN_POINT ( 'NONE',  ( -10.23413987642072165, -12.85783452779354086, 67.84558203418174571 ) ) ;
#32235=CARTESIAN_POINT ( 'NONE',  ( -14.72744631621160494, -8.295007313424175521, 60.60524229057013201 ) ) ;
#32236=CARTESIAN_POINT ( 'NONE',  ( -10.08080428754885105, -16.06609343925254763, 68.23413777636764621 ) ) ;
#32237=VERTEX_POINT ( 'NONE', #40103 ) ;
#32239=CARTESIAN_POINT ( 'NONE',  ( -13.41301606045583128, -21.08813317394188758, 65.17284274790917209 ) ) ;
#32240=CARTESIAN_POINT ( 'NONE',  ( -12.81584026802821974, -9.539888144265397329, 74.61922966036955529 ) ) ;
#32241=EDGE_CURVE ( 'NONE', #3454, #8916, #19388, .T. ) ;
#32242=VECTOR ( 'NONE', #24909, 1000.000000000000114 ) ;
#32243=CARTESIAN_POINT ( 'NONE',  ( -10.48020486909296523, -13.57339180249324784, 74.56328874061136958 ) ) ;
#32244=CARTESIAN_POINT ( 'NONE',  ( -15.63492442327685872, -7.577064122408605051, 70.74956509023566298 ) ) ;
#32245=EDGE_CURVE ( 'NONE', #997, #17474, #34028, .T. ) ;
#32246=CARTESIAN_POINT ( 'NONE',  ( -14.86627107493491984, -7.811969877679347363, 56.96504568426624360 ) ) ;
#32247=DIRECTION ( 'NONE',  ( 0.5562740912439652075, 0.8309988781043535777, 7.851267780903552829E-08 ) ) ;
#32248=ORIENTED_EDGE ( 'NONE', *, *, #34075, .F. ) ;
#32252=CARTESIAN_POINT ( 'NONE',  ( -21.52725980274252393, -9.076272844571150245, 70.43132538913752683 ) ) ;
#32254=EDGE_CURVE ( 'NONE', #38352, #25448, #28199, .T. ) ;
#32255=ORIENTED_EDGE ( 'NONE', *, *, #26397, .T. ) ;
#32256=DIRECTION ( 'NONE',  ( 1.568615312922261716E-06, 3.599473019824118231E-09, -0.9999999999987697619 ) ) ;
#32258=EDGE_LOOP ( 'NONE', ( #1735, #21608, #38509, #8627, #34951 ) ) ;
#32259=CARTESIAN_POINT ( 'NONE',  ( -23.70015292207183322, -18.82353835121273988, 69.47867366044893345 ) ) ;
#32262=CARTESIAN_POINT ( 'NONE',  ( -14.59650283654637271, -21.27602155829186259, 61.78033139454115030 ) ) ;
#32263=ORIENTED_EDGE ( 'NONE', *, *, #38261, .T. ) ;
#32264=DIRECTION ( 'NONE',  ( 0.9477661110324762106, -0.3189661404888857743, 2.738326501554842086E-08 ) ) ;
#32265=DIRECTION ( 'NONE',  ( -3.549360974554993999E-17, 6.371834667797928663E-18, 1.000000000000000000 ) ) ;
#32266=CARTESIAN_POINT ( 'NONE',  ( -24.03160971261424805, -17.26750559640275640, 69.71339792588547368 ) ) ;
#32267=DIRECTION ( 'NONE',  ( 0.8244078399817416081, 0.5659962132175737626, 7.627400655798536990E-08 ) ) ;
#32268=ORIENTED_EDGE ( 'NONE', *, *, #3898, .T. ) ;
#32271=CARTESIAN_POINT ( 'NONE',  ( -24.30686519033400828, -16.08525344109053634, 62.60831050571806600 ) ) ;
#32272=ORIENTED_EDGE ( 'NONE', *, *, #31263, .F. ) ;
#32273=CARTESIAN_POINT ( 'NONE',  ( -17.63801222301331251, -7.812475947363076045, 60.27163990856254117 ) ) ;
#32276=CARTESIAN_POINT ( 'NONE',  ( -10.42593258563390712, -14.97222729729766044, 74.81281306951763099 ) ) ;
#32279=CARTESIAN_POINT ( 'NONE',  ( -19.42896739221782809, -21.56812523091047851, 62.29503644570711174 ) ) ;
#32281=ORIENTED_EDGE ( 'NONE', *, *, #42818, .T. ) ;
#32282=LINE ( 'NONE', #5927, #16264 ) ;
#32283=CARTESIAN_POINT ( 'NONE',  ( -14.88752825633713606, -21.38711684928872003, 61.63600437443167834 ) ) ;
#32284=AXIS2_PLACEMENT_3D ( 'NONE', #40886, #2963, #17733 ) ;
#32285=CARTESIAN_POINT ( 'NONE',  ( -22.84295050904691138, -9.696552564295293664, 73.67499385951728641 ) ) ;
#32288=ORIENTED_EDGE ( 'NONE', *, *, #44137, .T. ) ;
#32289=B_SPLINE_CURVE_WITH_KNOTS ( 'NONE', 3,
 ( #20007, #16046, #35008, #47075, #46107, #13316, #39681, #46830, #24187, #5952 ),
 .UNSPECIFIED., .F., .F.,
 ( 4, 2, 2, 2, 4 ),
 ( 0.6272669072782346422, 0.7522669073001380102, 0.8772669073220412672, 1.002266907343944524, 1.127266907365847892 ),
 .UNSPECIFIED. ) ;
#32290=ORIENTED_EDGE ( 'NONE', *, *, #8078, .F. ) ;
#32291=CARTESIAN_POINT ( 'NONE',  ( -24.47066272824306665, -14.57993217219608795, 62.99824437345093031 ) ) ;
#32293=CARTESIAN_POINT ( 'NONE',  ( -10.00731240618708462, -14.10555136595099945, 61.10316694600977172 ) ) ;
#32294=VECTOR ( 'NONE', #17831, 1000.000000000000227 ) ;
#32295=ORIENTED_EDGE ( 'NONE', *, *, #23237, .F. ) ;
#32296=CARTESIAN_POINT ( 'NONE',  ( -16.16815255583688682, -7.465780795815666337, 60.39302609866659566 ) ) ;
#32299=CARTESIAN_POINT ( 'NONE',  ( -13.70540922824953078, -21.34346593505471290, 53.76227901944321275 ) ) ;
#32302=VERTEX_POINT ( 'NONE', #25800 ) ;
#32303=DIRECTION ( 'NONE',  ( -2.575747231244379256E-06, 1.267954838346457742E-05, 0.9999999999162972886 ) ) ;
#32304=ORIENTED_EDGE ( 'NONE', *, *, #26264, .T. ) ;
#32305=CARTESIAN_POINT ( 'NONE',  ( -11.96181431063714484, -19.87549516500596525, 58.11177798925346139 ) ) ;
#32306=DIRECTION ( 'NONE',  ( 0.4683180279402421875, -0.8835599723313410925, 4.589753183357165266E-08 ) ) ;
#32307=ADVANCED_FACE ( 'NONE', ( #14936 ), #35183, .T. ) ;
#32311=CARTESIAN_POINT ( 'NONE',  ( -20.16691314815865255, -21.73601827195274794, 72.58974169946205279 ) ) ;
#32312=DIRECTION ( 'NONE',  ( -0.3478314405900310158, -0.9375570856950865561, 0.000000000000000000 ) ) ;
#32313=ADVANCED_FACE ( 'NONE', ( #18154 ), #37107, .T. ) ;
#32315=( BOUNDED_CURVE ( )  B_SPLINE_CURVE ( 3, ( #43176, #9451, #39481, #21007 ),
 .UNSPECIFIED., .F., .F. ) 
 B_SPLINE_CURVE_WITH_KNOTS ( ( 4, 4 ),
 ( 0.000000000000000000, 0.4074455897393719495 ),
 .UNSPECIFIED. ) 
 CURVE ( )  GEOMETRIC_REPRESENTATION_ITEM ( )  RATIONAL_B_SPLINE_CURVE ( ( 1.000000000000000000, 0.4567392136813254733, 0.3561768502900278799, 0.6983129098261073864 ) ) 
 REPRESENTATION_ITEM ( '' )  );
#32316=CARTESIAN_POINT ( 'NONE',  ( -22.51726279860821478, -19.68384809141797120, 72.64400547081167758 ) ) ;
#32317=CARTESIAN_POINT ( 'NONE',  ( -23.99312268326606201, -11.29471679256767125, 66.60709928216182618 ) ) ;
#32319=VERTEX_POINT ( 'NONE', #15188 ) ;
#32320=VECTOR ( 'NONE', #25266, 1000.000000000000341 ) ;
#32321=CARTESIAN_POINT ( 'NONE',  ( -17.59211730330735435, -7.811223398082945302, 63.85057029380297422 ) ) ;
#32322=CARTESIAN_POINT ( 'NONE',  ( -11.88825570308877211, -19.09342130031698304, 71.79571799091935702 ) ) ;
#32324=DIRECTION ( 'NONE',  ( -0.9959323210854037489, 0.09010444948746665350, 2.601165157765155817E-08 ) ) ;
#32325=CARTESIAN_POINT ( 'NONE',  ( -19.96356197875924110, -21.81308687000214874, 69.04144176266291311 ) ) ;
#32326=CARTESIAN_POINT ( 'NONE',  ( -24.26647797581570032, -16.29234248507571081, 62.82158650101273167 ) ) ;
#32327=ORIENTED_EDGE ( 'NONE', *, *, #6136, .F. ) ;
#32329=CARTESIAN_POINT ( 'NONE',  ( -21.18398698114219769, -21.24092341087395752, 65.69958654271196963 ) ) ;
#32334=CARTESIAN_POINT ( 'NONE',  ( -12.79487214375358839, -8.971058656907512585, 71.03580700614087107 ) ) ;
#32335=CARTESIAN_POINT ( 'NONE',  ( -23.12302657392458016, -18.95946740514217765, 62.35406880581413702 ) ) ;
#32336=CARTESIAN_POINT ( 'NONE',  ( -17.00424539706637361, -22.24753552852095950, 72.32576587678371993 ) ) ;
#32337=VERTEX_POINT ( 'NONE', #33403 ) ;
#32340=( BOUNDED_SURFACE ( )  B_SPLINE_SURFACE ( 3, 1, ( 
 ( #27315, #42827 ),
 ( #5161, #35178 ),
 ( #19934, #1449 ),
 ( #1205, #19440 ),
 ( #38640, #4420 ),
 ( #12294, #19693 ),
 ( #8620, #42101 ) ),
 .UNSPECIFIED., .T., .F., .F. ) 
 B_SPLINE_SURFACE_WITH_KNOTS ( ( 4, 3, 4 ),
 ( 2, 2 ),
 ( 0.000000000000000000, 0.5000000000000000000, 1.000000000000000000 ),
 ( 0.000000000000000000, 1.000000000000000000 ),
 .UNSPECIFIED. ) 
 GEOMETRIC_REPRESENTATION_ITEM ( )  RATIONAL_B_SPLINE_SURFACE ( (
 ( 1.000000000000000000, 1.000000000000000000),
 ( 0.3333333333333335369, 0.3333333333333330373),
 ( 0.3333333333333335369, 0.3333333333333330373),
 ( 1.000000000000000000, 1.000000000000000000),
 ( 0.3333333333333333703, 0.3333333333333333703),
 ( 0.3333333333333333703, 0.3333333333333333703),
 ( 1.000000000000000000, 1.000000000000000000) ) ) 
 REPRESENTATION_ITEM ( '' )  SURFACE ( )  );
#32341=ADVANCED_FACE ( 'NONE', ( #48696 ), #47968, .T. ) ;
#32342=CARTESIAN_POINT ( 'NONE',  ( -10.83536388074712598, -17.31742051234312640, 64.92739380450886699 ) ) ;
#32345=EDGE_CURVE ( 'NONE', #25341, #31554, #41070, .T. ) ;
#32346=EDGE_CURVE ( 'NONE', #35350, #47755, #31162, .T. ) ;
#32349=CARTESIAN_POINT ( 'NONE',  ( -21.66670709193873634, -21.01608934220539027, 54.02312124697527906 ) ) ;
#32350=FILL_AREA_STYLE ('',( #43676 ) ) ;
#32351=CARTESIAN_POINT ( 'NONE',  ( -22.51726247777427758, -19.68384842258191725, 72.94400547081133368 ) ) ;
#32352=CARTESIAN_POINT ( 'NONE',  ( -21.13865688766858142, -18.88351593698935105, 53.69233794759168177 ) ) ;
#32353=CARTESIAN_POINT ( 'NONE',  ( -11.58273374504420516, -10.94902345701756730, 57.39830395176002042 ) ) ;
#32354=EDGE_LOOP ( 'NONE', ( #40065, #36987, #45866, #24375, #3207 ) ) ;
#32358=CARTESIAN_POINT ( 'NONE',  ( -13.19865322091292370, -9.228302641792829775, 63.98234477754206750 ) ) ;
#32359=VECTOR ( 'NONE', #37076, 999.9999999999998863 ) ;
#32360=FACE_OUTER_BOUND ( 'NONE', #18038, .T. ) ;
#32362=CARTESIAN_POINT ( 'NONE',  ( -23.00382044653182945, -10.58231046269237829, 59.60203429539187425 ) ) ;
#32369=CARTESIAN_POINT ( 'NONE',  ( -17.99281169931935409, -22.23759039661181802, 61.99723177674093222 ) ) ;
#32370=CARTESIAN_POINT ( 'NONE',  ( -12.90644216781524811, -9.461594527793637965, 74.33539679058131355 ) ) ;
#32372=CARTESIAN_POINT ( 'NONE',  ( -10.64331041279003642, -16.74977650942914309, 58.10249305398041741 ) ) ;
#32373=CARTESIAN_POINT ( 'NONE',  ( -18.64924655410156973, -21.70115844427598617, 72.39396872550724993 ) ) ;
#32374=VERTEX_POINT ( 'NONE', #36861 ) ;
#32376=EDGE_CURVE ( 'NONE', #46955, #13463, #34644, .T. ) ;
#32377=CARTESIAN_POINT ( 'NONE',  ( -24.41290230071813383, -15.73718799205770935, 69.82747671076849372 ) ) ;
#32378=CARTESIAN_POINT ( 'NONE',  ( -24.69822963474414479, -13.19963333263893190, 59.54763306486673713 ) ) ;
#32379=ORIENTED_EDGE ( 'NONE', *, *, #44027, .T. ) ;
#32380=CARTESIAN_POINT ( 'NONE',  ( -21.84103824432629892, -20.31425616591354455, 62.37872033649042436 ) ) ;
#32381=CARTESIAN_POINT ( 'NONE',  ( -19.80301194551662647, -21.44571530912114099, 68.93482476707502826 ) ) ;
#32384=CARTESIAN_POINT ( 'NONE',  ( -10.76763551407085373, -17.13171859787639661, 61.45743118825841833 ) ) ;
#32387=CARTESIAN_POINT ( 'NONE',  ( -23.35262004249965528, -18.62986191134476499, 65.70900547832829375 ) ) ;
#32388=ORIENTED_EDGE ( 'NONE', *, *, #1273, .T. ) ;
#32389=CARTESIAN_POINT ( 'NONE',  ( -18.50932193227059486, -21.77517953109191140, 72.58510940649487964 ) ) ;
#32391=VERTEX_POINT ( 'NONE', #14434 ) ;
#32392=LINE ( 'NONE', #32148, #1913 ) ;
#32393=VERTEX_POINT ( 'NONE', #22350 ) ;
#32394=EDGE_CURVE ( 'NONE', #10444, #37822, #22897, .T. ) ;
#32395=ADVANCED_FACE ( 'NONE', ( #18639 ), #6859, .T. ) ;
#32397=ORIENTED_EDGE ( 'NONE', *, *, #8543, .T. ) ;
#32398=CARTESIAN_POINT ( 'NONE',  ( -18.75871633935533112, -7.479601620491856728, 70.49255234965639261 ) ) ;
#32400=CARTESIAN_POINT ( 'NONE',  ( -12.81450638858427737, -9.474958432310776502, 74.46923006088778152 ) ) ;
#32403=ORIENTED_EDGE ( 'NONE', *, *, #41450, .F. ) ;
#32404=ORIENTED_EDGE ( 'NONE', *, *, #19369, .T. ) ;
#32405=EDGE_CURVE ( 'NONE', #5198, #27631, #21968, .T. ) ;
#32406=EDGE_CURVE ( 'NONE', #27240, #20428, #26457, .T. ) ;
#32408=CARTESIAN_POINT ( 'NONE',  ( -11.47692143115784447, -10.32194432912726612, 74.56168219205009962 ) ) ;
#32409=CARTESIAN_POINT ( 'NONE',  ( -23.21840254553152860, -18.73701819181863470, 66.12389378410178153 ) ) ;
#32411=ORIENTED_EDGE ( 'NONE', *, *, #44462, .F. ) ;
#32413=CARTESIAN_POINT ( 'NONE',  ( -23.92594474375018621, -12.07410526313069887, 59.78235714318768856 ) ) ;
#32415=LINE ( 'NONE', #17846, #38596 ) ;
#32419=CARTESIAN_POINT ( 'NONE',  ( -22.40414025807384135, -9.889859561998502357, 73.55449203743623343 ) ) ;
#32422=ORIENTED_EDGE ( 'NONE', *, *, #21502, .F. ) ;
#32424=CARTESIAN_POINT ( 'NONE',  ( -11.25989433568914855, -11.38792842781904469, 64.44882039367774951 ) ) ;
#32425=CARTESIAN_POINT ( 'NONE',  ( -10.38996398380459318, -17.26349193673827287, 61.30743118028662764 ) ) ;
#32427=CARTESIAN_POINT ( 'NONE',  ( -20.76327734442119066, -20.96149803180293247, 58.71763231260016624 ) ) ;
#32428=CARTESIAN_POINT ( 'NONE',  ( -18.24929096724884658, -21.81104555038653103, 68.82986815895560540 ) ) ;
#32429=VERTEX_POINT ( 'NONE', #19387 ) ;
#32430=CARTESIAN_POINT ( 'NONE',  ( -11.10470791607724550, -18.75498134223953883, 61.46206221440264983 ) ) ;
#32431=CARTESIAN_POINT ( 'NONE',  ( -9.983342151361524586, -14.43473985968501339, 67.99766747612557083 ) ) ;
#32432=ORIENTED_EDGE ( 'NONE', *, *, #31918, .F. ) ;
#32433=CARTESIAN_POINT ( 'NONE',  ( -21.06635048418738165, -21.30826373965517817, 62.29966805574095901 ) ) ;
#32434=CARTESIAN_POINT ( 'NONE',  ( -13.68948761385293800, -20.72981242130265045, 61.74319555004421289 ) ) ;
#32435=CARTESIAN_POINT ( 'NONE',  ( -24.11881394502254849, -17.01995806294775448, 73.16863963025599560 ) ) ;
#32438=CARTESIAN_POINT ( 'NONE',  ( -21.98930223717667332, -9.502567820616416583, 60.02171225693719947 ) ) ;
#32439=CARTESIAN_POINT ( 'NONE',  ( -19.05445285856947990, -7.539616405147045342, 67.04038455535467733 ) ) ;
#32440=DIRECTION ( 'NONE',  ( 0.5351595679979588294, 0.8447509909909772796, 1.584200591473933048E-17 ) ) ;
#32442=CARTESIAN_POINT ( 'NONE',  ( -23.91010245674826251, -17.57297063409389537, 62.75888927877479517 ) ) ;
#32443=CARTESIAN_POINT ( 'NONE',  ( -24.65061889199765233, -12.99785316138012270, 62.87618224063605510 ) ) ;
#32446=VERTEX_POINT ( 'NONE', #42536 ) ;
#32447=CARTESIAN_POINT ( 'NONE',  ( -23.59778322581706789, -11.38860327479983603, 63.10785482661193413 ) ) ;
#32448=CARTESIAN_POINT ( 'NONE',  ( -13.00647906721701297, -9.304695462141918227, 64.06513368409466125 ) ) ;
#32449=CARTESIAN_POINT ( 'NONE',  ( -11.33842141989115504, -11.24277552151799497, 57.20902919577373069 ) ) ;
#32451=CARTESIAN_POINT ( 'NONE',  ( -10.50893933415051507, -13.43540278197274063, 74.96345540680638919 ) ) ;
#32452=CARTESIAN_POINT ( 'NONE',  ( -19.41474841345058522, -21.52018966427049307, 62.29503644830997189 ) ) ;
#32453=( BOUNDED_CURVE ( )  B_SPLINE_CURVE ( 3, ( #19592, #39027, #34600, #5305 ),
 .UNSPECIFIED., .F., .F. ) 
 B_SPLINE_CURVE_WITH_KNOTS ( ( 4, 4 ),
 ( 4.712388980384689674, 4.921828490624009511 ),
 .UNSPECIFIED. ) 
 CURVE ( )  GEOMETRIC_REPRESENTATION_ITEM ( )  RATIONAL_B_SPLINE_CURVE ( ( 1.000000000000000000, 0.9963479302455154896, 0.9963479302455154896, 1.000000000000000000 ) ) 
 REPRESENTATION_ITEM ( '' )  );
#32454=CARTESIAN_POINT ( 'NONE',  ( -21.25771322586351886, -21.19734792347225749, 65.72307405023113347 ) ) ;
#32455=CARTESIAN_POINT ( 'NONE',  ( -12.19296425323979882, -20.11394705437778896, 65.02821367433101329 ) ) ;
#32456=CARTESIAN_POINT ( 'NONE',  ( -10.86088752666615065, -11.28245350497684818, 67.80519939327926693 ) ) ;
#32457=ORIENTED_EDGE ( 'NONE', *, *, #28655, .F. ) ;
#32459=EDGE_CURVE ( 'NONE', #40402, #12408, #18800, .T. ) ;
#32460=DIRECTION ( 'NONE',  ( -2.842893132017732099E-07, 1.090087350972575656E-07, -0.9999999999999535927 ) ) ;
#32463=CARTESIAN_POINT ( 'NONE',  ( -21.80947544975385810, -9.353161466788067813, 63.19153755920122251 ) ) ;
#32464=CARTESIAN_POINT ( 'NONE',  ( -18.97054302448013985, -7.521389842619064403, 67.08567168106696954 ) ) ;
#32465=CARTESIAN_POINT ( 'NONE',  ( -11.06571665854733766, -11.88142629960236718, 71.31534231900744203 ) ) ;
#32466=EDGE_CURVE ( 'NONE', #29981, #44852, #5288, .T. ) ;
#32469=ORIENTED_EDGE ( 'NONE', *, *, #34694, .F. ) ;
#32470=CARTESIAN_POINT ( 'NONE',  ( -20.04849592361258104, -21.35284569240296548, 72.69006679631316103 ) ) ;
#32472=CARTESIAN_POINT ( 'NONE',  ( -14.60628068055246942, -7.912570010659592867, 60.36350377317607752 ) ) ;
#32473=CARTESIAN_POINT ( 'NONE',  ( -11.17436915487612303, -18.86448991569423939, 64.86990214591243387 ) ) ;
#32475=( BOUNDED_SURFACE ( )  B_SPLINE_SURFACE ( 3, 1, ( 
 ( #4440, #7916 ),
 ( #22674, #12311 ),
 ( #22936, #279 ),
 ( #15258, #15011 ),
 ( #27333, #755 ),
 ( #19457, #37675 ),
 ( #15751, #34465 ) ),
 .UNSPECIFIED., .T., .F., .F. ) 
 B_SPLINE_SURFACE_WITH_KNOTS ( ( 4, 3, 4 ),
 ( 2, 2 ),
 ( 0.000000000000000000, 0.5000000000000000000, 1.000000000000000000 ),
 ( 0.000000000000000000, 1.000000000000000000 ),
 .UNSPECIFIED. ) 
 GEOMETRIC_REPRESENTATION_ITEM ( )  RATIONAL_B_SPLINE_SURFACE ( (
 ( 1.000000000000000000, 1.000000000000000000),
 ( 0.3333333333333335369, 0.3333333333333330373),
 ( 0.3333333333333335369, 0.3333333333333330373),
 ( 1.000000000000000000, 1.000000000000000000),
 ( 0.3333333333333333703, 0.3333333333333333703),
 ( 0.3333333333333333703, 0.3333333333333333703),
 ( 1.000000000000000000, 1.000000000000000000) ) ) 
 REPRESENTATION_ITEM ( '' )  SURFACE ( )  );
#32477=CARTESIAN_POINT ( 'NONE',  ( -12.84719963800786502, -9.512789006345032661, 74.31923006385322594 ) ) ;
#32478=CARTESIAN_POINT ( 'NONE',  ( -15.59637485834756809, -7.586876612986846347, 70.81001046420034584 ) ) ;
#32479=CARTESIAN_POINT ( 'NONE',  ( -16.03921789102526674, -7.892880921105984271, 60.40848222778001997 ) ) ;
#32481=CARTESIAN_POINT ( 'NONE',  ( -22.96484330895583881, -19.08706763331013434, 59.18410642315183878 ) ) ;
#32482=ORIENTED_EDGE ( 'NONE', *, *, #24414, .F. ) ;
#32485=PLANE ( 'NONE',  #10831 ) ;
#32487=ORIENTED_EDGE ( 'NONE', *, *, #13467, .T. ) ;
#32492=VERTEX_POINT ( 'NONE', #38578 ) ;
#32493=B_SPLINE_CURVE_WITH_KNOTS ( 'NONE', 3,
 ( #25498, #33103, #31749, #33342, #43065, #47256, #29435, #10718, #14618, #17188 ),
 .UNSPECIFIED., .F., .F.,
 ( 4, 2, 2, 2, 4 ),
 ( 0.000000000000000000, 0.2500000000000000000, 0.5000000000000000000, 0.7500000000000000000, 1.000000000000000000 ),
 .UNSPECIFIED. ) ;
#32494=CARTESIAN_POINT ( 'NONE',  ( -10.47299139157196990, -15.63514485490427575, 61.03789045487297926 ) ) ;
#32495=CARTESIAN_POINT ( 'NONE',  ( -21.00380318978402627, -21.34292366101719196, 62.22975991904223747 ) ) ;
#32496=B_SPLINE_CURVE_WITH_KNOTS ( 'NONE', 3,
 ( #46404, #23998, #39001, #5279, #22233, #9941, #44184, #18027, #3274, #6250 ),
 .UNSPECIFIED., .F., .F.,
 ( 4, 2, 2, 2, 4 ),
 ( 0.000000000000000000, 0.2500000000000000000, 0.5000000000000000000, 0.7500000000000000000, 1.000000000000000000 ),
 .UNSPECIFIED. ) ;
#32497=CARTESIAN_POINT ( 'NONE',  ( -11.96916353976625835, -10.42234295362220919, 67.57184930830715075 ) ) ;
#32502=CARTESIAN_POINT ( 'NONE',  ( -13.09516132467690674, -9.240204434965294311, 64.11766254823847078 ) ) ;
#32504=CARTESIAN_POINT ( 'NONE',  ( -20.75918756122348441, -8.147305293919229641, 63.42626095967343502 ) ) ;
#32506=CARTESIAN_POINT ( 'NONE',  ( -23.25657551529890554, -10.17392617991681192, 63.32831932546986309 ) ) ;
#32508=CARTESIAN_POINT ( 'NONE',  ( -12.40526403761170648, -9.927684372832816351, 60.78747871995254570 ) ) ;
#32509=ORIENTED_EDGE ( 'NONE', *, *, #25336, .F. ) ;
#32510=CARTESIAN_POINT ( 'NONE',  ( -21.94239175829699207, -20.22099772874085488, 59.06442899522711087 ) ) ;
#32514=CARTESIAN_POINT ( 'NONE',  ( -16.58980513972923276, -22.21251475926257513, 65.38597725124276394 ) ) ;
#32515=EDGE_CURVE ( 'NONE', #40340, #43582, #28870, .T. ) ;
#32517=EDGE_CURVE ( 'NONE', #6262, #20123, #27005, .T. ) ;
#32518=ORIENTED_EDGE ( 'NONE', *, *, #18522, .F. ) ;
#32519=CARTESIAN_POINT ( 'NONE',  ( -10.88757861317511200, -12.29993006150962387, 57.51784320375504933 ) ) ;
#32520=CARTESIAN_POINT ( 'NONE',  ( -12.34368963248081918, -19.70250163048094905, 65.16674848656688823 ) ) ;
#32522=B_SPLINE_CURVE_WITH_KNOTS ( 'NONE', 1,
 ( #33064, #14339 ),
 .UNSPECIFIED., .F., .F.,
 ( 2, 2 ),
 ( 0.000000000000000000, 1.000000000000000000 ),
 .UNSPECIFIED. ) ;
#32525=CARTESIAN_POINT ( 'NONE',  ( -23.93648101794248362, -17.51022725521227841, 65.95829288617392194 ) ) ;
#32526=CARTESIAN_POINT ( 'NONE',  ( -10.92750371411227128, -11.16255126880030701, 64.26386748351472988 ) ) ;
#32530=CARTESIAN_POINT ( 'NONE',  ( -19.69275026785852845, -21.90555837663575645, 65.60452853007984686 ) ) ;
#32531=CARTESIAN_POINT ( 'NONE',  ( -23.33239146409005471, -10.27081399407338758, 59.74056881163177479 ) ) ;
#32532=EDGE_LOOP ( 'NONE', ( #41259, #29423 ) ) ;
#32533=CARTESIAN_POINT ( 'NONE',  ( -14.19282086353638661, -8.542981675383003903, 71.01485553001869278 ) ) ;
#32534=ORIENTED_EDGE ( 'NONE', *, *, #18984, .T. ) ;
#32535=CARTESIAN_POINT ( 'NONE',  ( -17.42409385541300892, -14.80920654474439679, 56.49999999999994316 ) ) ;
#32536=FACE_OUTER_BOUND ( 'NONE', #19560, .T. ) ;
#32537=CARTESIAN_POINT ( 'NONE',  ( -17.42847466931223011, -7.755496545676928477, 70.79035813383782738 ) ) ;
#32538=VERTEX_POINT ( 'NONE', #17375 ) ;
#32539=CARTESIAN_POINT ( 'NONE',  ( -24.14668021940793707, -18.02031455489962042, 59.12661512767745364 ) ) ;
#32540=PLANE ( 'NONE',  #35960 ) ;
#32541=EDGE_CURVE ( 'NONE', #9708, #23907, #40236, .T. ) ;
#32542=CARTESIAN_POINT ( 'NONE',  ( -24.85884029783971982, -14.32113974155904046, 66.29637463883811677 ) ) ;
#32544=CARTESIAN_POINT ( 'NONE',  ( -19.21493033759332647, -8.042099214709203636, 59.97595409364182473 ) ) ;
#32546=CARTESIAN_POINT ( 'NONE',  ( -16.92711826723489921, -22.24266155258999333, 72.35881524769365569 ) ) ;
#32547=FACE_OUTER_BOUND ( 'NONE', #6399, .T. ) ;
#32548=CARTESIAN_POINT ( 'NONE',  ( -22.98865756656685022, -9.855479763439479512, 70.12683098403445570 ) ) ;
#32549=B_SPLINE_CURVE_WITH_KNOTS ( 'NONE', 3,
 ( #25688, #2795, #14334, #3033, #43950, #3778, #40243, #33796, #25941, #18535 ),
 .UNSPECIFIED., .F., .F.,
 ( 4, 2, 2, 2, 4 ),
 ( 0.6272669072977127280, 0.7522669073147477681, 0.8772669073317826971, 1.002266907348817737, 1.127266907365852777 ),
 .UNSPECIFIED. ) ;
#32550=CARTESIAN_POINT ( 'NONE',  ( -24.22177711603362482, -13.13842781680106420, 62.83264177645653348 ) ) ;
#32555=ORIENTED_EDGE ( 'NONE', *, *, #32166, .F. ) ;
#32556=CARTESIAN_POINT ( 'NONE',  ( -9.976686065099853451, -14.58608982656816622, 71.51437949254577120 ) ) ;
#32557=CARTESIAN_POINT ( 'NONE',  ( -10.65090206719884591, -13.04127257218233460, 68.03832310965621843 ) ) ;
#32558=CARTESIAN_POINT ( 'NONE',  ( -12.67164228717224361, -20.02160031757407310, 64.86674925084864185 ) ) ;
#32562=CARTESIAN_POINT ( 'NONE',  ( -24.90891992605694227, -15.28604896337863472, 54.27966884056655061 ) ) ;
#32563=FACE_BOUND ( 'NONE', #48233, .T. ) ;
#32564=ADVANCED_FACE ( 'NONE', ( #13663 ), #46707, .F. ) ;
#32565=CARTESIAN_POINT ( 'NONE',  ( -11.01266498513346015, -11.85818215851522339, 67.77431642774575948 ) ) ;
#32566=FACE_OUTER_BOUND ( 'NONE', #20707, .T. ) ;
#32568=CARTESIAN_POINT ( 'NONE',  ( -21.18398602608336745, -21.24092397535611809, 65.69958545398036165 ) ) ;
#32569=VERTEX_POINT ( 'NONE', #32641 ) ;
#32572=PLANE ( 'NONE',  #7794 ) ;
#32574=CARTESIAN_POINT ( 'NONE',  ( -21.12013209665166258, -20.75402305920365720, 69.05450231649803072 ) ) ;
#32575=CARTESIAN_POINT ( 'NONE',  ( -13.82689732469268407, -20.87277619789260186, 68.47097268802275494 ) ) ;
#32576=CARTESIAN_POINT ( 'NONE',  ( -20.60788153932096023, -8.518722016582882972, 63.32593600985608617 ) ) ;
#32577=VERTEX_POINT ( 'NONE', #25021 ) ;
#32578=EDGE_LOOP ( 'NONE', ( #14229, #27408, #11499, #47286, #46499 ) ) ;
#32581=CARTESIAN_POINT ( 'NONE',  ( -13.30711473254145716, -9.147892019113847084, 63.90946529584681457 ) ) ;
#32582=ADVANCED_FACE ( 'NONE', ( #28711 ), #9279, .T. ) ;
#32583=CARTESIAN_POINT ( 'NONE',  ( -23.98474789688958353, -17.25007084823549874, 69.71339792561613535 ) ) ;
#32585=B_SPLINE_CURVE_WITH_KNOTS ( 'NONE', 1,
 ( #34446, #37654 ),
 .UNSPECIFIED., .F., .F.,
 ( 2, 2 ),
 ( 0.000000000000000000, 1.000000000000000000 ),
 .UNSPECIFIED. ) ;
#32586=CARTESIAN_POINT ( 'NONE',  ( -20.70232273485035890, -8.624288160964143302, 60.14125250309182036 ) ) ;
#32587=ORIENTED_EDGE ( 'NONE', *, *, #14353, .F. ) ;
#32588=CARTESIAN_POINT ( 'NONE',  ( -11.34609264327665556, -11.23695660734646573, 60.97885752794695691 ) ) ;
#32589=FACE_OUTER_BOUND ( 'NONE', #25733, .T. ) ;
#32591=( BOUNDED_CURVE ( )  B_SPLINE_CURVE ( 3, ( #5736, #13568, #17016, #9425 ),
 .UNSPECIFIED., .F., .F. ) 
 B_SPLINE_CURVE_WITH_KNOTS ( ( 4, 4 ),
 ( 0.000000000000000000, 0.4074455897393696180 ),
 .UNSPECIFIED. ) 
 CURVE ( )  GEOMETRIC_REPRESENTATION_ITEM ( )  RATIONAL_B_SPLINE_CURVE ( ( 1.000000000000000000, 0.4567392136813241410, 0.3561768502900274358, 0.6983129098261098289 ) ) 
 REPRESENTATION_ITEM ( '' )  );
#32592=CARTESIAN_POINT ( 'NONE',  ( -17.92211955501489484, -22.24259483734421750, 61.98261762376255746 ) ) ;
#32593=EDGE_CURVE ( 'NONE', #33012, #4674, #24061, .T. ) ;
#32595=ADVANCED_FACE ( 'NONE', ( #1880 ), #39311, .F. ) ;
#32596=AXIS2_PLACEMENT_3D ( 'NONE', #14660, #48189, #33389 ) ;
#32597=EDGE_LOOP ( 'NONE', ( #17207, #24999, #43691, #8699, #43172 ) ) ;
#32598=DIRECTION ( 'NONE',  ( 0.9930145540378111368, -0.1179919296777755949, -4.526730170392852178E-08 ) ) ;
#32601=EDGE_CURVE ( 'NONE', #20357, #36713, #36982, .T. ) ;
#32602=CARTESIAN_POINT ( 'NONE',  ( -11.96181431063714484, -19.87549516500596525, 58.11177798925346139 ) ) ;
#32604=CARTESIAN_POINT ( 'NONE',  ( -24.00901317767524290, -17.32824147414624960, 69.42811846502259243 ) ) ;
#32605=B_SPLINE_CURVE_WITH_KNOTS ( 'NONE', 3,
 ( #44484, #41763, #48648, #7307, #18595, #14888, #48401, #30203, #45224, #11466 ),
 .UNSPECIFIED., .F., .F.,
 ( 4, 2, 2, 2, 4 ),
 ( 0.6272669072877415930, 0.7522669073072615342, 0.8772669073267813644, 1.002266907346301306, 1.127266907365821247 ),
 .UNSPECIFIED. ) ;
#32607=CARTESIAN_POINT ( 'NONE',  ( -21.99213670719075253, -20.17946569659695655, 59.04970794435396897 ) ) ;
#32610=CARTESIAN_POINT ( 'NONE',  ( -24.53826898343381302, -12.59737971884151975, 69.81597065678789704 ) ) ;
#32611=( BOUNDED_CURVE ( )  B_SPLINE_CURVE ( 3, ( #40737, #37514, #11431, #45429 ),
 .UNSPECIFIED., .F., .F. ) 
 B_SPLINE_CURVE_WITH_KNOTS ( ( 4, 4 ),
 ( 0.4074455897393594594, 0.5000000000000000000 ),
 .UNSPECIFIED. ) 
 CURVE ( )  GEOMETRIC_REPRESENTATION_ITEM ( )  RATIONAL_B_SPLINE_CURVE ( ( 0.6983129098260824064, 0.7760317562606884323, 0.8765941196519940748, 0.9999999999999990008 ) ) 
 REPRESENTATION_ITEM ( '' )  );
#32612=FACE_OUTER_BOUND ( 'NONE', #21043, .T. ) ;
#32613=CARTESIAN_POINT ( 'NONE',  ( -11.42962537269896117, -10.38539323336976494, 74.62380298385740218 ) ) ;
#32615=FACE_OUTER_BOUND ( 'NONE', #25813, .T. ) ;
#32616=ORIENTED_EDGE ( 'NONE', *, *, #20909, .T. ) ;
#32617=CARTESIAN_POINT ( 'NONE',  ( -24.32646187101298807, -17.61277681157253738, 66.04382984432405124 ) ) ;
#32618=CARTESIAN_POINT ( 'NONE',  ( -20.14428733920338743, -21.74485207141930587, 72.60467522768757931 ) ) ;
#32619=CARTESIAN_POINT ( 'NONE',  ( -10.00693228073093977, -15.50849547184718880, 57.76066962513968406 ) ) ;
#32620=ORIENTED_EDGE ( 'NONE', *, *, #9886, .F. ) ;
#32621=DIRECTION ( 'NONE',  ( -7.484513356303811700E-07, 7.898531944235430371E-07, 0.9999999999994079181 ) ) ;
#32622=ORIENTED_EDGE ( 'NONE', *, *, #33873, .T. ) ;
#32623=ADVANCED_FACE ( 'NONE', ( #28228 ), #39551, .T. ) ;
#32625=ORIENTED_EDGE ( 'NONE', *, *, #19264, .F. ) ;
#32626=B_SPLINE_CURVE_WITH_KNOTS ( 'NONE', 1,
 ( #33950, #2155 ),
 .UNSPECIFIED., .F., .F.,
 ( 2, 2 ),
 ( 0.000000000000000000, 1.000000000000000000 ),
 .UNSPECIFIED. ) ;
#32627=CARTESIAN_POINT ( 'NONE',  ( -10.03125382622086015, -15.73132242054001928, 61.21505925078393773 ) ) ;
#32629=B_SPLINE_CURVE_WITH_KNOTS ( 'NONE', 3,
 ( #29710, #37561, #25768, #33882, #26258, #45000, #38058, #41273, #4345, #15157 ),
 .UNSPECIFIED., .F., .F.,
 ( 4, 2, 2, 2, 4 ),
 ( 0.6272669072877971042, 0.7522669073073185997, 0.8772669073268399842, 1.002266907346361480, 1.127266907365882975 ),
 .UNSPECIFIED. ) ;
#32632=EDGE_LOOP ( 'NONE', ( #9111, #7602, #8393, #6596, #32411 ) ) ;
#32635=EDGE_CURVE ( 'NONE', #43582, #575, #43475, .T. ) ;
#32639=B_SPLINE_CURVE_WITH_KNOTS ( 'NONE', 3,
 ( #36717, #33511, #48310, #14542, #25914, #25197, #26165, #45133, #40929, #3497 ),
 .UNSPECIFIED., .F., .F.,
 ( 4, 2, 2, 2, 4 ),
 ( 0.000000000000000000, 0.2500000000000000000, 0.5000000000000000000, 0.7500000000000000000, 1.000000000000000000 ),
 .UNSPECIFIED. ) ;
#32641=CARTESIAN_POINT ( 'NONE',  ( -10.50893933415051507, -13.43540278197273885, 74.96345540680638919 ) ) ;
#32643=EDGE_LOOP ( 'NONE', ( #36360, #15175, #40230, #30799, #4416 ) ) ;
#32644=CARTESIAN_POINT ( 'NONE',  ( -16.39156059917436181, -21.78318494029796781, 62.05568132351888266 ) ) ;
#32645=EDGE_CURVE ( 'NONE', #6207, #36242, #42240, .T. ) ;
#32646=ORIENTED_EDGE ( 'NONE', *, *, #15687, .T. ) ;
#32647=CARTESIAN_POINT ( 'NONE',  ( -22.46950018977775088, -9.956826463545951356, 73.78161090405299660 ) ) ;
#32648=CARTESIAN_POINT ( 'NONE',  ( -16.20683463515880973, -21.70255690700738782, 58.28585572422844052 ) ) ;
#32649=EDGE_CURVE ( 'NONE', #27092, #46437, #24630, .T. ) ;
#32653=CARTESIAN_POINT ( 'NONE',  ( -12.76547314785493192, -9.517330534081262172, 74.60450883341005124 ) ) ;
#32655=CARTESIAN_POINT ( 'NONE',  ( -10.44104155427339364, -15.80511140325375763, 68.27768108067165542 ) ) ;
#32657=CARTESIAN_POINT ( 'NONE',  ( -24.83340397596770543, -15.58795518843777472, 73.12490970255963418 ) ) ;
#32658=DIRECTION ( 'NONE',  ( -0.5881408891789769999, -0.8087584895849666555, 7.565907428972491290E-08 ) ) ;
#32659=ORIENTED_EDGE ( 'NONE', *, *, #10058, .T. ) ;
#32661=CARTESIAN_POINT ( 'NONE',  ( -13.41658284876181995, -21.09041002232991957, 61.62990919978891924 ) ) ;
#32662=ADVANCED_FACE ( 'NONE', ( #10489 ), #2835, .F. ) ;
#32663=CARTESIAN_POINT ( 'NONE',  ( -24.22652117640109992, -16.69121458274543102, 59.26765574801870429 ) ) ;
#32664=EDGE_LOOP ( 'NONE', ( #19427, #11190, #28856, #20028, #25964 ) ) ;
#32665=CARTESIAN_POINT ( 'NONE',  ( -13.17178389636663027, -8.691783077619437137, 60.59983596220293833 ) ) ;
#32666=CARTESIAN_POINT ( 'NONE',  ( -13.16256456194319391, -9.182988408105495992, 60.59517097614691039 ) ) ;
#32668=ORIENTED_EDGE ( 'NONE', *, *, #31414, .F. ) ;
#32669=CARTESIAN_POINT ( 'NONE',  ( -10.47352315227043640, -13.96536545279488628, 61.10748405753005841 ) ) ;
#32671=CARTESIAN_POINT ( 'NONE',  ( -10.89357934009856521, -11.22367372050276302, 64.19236096111531253 ) ) ;
#32672=CARTESIAN_POINT ( 'NONE',  ( -21.56595869292629075, -8.616614785013410938, 73.70790421061784059 ) ) ;
#32673=EDGE_LOOP ( 'NONE', ( #3574, #24276, #31838, #33255, #7221 ) ) ;
#32674=CARTESIAN_POINT ( 'NONE',  ( -10.18225258457650106, -13.06019941856358102, 71.31554448562532400 ) ) ;
#32675=CARTESIAN_POINT ( 'NONE',  ( -24.66730423131801331, -13.06573828131289616, 62.94768895321241331 ) ) ;
#32676=B_SPLINE_CURVE_WITH_KNOTS ( 'NONE', 3,
 ( #1242, #13280, #35460, #12816, #16248, #27600, #24648, #1746, #28336, #43361 ),
 .UNSPECIFIED., .F., .F.,
 ( 4, 2, 2, 2, 4 ),
 ( 0.000000000000000000, 0.2500000000000000000, 0.5000000000000000000, 0.7500000000000000000, 1.000000000000000000 ),
 .UNSPECIFIED. ) ;
#32677=EDGE_CURVE ( 'NONE', #38392, #9477, #3412, .T. ) ;
#32680=CARTESIAN_POINT ( 'NONE',  ( -15.65722414396544870, -8.035737176819681693, 70.60989791501718571 ) ) ;
#32681=FACE_OUTER_BOUND ( 'NONE', #37570, .T. ) ;
#32683=CARTESIAN_POINT ( 'NONE',  ( -12.62695865377714277, -19.98037072250615154, 71.89833714498439576 ) ) ;
#32685=CARTESIAN_POINT ( 'NONE',  ( -12.30133590797630738, -20.21947593564565793, 68.52312695590214275 ) ) ;
#32686=CARTESIAN_POINT ( 'NONE',  ( -20.50783594841701785, -8.027295835816985914, 66.96599399791791996 ) ) ;
#32690=FACE_OUTER_BOUND ( 'NONE', #39222, .T. ) ;
#32691=CARTESIAN_POINT ( 'NONE',  ( -11.46876066122178095, -18.48806595306161071, 61.57710833523393035 ) ) ;
#32694=VECTOR ( 'NONE', #14987, 1000.000000000000000 ) ;
#32695=VERTEX_POINT ( 'NONE', #26227 ) ;
#32696=CARTESIAN_POINT ( 'NONE',  ( -16.75420032499500422, -21.83093626061109305, 72.25723304517680390 ) ) ;
#32697=CARTESIAN_POINT ( 'NONE',  ( -10.21985783787665802, -12.91125480557629146, 67.84494027641046898 ) ) ;
#32698=LINE ( 'NONE', #13726, #44998 ) ;
#32699=CARTESIAN_POINT ( 'NONE',  ( -10.03860189133040315, -15.79316336790978603, 61.15133701675058120 ) ) ;
#32701=CARTESIAN_POINT ( 'NONE',  ( -13.53325528467554406, -21.16256411608339150, 65.17124155742401115 ) ) ;
#32702=CARTESIAN_POINT ( 'NONE',  ( -16.91855014848012928, -22.24212009645463439, 72.28047803099305213 ) ) ;
#32703=EDGE_CURVE ( 'NONE', #29981, #26502, #11709, .T. ) ;
#32704=CARTESIAN_POINT ( 'NONE',  ( -15.49330550865652079, -21.58970246877112587, 72.34575444675695621 ) ) ;
#32708=ORIENTED_EDGE ( 'NONE', *, *, #35484, .T. ) ;
#32711=EDGE_CURVE ( 'NONE', #13315, #29603, #37045, .T. ) ;
#32712=CARTESIAN_POINT ( 'NONE',  ( -10.23791430846135597, -12.84371669600496801, 67.91645119285166743 ) ) ;
#32713=EDGE_LOOP ( 'NONE', ( #8192, #26967 ) ) ;
#32714=CARTESIAN_POINT ( 'NONE',  ( -13.67008536917650119, -21.24427532949667707, 68.55650896281578355 ) ) ;
#32715=EDGE_CURVE ( 'NONE', #7043, #22471, #28588, .T. ) ;
#32716=EDGE_LOOP ( 'NONE', ( #11877, #40999, #16279, #45915, #23945 ) ) ;
#32721=CARTESIAN_POINT ( 'NONE',  ( -23.52949419687348964, -11.28347464189849703, 70.17738639980606763 ) ) ;
#32722=ORIENTED_EDGE ( 'NONE', *, *, #22426, .T. ) ;
#32723=CARTESIAN_POINT ( 'NONE',  ( -13.46043688762014412, -21.11748779262230258, 65.14775429738139678 ) ) ;
#32724=AXIS2_PLACEMENT_3D ( 'NONE', #35385, #6324, #21106 ) ;
#32725=CARTESIAN_POINT ( 'NONE',  ( -17.53499440593470737, -7.752105970505813737, 70.63468544436783247 ) ) ;
#32727=CARTESIAN_POINT ( 'NONE',  ( -11.36243649338991091, -11.30818272981683137, 60.96420372599168758 ) ) ;
#32728=CARTESIAN_POINT ( 'NONE',  ( -23.23616516995063819, -18.79948553760870666, 65.97389430042666447 ) ) ;
#32730=VERTEX_POINT ( 'NONE', #15127 ) ;
#32732=FACE_OUTER_BOUND ( 'NONE', #20765, .T. ) ;
#32733=CARTESIAN_POINT ( 'NONE',  ( -24.31477923169101629, -16.30090137217950641, 59.40860294853779777 ) ) ;
#32735=CARTESIAN_POINT ( 'NONE',  ( -23.81337036566721466, -17.78917542641211469, 59.30378412513616126 ) ) ;
#32737=CARTESIAN_POINT ( 'NONE',  ( -23.65513889391139557, -11.50482878637529716, 62.83729622335476961 ) ) ;
#32738=CARTESIAN_POINT ( 'NONE',  ( -16.86517901922215756, -21.78691905967089326, 68.98095278456760582 ) ) ;
#32739=CARTESIAN_POINT ( 'NONE',  ( -15.36003256934816719, -8.059790721335600594, 70.76556701434653007 ) ) ;
#32740=( BOUNDED_CURVE ( )  B_SPLINE_CURVE ( 3, ( #28198, #16369, #1352, #20079 ),
 .UNSPECIFIED., .F., .F. ) 
 B_SPLINE_CURVE_WITH_KNOTS ( ( 4, 4 ),
 ( 0.000000000000000000, 0.4074455897393645665 ),
 .UNSPECIFIED. ) 
 CURVE ( )  GEOMETRIC_REPRESENTATION_ITEM ( )  RATIONAL_B_SPLINE_CURVE ( ( 1.000000000000000000, 0.4567392136813283599, 0.3561768502900289901, 0.6983129098261017242 ) ) 
 REPRESENTATION_ITEM ( '' )  );
#32742=ORIENTED_EDGE ( 'NONE', *, *, #7295, .T. ) ;
#32743=CARTESIAN_POINT ( 'NONE',  ( -10.55572857713978685, -13.45776460179270373, 74.69320064931967806 ) ) ;
#32744=CARTESIAN_POINT ( 'NONE',  ( -10.80649751745619724, -11.38720838924848522, 67.71840977816552254 ) ) ;
#32745=VERTEX_POINT ( 'NONE', #18574 ) ;
#32746=( BOUNDED_CURVE ( )  B_SPLINE_CURVE ( 3, ( #41009, #29930, #33589, #37048 ),
 .UNSPECIFIED., .F., .F. ) 
 B_SPLINE_CURVE_WITH_KNOTS ( ( 4, 4 ),
 ( 0.9074455897393652881, 1.000000000000000000 ),
 .UNSPECIFIED. ) 
 CURVE ( )  GEOMETRIC_REPRESENTATION_ITEM ( )  RATIONAL_B_SPLINE_CURVE ( ( 0.6983129098260870693, 0.7760317562606930952, 0.8765941196519974055, 1.000000000000000000 ) ) 
 REPRESENTATION_ITEM ( '' )  );
#32747=B_SPLINE_CURVE_WITH_KNOTS ( 'NONE', 3,
 ( #18896, #48684, #14928, #33909, #15177, #30240, #45259, #11502, #39301, #13173 ),
 .UNSPECIFIED., .F., .F.,
 ( 4, 2, 2, 2, 4 ),
 ( 0.1272669073658319605, 0.2522669073463114642, 0.3772669073267909123, 0.5022669073072704160, 0.6272669072877499197 ),
 .UNSPECIFIED. ) ;
#32749=CARTESIAN_POINT ( 'NONE',  ( -10.83536385990051798, -17.31742045656482176, 64.77739380450887552 ) ) ;
#32750=CARTESIAN_POINT ( 'NONE',  ( -10.00591001363343580, -14.11961505468812206, 61.05674763264026694 ) ) ;
#32752=EDGE_CURVE ( 'NONE', #19668, #33183, #29195, .T. ) ;
#32753=VERTEX_POINT ( 'NONE', #10966 ) ;
#32754=CARTESIAN_POINT ( 'NONE',  ( -24.23612025527544134, -13.19763772753531406, 59.58941156045592180 ) ) ;
#32755=AXIS2_PLACEMENT_3D ( 'NONE', #41363, #44839, #26852 ) ;
#32756=CARTESIAN_POINT ( 'NONE',  ( -23.81448002858924795, -17.66644687436950178, 59.23051795168259304 ) ) ;
#32757=ADVANCED_FACE ( 'NONE', ( #25493 ), #25991, .T. ) ;
#32761=CARTESIAN_POINT ( 'NONE',  ( -17.91839958824308709, -21.79173199888728263, 61.87535923606637311 ) ) ;
#32763=CARTESIAN_POINT ( 'NONE',  ( -15.03744282974918178, -5.447548802137111679, 54.49999999999995026 ) ) ;
#32765=CARTESIAN_POINT ( 'NONE',  ( -17.00410561000564513, -7.771727611841390271, 74.26018273220859101 ) ) ;
#32766=CARTESIAN_POINT ( 'NONE',  ( -22.65953014494242979, -19.53520302830625965, 72.52911954723420251 ) ) ;
#32767=CARTESIAN_POINT ( 'NONE',  ( -23.67763357919828948, -11.55377495691942791, 66.42774300827811373 ) ) ;
#32768=ORIENTED_EDGE ( 'NONE', *, *, #45192, .F. ) ;
#32769=CARTESIAN_POINT ( 'NONE',  ( -22.53429319464570924, -9.952421322533329118, 73.48161091678163359 ) ) ;
#32770=CARTESIAN_POINT ( 'NONE',  ( -10.48201079127635715, -16.05857626038448061, 64.71591366516646815 ) ) ;
#32773=ADVANCED_FACE ( 'NONE', ( #18838 ), #38936, .T. ) ;
#32774=CARTESIAN_POINT ( 'NONE',  ( -10.05737394094114912, -15.92036584257266263, 64.61433266094377359 ) ) ;
#32775=PLANE ( 'NONE',  #29231 ) ;
#32776=CARTESIAN_POINT ( 'NONE',  ( -12.38697808428427827, -19.74705103147751117, 57.92682335111648939 ) ) ;
#32777=ORIENTED_EDGE ( 'NONE', *, *, #28274, .F. ) ;
#32778=CARTESIAN_POINT ( 'NONE',  ( -24.87089661258515960, -14.58528678170222470, 62.87329882295441763 ) ) ;
#32779=DIRECTION ( 'NONE',  ( 0.9466432954593471116, 0.3222832157619555660, 8.771047036255756069E-09 ) ) ;
#32780=CARTESIAN_POINT ( 'NONE',  ( -22.69651743546460665, -20.07290662366753864, 69.31271507414059840 ) ) ;
#32781=CARTESIAN_POINT ( 'NONE',  ( -13.29979614553676370, -21.01354653661592664, 61.77292273241334186 ) ) ;
#32782=EDGE_CURVE ( 'NONE', #5852, #486, #39266, .T. ) ;
#32783=CARTESIAN_POINT ( 'NONE',  ( -18.58465539680892320, -7.906023667314016734, 70.44355971113242276 ) ) ;
#32784=ORIENTED_EDGE ( 'NONE', *, *, #14006, .F. ) ;
#32785=ORIENTED_EDGE ( 'NONE', *, *, #92, .T. ) ;
#32786=CARTESIAN_POINT ( 'NONE',  ( -22.75923595801102550, -10.27751167601812909, 66.54182257657851096 ) ) ;
#32788=EDGE_LOOP ( 'NONE', ( #40316, #16734, #44199, #31681 ) ) ;
#32790=CARTESIAN_POINT ( 'NONE',  ( -14.11063322135152909, -21.03236308526469855, 72.21135587486895702 ) ) ;
#32792=DIRECTION ( 'NONE',  ( -0.6562885720885138774, 0.7545099801500438907, 1.193821363054685294E-08 ) ) ;
#32793=CARTESIAN_POINT ( 'NONE',  ( -12.13424045023392139, -19.48172391048287011, 61.54111352175390692 ) ) ;
#32794=ADVANCED_FACE ( 'NONE', ( #30911 ), #8029, .T. ) ;
#32795=DIRECTION ( 'NONE',  ( 0.8960627639203804229, -0.4439273849576848563, 1.473420430759783058E-16 ) ) ;
#32796=FACE_BOUND ( 'NONE', #6082, .T. ) ;
#32797=DIRECTION ( 'NONE',  ( 0.9710973231077276724, -0.2386838684389877008, 7.431671637556431570E-08 ) ) ;
#32799=DIRECTION ( 'NONE',  ( 0.8244078399817416081, 0.5659962132175737626, 7.627400655798536990E-08 ) ) ;
#32800=VERTEX_POINT ( 'NONE', #46157 ) ;
#32802=CARTESIAN_POINT ( 'NONE',  ( -11.60006209888454443, -10.16330164164447325, 71.08397698276321819 ) ) ;
#32805=CARTESIAN_POINT ( 'NONE',  ( -20.80646516979311755, -21.44732190390276472, 58.78441795439189121 ) ) ;
#32807=CARTESIAN_POINT ( 'NONE',  ( -11.50273385864769438, -11.07591097799543256, 57.50903212538073461 ) ) ;
#32808=VERTEX_POINT ( 'NONE', #11447 ) ;
#32809=ORIENTED_EDGE ( 'NONE', *, *, #22694, .F. ) ;
#32813=CARTESIAN_POINT ( 'NONE',  ( -18.98390459359973548, -7.933620001262258192, 66.91543923465638954 ) ) ;
#32814=EDGE_CURVE ( 'NONE', #26255, #12784, #19294, .T. ) ;
#32816=CARTESIAN_POINT ( 'NONE',  ( -9.973358241295501969, -14.79494948476079941, 74.98434255746357735 ) ) ;
#32817=VERTEX_POINT ( 'NONE', #12419 ) ;
#32818=CARTESIAN_POINT ( 'NONE',  ( -11.03230881600246427, -10.98182333549695322, 60.79390388117851529 ) ) ;
#32821=CARTESIAN_POINT ( 'NONE',  ( -24.41887989065141795, -14.52796127067242971, 66.46676134466591179 ) ) ;
#32823=VERTEX_POINT ( 'NONE', #27199 ) ;
#32824=CARTESIAN_POINT ( 'NONE',  ( -17.79108452803360763, -21.84994637594637368, 58.69081321602850920 ) ) ;
#32825=CARTESIAN_POINT ( 'NONE',  ( -21.42336286209559759, -21.09487474236010485, 69.23945462178221533 ) ) ;
#32826=LINE ( 'NONE', #29886, #16334 ) ;
#32832=CARTESIAN_POINT ( 'NONE',  ( -15.27411149333911133, -8.091140114039422571, 74.07985455727100543 ) ) ;
#32833=EDGE_LOOP ( 'NONE', ( #34034, #19178, #11115, #26775, #37487 ) ) ;
#32835=CARTESIAN_POINT ( 'NONE',  ( -20.04849592361258104, -21.35284569240296548, 72.69006679631317525 ) ) ;
#32836=CARTESIAN_POINT ( 'NONE',  ( -15.55648817577099585, -8.010769314271311003, 74.09457776258329886 ) ) ;
#32837=ADVANCED_FACE ( 'NONE', ( #26962 ), #267, .T. ) ;
#32838=CARTESIAN_POINT ( 'NONE',  ( -11.81042834955647258, -10.54382735031610174, 74.45357240259568243 ) ) ;
#32839=CARTESIAN_POINT ( 'NONE',  ( -20.64396943983181743, -21.02470340508176250, 58.94475165022391394 ) ) ;
#32843=ADVANCED_FACE ( 'NONE', ( #34091 ), #3699, .T. ) ;
#32844=CARTESIAN_POINT ( 'NONE',  ( -18.49053343615340239, -7.435173160506244550, 73.95409006490955051 ) ) ;
#32845=ORIENTED_EDGE ( 'NONE', *, *, #29318, .T. ) ;
#32846=CARTESIAN_POINT ( 'NONE',  ( -10.04710569707986778, -15.85056516143637140, 64.63054717507066016 ) ) ;
#32849=ORIENTED_EDGE ( 'NONE', *, *, #72, .F. ) ;
#32850=CARTESIAN_POINT ( 'NONE',  ( -15.46629645379085893, -8.032742063557217094, 70.81809580567336582 ) ) ;
#32851=CARTESIAN_POINT ( 'NONE',  ( -11.03230825063491594, -10.98182429003440674, 60.79390496990795612 ) ) ;
#32852=DIRECTION ( 'NONE',  ( 0.7437128929774847741, -0.6684991644116392573, 1.736198598216997869E-08 ) ) ;
#32853=EDGE_CURVE ( 'NONE', #13885, #16707, #42403, .T. ) ;
#32860=EDGE_CURVE ( 'NONE', #33937, #47544, #8146, .T. ) ;
#32863=CARTESIAN_POINT ( 'NONE',  ( -10.81484411697162962, -17.11524594140972155, 61.15743118925659161 ) ) ;
#32864=( BOUNDED_CURVE ( )  B_SPLINE_CURVE ( 3, ( #684, #47445, #21349, #6565 ),
 .UNSPECIFIED., .F., .F. ) 
 B_SPLINE_CURVE_WITH_KNOTS ( ( 4, 4 ),
 ( 0.4074455897393661763, 0.5000000000000000000 ),
 .UNSPECIFIED. ) 
 CURVE ( )  GEOMETRIC_REPRESENTATION_ITEM ( )  RATIONAL_B_SPLINE_CURVE ( ( 0.6983129098260940637, 0.7760317562607209618, 0.8765941196520292689, 1.000000000000034639 ) ) 
 REPRESENTATION_ITEM ( '' )  );
#32866=ORIENTED_EDGE ( 'NONE', *, *, #3038, .T. ) ;
#32867=B_SPLINE_CURVE_WITH_KNOTS ( 'NONE', 3,
 ( #16184, #12509, #5134, #20142, #27531, #24331, #28008, #31467, #24087, #5627 ),
 .UNSPECIFIED., .F., .F.,
 ( 4, 2, 2, 2, 4 ),
 ( 0.1272669073658321548, 0.2522669073484877789, 0.3772669073311433197, 0.5022669073137989715, 0.6272669072964545123 ),
 .UNSPECIFIED. ) ;
#32868=DIRECTION ( 'NONE',  ( 0.1847813031241906101, -0.9827796650397888634, 7.910442904995644076E-08 ) ) ;
#32869=CARTESIAN_POINT ( 'NONE',  ( -22.14090652532222236, -20.04928072148792495, 62.51967078134249078 ) ) ;
#32870=ORIENTED_EDGE ( 'NONE', *, *, #18050, .T. ) ;
#32871=FACE_OUTER_BOUND ( 'NONE', #11152, .T. ) ;
#32872=( BOUNDED_CURVE ( )  B_SPLINE_CURVE ( 3, ( #35339, #5312, #9012, #39032 ),
 .UNSPECIFIED., .F., .F. ) 
 B_SPLINE_CURVE_WITH_KNOTS ( ( 4, 4 ),
 ( 0.000000000000000000, 0.4074455897393750581 ),
 .UNSPECIFIED. ) 
 CURVE ( )  GEOMETRIC_REPRESENTATION_ITEM ( )  RATIONAL_B_SPLINE_CURVE ( ( 1.000000000000000000, 0.4567392136813260839, 0.3561768502900281574, 0.6983129098261062762 ) ) 
 REPRESENTATION_ITEM ( '' )  );
#32874=CARTESIAN_POINT ( 'NONE',  ( -14.42683419600288985, -8.428067575814653267, 67.55975083869262221 ) ) ;
#32875=CARTESIAN_POINT ( 'NONE',  ( -19.47326802145739322, -21.50389079897565736, 65.69316087734659959 ) ) ;
#32876=CARTESIAN_POINT ( 'NONE',  ( -16.98991503782990975, -22.24662993548692214, 72.35038528954983406 ) ) ;
#32878=AXIS2_PLACEMENT_3D ( 'NONE', #25695, #17807, #7742 ) ;
#32879=CYLINDRICAL_SURFACE ( 'NONE', #20297, 0.1500000000000015210 ) ;
#32881=CARTESIAN_POINT ( 'NONE',  ( -10.46944733747312917, -15.96661384539355133, 67.99239968927004441 ) ) ;
#32882=ORIENTED_EDGE ( 'NONE', *, *, #2708, .F. ) ;
#32883=CARTESIAN_POINT ( 'NONE',  ( -24.82475127085388422, -15.66597259679895693, 73.11808347143848152 ) ) ;
#32885=VECTOR ( 'NONE', #29962, 1000.000000000000114 ) ;
#32886=VECTOR ( 'NONE', #4572, 1000.000000000000114 ) ;
#32887=ORIENTED_EDGE ( 'NONE', *, *, #20219, .T. ) ;
#32888=CARTESIAN_POINT ( 'NONE',  ( -13.60236376389480384, -20.73382277062339085, 61.80174179654961364 ) ) ;
#32891=CARTESIAN_POINT ( 'NONE',  ( -22.18998830427770841, -20.00468049915955859, 65.71893796558269685 ) ) ;
#32892=CARTESIAN_POINT ( 'NONE',  ( -13.10056816152199843, -9.240526811222729009, 67.67942760033977834 ) ) ;
#32894=CARTESIAN_POINT ( 'NONE',  ( -23.22266324395799231, -18.81915189215696671, 65.82389459980581137 ) ) ;
#32895=VERTEX_POINT ( 'NONE', #5776 ) ;
#32896=CARTESIAN_POINT ( 'NONE',  ( -10.46253582967156426, -14.07554997744959024, 61.21821325757298382 ) ) ;
#32897=VECTOR ( 'NONE', #7052, 1000.000000000000114 ) ;
#32898=CARTESIAN_POINT ( 'NONE',  ( -14.84764829735760827, -8.246537290690364230, 60.33468334944129197 ) ) ;
#32899=CARTESIAN_POINT ( 'NONE',  ( -24.34138250757122535, -16.17068267630804357, 62.89328676667766160 ) ) ;
#32901=FACE_OUTER_BOUND ( 'NONE', #32716, .T. ) ;
#32902=CARTESIAN_POINT ( 'NONE',  ( -24.76666462671617097, -16.07013689822947455, 66.17050792933571302 ) ) ;
#32903=ORIENTED_EDGE ( 'NONE', *, *, #35484, .F. ) ;
#32904=ORIENTED_EDGE ( 'NONE', *, *, #21237, .F. ) ;
#32905=CARTESIAN_POINT ( 'NONE',  ( -15.41198273355754900, -21.57429164360176799, 65.26163917071316689 ) ) ;
#32906=CARTESIAN_POINT ( 'NONE',  ( -13.24203256135214346, -20.97556893053616989, 58.15994682967826179 ) ) ;
#32908=CARTESIAN_POINT ( 'NONE',  ( -23.92719381113450083, -11.17417296164256157, 70.00715453762190066 ) ) ;
#32909=CARTESIAN_POINT ( 'NONE',  ( -23.48344415125163565, -18.41350569598871090, 73.04896097104848707 ) ) ;
#32911=CARTESIAN_POINT ( 'NONE',  ( -22.78151580134219500, -19.98625284378301004, 72.75905219260647527 ) ) ;
#32912=EDGE_CURVE ( 'NONE', #27105, #32937, #47133, .T. ) ;
#32913=EDGE_LOOP ( 'NONE', ( #3691, #18076, #44362, #16618, #42849 ) ) ;
#32914=VERTEX_POINT ( 'NONE', #39498 ) ;
#32917=EDGE_CURVE ( 'NONE', #45841, #29545, #36025, .T. ) ;
#32919=CARTESIAN_POINT ( 'NONE',  ( -19.95257394585953747, -8.281687416969214510, 74.02096610897844187 ) ) ;
#32920=CARTESIAN_POINT ( 'NONE',  ( -14.81535805098777736, -7.777528402031244958, 77.49999999999994316 ) ) ;
#32921=CARTESIAN_POINT ( 'NONE',  ( -19.03296962921835345, -7.534949906353642923, 67.00797648986954869 ) ) ;
#32922=CARTESIAN_POINT ( 'NONE',  ( -18.58265938564740338, -7.449833053036199360, 73.94040763329604715 ) ) ;
#32923=ORIENTED_EDGE ( 'NONE', *, *, #15090, .F. ) ;
#32925=AXIS2_PLACEMENT_3D ( 'NONE', #14787, #10888, #29604 ) ;
#32927=ORIENTED_EDGE ( 'NONE', *, *, #39826, .T. ) ;
#32928=CARTESIAN_POINT ( 'NONE',  ( -14.60479746972646886, -7.913168098764732150, 60.50491608655884335 ) ) ;
#32929=CARTESIAN_POINT ( 'NONE',  ( -10.03016471889695183, -15.72215649304404117, 61.08143109537672188 ) ) ;
#32930=AXIS2_PLACEMENT_3D ( 'NONE', #30328, #37683, #45339 ) ;
#32931=VERTEX_POINT ( 'NONE', #43200 ) ;
#32932=CARTESIAN_POINT ( 'NONE',  ( -17.85555652284939043, -7.772123375420258107, 60.09532845646905486 ) ) ;
#32933=ADVANCED_FACE ( 'NONE', ( #5534 ), #9471, .T. ) ;
#32935=ORIENTED_EDGE ( 'NONE', *, *, #13, .T. ) ;
#32937=VERTEX_POINT ( 'NONE', #24961 ) ;
#32938=CARTESIAN_POINT ( 'NONE',  ( -23.86582823559828626, -17.67428107336104404, 62.47920748027621585 ) ) ;
#32939=CARTESIAN_POINT ( 'NONE',  ( -12.25438268106910833, -10.01050553627876383, 57.29755567529926452 ) ) ;
#32940=ORIENTED_EDGE ( 'NONE', *, *, #40091, .T. ) ;
#32943=EDGE_CURVE ( 'NONE', #773, #39013, #19916, .T. ) ;
#32944=EDGE_LOOP ( 'NONE', ( #29422, #14423, #26862, #44495, #31642 ) ) ;
#32945=CARTESIAN_POINT ( 'NONE',  ( -12.45873566688477929, -9.804017486950373339, 57.10407583662104258 ) ) ;
#32946=( BOUNDED_SURFACE ( )  B_SPLINE_SURFACE ( 3, 1, ( 
 ( #41106, #42084 ),
 ( #3934, #45069 ),
 ( #34685, #15959 ),
 ( #7636, #27059 ),
 ( #4404, #18681 ),
 ( #8352, #8122 ),
 ( #248, #11316 ) ),
 .UNSPECIFIED., .T., .F., .F. ) 
 B_SPLINE_SURFACE_WITH_KNOTS ( ( 4, 3, 4 ),
 ( 2, 2 ),
 ( 0.000000000000000000, 0.5000000000000000000, 1.000000000000000000 ),
 ( 0.000000000000000000, 1.000000000000000000 ),
 .UNSPECIFIED. ) 
 GEOMETRIC_REPRESENTATION_ITEM ( )  RATIONAL_B_SPLINE_SURFACE ( (
 ( 1.000000000000000000, 1.000000000000000000),
 ( 0.3333333333333335369, 0.3333333333333330373),
 ( 0.3333333333333335369, 0.3333333333333330373),
 ( 1.000000000000000000, 1.000000000000000000),
 ( 0.3333333333333333703, 0.3333333333333333703),
 ( 0.3333333333333333703, 0.3333333333333333703),
 ( 1.000000000000000000, 1.000000000000000000) ) ) 
 REPRESENTATION_ITEM ( '' )  SURFACE ( )  );
#32950=CARTESIAN_POINT ( 'NONE',  ( -19.91241090325594243, -21.83142246198826797, 69.12820776009694157 ) ) ;
#32953=CARTESIAN_POINT ( 'NONE',  ( -11.33353553667378044, -11.35870856699622955, 60.75173739346320190 ) ) ;
#32954=DIRECTION ( 'NONE',  ( 0.6043825497304157190, -0.7966942535134532433, 5.656674838975381179E-08 ) ) ;
#32955=ORIENTED_EDGE ( 'NONE', *, *, #9747, .F. ) ;
#32957=CARTESIAN_POINT ( 'NONE',  ( -6.792537093481112898, -14.13189257747792738, 54.60745305979834541 ) ) ;
#32958=CARTESIAN_POINT ( 'NONE',  ( -11.90533692723668224, -10.50281135863178150, 71.26893075534566435 ) ) ;
#32965=CARTESIAN_POINT ( 'NONE',  ( -16.49760773099677991, -22.20149646633050367, 65.40377166897843608 ) ) ;
#32966=VERTEX_POINT ( 'NONE', #31865 ) ;
#32967=CYLINDRICAL_SURFACE ( 'NONE', #14690, 0.1500000000000066835 ) ;
#32971=CARTESIAN_POINT ( 'NONE',  ( -16.50454536406711981, -22.20232556258728351, 65.34068991928313608 ) ) ;
#32972=VERTEX_POINT ( 'NONE', #40229 ) ;
#32973=ADVANCED_FACE ( 'NONE', ( #18030 ), #10324, .T. ) ;
#32977=CARTESIAN_POINT ( 'NONE',  ( -19.83053741356648558, -21.43962678742999728, 65.67306095859845527 ) ) ;
#32978=EDGE_CURVE ( 'NONE', #39540, #7278, #8761, .T. ) ;
#32980=CARTESIAN_POINT ( 'NONE',  ( -23.30384418855528139, -19.38433790851559735, 58.99136497286766456 ) ) ;
#32981=DIRECTION ( 'NONE',  ( -0.7841839494287597967, 0.6205284308219183309, 3.872224938349061382E-17 ) ) ;
#32983=CARTESIAN_POINT ( 'NONE',  ( -10.43949455435184603, -13.84896052950683476, 57.46297163929641982 ) ) ;
#32985=ORIENTED_EDGE ( 'NONE', *, *, #25774, .T. ) ;
#32986=CARTESIAN_POINT ( 'NONE',  ( -21.93816111929147539, -20.22843456855405364, 62.64927864921646261 ) ) ;
#32987=AXIS2_PLACEMENT_3D ( 'NONE', #44303, #32247, #39622 ) ;
#32988=CARTESIAN_POINT ( 'NONE',  ( -24.46435014771442695, -14.30944682264569856, 62.86863794226144364 ) ) ;
#32989=( BOUNDED_CURVE ( )  B_SPLINE_CURVE ( 3, ( #40502, #33334, #36546, #25980 ),
 .UNSPECIFIED., .F., .F. ) 
 B_SPLINE_CURVE_WITH_KNOTS ( ( 4, 4 ),
 ( 0.5000000000000000000, 0.9074455897393675086 ),
 .UNSPECIFIED. ) 
 CURVE ( )  GEOMETRIC_REPRESENTATION_ITEM ( )  RATIONAL_B_SPLINE_CURVE ( ( 1.000000000000003775, 0.4567392136813254178, 0.3561768502900251598, 0.6983129098261069423 ) ) 
 REPRESENTATION_ITEM ( '' )  );
#32990=CARTESIAN_POINT ( 'NONE',  ( -23.29918407416772297, -19.39037376486758646, 58.99915347576865088 ) ) ;
#32992=CARTESIAN_POINT ( 'NONE',  ( -24.14084261439634460, -12.83653908289654488, 70.05626466142305731 ) ) ;
#32993=ORIENTED_EDGE ( 'NONE', *, *, #47773, .F. ) ;
#32995=CARTESIAN_POINT ( 'NONE',  ( -24.38874385864151506, -14.10660391674899827, 69.76161322672021470 ) ) ;
#32996=VERTEX_POINT ( 'NONE', #32586 ) ;
#32997=PLANE ( 'NONE',  #39600 ) ;
#32999=CARTESIAN_POINT ( 'NONE',  ( -24.28579947082789303, -13.18942387424446316, 62.84736316175410309 ) ) ;
#33000=CARTESIAN_POINT ( 'NONE',  ( -14.38541658028441184, -8.447521680442473979, 67.55415319938168750 ) ) ;
#33004=VERTEX_POINT ( 'NONE', #25447 ) ;
#33005=( BOUNDED_SURFACE ( )  B_SPLINE_SURFACE ( 3, 1, ( 
 ( #38673, #5193 ),
 ( #45836, #43094 ),
 ( #35212, #31532 ),
 ( #46567, #24148 ),
 ( #12807, #35455 ),
 ( #8398, #16242 ),
 ( #34969, #38418 ) ),
 .UNSPECIFIED., .T., .F., .F. ) 
 B_SPLINE_SURFACE_WITH_KNOTS ( ( 4, 3, 4 ),
 ( 2, 2 ),
 ( 0.000000000000000000, 0.5000000000000000000, 1.000000000000000000 ),
 ( 0.000000000000000000, 1.000000000000000000 ),
 .UNSPECIFIED. ) 
 GEOMETRIC_REPRESENTATION_ITEM ( )  RATIONAL_B_SPLINE_SURFACE ( (
 ( 1.000000000000000000, 1.000000000000000000),
 ( 0.3333333333333335369, 0.3333333333333330373),
 ( 0.3333333333333335369, 0.3333333333333330373),
 ( 1.000000000000000000, 1.000000000000000000),
 ( 0.3333333333333333703, 0.3333333333333333703),
 ( 0.3333333333333333703, 0.3333333333333333703),
 ( 1.000000000000000000, 1.000000000000000000) ) ) 
 REPRESENTATION_ITEM ( '' )  SURFACE ( )  );
#33006=CARTESIAN_POINT ( 'NONE',  ( -11.93522140360746242, -14.45952210441258678, 54.07175714974879099 ) ) ;
#33007=CYLINDRICAL_SURFACE ( 'NONE', #2223, 0.1500000000000000777 ) ;
#33008=CARTESIAN_POINT ( 'NONE',  ( -22.69667682133237463, -20.07274909735609825, 69.33451383057273176 ) ) ;
#33009=CARTESIAN_POINT ( 'NONE',  ( -19.54271803596333257, -21.95161028251255786, 62.14503642488964630 ) ) ;
#33010=PLANE ( 'NONE',  #11718 ) ;
#33011=CARTESIAN_POINT ( 'NONE',  ( -24.27720235214249200, -16.23785455720555859, 62.60945374813341147 ) ) ;
#33012=VERTEX_POINT ( 'NONE', #44412 ) ;
#33013=ORIENTED_EDGE ( 'NONE', *, *, #16484, .F. ) ;
#33015=CARTESIAN_POINT ( 'NONE',  ( -11.16720021946830244, -11.56054808309503734, 67.91864607954204303 ) ) ;
#33017=ORIENTED_EDGE ( 'NONE', *, *, #43997, .T. ) ;
#33018=CARTESIAN_POINT ( 'NONE',  ( -23.75243126011088890, -11.69520888738364306, 66.83703234806088744 ) ) ;
#33020=CARTESIAN_POINT ( 'NONE',  ( -11.34825610409693475, -18.28566130560761849, 57.80714629623370371 ) ) ;
#33022=FACE_OUTER_BOUND ( 'NONE', #26553, .T. ) ;
#33023=CARTESIAN_POINT ( 'NONE',  ( -21.73633048181673999, -9.221757950931626979, 59.87738363463013513 ) ) ;
#33024=EDGE_CURVE ( 'NONE', #46985, #9191, #11158, .T. ) ;
#33025=CARTESIAN_POINT ( 'NONE',  ( -22.18998830427770841, -20.00468049915955859, 65.71893796558269685 ) ) ;
#33026=CARTESIAN_POINT ( 'NONE',  ( -16.88181972730358638, -20.29590995520119989, 53.69233794759168887 ) ) ;
#33027=CYLINDRICAL_SURFACE ( 'NONE', #16127, 0.1499999999999994116 ) ;
#33028=( BOUNDED_SURFACE ( )  B_SPLINE_SURFACE ( 3, 1, ( 
 ( #8202, #38459 ),
 ( #34522, #41684 ),
 ( #23219, #27382 ),
 ( #22986, #31081 ),
 ( #20236, #11891 ),
 ( #37973, #34272 ),
 ( #35004, #26666 ) ),
 .UNSPECIFIED., .T., .F., .F. ) 
 B_SPLINE_SURFACE_WITH_KNOTS ( ( 4, 3, 4 ),
 ( 2, 2 ),
 ( 0.000000000000000000, 0.5000000000000000000, 1.000000000000000000 ),
 ( 0.000000000000000000, 1.000000000000000000 ),
 .UNSPECIFIED. ) 
 GEOMETRIC_REPRESENTATION_ITEM ( )  RATIONAL_B_SPLINE_SURFACE ( (
 ( 1.000000000000000000, 1.000000000000000000),
 ( 0.3333333333333335369, 0.3333333333333330373),
 ( 0.3333333333333335369, 0.3333333333333330373),
 ( 1.000000000000000000, 1.000000000000000000),
 ( 0.3333333333333333703, 0.3333333333333333703),
 ( 0.3333333333333333703, 0.3333333333333333703),
 ( 1.000000000000000000, 1.000000000000000000) ) ) 
 REPRESENTATION_ITEM ( '' )  SURFACE ( )  );
#33029=CARTESIAN_POINT ( 'NONE',  ( -16.42041309862903375, -21.79104485276047853, 58.49405286284293481 ) ) ;
#33030=EDGE_CURVE ( 'NONE', #46821, #12740, #2783, .T. ) ;
#33033=CARTESIAN_POINT ( 'NONE',  ( -11.59474043620840966, -10.17003886705225568, 71.16231417095823986 ) ) ;
#33034=CARTESIAN_POINT ( 'NONE',  ( -14.69705846215979328, -19.60099676430529314, 53.69233794759168177 ) ) ;
#33035=CARTESIAN_POINT ( 'NONE',  ( -17.89121901661899727, -21.84743352196291255, 65.64532279319318775 ) ) ;
#33037=DIRECTION ( 'NONE',  ( -0.3478314405900309048, -0.9375570856950864451, 0.000000000000000000 ) ) ;
#33038=CARTESIAN_POINT ( 'NONE',  ( -22.16371339239454130, -9.585275839764586081, 59.81351278129218230 ) ) ;
#33043=EDGE_LOOP ( 'NONE', ( #9356, #3660 ) ) ;
#33045=EDGE_CURVE ( 'NONE', #33991, #24829, #29620, .T. ) ;
#33047=ADVANCED_FACE ( 'NONE', ( #43938 ), #25134, .T. ) ;
#33049=CARTESIAN_POINT ( 'NONE',  ( -9.975093131592752016, -14.93635113986534257, 74.98274190467411415 ) ) ;
#33051=CARTESIAN_POINT ( 'NONE',  ( -23.13450524283604182, -10.02421013782724657, 66.70328774705285468 ) ) ;
#33052=CARTESIAN_POINT ( 'NONE',  ( -11.64902330566212463, -10.02396254413167576, 53.49999999999994316 ) ) ;
#33053=ORIENTED_EDGE ( 'NONE', *, *, #36737, .F. ) ;
#33054=FACE_OUTER_BOUND ( 'NONE', #6257, .T. ) ;
#33056=CARTESIAN_POINT ( 'NONE',  ( -12.36794914932409561, -19.72224030764921565, 61.39678633597973345 ) ) ;
#33058=CARTESIAN_POINT ( 'NONE',  ( -10.88286923018596575, -17.43962093083235843, 68.11193994895104709 ) ) ;
#33060=CARTESIAN_POINT ( 'NONE',  ( -23.34092642400682038, -10.28208056094584677, 59.78698708435513254 ) ) ;
#33063=CARTESIAN_POINT ( 'NONE',  ( -24.36966136476852540, -17.50601128794927774, 69.59995046513768102 ) ) ;
#33064=CARTESIAN_POINT ( 'NONE',  ( -19.17604249790256077, -21.63836284480991878, 58.53979515915469278 ) ) ;
#33065=CARTESIAN_POINT ( 'NONE',  ( -11.03557423443333008, -17.80950410671109196, 68.25289248663547426 ) ) ;
#33067=LINE ( 'NONE', #18055, #6968 ) ;
#33068=DIRECTION ( 'NONE',  ( -5.888300610989836252E-06, -9.662809626516592716E-06, 0.9999999999359789893 ) ) ;
#33069=CYLINDRICAL_SURFACE ( 'NONE', #27048, 0.1500000000000002165 ) ;
#33071=CARTESIAN_POINT ( 'NONE',  ( -23.30963478160716562, -18.69084381296369557, 69.30844128244088154 ) ) ;
#33072=DIRECTION ( 'NONE',  ( 2.083496782661112619E-06, -1.347747140477569176E-07, -0.9999999999978204102 ) ) ;
#33073=ORIENTED_EDGE ( 'NONE', *, *, #23059, .T. ) ;
#33074=CARTESIAN_POINT ( 'NONE',  ( -10.37497031247464463, -14.69804315800203298, 71.62782692816419683 ) ) ;
#33075=CARTESIAN_POINT ( 'NONE',  ( -24.18470913683765389, -12.80901137141652768, 69.78715111652664405 ) ) ;
#33076=CARTESIAN_POINT ( 'NONE',  ( -18.63018860987378389, -7.457396320151260305, 73.95569119842126327 ) ) ;
#33077=EDGE_CURVE ( 'NONE', #35817, #20111, #27143, .T. ) ;
#33078=ORIENTED_EDGE ( 'NONE', *, *, #11707, .T. ) ;
#33079=CARTESIAN_POINT ( 'NONE',  ( -10.05191582289251961, -15.88326310211563275, 64.70782794937979077 ) ) ;
#33083=AXIS2_PLACEMENT_3D ( 'NONE', #40841, #7126, #37125 ) ;
#33084=CARTESIAN_POINT ( 'NONE',  ( -18.84335783304844369, -7.495515834006305056, 70.49351169566308783 ) ) ;
#33085=CYLINDRICAL_SURFACE ( 'NONE', #9449, 0.1500000000000041578 ) ;
#33086=CYLINDRICAL_SURFACE ( 'NONE', #29931, 0.1500000000000050460 ) ;
#33091=EDGE_CURVE ( 'NONE', #27869, #31116, #23217, .T. ) ;
#33094=CARTESIAN_POINT ( 'NONE',  ( -23.44980453451080393, -18.46889374286061525, 73.06368236440982855 ) ) ;
#33096=B_SPLINE_CURVE_WITH_KNOTS ( 'NONE', 3,
 ( #37878, #8339, #33674, #38114, #42068, #48718, #26313, #19170, #18926, #3657 ),
 .UNSPECIFIED., .F., .F.,
 ( 4, 2, 2, 2, 4 ),
 ( 0.1272669073658372341, 0.2522669073463233991, 0.3772669073268095641, 0.5022669073072957291, 0.6272669072877818941 ),
 .UNSPECIFIED. ) ;
#33098=ORIENTED_EDGE ( 'NONE', *, *, #32601, .T. ) ;
#33099=EDGE_CURVE ( 'NONE', #12632, #38388, #37176, .T. ) ;
#33100=CARTESIAN_POINT ( 'NONE',  ( -10.33531725737393181, -17.10115422170377641, 57.87255955594724810 ) ) ;
#33102=CARTESIAN_POINT ( 'NONE',  ( -18.77776586261893144, -7.941280436638581186, 66.97359733704600160 ) ) ;
#33103=CARTESIAN_POINT ( 'NONE',  ( -24.40527839663079845, -14.29480931175867120, 69.65275285367388847 ) ) ;
#33104=ADVANCED_FACE ( 'NONE', ( #11632 ), #23856, .T. ) ;
#33105=VERTEX_POINT ( 'NONE', #33785 ) ;
#33106=CARTESIAN_POINT ( 'NONE',  ( -11.22967102384216886, -11.54873604311523039, 67.91864634137124312 ) ) ;
#33107=EDGE_CURVE ( 'NONE', #46816, #35760, #11097, .T. ) ;
#33110=B_SPLINE_CURVE_WITH_KNOTS ( 'NONE', 3,
 ( #20050, #38757, #8739, #35056 ),
 .UNSPECIFIED., .F., .F.,
 ( 4, 4 ),
 ( 0.000000000000000000, 0.2909959651135547443 ),
 .UNSPECIFIED. ) ;
#33112=CARTESIAN_POINT ( 'NONE',  ( -10.13258936719380898, -16.33817337277914561, 71.63245765104117879 ) ) ;
#33115=B_SPLINE_CURVE_WITH_KNOTS ( 'NONE', 3,
 ( #39790, #44718, #34095, #14872, #26475, #15366, #11701, #384, #18844, #7293 ),
 .UNSPECIFIED., .F., .F.,
 ( 4, 2, 2, 2, 4 ),
 ( 0.000000000000000000, 0.2500000000000000000, 0.5000000000000000000, 0.7500000000000000000, 1.000000000000000000 ),
 .UNSPECIFIED. ) ;
#33118=CARTESIAN_POINT ( 'NONE',  ( -10.33431758219403207, -12.52035302217920254, 60.98348881056122650 ) ) ;
#33119=CARTESIAN_POINT ( 'NONE',  ( -22.81416393091693706, -19.95214112651346383, 72.84389334246579040 ) ) ;
#33121=CARTESIAN_POINT ( 'NONE',  ( -14.79922817013080483, -7.836842635312091687, 57.03495431467663224 ) ) ;
#33122=DIRECTION ( 'NONE',  ( 0.9774082387306984865, -0.2113602016968848807, 7.903122840289808494E-08 ) ) ;
#33124=DIRECTION ( 'NONE',  ( 5.854827030937197869E-31, 1.020425574103664912E-16, 1.000000000000000000 ) ) ;
#33125=CARTESIAN_POINT ( 'NONE',  ( -14.60689764421331738, -8.346551857622415582, 63.78978840692987262 ) ) ;
#33126=CARTESIAN_POINT ( 'NONE',  ( -12.64016520574754843, -19.91947694667972968, 64.93963025601375705 ) ) ;
#33127=ORIENTED_EDGE ( 'NONE', *, *, #26864, .T. ) ;
#33128=FACE_BOUND ( 'NONE', #9759, .T. ) ;
#33129=EDGE_LOOP ( 'NONE', ( #34036, #10625 ) ) ;
#33131=LINE ( 'NONE', #48169, #30261 ) ;
#33132=CARTESIAN_POINT ( 'NONE',  ( -21.18398602608336745, -21.24092397535611809, 65.69958545398036165 ) ) ;
#33133=ORIENTED_EDGE ( 'NONE', *, *, #9149, .T. ) ;
#33135=ORIENTED_EDGE ( 'NONE', *, *, #4493, .T. ) ;
#33137=ADVANCED_FACE ( 'NONE', ( #19506 ), #36738, .T. ) ;
#33138=CARTESIAN_POINT ( 'NONE',  ( -23.32532355526320345, -18.57446955825106016, 69.59371930732142175 ) ) ;
#33139=B_SPLINE_CURVE_WITH_KNOTS ( 'NONE', 1,
 ( #9004, #46904 ),
 .UNSPECIFIED., .F., .F.,
 ( 2, 2 ),
 ( 0.000000000000000000, 1.000000000000000000 ),
 .UNSPECIFIED. ) ;
#33140=VERTEX_POINT ( 'NONE', #41253 ) ;
#33141=CARTESIAN_POINT ( 'NONE',  ( -23.83043763270304183, -11.86620476845630101, 59.48235732590898550 ) ) ;
#33142=CARTESIAN_POINT ( 'NONE',  ( -24.63355139826557760, -12.92841318297298692, 62.94608782021682458 ) ) ;
#33143=B_SPLINE_CURVE_WITH_KNOTS ( 'NONE', 3,
 ( #32648, #47196, #21342, #44004, #16888, #31928, #40289, #36090, #2128, #13187 ),
 .UNSPECIFIED., .F., .F.,
 ( 4, 2, 2, 2, 4 ),
 ( 0.000000000000000000, 0.2500000000000000000, 0.5000000000000000000, 0.7500000000000000000, 1.000000000000000000 ),
 .UNSPECIFIED. ) ;
#33146=VERTEX_POINT ( 'NONE', #18850 ) ;
#33148=DIRECTION ( 'NONE',  ( -8.766499794606700203E-07, -3.805972782304116817E-07, 0.9999999999995433653 ) ) ;
#33149=CARTESIAN_POINT ( 'NONE',  ( -10.60168018607446960, -13.23530295033109638, 74.86744747271762890 ) ) ;
#33150=( BOUNDED_CURVE ( )  B_SPLINE_CURVE ( 3, ( #43659, #17031, #24211, #32079 ),
 .UNSPECIFIED., .F., .F. ) 
 B_SPLINE_CURVE_WITH_KNOTS ( ( 4, 4 ),
 ( 0.5000000000000000000, 0.9074455897393600701 ),
 .UNSPECIFIED. ) 
 CURVE ( )  GEOMETRIC_REPRESENTATION_ITEM ( )  RATIONAL_B_SPLINE_CURVE ( ( 1.000000000000019762, 0.4567392136813480108, 0.3561768502900223288, 0.6983129098260643097 ) ) 
 REPRESENTATION_ITEM ( '' )  );
#33151=CARTESIAN_POINT ( 'NONE',  ( -21.24554616535955631, -21.20453920045676810, 65.76949338751086316 ) ) ;
#33152=PLANE ( 'NONE',  #32596 ) ;
#33153=EDGE_CURVE ( 'NONE', #35243, #30729, #38125, .T. ) ;
#33154=CARTESIAN_POINT ( 'NONE',  ( -20.44433886619616914, -7.998055119120133227, 66.89448804686142580 ) ) ;
#33155=VERTEX_POINT ( 'NONE', #26001 ) ;
#33156=VERTEX_POINT ( 'NONE', #10727 ) ;
#33159=CARTESIAN_POINT ( 'NONE',  ( -21.06635048418738165, -21.30826373965517817, 62.29966805574095901 ) ) ;
#33160=CARTESIAN_POINT ( 'NONE',  ( -18.95673185541715711, -7.518389839197517688, 67.03925230700772886 ) ) ;
#33161=FACE_OUTER_BOUND ( 'NONE', #7201, .T. ) ;
#33162=VERTEX_POINT ( 'NONE', #3340 ) ;
#33164=( BOUNDED_SURFACE ( )  B_SPLINE_SURFACE ( 3, 1, ( 
 ( #23851, #20637 ),
 ( #35632, #1908 ),
 ( #13212, #44266 ),
 ( #14408, #36583 ),
 ( #37080, #7071 ),
 ( #40312, #3115 ),
 ( #6581, #48416 ) ),
 .UNSPECIFIED., .T., .F., .F. ) 
 B_SPLINE_SURFACE_WITH_KNOTS ( ( 4, 3, 4 ),
 ( 2, 2 ),
 ( 0.000000000000000000, 0.5000000000000000000, 1.000000000000000000 ),
 ( 0.000000000000000000, 1.000000000000000000 ),
 .UNSPECIFIED. ) 
 GEOMETRIC_REPRESENTATION_ITEM ( )  RATIONAL_B_SPLINE_SURFACE ( (
 ( 1.000000000000000000, 1.000000000000000000),
 ( 0.3333333333333335369, 0.3333333333333330373),
 ( 0.3333333333333335369, 0.3333333333333330373),
 ( 1.000000000000000000, 1.000000000000000000),
 ( 0.3333333333333333703, 0.3333333333333333703),
 ( 0.3333333333333333703, 0.3333333333333333703),
 ( 1.000000000000000000, 1.000000000000000000) ) ) 
 REPRESENTATION_ITEM ( '' )  SURFACE ( )  );
#33165=VERTEX_POINT ( 'NONE', #25745 ) ;
#33167=DIRECTION ( 'NONE',  ( 0.7029450532227031756, 0.7112441579020042370, -7.405715380709557223E-09 ) ) ;
#33169=EDGE_CURVE ( 'NONE', #25610, #42180, #37539, .T. ) ;
#33170=CARTESIAN_POINT ( 'NONE',  ( -10.76542914127749739, -16.97361976459616173, 61.34670158936435769 ) ) ;
#33171=CARTESIAN_POINT ( 'NONE',  ( -10.49189908542464700, -16.09426454567519116, 68.26295692486267797 ) ) ;
#33172=EDGE_CURVE ( 'NONE', #21219, #38940, #3402, .T. ) ;
#33174=DIRECTION ( 'NONE',  ( -0.7489133456531320565, -0.6626679415081376812, 6.686399169904807862E-09 ) ) ;
#33178=EDGE_CURVE ( 'NONE', #35366, #33155, #6998, .T. ) ;
#33179=CARTESIAN_POINT ( 'NONE',  ( -20.19231670334047735, -8.325423520194950910, 70.40100341277891971 ) ) ;
#33181=CARTESIAN_POINT ( 'NONE',  ( -20.91839533430741227, -20.87517621519315369, 65.86837424650867945 ) ) ;
#33182=EDGE_CURVE ( 'NONE', #28748, #10266, #35770, .T. ) ;
#33183=VERTEX_POINT ( 'NONE', #25275 ) ;
#33184=CARTESIAN_POINT ( 'NONE',  ( -11.81042834955647258, -10.54382735031610174, 74.45357240259568243 ) ) ;
#33185=CARTESIAN_POINT ( 'NONE',  ( -17.63008012001554192, -7.362005203207129256, 63.74395322827410126 ) ) ;
#33186=EDGE_LOOP ( 'NONE', ( #23797, #20946, #14674, #386, #28860 ) ) ;
#33187=EDGE_CURVE ( 'NONE', #10912, #15909, #30182, .T. ) ;
#33188=EDGE_CURVE ( 'NONE', #8644, #45412, #4651, .T. ) ;
#33189=CARTESIAN_POINT ( 'NONE',  ( -18.46282016565315587, -21.73182091564523688, 72.28510983673571388 ) ) ;
#33190=CARTESIAN_POINT ( 'NONE',  ( -10.38078067960954698, -14.50222210708341919, 68.15800126083216526 ) ) ;
#33191=ORIENTED_EDGE ( 'NONE', *, *, #5733, .T. ) ;
#33193=CARTESIAN_POINT ( 'NONE',  ( -19.42045769886998841, -21.57377358197381412, 65.87974951360257592 ) ) ;
#33194=DIRECTION ( 'NONE',  ( -0.9501515917649785425, -0.3117883138709295898, 1.594035198720926202E-08 ) ) ;
#33195=ORIENTED_EDGE ( 'NONE', *, *, #34504, .F. ) ;
#33196=CARTESIAN_POINT ( 'NONE',  ( -12.00582977146459562, -10.37713343423881796, 67.78431519901778302 ) ) ;
#33198=ORIENTED_EDGE ( 'NONE', *, *, #15111, .F. ) ;
#33200=CARTESIAN_POINT ( 'NONE',  ( -12.78872866433637867, -9.492418930890588413, 70.84925165228416688 ) ) ;
#33201=DIRECTION ( 'NONE',  ( -1.027096117176089930E-05, -2.598167872330529078E-06, -0.9999999999438783371 ) ) ;
#33203=CARTESIAN_POINT ( 'NONE',  ( -23.16908677366360436, -10.06487111558154801, 63.18530634343710517 ) ) ;
#33204=CARTESIAN_POINT ( 'NONE',  ( -16.82992792493983458, -21.78406743069276885, 68.99560622300008106 ) ) ;
#33205=CARTESIAN_POINT ( 'NONE',  ( -12.36731040760125744, -9.968228163758537264, 60.57534674602654690 ) ) ;
#33206=CYLINDRICAL_SURFACE ( 'NONE', #30037, 0.1499999999999964972 ) ;
#33208=CARTESIAN_POINT ( 'NONE',  ( -21.99213670719075253, -20.17946569659695299, 59.04970794435396897 ) ) ;
#33209=EDGE_CURVE ( 'NONE', #32817, #17131, #45703, .T. ) ;
#33210=CARTESIAN_POINT ( 'NONE',  ( -14.30855566557790226, -8.484641631233271752, 70.74429704309763167 ) ) ;
#33212=CYLINDRICAL_SURFACE ( 'NONE', #18218, 0.1500000000000006883 ) ;
#33213=EDGE_LOOP ( 'NONE', ( #37631, #35381, #832, #46037, #12112 ) ) ;
#33214=VERTEX_POINT ( 'NONE', #11961 ) ;
#33215=CARTESIAN_POINT ( 'NONE',  ( -16.94458633259734270, -7.374567983260779336, 74.14513688882354359 ) ) ;
#33216=CARTESIAN_POINT ( 'NONE',  ( -13.88293547364789227, -20.90532801101632643, 68.75625136993008368 ) ) ;
#33217=CARTESIAN_POINT ( 'NONE',  ( -10.70532053225239544, -12.67267096592666498, 61.08381491717225487 ) ) ;
#33218=FACE_OUTER_BOUND ( 'NONE', #12272, .T. ) ;
#33220=B_SPLINE_CURVE_WITH_KNOTS ( 'NONE', 1,
 ( #43546, #47703 ),
 .UNSPECIFIED., .F., .F.,
 ( 2, 2 ),
 ( 0.000000000000000000, 1.000000000000000000 ),
 .UNSPECIFIED. ) ;
#33221=CARTESIAN_POINT ( 'NONE',  ( -12.86353962931362283, -9.432586330540292607, 74.33395128836551180 ) ) ;
#33222=VERTEX_POINT ( 'NONE', #38268 ) ;
#33223=CARTESIAN_POINT ( 'NONE',  ( -13.63868562514487870, -21.22603565268462233, 68.59591802951210582 ) ) ;
#33224=( BOUNDED_SURFACE ( )  B_SPLINE_SURFACE ( 3, 1, ( 
 ( #6574, #47209 ),
 ( #47933, #36349 ),
 ( #10512, #25518 ),
 ( #35625, #1902 ),
 ( #16905, #48654 ),
 ( #33364, #10741 ),
 ( #34115, #406 ) ),
 .UNSPECIFIED., .T., .F., .F. ) 
 B_SPLINE_SURFACE_WITH_KNOTS ( ( 4, 3, 4 ),
 ( 2, 2 ),
 ( 0.000000000000000000, 0.5000000000000000000, 1.000000000000000000 ),
 ( 0.000000000000000000, 1.000000000000000000 ),
 .UNSPECIFIED. ) 
 GEOMETRIC_REPRESENTATION_ITEM ( )  RATIONAL_B_SPLINE_SURFACE ( (
 ( 1.000000000000000000, 1.000000000000000000),
 ( 0.3333333333333335369, 0.3333333333333330373),
 ( 0.3333333333333335369, 0.3333333333333330373),
 ( 1.000000000000000000, 1.000000000000000000),
 ( 0.3333333333333333703, 0.3333333333333333703),
 ( 0.3333333333333333703, 0.3333333333333333703),
 ( 1.000000000000000000, 1.000000000000000000) ) ) 
 REPRESENTATION_ITEM ( '' )  SURFACE ( )  );
#33225=CARTESIAN_POINT ( 'NONE',  ( -24.46479344177693349, -14.44719919422189491, 66.18292729247950490 ) ) ;
#33228=DIRECTION ( 'NONE',  ( 0.9811758422909350186, 0.1931164583992469597, 7.863147543881891826E-08 ) ) ;
#33230=CARTESIAN_POINT ( 'NONE',  ( -22.56207008003183745, -19.63703213565221262, 72.92928497383269359 ) ) ;
#33231=CARTESIAN_POINT ( 'NONE',  ( -19.42896739221782809, -21.56812523091047851, 62.29503644570711174 ) ) ;
#33233=CARTESIAN_POINT ( 'NONE',  ( -21.42336380182764088, -21.09487415076890215, 69.23945570945444672 ) ) ;
#33234=EDGE_CURVE ( 'NONE', #15728, #2461, #16102, .T. ) ;
#33235=ADVANCED_FACE ( 'NONE', ( #4559 ), #19331, .F. ) ;
#33236=CARTESIAN_POINT ( 'NONE',  ( -10.27345486655506868, -12.71824029969684844, 64.45331411623358520 ) ) ;
#33240=CARTESIAN_POINT ( 'NONE',  ( -23.85820194903862657, -17.69173191509663923, 62.48833042115953873 ) ) ;
#33242=CARTESIAN_POINT ( 'NONE',  ( -13.65684165595416921, -8.849801312179289781, 56.98439896120441261 ) ) ;
#33243=ORIENTED_EDGE ( 'NONE', *, *, #28832, .F. ) ;
#33244=CARTESIAN_POINT ( 'NONE',  ( -24.87272206221888737, -14.66350473979836444, 62.82022316917439042 ) ) ;
#33245=CYLINDRICAL_SURFACE ( 'NONE', #39194, 0.1499999999999995226 ) ;
#33246=CARTESIAN_POINT ( 'NONE',  ( -14.49299406798265011, -7.959851448313194133, 63.92945445847834662 ) ) ;
#33247=ADVANCED_FACE ( 'NONE', ( #42485 ), #19093, .T. ) ;
#33248=EDGE_CURVE ( 'NONE', #27479, #8282, #4054, .T. ) ;
#33251=CARTESIAN_POINT ( 'NONE',  ( -22.79434678427405814, -9.645412829818440059, 73.65878004203302964 ) ) ;
#33252=VERTEX_POINT ( 'NONE', #45932 ) ;
#33253=ORIENTED_EDGE ( 'NONE', *, *, #3409, .T. ) ;
#33254=CARTESIAN_POINT ( 'NONE',  ( -11.10470733248389230, -18.75498039752055490, 61.46206112672981448 ) ) ;
#33255=ORIENTED_EDGE ( 'NONE', *, *, #23876, .T. ) ;
#33256=CARTESIAN_POINT ( 'NONE',  ( -15.34355019510111617, -7.655489747179978544, 74.20172882442081175 ) ) ;
#33257=CARTESIAN_POINT ( 'NONE',  ( -11.71829917361626627, -18.86652339032711012, 71.75856246530707949 ) ) ;
#33258=CYLINDRICAL_SURFACE ( 'NONE', #34172, 0.4000000000000006883 ) ;
#33259=CARTESIAN_POINT ( 'NONE',  ( -12.50376689573318956, -9.829596806175777246, 57.37318925805055159 ) ) ;
#33260=CARTESIAN_POINT ( 'NONE',  ( -22.27695970603427966, -9.156476278077038344, 59.97817131676683999 ) ) ;
#33261=FACE_BOUND ( 'NONE', #17019, .T. ) ;
#33262=DIRECTION ( 'NONE',  ( -0.5652317888644005084, -0.8249321334856241084, 7.911723905267715079E-08 ) ) ;
#33263=CARTESIAN_POINT ( 'NONE',  ( -11.42803680512448850, -19.23074358453217414, 71.78711645111522444 ) ) ;
#33264=CARTESIAN_POINT ( 'NONE',  ( -16.74954601956997635, -21.77674034875754927, 68.69560679921868029 ) ) ;
#33265=EDGE_CURVE ( 'NONE', #18111, #14728, #43696, .T. ) ;
#33266=ORIENTED_EDGE ( 'NONE', *, *, #40247, .T. ) ;
#33268=CARTESIAN_POINT ( 'NONE',  ( -10.21764062494887781, -12.91954801228597915, 67.92327636273336111 ) ) ;
#33272=CARTESIAN_POINT ( 'NONE',  ( -13.71154894328531704, -21.26836094557570433, 68.49979187789318757 ) ) ;
#33273=CARTESIAN_POINT ( 'NONE',  ( -16.46055638328560278, -21.74386646685260160, 65.29734724012402580 ) ) ;
#33274=ORIENTED_EDGE ( 'NONE', *, *, #47084, .F. ) ;
#33275=EDGE_LOOP ( 'NONE', ( #41842, #20415 ) ) ;
#33277=EDGE_LOOP ( 'NONE', ( #37118, #46676, #47168, #9656, #25968 ) ) ;
#33280=CARTESIAN_POINT ( 'NONE',  ( -24.03543181337825629, -17.10925231076594599, 69.52225900064301811 ) ) ;
#33281=( BOUNDED_CURVE ( )  B_SPLINE_CURVE ( 3, ( #6252, #3507, #25675, #3021 ),
 .UNSPECIFIED., .F., .F. ) 
 B_SPLINE_CURVE_WITH_KNOTS ( ( 4, 4 ),
 ( 0.4074455897393663983, 0.5000000000000000000 ),
 .UNSPECIFIED. ) 
 CURVE ( )  GEOMETRIC_REPRESENTATION_ITEM ( )  RATIONAL_B_SPLINE_CURVE ( ( 0.6983129098260830725, 0.7760317562606791064, 0.8765941196519817513, 0.9999999999999834577 ) ) 
 REPRESENTATION_ITEM ( '' )  );
#33285=CARTESIAN_POINT ( 'NONE',  ( -13.42824119710918573, -20.62712141855529779, 65.13062048310476371 ) ) ;
#33286=CARTESIAN_POINT ( 'NONE',  ( -21.00380416015782004, -21.34292312329482399, 62.22976100777699315 ) ) ;
#33289=( BOUNDED_CURVE ( )  B_SPLINE_CURVE ( 3, ( #39877, #6151, #10086, #25110 ),
 .UNSPECIFIED., .F., .F. ) 
 B_SPLINE_CURVE_WITH_KNOTS ( ( 4, 4 ),
 ( 1.570796326794896558, 1.780235837034217283 ),
 .UNSPECIFIED. ) 
 CURVE ( )  GEOMETRIC_REPRESENTATION_ITEM ( )  RATIONAL_B_SPLINE_CURVE ( ( 1.000000000000000000, 0.9963479302455154896, 0.9963479302455154896, 1.000000000000000000 ) ) 
 REPRESENTATION_ITEM ( '' )  );
#33292=DIRECTION ( 'NONE',  ( -5.731567514496413899E-31, -1.020425574103664789E-16, -1.000000000000000000 ) ) ;
#33294=FACE_OUTER_BOUND ( 'NONE', #21786, .T. ) ;
#33296=CARTESIAN_POINT ( 'NONE',  ( -11.91859816416373441, -19.82845034313010402, 58.03408211766759450 ) ) ;
#33297=EDGE_CURVE ( 'NONE', #29013, #5623, #41753, .T. ) ;
#33298=DIRECTION ( 'NONE',  ( -1.684279434840741878E-06, 5.535644405454969375E-06, -0.9999999999832599462 ) ) ;
#33299=LINE ( 'NONE', #14575, #39204 ) ;
#33300=CARTESIAN_POINT ( 'NONE',  ( -17.28496127917699710, -14.43418371046636217, 47.99999999999994316 ) ) ;
#33301=ORIENTED_EDGE ( 'NONE', *, *, #16075, .F. ) ;
#33303=DIRECTION ( 'NONE',  ( 0.1539336739619741601, 0.9880811829098681276, 6.607022902453645889E-08 ) ) ;
#33304=CARTESIAN_POINT ( 'NONE',  ( -18.05334954050576357, -21.78092763974751733, 62.10209302353499794 ) ) ;
#33309=ORIENTED_EDGE ( 'NONE', *, *, #20237, .T. ) ;
#33311=CARTESIAN_POINT ( 'NONE',  ( -16.16063142123006813, -7.467037929575190525, 60.38523757159160965 ) ) ;
#33313=ORIENTED_EDGE ( 'NONE', *, *, #12884, .T. ) ;
#33314=CARTESIAN_POINT ( 'NONE',  ( -18.37542852932119430, -7.874153375602881866, 74.03167481725151333 ) ) ;
#33315=EDGE_CURVE ( 'NONE', #19358, #11201, #15330, .T. ) ;
#33316=CARTESIAN_POINT ( 'NONE',  ( -15.46798524158586119, -8.087945009721268619, 74.37985622463165214 ) ) ;
#33317=DIRECTION ( 'NONE',  ( -0.9796876409582463419, 0.2005296141562636081, 7.890952370353029293E-08 ) ) ;
#33318=ORIENTED_EDGE ( 'NONE', *, *, #20298, .F. ) ;
#33319=CARTESIAN_POINT ( 'NONE',  ( -10.04821600842096174, -15.85811274820897410, 64.62276192103250594 ) ) ;
#33320=CARTESIAN_POINT ( 'NONE',  ( -10.68182900717074091, -12.92559417569690439, 68.02215820193474372 ) ) ;
#33321=ORIENTED_EDGE ( 'NONE', *, *, #45847, .T. ) ;
#33323=ADVANCED_FACE ( 'NONE', ( #15136 ), #4326, .F. ) ;
#33324=VERTEX_POINT ( 'NONE', #30438 ) ;
#33326=CARTESIAN_POINT ( 'NONE',  ( -20.43185948505062299, -8.432683554863363184, 66.79576150497511833 ) ) ;
#33327=CARTESIAN_POINT ( 'NONE',  ( -18.57335281209669731, -21.76520412651811043, 72.57038810541313012 ) ) ;
#33328=CARTESIAN_POINT ( 'NONE',  ( -24.84853950285492630, -14.19203740149359483, 69.84549430759402355 ) ) ;
#33329=CARTESIAN_POINT ( 'NONE',  ( -13.30028440927262068, -8.603736347584243660, 60.62605674953037749 ) ) ;
#33330=ORIENTED_EDGE ( 'NONE', *, *, #47603, .F. ) ;
#33331=VERTEX_POINT ( 'NONE', #30194 ) ;
#33333=B_SPLINE_CURVE_WITH_KNOTS ( 'NONE', 3,
 ( #37837, #41054, #11749, #41541, #44764, #22334, #37094, #3881, #33636, #7826 ),
 .UNSPECIFIED., .F., .F.,
 ( 4, 2, 2, 2, 4 ),
 ( 0.000000000000000000, 0.2500000000000000000, 0.5000000000000000000, 0.7500000000000000000, 1.000000000000000000 ),
 .UNSPECIFIED. ) ;
#33334=CARTESIAN_POINT ( 'NONE',  ( -10.75506213788527887, -17.10647899198255217, 64.71919382801875997 ) ) ;
#33335=CARTESIAN_POINT ( 'NONE',  ( -10.81484442788029376, -17.11524687497682251, 61.45743118925498294 ) ) ;
#33338=( BOUNDED_SURFACE ( )  B_SPLINE_SURFACE ( 3, 1, ( 
 ( #25504, #16711 ),
 ( #17192, #24123 ),
 ( #32243, #42841 ),
 ( #28306, #20675 ),
 ( #36804, #31752 ),
 ( #24616, #44474 ),
 ( #46772, #40761 ) ),
 .UNSPECIFIED., .T., .F., .F. ) 
 B_SPLINE_SURFACE_WITH_KNOTS ( ( 4, 3, 4 ),
 ( 2, 2 ),
 ( 0.000000000000000000, 0.5000000000000000000, 1.000000000000000000 ),
 ( 0.000000000000000000, 1.000000000000000000 ),
 .UNSPECIFIED. ) 
 GEOMETRIC_REPRESENTATION_ITEM ( )  RATIONAL_B_SPLINE_SURFACE ( (
 ( 1.000000000000000000, 1.000000000000000000),
 ( 0.3333333333333335369, 0.3333333333333330373),
 ( 0.3333333333333335369, 0.3333333333333330373),
 ( 1.000000000000000000, 1.000000000000000000),
 ( 0.3333333333333333703, 0.3333333333333333703),
 ( 0.3333333333333333703, 0.3333333333333333703),
 ( 1.000000000000000000, 1.000000000000000000) ) ) 
 REPRESENTATION_ITEM ( '' )  SURFACE ( )  );
#33339=VERTEX_POINT ( 'NONE', #30921 ) ;
#33340=DIRECTION ( 'NONE',  ( 0.9375570856950865561, -0.3478314405900308492, 0.000000000000000000 ) ) ;
#33341=CARTESIAN_POINT ( 'NONE',  ( -12.26752988409003287, -16.72227946798956211, 54.49999999999995026 ) ) ;
#33342=CARTESIAN_POINT ( 'NONE',  ( -24.41275632663629125, -14.38907708926503126, 69.72445513987456422 ) ) ;
#33343=EDGE_CURVE ( 'NONE', #32538, #35964, #38649, .T. ) ;
#33344=ORIENTED_EDGE ( 'NONE', *, *, #31692, .F. ) ;
#33346=ORIENTED_EDGE ( 'NONE', *, *, #1151, .F. ) ;
#33347=CARTESIAN_POINT ( 'NONE',  ( -13.44410990971816666, -8.986443949771105721, 64.32435409333248799 ) ) ;
#33348=CARTESIAN_POINT ( 'NONE',  ( -19.56314425575162730, -21.47449014599886752, 65.46486235662891318 ) ) ;
#33350=CARTESIAN_POINT ( 'NONE',  ( -11.39127492490111315, -11.16067319722467843, 60.69357916181100876 ) ) ;
#33351=EDGE_CURVE ( 'NONE', #7024, #32569, #11913, .T. ) ;
#33355=CARTESIAN_POINT ( 'NONE',  ( -19.36100759928269355, -7.615224647604666330, 60.12126342487893282 ) ) ;
#33357=VERTEX_POINT ( 'NONE', #8994 ) ;
#33360=CARTESIAN_POINT ( 'NONE',  ( -18.90456104531098092, -7.507023198961870314, 70.55723427638547207 ) ) ;
#33362=FACE_BOUND ( 'NONE', #564, .T. ) ;
#33363=ORIENTED_EDGE ( 'NONE', *, *, #39179, .F. ) ;
#33364=CARTESIAN_POINT ( 'NONE',  ( -10.64331041279003642, -16.74977650942914309, 58.10249305398041741 ) ) ;
#33365=CARTESIAN_POINT ( 'NONE',  ( -13.57571756020798581, -20.65642803140422856, 61.51646323935151628 ) ) ;
#33366=CARTESIAN_POINT ( 'NONE',  ( -14.90981263331598328, -21.39562362703504306, 61.93600440604522817 ) ) ;
#33367=ADVANCED_FACE ( 'NONE', ( #47393 ), #45572, .T. ) ;
#33369=ORIENTED_EDGE ( 'NONE', *, *, #10601, .F. ) ;
#33370=CARTESIAN_POINT ( 'NONE',  ( -10.45275823860530906, -14.15883715200053317, 64.49876946959942359 ) ) ;
#33372=ORIENTED_EDGE ( 'NONE', *, *, #19487, .F. ) ;
#33373=DIRECTION ( 'NONE',  ( -0.6990986543038602008, -0.7150252244155670400, 1.750055599226864974E-16 ) ) ;
#33374=CARTESIAN_POINT ( 'NONE',  ( -23.37526786102125342, -18.49490670617680266, 69.52045215527557787 ) ) ;
#33375=ORIENTED_EDGE ( 'NONE', *, *, #33182, .F. ) ;
#33376=CARTESIAN_POINT ( 'NONE',  ( -10.53028993777715883, -16.28642212234895226, 71.73278239416407587 ) ) ;
#33378=EDGE_CURVE ( 'NONE', #32027, #22984, #1834, .T. ) ;
#33379=CARTESIAN_POINT ( 'NONE',  ( -14.96332094776524357, -21.84106950312725459, 65.25596681347286676 ) ) ;
#33381=ORIENTED_EDGE ( 'NONE', *, *, #150, .T. ) ;
#33384=CARTESIAN_POINT ( 'NONE',  ( -22.34470984022960138, -19.78791505225649416, 69.17417989488706098 ) ) ;
#33385=CARTESIAN_POINT ( 'NONE',  ( -10.12326218194131044, -13.32541594658350448, 74.86312942357149325 ) ) ;
#33386=CARTESIAN_POINT ( 'NONE',  ( -10.03304496037382698, -13.87377773147474613, 57.64813805078288311 ) ) ;
#33389=DIRECTION ( 'NONE',  ( 2.515468002857175786E-08, 7.569577117229404680E-10, -0.9999999999999997780 ) ) ;
#33391=ORIENTED_EDGE ( 'NONE', *, *, #23691, .F. ) ;
#33393=B_SPLINE_CURVE_WITH_KNOTS ( 'NONE', 1,
 ( #3908, #19154 ),
 .UNSPECIFIED., .F., .F.,
 ( 2, 2 ),
 ( 0.000000000000000000, 1.000000000000000000 ),
 .UNSPECIFIED. ) ;
#33394=CARTESIAN_POINT ( 'NONE',  ( -12.09316379863263613, -10.27246524284629636, 64.10202428021784726 ) ) ;
#33395=DIRECTION ( 'NONE',  ( 1.148482745121145911E-06, -2.957121390393632846E-08, -0.9999999999993400834 ) ) ;
#33396=CARTESIAN_POINT ( 'NONE',  ( -21.07246205680086959, -21.30487707300596512, 62.23658632844267657 ) ) ;
#33401=ORIENTED_EDGE ( 'NONE', *, *, #39173, .F. ) ;
#33402=CARTESIAN_POINT ( 'NONE',  ( -24.33858701346967734, -15.90815918667622775, 69.76137442214673001 ) ) ;
#33403=CARTESIAN_POINT ( 'NONE',  ( -24.08517543038346531, -12.49907855475201579, 73.52753481283211556 ) ) ;
#33404=DIRECTION ( 'NONE',  ( -0.9974380310868017352, -0.07153582418399355436, 3.008056591778321396E-08 ) ) ;
#33405=EDGE_CURVE ( 'NONE', #48003, #28824, #21548, .T. ) ;
#33406=VERTEX_POINT ( 'NONE', #6263 ) ;
#33407=B_SPLINE_CURVE_WITH_KNOTS ( 'NONE', 3,
 ( #17866, #9789, #32665, #2386, #6078, #13924, #47685, #10019, #14164, #25289 ),
 .UNSPECIFIED., .F., .F.,
 ( 4, 2, 2, 2, 4 ),
 ( 0.6272669072877528063, 0.7522669073072690837, 0.8772669073267853612, 1.002266907346301750, 1.127266907365817916 ),
 .UNSPECIFIED. ) ;
#33408=VECTOR ( 'NONE', #6477, 1000.000000000000114 ) ;
#33409=CARTESIAN_POINT ( 'NONE',  ( -10.49189908542464522, -16.09426454567519116, 68.26295692486267797 ) ) ;
#33410=ORIENTED_EDGE ( 'NONE', *, *, #31504, .T. ) ;
#33411=DIRECTION ( 'NONE',  ( 0.9640890753730593232, -0.2655790932026004803, 6.310348465037888425E-08 ) ) ;
#33412=( BOUNDED_CURVE ( )  B_SPLINE_CURVE ( 3, ( #43424, #47822, #14058, #39711 ),
 .UNSPECIFIED., .F., .F. ) 
 B_SPLINE_CURVE_WITH_KNOTS ( ( 4, 4 ),
 ( 0.4074455897393701731, 0.5000000000000000000 ),
 .UNSPECIFIED. ) 
 CURVE ( )  GEOMETRIC_REPRESENTATION_ITEM ( )  RATIONAL_B_SPLINE_CURVE ( ( 0.6983129098261028345, 0.7760317562607076392, 0.8765941196520069534, 1.000000000000001554 ) ) 
 REPRESENTATION_ITEM ( '' )  );
#33414=EDGE_LOOP ( 'NONE', ( #46475, #12153, #14173, #5557, #37945 ) ) ;
#33415=CARTESIAN_POINT ( 'NONE',  ( -15.68502974777997316, -7.977065180327442384, 70.90989839958919561 ) ) ;
#33416=ORIENTED_EDGE ( 'NONE', *, *, #18522, .T. ) ;
#33419=CARTESIAN_POINT ( 'NONE',  ( -12.25221656496721856, -10.01269428147863749, 57.08935561312273421 ) ) ;
#33420=ORIENTED_EDGE ( 'NONE', *, *, #16956, .F. ) ;
#33421=CARTESIAN_POINT ( 'NONE',  ( -22.26148258426732340, -19.94273495432607035, 62.44259083056840609 ) ) ;
#33422=CARTESIAN_POINT ( 'NONE',  ( -18.58312024667335294, -22.16850747602615357, 72.38487304212588924 ) ) ;
#33423=EDGE_CURVE ( 'NONE', #6404, #20491, #42124, .T. ) ;
#33424=EDGE_LOOP ( 'NONE', ( #25243, #13059 ) ) ;
#33425=LINE ( 'NONE', #22377, #11890 ) ;
#33427=( BOUNDED_CURVE ( )  B_SPLINE_CURVE ( 3, ( #7539, #4328, #23286, #41255 ),
 .UNSPECIFIED., .F., .F. ) 
 B_SPLINE_CURVE_WITH_KNOTS ( ( 4, 4 ),
 ( 0.5000000000000000000, 0.9074455897393596260 ),
 .UNSPECIFIED. ) 
 CURVE ( )  GEOMETRIC_REPRESENTATION_ITEM ( )  RATIONAL_B_SPLINE_CURVE ( ( 1.000000000000021538, 0.4567392136813413495, 0.3561768502900184985, 0.6983129098260767442 ) ) 
 REPRESENTATION_ITEM ( '' )  );
#33428=CARTESIAN_POINT ( 'NONE',  ( -23.85760449859744625, -11.05106826658364838, 70.00555402674318373 ) ) ;
#33430=( BOUNDED_CURVE ( )  B_SPLINE_CURVE ( 3, ( #6787, #31987, #21800, #7038 ),
 .UNSPECIFIED., .F., .F. ) 
 B_SPLINE_CURVE_WITH_KNOTS ( ( 4, 4 ),
 ( 0.9074455897393665094, 1.000000000000000000 ),
 .UNSPECIFIED. ) 
 CURVE ( )  GEOMETRIC_REPRESENTATION_ITEM ( )  RATIONAL_B_SPLINE_CURVE ( ( 0.6983129098260950629, 0.7760317562606999786, 0.8765941196520016243, 1.000000000000000000 ) ) 
 REPRESENTATION_ITEM ( '' )  );
#33432=EDGE_CURVE ( 'NONE', #20123, #12513, #43462, .T. ) ;
#33433=CARTESIAN_POINT ( 'NONE',  ( -12.81450749931373245, -9.474957484202729319, 74.31923006089486705 ) ) ;
#33434=DIRECTION ( 'NONE',  ( -3.827383491158052452E-06, 8.363078748037870009E-06, 0.9999999999577049437 ) ) ;
#33435=ORIENTED_EDGE ( 'NONE', *, *, #38447, .T. ) ;
#33436=ORIENTED_EDGE ( 'NONE', *, *, #16204, .F. ) ;
#33437=CARTESIAN_POINT ( 'NONE',  ( -22.91296630721855365, -15.15889098507617128, 53.49999999999995026 ) ) ;
#33438=CARTESIAN_POINT ( 'NONE',  ( -24.37445139888341927, -16.03700657411734198, 59.27899288712937675 ) ) ;
#33439=DIRECTION ( 'NONE',  ( 0.2075053346947366428, -0.3961584734335814040, 0.8944271909999158554 ) ) ;
#33442=DIRECTION ( 'NONE',  ( 0.8858372764600287441, 0.4639960340712823705, 2.848505657311695038E-17 ) ) ;
#33443=CARTESIAN_POINT ( 'NONE',  ( -12.95890174405234241, -8.844667670358365541, 67.56598159878524257 ) ) ;
#33444=CARTESIAN_POINT ( 'NONE',  ( -24.08638337272136098, -17.13919944035470522, 66.09924551876292753 ) ) ;
#33445=( BOUNDED_CURVE ( )  B_SPLINE_CURVE ( 3, ( #19410, #27288, #30759, #46012 ),
 .UNSPECIFIED., .F., .F. ) 
 B_SPLINE_CURVE_WITH_KNOTS ( ( 4, 4 ),
 ( 0.5000000000000000000, 0.9074455897393702841 ),
 .UNSPECIFIED. ) 
 CURVE ( )  GEOMETRIC_REPRESENTATION_ITEM ( )  RATIONAL_B_SPLINE_CURVE ( ( 1.000000000000007772, 0.4567392136813255843, 0.3561768502900223288, 0.6983129098261066092 ) ) 
 REPRESENTATION_ITEM ( '' )  );
#33448=ORIENTED_EDGE ( 'NONE', *, *, #15545, .T. ) ;
#33449=CARTESIAN_POINT ( 'NONE',  ( -24.32852063849251323, -13.38246526728995001, 59.37740068604990995 ) ) ;
#33450=CARTESIAN_POINT ( 'NONE',  ( -14.19282086353638839, -8.542981675383003903, 71.01485553001869278 ) ) ;
#33451=CARTESIAN_POINT ( 'NONE',  ( -19.99112977906324318, -8.296885409642934306, 74.02096600045412345 ) ) ;
#33452=CARTESIAN_POINT ( 'NONE',  ( -10.52701369859243208, -13.34860595097322111, 74.67817664682546308 ) ) ;
#33453=ADVANCED_FACE ( 'NONE', ( #16359 ), #31389, .T. ) ;
#33456=ORIENTED_EDGE ( 'NONE', *, *, #19264, .T. ) ;
#33459=CARTESIAN_POINT ( 'NONE',  ( -10.64450000169400035, -13.06134498814596334, 71.27998937039448890 ) ) ;
#33460=CARTESIAN_POINT ( 'NONE',  ( -11.68183240635974407, -10.06254296414596539, 67.67613765047124730 ) ) ;
#33461=DIRECTION ( 'NONE',  ( 0.9991556020692451412, -0.04108628546905146450, 1.062351070541542511E-16 ) ) ;
#33462=ORIENTED_EDGE ( 'NONE', *, *, #32405, .F. ) ;
#33463=CARTESIAN_POINT ( 'NONE',  ( -11.42622084110231029, -18.51434063454204093, 61.27710833181470917 ) ) ;
#33464=CARTESIAN_POINT ( 'NONE',  ( -22.98984126167822239, -19.13650646057006099, 58.88410662258176842 ) ) ;
#33465=ORIENTED_EDGE ( 'NONE', *, *, #24071, .T. ) ;
#33467=CARTESIAN_POINT ( 'NONE',  ( -17.49776267610204528, -21.86253320314435200, 58.70553367701982239 ) ) ;
#33468=CARTESIAN_POINT ( 'NONE',  ( -14.01837044221388417, -8.636059239884620098, 74.48482605064899076 ) ) ;
#33469=ORIENTED_EDGE ( 'NONE', *, *, #40499, .F. ) ;
#33470=CARTESIAN_POINT ( 'NONE',  ( -21.65477468606848532, -9.232349032746775208, 66.96149992608901869 ) ) ;
#33473=B_SPLINE_CURVE_WITH_KNOTS ( 'NONE', 1,
 ( #42383, #46070 ),
 .UNSPECIFIED., .F., .F.,
 ( 2, 2 ),
 ( 0.000000000000000000, 1.000000000000000000 ),
 .UNSPECIFIED. ) ;
#33474=CARTESIAN_POINT ( 'NONE',  ( -10.44610064225645019, -17.41918600737009015, 64.75022468138659804 ) ) ;
#33475=CARTESIAN_POINT ( 'NONE',  ( -17.19980212172655953, -7.762775302065858085, 70.79035839668003405 ) ) ;
#33477=CARTESIAN_POINT ( 'NONE',  ( -16.19792114999740562, -7.866354181730329742, 60.48556343814865954 ) ) ;
#33480=DIRECTION ( 'NONE',  ( -0.6771828760946864145, 0.7358147540815750398, -3.419290845356464415E-09 ) ) ;
#33481=CARTESIAN_POINT ( 'NONE',  ( -10.53536195276627829, -13.30851587854854579, 74.69289754060230280 ) ) ;
#33483=FACE_OUTER_BOUND ( 'NONE', #26928, .T. ) ;
#33484=EDGE_LOOP ( 'NONE', ( #40136, #1415 ) ) ;
#33487=CARTESIAN_POINT ( 'NONE',  ( -14.42127303407290384, -7.991116021394736535, 63.98253012168138554 ) ) ;
#33488=DIRECTION ( 'NONE',  ( 0.3478314405900309603, 0.9375570856950864451, -9.567072274253696421E-17 ) ) ;
#33489=ADVANCED_FACE ( 'NONE', ( #2320 ), #13465, .T. ) ;
#33490=CARTESIAN_POINT ( 'NONE',  ( -16.13432406759100246, -21.74052631579560568, 58.30057715624173653 ) ) ;
#33491=CARTESIAN_POINT ( 'NONE',  ( -17.15997071016939302, -7.814068483533316289, 70.79035844394253729 ) ) ;
#33493=ORIENTED_EDGE ( 'NONE', *, *, #46151, .T. ) ;
#33494=B_SPLINE_CURVE_WITH_KNOTS ( 'NONE', 3,
 ( #15933, #46486, #16662, #31449, #5357, #38593, #30977, #27755, #31696, #27272 ),
 .UNSPECIFIED., .F., .F.,
 ( 4, 2, 2, 2, 4 ),
 ( 0.000000000000000000, 0.2500000000000000000, 0.5000000000000000000, 0.7500000000000000000, 1.000000000000000000 ),
 .UNSPECIFIED. ) ;
#33495=CARTESIAN_POINT ( 'NONE',  ( -11.13733870171179596, -11.61806121328041996, 67.90392505421056057 ) ) ;
#33497=EDGE_LOOP ( 'NONE', ( #24461, #29373, #32887, #43165, #10521 ) ) ;
#33498=CARTESIAN_POINT ( 'NONE',  ( -10.74628672884880132, -17.07053172313825939, 61.17215199736627795 ) ) ;
#33501=CARTESIAN_POINT ( 'NONE',  ( -20.68882847039305872, -8.112503303873584315, 63.43308756725068775 ) ) ;
#33502=CARTESIAN_POINT ( 'NONE',  ( -21.94242186726961208, -9.397052521110282441, 60.00699132926281010 ) ) ;
#33503=CARTESIAN_POINT ( 'NONE',  ( -17.42409385541300892, -14.80920654474439679, 47.99999999999994316 ) ) ;
#33504=CARTESIAN_POINT ( 'NONE',  ( -11.44306888606149819, -19.25104975142471986, 71.88674653068365217 ) ) ;
#33505=CARTESIAN_POINT ( 'NONE',  ( -11.41497376296057098, -19.21309731666858411, 71.80190493362104576 ) ) ;
#33506=CARTESIAN_POINT ( 'NONE',  ( -21.99178428503401861, -9.439038574390064440, 60.02171213140443484 ) ) ;
#33508=CARTESIAN_POINT ( 'NONE',  ( -24.30048669258562200, -16.36410883687464590, 59.42332431756338451 ) ) ;
#33509=CARTESIAN_POINT ( 'NONE',  ( -11.50943330868083514, -18.55322154803265988, 61.56245428017365384 ) ) ;
#33511=CARTESIAN_POINT ( 'NONE',  ( -24.27425349805069033, -13.36807680166415402, 59.36267976138583435 ) ) ;
#33512=CARTESIAN_POINT ( 'NONE',  ( -11.77467277675836321, -9.951459619914194477, 64.14259051640634368 ) ) ;
#33514=FACE_OUTER_BOUND ( 'NONE', #21679, .T. ) ;
#33519=AXIS2_PLACEMENT_3D ( 'NONE', #38383, #42099, #12293 ) ;
#33523=EDGE_CURVE ( 'NONE', #12218, #31226, #2781, .T. ) ;
#33524=DIRECTION ( 'NONE',  ( 0.6827297667453423591, 0.7306709694519485376, 5.176517822219622992E-09 ) ) ;
#33525=CARTESIAN_POINT ( 'NONE',  ( -22.47245519635065492, -19.73066437834766873, 72.65872596779033188 ) ) ;
#33526=( BOUNDED_CURVE ( )  B_SPLINE_CURVE ( 3, ( #40623, #37159, #29808, #44838 ),
 .UNSPECIFIED., .F., .F. ) 
 B_SPLINE_CURVE_WITH_KNOTS ( ( 4, 4 ),
 ( 1.570796326794896558, 1.780235837034216617 ),
 .UNSPECIFIED. ) 
 CURVE ( )  GEOMETRIC_REPRESENTATION_ITEM ( )  RATIONAL_B_SPLINE_CURVE ( ( 1.000000000000000000, 0.9963479302455154896, 0.9963479302455154896, 1.000000000000000000 ) ) 
 REPRESENTATION_ITEM ( '' )  );
#33528=CARTESIAN_POINT ( 'NONE',  ( -23.23616624490289695, -18.79948399208958776, 66.12389430041484673 ) ) ;
#33529=VERTEX_POINT ( 'NONE', #18537 ) ;
#33532=ORIENTED_EDGE ( 'NONE', *, *, #36457, .F. ) ;
#33533=CARTESIAN_POINT ( 'NONE',  ( -23.49605051889219709, -11.22618518380361152, 73.37665428612797314 ) ) ;
#33534=CARTESIAN_POINT ( 'NONE',  ( -14.69894550035548875, -21.31512775581534669, 61.72780404081314742 ) ) ;
#33535=ORIENTED_EDGE ( 'NONE', *, *, #39480, .T. ) ;
#33536=CARTESIAN_POINT ( 'NONE',  ( -17.76832444385116005, -7.367037027254299986, 60.25777669754219801 ) ) ;
#33539=ORIENTED_EDGE ( 'NONE', *, *, #25989, .F. ) ;
#33543=B_SPLINE_CURVE_WITH_KNOTS ( 'NONE', 3,
 ( #35347, #42020, #8289, #1615, #6228, #27237, #21253, #46445, #900, #20339 ),
 .UNSPECIFIED., .F., .F.,
 ( 4, 2, 2, 2, 4 ),
 ( 0.1272669073658828920, 0.2522669073463614242, 0.3772669073268399842, 0.5022669073073184887, 0.6272669072877969931 ),
 .UNSPECIFIED. ) ;
#33544=CARTESIAN_POINT ( 'NONE',  ( -10.75256062612175967, -17.08851307629239358, 61.16302898656469722 ) ) ;
#33545=CARTESIAN_POINT ( 'NONE',  ( -15.50089181596375276, -21.59567371606877728, 68.57592836473452280 ) ) ;
#33546=ORIENTED_EDGE ( 'NONE', *, *, #977, .T. ) ;
#33547=CARTESIAN_POINT ( 'NONE',  ( -11.95727733380162050, -19.27338395605723420, 71.84252737392968413 ) ) ;
#33548=LINE ( 'NONE', #48593, #11711 ) ;
#33552=CARTESIAN_POINT ( 'NONE',  ( -17.99499063918263886, -21.78594895119847763, 62.16070588972903010 ) ) ;
#33554=EDGE_CURVE ( 'NONE', #42239, #42405, #29633, .T. ) ;
#33555=VERTEX_POINT ( 'NONE', #10678 ) ;
#33557=CARTESIAN_POINT ( 'NONE',  ( -24.69852204723760281, -16.41745771733451775, 59.30827817708741634 ) ) ;
#33558=CARTESIAN_POINT ( 'NONE',  ( -24.69822986944709697, -13.19963441799314197, 59.54763197719577761 ) ) ;
#33561=CARTESIAN_POINT ( 'NONE',  ( -11.57425499491753307, -18.65360305739656610, 64.74707076836355668 ) ) ;
#33562=DIRECTION ( 'NONE',  ( -2.526377660313140381E-06, -1.273612632024531482E-05, 0.9999999999157043185 ) ) ;
#33563=EDGE_LOOP ( 'NONE', ( #43382, #19179, #27654, #40273, #47946 ) ) ;
#33564=FACE_OUTER_BOUND ( 'NONE', #19194, .T. ) ;
#33565=CARTESIAN_POINT ( 'NONE',  ( -14.59990505495813728, -21.70320363700883703, 58.27279595847587501 ) ) ;
#33567=ORIENTED_EDGE ( 'NONE', *, *, #40332, .F. ) ;
#33569=CARTESIAN_POINT ( 'NONE',  ( -14.27319502748954783, -8.558459675072437989, 70.72957628730870283 ) ) ;
#33570=FACE_OUTER_BOUND ( 'NONE', #41136, .T. ) ;
#33571=( BOUNDED_SURFACE ( )  B_SPLINE_SURFACE ( 3, 1, ( 
 ( #37254, #41455 ),
 ( #29407, #30395 ),
 ( #36759, #37755 ),
 ( #19054, #22019 ),
 ( #4055, #34060 ),
 ( #15336, #44440 ),
 ( #3301, #37016 ) ),
 .UNSPECIFIED., .T., .F., .F. ) 
 B_SPLINE_SURFACE_WITH_KNOTS ( ( 4, 3, 4 ),
 ( 2, 2 ),
 ( 0.000000000000000000, 0.5000000000000000000, 1.000000000000000000 ),
 ( 0.000000000000000000, 1.000000000000000000 ),
 .UNSPECIFIED. ) 
 GEOMETRIC_REPRESENTATION_ITEM ( )  RATIONAL_B_SPLINE_SURFACE ( (
 ( 1.000000000000000000, 1.000000000000000000),
 ( 0.3333333333333335369, 0.3333333333333330373),
 ( 0.3333333333333335369, 0.3333333333333330373),
 ( 1.000000000000000000, 1.000000000000000000),
 ( 0.3333333333333333703, 0.3333333333333333703),
 ( 0.3333333333333333703, 0.3333333333333333703),
 ( 1.000000000000000000, 1.000000000000000000) ) ) 
 REPRESENTATION_ITEM ( '' )  SURFACE ( )  );
#33573=CARTESIAN_POINT ( 'NONE',  ( -21.34582186320181307, -20.66775149956831115, 72.82446429489806405 ) ) ;
#33574=ORIENTED_EDGE ( 'NONE', *, *, #21074, .T. ) ;
#33575=VERTEX_POINT ( 'NONE', #2570 ) ;
#33577=ADVANCED_FACE ( 'NONE', ( #29889 ), #25690, .T. ) ;
#33578=EDGE_CURVE ( 'NONE', #44829, #23300, #44480, .T. ) ;
#33579=CARTESIAN_POINT ( 'NONE',  ( -11.44414087091985621, -10.36592030450376711, 74.63873809041486140 ) ) ;
#33580=CARTESIAN_POINT ( 'NONE',  ( -10.86049441902023460, -17.24231142387962024, 61.23031190884537978 ) ) ;
#33582=( BOUNDED_CURVE ( )  B_SPLINE_CURVE ( 3, ( #24692, #13332, #20257, #16298 ),
 .UNSPECIFIED., .F., .F. ) 
 B_SPLINE_CURVE_WITH_KNOTS ( ( 4, 4 ),
 ( 0.5000000000000000000, 0.9074455897393632897 ),
 .UNSPECIFIED. ) 
 CURVE ( )  GEOMETRIC_REPRESENTATION_ITEM ( )  RATIONAL_B_SPLINE_CURVE ( ( 1.000000000000013989, 0.4567392136813422931, 0.3561768502900243827, 0.6983129098260750789 ) ) 
 REPRESENTATION_ITEM ( '' )  );
#33585=EDGE_CURVE ( 'NONE', #42260, #42072, #3118, .T. ) ;
#33586=ORIENTED_EDGE ( 'NONE', *, *, #28188, .F. ) ;
#33587=CARTESIAN_POINT ( 'NONE',  ( -21.01124108229941001, -20.87838065962769463, 65.88453944495783787 ) ) ;
#33588=EDGE_CURVE ( 'NONE', #44748, #21822, #5011, .T. ) ;
#33589=CARTESIAN_POINT ( 'NONE',  ( -10.48860011681506599, -16.07550809128320424, 68.27208010408295991 ) ) ;
#33591=EDGE_CURVE ( 'NONE', #45956, #1066, #6584, .T. ) ;
#33592=CARTESIAN_POINT ( 'NONE',  ( -24.34278085428046268, -16.17909949234452682, 66.47813813521833026 ) ) ;
#33593=ORIENTED_EDGE ( 'NONE', *, *, #26943, .T. ) ;
#33594=CARTESIAN_POINT ( 'NONE',  ( -24.47368665962210343, -14.70950332193510590, 62.72768537250228604 ) ) ;
#33596=CARTESIAN_POINT ( 'NONE',  ( -13.11130243257871264, -9.228466417706050251, 63.79457649077198056 ) ) ;
#33597=CARTESIAN_POINT ( 'NONE',  ( -10.11537057477133139, -16.25405092646076710, 71.58717057996463495 ) ) ;
#33599=DIRECTION ( 'NONE',  ( 0.4846961512978548159, 0.8746825943832683414, 4.196010046976493442E-08 ) ) ;
#33600=EDGE_CURVE ( 'NONE', #18426, #21687, #35656, .T. ) ;
#33601=ORIENTED_EDGE ( 'NONE', *, *, #13096, .F. ) ;
#33602=CARTESIAN_POINT ( 'NONE',  ( -10.40174226954351866, -17.29724918936392442, 61.34238429002267878 ) ) ;
#33604=DIRECTION ( 'NONE',  ( 3.549360974554993999E-17, -6.371834667797928663E-18, -1.000000000000000000 ) ) ;
#33605=CARTESIAN_POINT ( 'NONE',  ( -10.64577744754535082, -11.71757184301072563, 74.67344733366148546 ) ) ;
#33608=DIRECTION ( 'NONE',  ( 0.1666496227699783561, -0.9805797387979530155, 0.1033986416233892980 ) ) ;
#33609=CARTESIAN_POINT ( 'NONE',  ( -10.72305181292425758, -11.55365095252855490, 71.28872070803703309 ) ) ;
#33610=FACE_BOUND ( 'NONE', #25811, .T. ) ;
#33611=EDGE_LOOP ( 'NONE', ( #3091, #31255, #2958, #22381, #41533 ) ) ;
#33612=CARTESIAN_POINT ( 'NONE',  ( -21.37361950556103807, -20.65352744038741051, 69.05449913549048802 ) ) ;
#33613=CARTESIAN_POINT ( 'NONE',  ( -10.81908394905857129, -17.27465539222630042, 64.63299147090781105 ) ) ;
#33616=CARTESIAN_POINT ( 'NONE',  ( -21.50087588749055811, -8.572740410265922151, 73.71473348964758543 ) ) ;
#33617=ORIENTED_EDGE ( 'NONE', *, *, #21097, .T. ) ;
#33619=ORIENTED_EDGE ( 'NONE', *, *, #27212, .T. ) ;
#33620=CARTESIAN_POINT ( 'NONE',  ( -21.36489679027069499, -8.963475500412677377, 73.60128753237400190 ) ) ;
#33621=CARTESIAN_POINT ( 'NONE',  ( -21.61813339613238227, -8.651787399021619862, 73.71633365192373333 ) ) ;
#33623=CARTESIAN_POINT ( 'NONE',  ( -12.68532353738824803, -9.060482037740600347, 71.03420644255490402 ) ) ;
#33626=CARTESIAN_POINT ( 'NONE',  ( -18.32164519516739531, -22.20506541443370452, 68.99327472290880792 ) ) ;
#33627=ORIENTED_EDGE ( 'NONE', *, *, #12067, .T. ) ;
#33628=ORIENTED_EDGE ( 'NONE', *, *, #31968, .F. ) ;
#33629=ORIENTED_EDGE ( 'NONE', *, *, #40609, .T. ) ;
#33630=CARTESIAN_POINT ( 'NONE',  ( -12.01648161716052776, -10.28590799842451098, 67.79896869921920199 ) ) ;
#33631=CARTESIAN_POINT ( 'NONE',  ( -22.71446019751790502, -13.25678923272456977, 53.88362224778183673 ) ) ;
#33633=CARTESIAN_POINT ( 'NONE',  ( -12.50776718604994109, -20.40684089597385764, 71.92158360616595303 ) ) ;
#33634=PLANE ( 'NONE',  #38138 ) ;
#33635=ADVANCED_FACE ( 'NONE', ( #26679 ), #12138, .T. ) ;
#33636=CARTESIAN_POINT ( 'NONE',  ( -14.13370355700781822, -8.630624683693202570, 74.49954649408729779 ) ) ;
#33640=ORIENTED_EDGE ( 'NONE', *, *, #41129, .T. ) ;
#33641=CARTESIAN_POINT ( 'NONE',  ( -16.23115966991289127, -7.455249367085269974, 60.31533194998537084 ) ) ;
#33642=EDGE_CURVE ( 'NONE', #41432, #15343, #37385, .T. ) ;
#33643=CARTESIAN_POINT ( 'NONE',  ( -22.50034801104533599, -20.26212632374907230, 65.80447478980116216 ) ) ;
#33644=DIRECTION ( 'NONE',  ( -0.3996021513128670266, -0.9166886716143755054, -9.834836654444679756E-09 ) ) ;
#33645=CARTESIAN_POINT ( 'NONE',  ( -24.44689184067228638, -14.18710713894228270, 69.93803194250308763 ) ) ;
#33648=ORIENTED_EDGE ( 'NONE', *, *, #35573, .T. ) ;
#33649=CARTESIAN_POINT ( 'NONE',  ( -11.96181355942711910, -19.87549434724351727, 58.11177690156993947 ) ) ;
#33650=EDGE_CURVE ( 'NONE', #15048, #32429, #19186, .T. ) ;
#33652=CARTESIAN_POINT ( 'NONE',  ( -15.29809733969474195, -21.47854975192407778, 68.87592918283094434 ) ) ;
#33655=ORIENTED_EDGE ( 'NONE', *, *, #33315, .F. ) ;
#33656=CARTESIAN_POINT ( 'NONE',  ( -20.39526016292127863, -7.977138075681091678, 70.41246825231446849 ) ) ;
#33659=CARTESIAN_POINT ( 'NONE',  ( -22.96484172783137012, -19.08706962207428504, 58.88410642316259214 ) ) ;
#33660=VERTEX_POINT ( 'NONE', #34786 ) ;
#33661=CARTESIAN_POINT ( 'NONE',  ( -22.23733845922741637, -19.96043711175405733, 66.00421731380804147 ) ) ;
#33662=EDGE_CURVE ( 'NONE', #44341, #28874, #7517, .T. ) ;
#33663=CARTESIAN_POINT ( 'NONE',  ( -10.13542349758729522, -16.35201950153232175, 71.58603826798915293 ) ) ;
#33664=CARTESIAN_POINT ( 'NONE',  ( -19.11145557798581152, -7.964112677450091660, 63.73089235102099792 ) ) ;
#33666=LINE ( 'NONE', #33415, #14130 ) ;
#33667=ORIENTED_EDGE ( 'NONE', *, *, #618, .F. ) ;
#33668=CARTESIAN_POINT ( 'NONE',  ( -10.15133553508400510, -13.19036488398009510, 71.32173201719281508 ) ) ;
#33669=CYLINDRICAL_SURFACE ( 'NONE', #30405, 0.1500000000000051847 ) ;
#33670=EDGE_LOOP ( 'NONE', ( #12870, #11981, #37508, #23446 ) ) ;
#33671=CARTESIAN_POINT ( 'NONE',  ( -12.90353999865511625, -8.887351178413068098, 67.49447498869417927 ) ) ;
#33673=ORIENTED_EDGE ( 'NONE', *, *, #2469, .T. ) ;
#33674=CARTESIAN_POINT ( 'NONE',  ( -22.13045097303941233, -9.033809248834419492, 63.33120398871400170 ) ) ;
#33675=CARTESIAN_POINT ( 'NONE',  ( -22.30126494710644636, -19.83056690705673830, 65.93095126885788204 ) ) ;
#33677=EDGE_LOOP ( 'NONE', ( #24332, #3874 ) ) ;
#33678=CARTESIAN_POINT ( 'NONE',  ( -12.74836358285320159, -20.08597126951521261, 71.82125749157572159 ) ) ;
#33679=CARTESIAN_POINT ( 'NONE',  ( -20.81428279164019202, -20.99479176755810883, 65.88454167459703115 ) ) ;
#33680=CARTESIAN_POINT ( 'NONE',  ( -20.19231657184298356, -8.325423463105360966, 70.25100341277898508 ) ) ;
#33681=ORIENTED_EDGE ( 'NONE', *, *, #46762, .F. ) ;
#33682=ORIENTED_EDGE ( 'NONE', *, *, #24409, .F. ) ;
#33683=CARTESIAN_POINT ( 'NONE',  ( -18.72680909822608797, -7.880611277284092608, 70.52068030200462090 ) ) ;
#33687=CARTESIAN_POINT ( 'NONE',  ( -12.49904425988397705, -19.78361547748746219, 61.62352050562626005 ) ) ;
#33689=EDGE_CURVE ( 'NONE', #28462, #42817, #39145, .T. ) ;
#33690=CYLINDRICAL_SURFACE ( 'NONE', #20438, 0.1500000000000015488 ) ;
#33691=CARTESIAN_POINT ( 'NONE',  ( -16.95315630909070848, -7.374056537354511498, 74.06679967459766090 ) ) ;
#33692=B_SPLINE_CURVE_WITH_KNOTS ( 'NONE', 1,
 ( #37049, #22291 ),
 .UNSPECIFIED., .F., .F.,
 ( 2, 2 ),
 ( 0.000000000000000000, 1.000000000000000000 ),
 .UNSPECIFIED. ) ;
#33693=AXIS2_PLACEMENT_3D ( 'NONE', #46965, #16180, #28261 ) ;
#33696=EDGE_LOOP ( 'NONE', ( #5294, #18996, #40802, #5963 ) ) ;
#33698=DIRECTION ( 'NONE',  ( 1.000000000000000000, 0.000000000000000000, 0.000000000000000000 ) ) ;
#33700=DIRECTION ( 'NONE',  ( 0.2466764125338440639, 0.9690979039805150963, -7.162324212090305750E-08 ) ) ;
#33705=DIRECTION ( 'NONE',  ( 0.7915359335728472390, 0.6111226275167354061, 5.146443701300905010E-08 ) ) ;
#33706=EDGE_CURVE ( 'NONE', #6465, #33919, #20394, .T. ) ;
#33707=FACE_OUTER_BOUND ( 'NONE', #37462, .T. ) ;
#33708=CARTESIAN_POINT ( 'NONE',  ( -11.49500183448702906, -10.99442376238782515, 57.22375354680192316 ) ) ;
#33710=( BOUNDED_CURVE ( )  B_SPLINE_CURVE ( 3, ( #30457, #22567, #15649, #26505 ),
 .UNSPECIFIED., .F., .F. ) 
 B_SPLINE_CURVE_WITH_KNOTS ( ( 4, 4 ),
 ( 4.712388980384690562, 4.921828490624009511 ),
 .UNSPECIFIED. ) 
 CURVE ( )  GEOMETRIC_REPRESENTATION_ITEM ( )  RATIONAL_B_SPLINE_CURVE ( ( 1.000000000000000000, 0.9963479302455156006, 0.9963479302455156006, 1.000000000000000000 ) ) 
 REPRESENTATION_ITEM ( '' )  );
#33712=CARTESIAN_POINT ( 'NONE',  ( -13.56393070069739437, -8.909737636684434747, 57.26407933515372406 ) ) ;
#33714=CARTESIAN_POINT ( 'NONE',  ( -14.22441598498101989, -8.081217260141077219, 67.44470407312981308 ) ) ;
#33718=EDGE_CURVE ( 'NONE', #12524, #2153, #450, .T. ) ;
#33720=CARTESIAN_POINT ( 'NONE',  ( -24.65023647254185590, -12.99629722456026393, 63.01759562046499497 ) ) ;
#33721=CARTESIAN_POINT ( 'NONE',  ( -24.36611147337434957, -16.04009697885371111, 66.07797069094537790 ) ) ;
#33722=( BOUNDED_SURFACE ( )  B_SPLINE_SURFACE ( 3, 1, ( 
 ( #33794, #44661 ),
 ( #37484, #21529 ),
 ( #18533, #10675 ),
 ( #3031, #3776 ),
 ( #25217, #36509 ),
 ( #6982, #7242 ),
 ( #10921, #47862 ) ),
 .UNSPECIFIED., .T., .F., .F. ) 
 B_SPLINE_SURFACE_WITH_KNOTS ( ( 4, 3, 4 ),
 ( 2, 2 ),
 ( 0.000000000000000000, 0.5000000000000000000, 1.000000000000000000 ),
 ( 0.000000000000000000, 1.000000000000000000 ),
 .UNSPECIFIED. ) 
 GEOMETRIC_REPRESENTATION_ITEM ( )  RATIONAL_B_SPLINE_SURFACE ( (
 ( 1.000000000000000000, 1.000000000000000000),
 ( 0.3333333333333335369, 0.3333333333333330373),
 ( 0.3333333333333335369, 0.3333333333333330373),
 ( 1.000000000000000000, 1.000000000000000000),
 ( 0.3333333333333333703, 0.3333333333333333703),
 ( 0.3333333333333333703, 0.3333333333333333703),
 ( 1.000000000000000000, 1.000000000000000000) ) ) 
 REPRESENTATION_ITEM ( '' )  SURFACE ( )  );
#33724=( BOUNDED_CURVE ( )  B_SPLINE_CURVE ( 3, ( #13618, #29383, #25680, #44654 ),
 .UNSPECIFIED., .F., .F. ) 
 B_SPLINE_CURVE_WITH_KNOTS ( ( 4, 4 ),
 ( 0.4074455897393692849, 0.5000000000000000000 ),
 .UNSPECIFIED. ) 
 CURVE ( )  GEOMETRIC_REPRESENTATION_ITEM ( )  RATIONAL_B_SPLINE_CURVE ( ( 0.6983129098261070533, 0.7760317562606993125, 0.8765941196519936307, 0.9999999999999824585 ) ) 
 REPRESENTATION_ITEM ( '' )  );
#33725=CARTESIAN_POINT ( 'NONE',  ( -12.25434429315920859, -20.17366997322574562, 65.05170215947674706 ) ) ;
#33727=EDGE_LOOP ( 'NONE', ( #2777, #5275 ) ) ;
#33728=CARTESIAN_POINT ( 'NONE',  ( -19.64401462542318200, -21.92156298671864434, 62.10848288909245696 ) ) ;
#33730=B_SPLINE_CURVE_WITH_KNOTS ( 'NONE', 1,
 ( #18146, #21390 ),
 .UNSPECIFIED., .F., .F.,
 ( 2, 2 ),
 ( 0.000000000000000000, 1.000000000000000000 ),
 .UNSPECIFIED. ) ;
#33731=ORIENTED_EDGE ( 'NONE', *, *, #3935, .F. ) ;
#33735=CARTESIAN_POINT ( 'NONE',  ( -10.35661233123872371, -12.45241144375540365, 60.91358254413026430 ) ) ;
#33738=FACE_OUTER_BOUND ( 'NONE', #6532, .T. ) ;
#33740=PLANE ( 'NONE',  #5425 ) ;
#33743=( BOUNDED_CURVE ( )  B_SPLINE_CURVE ( 3, ( #45649, #569, #4032, #11645 ),
 .UNSPECIFIED., .F., .F. ) 
 B_SPLINE_CURVE_WITH_KNOTS ( ( 4, 4 ),
 ( 4.712388980384690562, 4.921828490624010399 ),
 .UNSPECIFIED. ) 
 CURVE ( )  GEOMETRIC_REPRESENTATION_ITEM ( )  RATIONAL_B_SPLINE_CURVE ( ( 1.000000000000000000, 0.9963479302455154896, 0.9963479302455154896, 1.000000000000000000 ) ) 
 REPRESENTATION_ITEM ( '' )  );
#33745=DIRECTION ( 'NONE',  ( -0.3478314405900307937, -0.9375570856950865561, 0.000000000000000000 ) ) ;
#33746=CARTESIAN_POINT ( 'NONE',  ( -18.26273199447633999, -21.75878827259743886, 65.45418175178663489 ) ) ;
#33747=CARTESIAN_POINT ( 'NONE',  ( -11.90657572125106967, -10.42057778141185231, 70.96893122942475429 ) ) ;
#33750=ORIENTED_EDGE ( 'NONE', *, *, #28959, .T. ) ;
#33752=CARTESIAN_POINT ( 'NONE',  ( -23.99387123153590551, -11.29613222128559258, 66.46568589023691231 ) ) ;
#33753=CARTESIAN_POINT ( 'NONE',  ( -9.975693985146712350, -14.64899972753946145, 71.50595426662775367 ) ) ;
#33757=CARTESIAN_POINT ( 'NONE',  ( -24.20826218283995246, -13.07918557588831376, 66.53076680535011178 ) ) ;
#33760=EDGE_CURVE ( 'NONE', #10444, #42299, #32032, .T. ) ;
#33761=CARTESIAN_POINT ( 'NONE',  ( -12.06214182864563078, -19.98150860846456212, 61.59016925282919885 ) ) ;
#33763=CARTESIAN_POINT ( 'NONE',  ( -13.96821274855622441, -8.721769818545135777, 74.30840771363131125 ) ) ;
#33765=B_SPLINE_CURVE_WITH_KNOTS ( 'NONE', 1,
 ( #14995, #30548 ),
 .UNSPECIFIED., .F., .F.,
 ( 2, 2 ),
 ( 0.000000000000000000, 1.000000000000000000 ),
 .UNSPECIFIED. ) ;
#33766=CARTESIAN_POINT ( 'NONE',  ( -17.11594671439511828, -7.315539529225059567, 47.99999999999994316 ) ) ;
#33768=CARTESIAN_POINT ( 'NONE',  ( -14.25068859620040840, -8.513811488652077486, 70.72957628655862550 ) ) ;
#33771=CARTESIAN_POINT ( 'NONE',  ( -12.08969920365285944, -20.00986870243187710, 61.49655014346812720 ) ) ;
#33772=CARTESIAN_POINT ( 'NONE',  ( -10.66703313327717240, -12.79807994555918960, 64.56836111017611302 ) ) ;
#33773=CARTESIAN_POINT ( 'NONE',  ( -24.30998853687411554, -13.26019858907717897, 66.44679832887018733 ) ) ;
#33774=CARTESIAN_POINT ( 'NONE',  ( -13.93897074462874919, -20.93787812888889377, 68.74153005185598886 ) ) ;
#33777=EDGE_LOOP ( 'NONE', ( #7960, #2442, #19817, #24611, #8786 ) ) ;
#33778=EDGE_LOOP ( 'NONE', ( #7372, #41511, #43646, #36418, #43791 ) ) ;
#33784=CARTESIAN_POINT ( 'NONE',  ( -11.23238687730323626, -11.54381762185194660, 64.25767991630246456 ) ) ;
#33785=CARTESIAN_POINT ( 'NONE',  ( -17.19980177718173309, -7.762775310937220397, 70.49035839668022163 ) ) ;
#33788=EDGE_CURVE ( 'NONE', #4739, #44291, #27642, .T. ) ;
#33789=CARTESIAN_POINT ( 'NONE',  ( -10.98557796499954087, -17.68114198556070349, 71.86718193507100239 ) ) ;
#33790=ORIENTED_EDGE ( 'NONE', *, *, #20870, .F. ) ;
#33791=CARTESIAN_POINT ( 'NONE',  ( -22.32470100883011099, -20.42066193515545791, 62.35722264172714802 ) ) ;
#33793=EDGE_LOOP ( 'NONE', ( #3509, #5550, #34486, #47937, #26278 ) ) ;
#33794=CARTESIAN_POINT ( 'NONE',  ( -19.49109506855409180, -21.54969648977046148, 62.28031529404344013 ) ) ;
#33796=CARTESIAN_POINT ( 'NONE',  ( -9.981760932757149263, -14.47101872614397955, 67.95825874778591924 ) ) ;
#33798=AXIS2_PLACEMENT_3D ( 'NONE', #34659, #27515, #5117 ) ;
#33799=AXIS2_PLACEMENT_3D ( 'NONE', #4942, #34952, #16226 ) ;
#33801=CARTESIAN_POINT ( 'NONE',  ( -24.69856829750257177, -13.20119948815759159, 59.40621968628075678 ) ) ;
#33802=CARTESIAN_POINT ( 'NONE',  ( -21.78444843227217120, -20.35286453386188299, 59.17931667745679647 ) ) ;
#33804=FACE_OUTER_BOUND ( 'NONE', #10638, .T. ) ;
#33807=DIRECTION ( 'NONE',  ( -1.075201462585828720E-05, 1.608194665399622665E-06, 0.9999999999409039386 ) ) ;
#33809=CARTESIAN_POINT ( 'NONE',  ( -17.99534012058598620, -21.78591885189985788, 61.89038380837850184 ) ) ;
#33810=CARTESIAN_POINT ( 'NONE',  ( -23.89575787814031926, -11.11856224597834242, 70.08484892979208780 ) ) ;
#33811=CARTESIAN_POINT ( 'NONE',  ( -10.47914989750023729, -15.69558448425602926, 64.73601526215637136 ) ) ;
#33812=EDGE_CURVE ( 'NONE', #27713, #7442, #17435, .T. ) ;
#33815=EDGE_CURVE ( 'NONE', #42531, #35822, #13314, .T. ) ;
#33816=VERTEX_POINT ( 'NONE', #12853 ) ;
#33817=FACE_OUTER_BOUND ( 'NONE', #19952, .T. ) ;
#33818=CARTESIAN_POINT ( 'NONE',  ( -14.35020019311386719, -8.022098033332648370, 63.90323595109556720 ) ) ;
#33819=ORIENTED_EDGE ( 'NONE', *, *, #30844, .F. ) ;
#33823=DIRECTION ( 'NONE',  ( 0.3478314405900310158, 0.9375570856950865561, 6.371834667863454192E-18 ) ) ;
#33824=B_SPLINE_CURVE_WITH_KNOTS ( 'NONE', 3,
 ( #20437, #1722, #16715, #16950, #20181, #24127, #12306, #43336, #42359, #4684 ),
 .UNSPECIFIED., .F., .F.,
 ( 4, 2, 2, 2, 4 ),
 ( 0.6272669072877878893, 0.7522669073072835166, 0.8772669073267791440, 1.002266907346274660, 1.127266907365770399 ),
 .UNSPECIFIED. ) ;
#33826=CARTESIAN_POINT ( 'NONE',  ( -24.47217469780903798, -14.64471797168181233, 63.01296487297644688 ) ) ;
#33827=CARTESIAN_POINT ( 'NONE',  ( -10.39241571269986331, -17.41794234916963191, 54.27966884056652219 ) ) ;
#33828=ORIENTED_EDGE ( 'NONE', *, *, #2789, .F. ) ;
#33830=( BOUNDED_CURVE ( )  B_SPLINE_CURVE ( 3, ( #11943, #855, #31626, #27434 ),
 .UNSPECIFIED., .F., .F. ) 
 B_SPLINE_CURVE_WITH_KNOTS ( ( 4, 4 ),
 ( 0.4074455897393707282, 0.5000000000000000000 ),
 .UNSPECIFIED. ) 
 CURVE ( )  GEOMETRIC_REPRESENTATION_ITEM ( )  RATIONAL_B_SPLINE_CURVE ( ( 0.6983129098261023904, 0.7760317562606998676, 0.8765941196519971834, 0.9999999999999897859 ) ) 
 REPRESENTATION_ITEM ( '' )  );
#33832=CARTESIAN_POINT ( 'NONE',  ( -14.36817892824948473, -8.455618309860652104, 67.54503025475186462 ) ) ;
#33833=B_SPLINE_CURVE_WITH_KNOTS ( 'NONE', 1,
 ( #42675, #4503 ),
 .UNSPECIFIED., .F., .F.,
 ( 2, 2 ),
 ( 0.000000000000000000, 1.000000000000000000 ),
 .UNSPECIFIED. ) ;
#33835=CARTESIAN_POINT ( 'NONE',  ( -13.51640533490032503, -9.001381809737894812, 57.19640993782574157 ) ) ;
#33836=EDGE_LOOP ( 'NONE', ( #37582, #4753, #22672, #10481, #24777 ) ) ;
#33841=CARTESIAN_POINT ( 'NONE',  ( -23.34117154248328063, -11.06912743251672104, 73.47079241152631823 ) ) ;
#33846=ORIENTED_EDGE ( 'NONE', *, *, #3901, .F. ) ;
#33847=CARTESIAN_POINT ( 'NONE',  ( -15.79261328423922706, -21.67602794760135154, 72.20142491214876657 ) ) ;
#33852=ORIENTED_EDGE ( 'NONE', *, *, #45557, .T. ) ;
#33854=VERTEX_POINT ( 'NONE', #22190 ) ;
#33855=CARTESIAN_POINT ( 'NONE',  ( -12.53168694236654979, -9.190697399280059798, 74.51197142868565493 ) ) ;
#33856=DIRECTION ( 'NONE',  ( -2.699622400625883127E-06, 1.161037828378819543E-05, 0.9999999999289554964 ) ) ;
#33858=CARTESIAN_POINT ( 'NONE',  ( -21.54575282610021247, -21.01526529837170543, 72.71784754957664632 ) ) ;
#33860=ORIENTED_EDGE ( 'NONE', *, *, #25648, .T. ) ;
#33861=CARTESIAN_POINT ( 'NONE',  ( -10.74628672884880309, -17.07053172313825939, 61.17215199736627795 ) ) ;
#33863=CARTESIAN_POINT ( 'NONE',  ( -23.54569140518488624, -19.05536029250058050, 65.93894040291287695 ) ) ;
#33864=CARTESIAN_POINT ( 'NONE',  ( -24.37683854932038585, -15.97618581480151434, 66.21324926630431662 ) ) ;
#33865=EDGE_LOOP ( 'NONE', ( #27721, #19277, #10887, #45893 ) ) ;
#33866=CARTESIAN_POINT ( 'NONE',  ( -19.55370996603141975, -21.94834978302637651, 62.19492417698030806 ) ) ;
#33867=CARTESIAN_POINT ( 'NONE',  ( -18.30602013973305020, -21.80685202924323463, 72.69999788315199396 ) ) ;
#33869=FACE_BOUND ( 'NONE', #37087, .T. ) ;
#33871=AXIS2_PLACEMENT_3D ( 'NONE', #29488, #25795, #36609 ) ;
#33872=EDGE_CURVE ( 'NONE', #34362, #31797, #37043, .T. ) ;
#33873=EDGE_CURVE ( 'NONE', #10223, #34949, #2968, .T. ) ;
#33874=CARTESIAN_POINT ( 'NONE',  ( -16.57554889599778747, -22.21081103083016117, 65.41059783760971413 ) ) ;
#33875=CARTESIAN_POINT ( 'NONE',  ( -10.55057824423783153, -16.13620093359754293, 71.73133888826306759 ) ) ;
#33878=CARTESIAN_POINT ( 'NONE',  ( -12.90354087724769272, -8.887350501024684490, 67.49447389996370816 ) ) ;
#33879=ORIENTED_EDGE ( 'NONE', *, *, #15456, .T. ) ;
#33880=CARTESIAN_POINT ( 'NONE',  ( -11.21157628577468657, -11.58358644131346082, 67.61864608155907774 ) ) ;
#33882=CARTESIAN_POINT ( 'NONE',  ( -12.67437386012394640, -9.069420147667823784, 70.98778821476909684 ) ) ;
#33884=( BOUNDED_CURVE ( )  B_SPLINE_CURVE ( 3, ( #1068, #31108, #16066, #5017 ),
 .UNSPECIFIED., .F., .F. ) 
 B_SPLINE_CURVE_WITH_KNOTS ( ( 4, 4 ),
 ( 0.000000000000000000, 0.4074455897393629011 ),
 .UNSPECIFIED. ) 
 CURVE ( )  GEOMETRIC_REPRESENTATION_ITEM ( )  RATIONAL_B_SPLINE_CURVE ( ( 1.000000000000000000, 0.4567392136813334669, 0.3561768502900308775, 0.6983129098260921763 ) ) 
 REPRESENTATION_ITEM ( '' )  );
#33885=CARTESIAN_POINT ( 'NONE',  ( -14.41574869888453136, -7.993524183322376686, 63.83332938139840707 ) ) ;
#33886=EDGE_LOOP ( 'NONE', ( #5174, #23109, #41783, #39373, #17879 ) ) ;
#33887=CARTESIAN_POINT ( 'NONE',  ( -21.53994948931798703, -21.01915008201228474, 72.78092378945153484 ) ) ;
#33890=EDGE_CURVE ( 'NONE', #9441, #26904, #18642, .T. ) ;
#33892=VERTEX_POINT ( 'NONE', #47566 ) ;
#33894=ORIENTED_EDGE ( 'NONE', *, *, #41120, .F. ) ;
#33895=CARTESIAN_POINT ( 'NONE',  ( -18.37786432726835883, -21.79469297182707521, 69.10042588711679912 ) ) ;
#33896=CARTESIAN_POINT ( 'NONE',  ( -18.12273401612753077, -22.22646211661374593, 65.46036745194116691 ) ) ;
#33898=CARTESIAN_POINT ( 'NONE',  ( -12.50897416063251733, -20.40789074996439112, 72.06299591474957822 ) ) ;
#33899=CARTESIAN_POINT ( 'NONE',  ( -10.58706297158214404, -13.30549792062637593, 74.69434300862685916 ) ) ;
#33901=CARTESIAN_POINT ( 'NONE',  ( -14.03871066829747249, -8.172719617054283958, 70.91452941929576070 ) ) ;
#33902=CARTESIAN_POINT ( 'NONE',  ( -19.28939690137687535, -8.062307696266060475, 59.96092997387292201 ) ) ;
#33903=( BOUNDED_CURVE ( )  B_SPLINE_CURVE ( 3, ( #16210, #31016, #23641, #5404 ),
 .UNSPECIFIED., .F., .F. ) 
 B_SPLINE_CURVE_WITH_KNOTS ( ( 4, 4 ),
 ( 1.570796326794897002, 1.780235837034216617 ),
 .UNSPECIFIED. ) 
 CURVE ( )  GEOMETRIC_REPRESENTATION_ITEM ( )  RATIONAL_B_SPLINE_CURVE ( ( 1.000000000000000000, 0.9963479302455154896, 0.9963479302455154896, 1.000000000000000000 ) ) 
 REPRESENTATION_ITEM ( '' )  );
#33904=ORIENTED_EDGE ( 'NONE', *, *, #20607, .T. ) ;
#33905=ORIENTED_EDGE ( 'NONE', *, *, #7569, .T. ) ;
#33906=CARTESIAN_POINT ( 'NONE',  ( -12.13107248898915635, -10.22829150951328003, 64.31448999593079918 ) ) ;
#33907=EDGE_CURVE ( 'NONE', #10902, #35257, #12729, .T. ) ;
#33909=CARTESIAN_POINT ( 'NONE',  ( -13.92930047287831741, -8.229585886706207276, 74.36101136741100959 ) ) ;
#33910=CYLINDRICAL_SURFACE ( 'NONE', #863, 0.1500000000000059897 ) ;
#33911=CARTESIAN_POINT ( 'NONE',  ( -10.74573065459234478, -12.54952415110468422, 60.81325645027152405 ) ) ;
#33912=VERTEX_POINT ( 'NONE', #3223 ) ;
#33914=EDGE_LOOP ( 'NONE', ( #45010, #41823 ) ) ;
#33916=CARTESIAN_POINT ( 'NONE',  ( -14.80056043599933524, -21.78207186541723317, 61.82095768364339960 ) ) ;
#33917=DIRECTION ( 'NONE',  ( -0.6408936281290997794, -0.7676297007174210929, -4.260501105223894736E-08 ) ) ;
#33918=CARTESIAN_POINT ( 'NONE',  ( -15.78771722930723875, -7.541141403809244359, 67.29007275881872374 ) ) ;
#33919=VERTEX_POINT ( 'NONE', #6679 ) ;
#33920=CARTESIAN_POINT ( 'NONE',  ( -23.46901572703396255, -18.44427995754907457, 69.29371686567111510 ) ) ;
#33922=CARTESIAN_POINT ( 'NONE',  ( -10.95467737376780271, -17.63084047650967889, 64.78306623841410783 ) ) ;
#33923=ORIENTED_EDGE ( 'NONE', *, *, #16982, .T. ) ;
#33925=CARTESIAN_POINT ( 'NONE',  ( -23.91010245674826251, -17.57297063409389537, 62.75888927877479517 ) ) ;
#33926=PLANE ( 'NONE',  #18090 ) ;
#33927=CARTESIAN_POINT ( 'NONE',  ( -19.42896492416523913, -21.56812594671148275, 61.99503644571810668 ) ) ;
#33929=CARTESIAN_POINT ( 'NONE',  ( -24.68106799395027906, -16.49464666695222803, 59.24615566633954700 ) ) ;
#33930=ORIENTED_EDGE ( 'NONE', *, *, #3655, .F. ) ;
#33931=LINE ( 'NONE', #45282, #43110 ) ;
#33932=CARTESIAN_POINT ( 'NONE',  ( -11.55268793888200918, -18.62078556539334073, 64.74707126777444444 ) ) ;
#33934=EDGE_CURVE ( 'NONE', #21199, #36781, #13798, .T. ) ;
#33935=CARTESIAN_POINT ( 'NONE',  ( -12.90227214125716237, -8.888328675545798419, 67.63588728319849963 ) ) ;
#33936=CARTESIAN_POINT ( 'NONE',  ( -24.51735291603774058, -12.52900075589524498, 69.88587656176791540 ) ) ;
#33937=VERTEX_POINT ( 'NONE', #25396 ) ;
#33939=CARTESIAN_POINT ( 'NONE',  ( -23.80321451250838649, -17.81075939459467961, 59.00378417737415049 ) ) ;
#33941=CYLINDRICAL_SURFACE ( 'NONE', #8228, 0.1500000000000035749 ) ;
#33942=EDGE_CURVE ( 'NONE', #13213, #15728, #3459, .T. ) ;
#33943=CARTESIAN_POINT ( 'NONE',  ( -21.76846758817612937, -8.757014937261180521, 70.33143745189734375 ) ) ;
#33944=AXIS2_PLACEMENT_3D ( 'NONE', #39058, #6305, #5594 ) ;
#33945=ORIENTED_EDGE ( 'NONE', *, *, #8908, .F. ) ;
#33946=VERTEX_POINT ( 'NONE', #6451 ) ;
#33947=EDGE_CURVE ( 'NONE', #31415, #28201, #25425, .T. ) ;
#33949=CARTESIAN_POINT ( 'NONE',  ( -10.47299139157196990, -15.63514485490427575, 61.03789045487297926 ) ) ;
#33950=CARTESIAN_POINT ( 'NONE',  ( -11.79630000206883977, -19.05592701419838519, 71.97213747039440079 ) ) ;
#33951=CARTESIAN_POINT ( 'NONE',  ( -23.38417127501956116, -19.28035200660907122, 62.54062256979923973 ) ) ;
#33954=ADVANCED_FACE ( 'NONE', ( #6198 ), #32997, .T. ) ;
#33955=CARTESIAN_POINT ( 'NONE',  ( -10.55500638036946448, -13.20637168857014387, 67.94652154688694168 ) ) ;
#33956=CARTESIAN_POINT ( 'NONE',  ( -11.59906938467913484, -10.16455840884576389, 71.22539037155303276 ) ) ;
#33958=CARTESIAN_POINT ( 'NONE',  ( -9.974987818700082443, -14.92776730449068445, 74.90440581841637879 ) ) ;
#33959=ORIENTED_EDGE ( 'NONE', *, *, #17688, .T. ) ;
#33960=LINE ( 'NONE', #15231, #35185 ) ;
#33962=CARTESIAN_POINT ( 'NONE',  ( -9.975093145215874202, -14.93635225021824198, 74.98274299234972773 ) ) ;
#33963=CARTESIAN_POINT ( 'NONE',  ( -13.59121753182073178, -8.949892528329046471, 60.55023482345360719 ) ) ;
#33964=EDGE_LOOP ( 'NONE', ( #29213, #4621, #32616, #48181, #43138 ) ) ;
#33965=ORIENTED_EDGE ( 'NONE', *, *, #38381, .T. ) ;
#33966=CARTESIAN_POINT ( 'NONE',  ( -19.87909365843526643, -21.36461952118570196, 68.96923927572292712 ) ) ;
#33967=LINE ( 'NONE', #7156, #37852 ) ;
#33969=CARTESIAN_POINT ( 'NONE',  ( -8.621879165042305004, -16.10189953769286575, 53.49999999999995026 ) ) ;
#33971=CARTESIAN_POINT ( 'NONE',  ( -10.96069643151774109, -18.51437482595545347, 57.92219192461608657 ) ) ;
#33972=CARTESIAN_POINT ( 'NONE',  ( -14.35241195940507808, -8.021096776717739019, 67.44630344931481147 ) ) ;
#33974=CARTESIAN_POINT ( 'NONE',  ( -22.80070500595625660, -9.652102806524988310, 73.52515182072782807 ) ) ;
#33975=FACE_OUTER_BOUND ( 'NONE', #46196, .T. ) ;
#33976=CARTESIAN_POINT ( 'NONE',  ( -23.25646303129147441, -19.44570675813884009, 59.07065992548621125 ) ) ;
#33977=ADVANCED_FACE ( 'NONE', ( #36454 ), #36221, .T. ) ;
#33978=EDGE_LOOP ( 'NONE', ( #19895, #20272, #29098, #13100, #36913 ) ) ;
#33979=CARTESIAN_POINT ( 'NONE',  ( -17.47591156279055724, -7.808960447294257534, 67.03656176308530235 ) ) ;
#33981=CARTESIAN_POINT ( 'NONE',  ( -22.82985190038863621, -19.93574988146554006, 72.68754644230530459 ) ) ;
#33982=DIRECTION ( 'NONE',  ( 0.4846961512978548159, 0.8746825943832683414, 4.196010046976494103E-08 ) ) ;
#33984=CARTESIAN_POINT ( 'NONE',  ( -13.47433711440449144, -8.491526086692950059, 57.15623147539552917 ) ) ;
#33985=LINE ( 'NONE', #15260, #10066 ) ;
#33989=CARTESIAN_POINT ( 'NONE',  ( -10.51977190731649614, -16.25273689702515156, 68.18587563686374153 ) ) ;
#33991=VERTEX_POINT ( 'NONE', #19221 ) ;
#33993=CARTESIAN_POINT ( 'NONE',  ( -15.12009195233319936, -21.89411708065309625, 68.69876018860922784 ) ) ;
#33994=CARTESIAN_POINT ( 'NONE',  ( -13.33151401730585306, -20.55006798877650454, 58.06122216312902395 ) ) ;
#33995=CARTESIAN_POINT ( 'NONE',  ( -22.37756982068451705, -20.37394496578614422, 62.34100857704530796 ) ) ;
#33996=CARTESIAN_POINT ( 'NONE',  ( -18.45552443373157914, -21.73280034295336449, 68.92400672263725880 ) ) ;
#33997=CARTESIAN_POINT ( 'NONE',  ( -23.77758468005085390, -18.69975821216192813, 72.95706560366770077 ) ) ;
#33998=ORIENTED_EDGE ( 'NONE', *, *, #13071, .T. ) ;
#33999=ORIENTED_EDGE ( 'NONE', *, *, #39665, .T. ) ;
#34001=CARTESIAN_POINT ( 'NONE',  ( -24.02655244371635845, -11.35792869308308717, 66.53719207489109522 ) ) ;
#34002=CARTESIAN_POINT ( 'NONE',  ( -14.84764829735760649, -8.246537290690364230, 60.33468334944129197 ) ) ;
#34003=EDGE_LOOP ( 'NONE', ( #17437, #11295 ) ) ;
#34004=CARTESIAN_POINT ( 'NONE',  ( -12.84615363328625648, -20.17103110633857455, 72.09181604382622766 ) ) ;
#34005=CARTESIAN_POINT ( 'NONE',  ( -16.31932525666466915, -22.17685042118995398, 61.85593892610445010 ) ) ;
#34006=DIRECTION ( 'NONE',  ( 8.478320013641884810E-07, -8.009068454735622942E-06, 0.9999999999675679430 ) ) ;
#34008=CARTESIAN_POINT ( 'NONE',  ( -17.33515904569749466, -7.808492149107161495, 70.71865624139128670 ) ) ;
#34009=CARTESIAN_POINT ( 'NONE',  ( -21.55686273300884181, -21.00782827186807467, 72.62472190808057348 ) ) ;
#34010=CARTESIAN_POINT ( 'NONE',  ( -23.58616520728616806, -18.99640775243969060, 66.00884813586510802 ) ) ;
#34012=ADVANCED_FACE ( 'NONE', ( #22676 ), #48709, .T. ) ;
#34014=LINE ( 'NONE', #33766, #28871 ) ;
#34017=CARTESIAN_POINT ( 'NONE',  ( -12.11130846069154288, -20.03210741469327871, 61.57395550916974969 ) ) ;
#34018=CARTESIAN_POINT ( 'NONE',  ( -13.90530646979310525, -20.92243618544410921, 65.19448602716460073 ) ) ;
#34021=( BOUNDED_SURFACE ( )  B_SPLINE_SURFACE ( 3, 1, ( 
 ( #25790, #43792 ),
 ( #25071, #7089 ),
 ( #32221, #6355 ),
 ( #47237, #13483 ),
 ( #43554, #21386 ),
 ( #23087, #22849 ),
 ( #15667, #30721 ) ),
 .UNSPECIFIED., .T., .F., .F. ) 
 B_SPLINE_SURFACE_WITH_KNOTS ( ( 4, 3, 4 ),
 ( 2, 2 ),
 ( 0.000000000000000000, 0.5000000000000000000, 1.000000000000000000 ),
 ( 0.000000000000000000, 1.000000000000000000 ),
 .UNSPECIFIED. ) 
 GEOMETRIC_REPRESENTATION_ITEM ( )  RATIONAL_B_SPLINE_SURFACE ( (
 ( 1.000000000000000000, 1.000000000000000000),
 ( 0.3333333333333335369, 0.3333333333333330373),
 ( 0.3333333333333335369, 0.3333333333333330373),
 ( 1.000000000000000000, 1.000000000000000000),
 ( 0.3333333333333333703, 0.3333333333333333703),
 ( 0.3333333333333333703, 0.3333333333333333703),
 ( 1.000000000000000000, 1.000000000000000000) ) ) 
 REPRESENTATION_ITEM ( '' )  SURFACE ( )  );
#34023=EDGE_LOOP ( 'NONE', ( #13852, #10396, #34184, #43830 ) ) ;
#34024=VERTEX_POINT ( 'NONE', #4691 ) ;
#34028=B_SPLINE_CURVE_WITH_KNOTS ( 'NONE', 3,
 ( #5654, #40336, #20664, #21629, #21397, #35659, #31744, #28037, #43061, #16938 ),
 .UNSPECIFIED., .F., .F.,
 ( 4, 2, 2, 2, 4 ),
 ( 0.6272669072877513630, 0.7522669073072717483, 0.8772669073267922446, 1.002266907346312630, 1.127266907365833015 ),
 .UNSPECIFIED. ) ;
#34029=CARTESIAN_POINT ( 'NONE',  ( -10.03904583415351581, -13.82694187778184158, 57.56329747881408565 ) ) ;
#34030=( BOUNDED_CURVE ( )  B_SPLINE_CURVE ( 3, ( #28255, #12747, #24576, #27999 ),
 .UNSPECIFIED., .F., .F. ) 
 B_SPLINE_CURVE_WITH_KNOTS ( ( 4, 4 ),
 ( 0.000000000000000000, 0.4074455897393731707 ),
 .UNSPECIFIED. ) 
 CURVE ( )  GEOMETRIC_REPRESENTATION_ITEM ( )  RATIONAL_B_SPLINE_CURVE ( ( 1.000000000000000000, 0.4567392136813203107, 0.3561768502900259925, 0.6983129098261171563 ) ) 
 REPRESENTATION_ITEM ( '' )  );
#34031=CARTESIAN_POINT ( 'NONE',  ( -13.62591331635612057, -20.69068061466207453, 65.21458850650557793 ) ) ;
#34032=CARTESIAN_POINT ( 'NONE',  ( -16.13987559120563731, -22.14769509179112106, 58.48574339058551885 ) ) ;
#34033=VECTOR ( 'NONE', #45636, 999.9999999999998863 ) ;
#34034=ORIENTED_EDGE ( 'NONE', *, *, #10297, .F. ) ;
#34035=CARTESIAN_POINT ( 'NONE',  ( -15.94958553992630002, -7.506453220755747502, 63.84727885063741581 ) ) ;
#34036=ORIENTED_EDGE ( 'NONE', *, *, #19938, .T. ) ;
#34039=( BOUNDED_SURFACE ( )  B_SPLINE_SURFACE ( 3, 1, ( 
 ( #29392, #33060 ),
 ( #6745, #14818 ),
 ( #26190, #21759 ),
 ( #36745, #48103 ),
 ( #3521, #44424 ),
 ( #7488, #40708 ),
 ( #22003, #37001 ) ),
 .UNSPECIFIED., .T., .F., .F. ) 
 B_SPLINE_SURFACE_WITH_KNOTS ( ( 4, 3, 4 ),
 ( 2, 2 ),
 ( 0.000000000000000000, 0.5000000000000000000, 1.000000000000000000 ),
 ( 0.000000000000000000, 1.000000000000000000 ),
 .UNSPECIFIED. ) 
 GEOMETRIC_REPRESENTATION_ITEM ( )  RATIONAL_B_SPLINE_SURFACE ( (
 ( 1.000000000000000000, 1.000000000000000000),
 ( 0.3333333333333335369, 0.3333333333333330373),
 ( 0.3333333333333335369, 0.3333333333333330373),
 ( 1.000000000000000000, 1.000000000000000000),
 ( 0.3333333333333333703, 0.3333333333333333703),
 ( 0.3333333333333333703, 0.3333333333333333703),
 ( 1.000000000000000000, 1.000000000000000000) ) ) 
 REPRESENTATION_ITEM ( '' )  SURFACE ( )  );
#34041=DIRECTION ( 'NONE',  ( -0.7847243476406476903, -0.6198448985189423110, 4.433022207822355740E-08 ) ) ;
#34042=CARTESIAN_POINT ( 'NONE',  ( -14.07761835836965858, -20.95746660330474143, 72.22607703844037985 ) ) ;
#34043=CARTESIAN_POINT ( 'NONE',  ( -22.44685545595405785, -12.53547801027385766, 53.69233794759168887 ) ) ;
#34044=ORIENTED_EDGE ( 'NONE', *, *, #43383, .F. ) ;
#34045=CARTESIAN_POINT ( 'NONE',  ( -23.25757785049868787, -10.17517560731475967, 63.18690593950643120 ) ) ;
#34046=FACE_OUTER_BOUND ( 'NONE', #45738, .T. ) ;
#34048=CARTESIAN_POINT ( 'NONE',  ( -24.51865387586880729, -12.53305138704347144, 73.42880879726919829 ) ) ;
#34049=ORIENTED_EDGE ( 'NONE', *, *, #17824, .T. ) ;
#34050=CARTESIAN_POINT ( 'NONE',  ( -11.75774095458083224, -19.00383931511213120, 71.68685884783836570 ) ) ;
#34051=CARTESIAN_POINT ( 'NONE',  ( -10.98602742111231478, -11.93616459261413354, 74.85840217524429363 ) ) ;
#34052=EDGE_CURVE ( 'NONE', #21243, #15104, #45280, .T. ) ;
#34054=CARTESIAN_POINT ( 'NONE',  ( -10.38078067960954520, -14.50222210708341741, 68.15800126083217947 ) ) ;
#34055=CARTESIAN_POINT ( 'NONE',  ( -20.81696448553514855, -20.93198605141084201, 62.41471400679856885 ) ) ;
#34058=ORIENTED_EDGE ( 'NONE', *, *, #32912, .T. ) ;
#34059=ADVANCED_FACE ( 'NONE', ( #4213 ), #45099, .T. ) ;
#34060=CARTESIAN_POINT ( 'NONE',  ( -24.68398957063837074, -13.13362340124566785, 63.01919566578877152 ) ) ;
#34061=CARTESIAN_POINT ( 'NONE',  ( -17.15134030326023051, -7.364115279526828317, 70.67531275522621570 ) ) ;
#34062=VERTEX_POINT ( 'NONE', #11586 ) ;
#34063=B_SPLINE_CURVE_WITH_KNOTS ( 'NONE', 1,
 ( #27236, #8524 ),
 .UNSPECIFIED., .F., .F.,
 ( 2, 2 ),
 ( 0.000000000000000000, 1.000000000000000000 ),
 .UNSPECIFIED. ) ;
#34064=CARTESIAN_POINT ( 'NONE',  ( -18.44824984440512594, -7.884471009248593454, 74.12598989606129862 ) ) ;
#34065=CARTESIAN_POINT ( 'NONE',  ( -24.45777360974264170, -14.27930545299182619, 73.21451642246609026 ) ) ;
#34066=CARTESIAN_POINT ( 'NONE',  ( -24.33254494401252188, -16.21558397985894473, 62.59888500697857694 ) ) ;
#34067=ORIENTED_EDGE ( 'NONE', *, *, #22323, .F. ) ;
#34068=CARTESIAN_POINT ( 'NONE',  ( -14.78754716229542687, -8.270772359302402066, 60.31996282000579157 ) ) ;
#34069=CARTESIAN_POINT ( 'NONE',  ( -10.03804196927290882, -15.78895246822652076, 64.69426957934942379 ) ) ;
#34071=CARTESIAN_POINT ( 'NONE',  ( -10.67174945191680813, -12.96329562009371550, 67.73832382197451807 ) ) ;
#34072=ORIENTED_EDGE ( 'NONE', *, *, #15513, .T. ) ;
#34075=EDGE_CURVE ( 'NONE', #3502, #19604, #11612, .T. ) ;
#34077=DIRECTION ( 'NONE',  ( -5.731567514496413899E-31, -1.020425574103664789E-16, -1.000000000000000000 ) ) ;
#34078=CARTESIAN_POINT ( 'NONE',  ( -17.26457240846633923, -7.760713630915982542, 70.50507891880883449 ) ) ;
#34079=CARTESIAN_POINT ( 'NONE',  ( -13.59468179584094472, -8.949401161162814589, 56.96967704137573207 ) ) ;
#34080=ORIENTED_EDGE ( 'NONE', *, *, #13785, .T. ) ;
#34081=VERTEX_POINT ( 'NONE', #512 ) ;
#34084=CARTESIAN_POINT ( 'NONE',  ( -20.13271805750754595, -8.299978134201072777, 70.53628287813307907 ) ) ;
#34087=EDGE_CURVE ( 'NONE', #32823, #1260, #14906, .T. ) ;
#34089=CARTESIAN_POINT ( 'NONE',  ( -14.97035482569482312, -21.41873484682592377, 61.92128389535452015 ) ) ;
#34091=FACE_OUTER_BOUND ( 'NONE', #45464, .T. ) ;
#34092=DIRECTION ( 'NONE',  ( 0.9087012777736581670, -0.4174469879787381932, -4.853707507795077342E-09 ) ) ;
#34093=CARTESIAN_POINT ( 'NONE',  ( -13.60236376389480384, -20.73382277062339085, 61.80174179654961364 ) ) ;
#34095=CARTESIAN_POINT ( 'NONE',  ( -23.03651554467916185, -18.99332579461250603, 62.37023563316526520 ) ) ;
#34096=EDGE_LOOP ( 'NONE', ( #36396, #2852, #34339, #18181 ) ) ;
#34097=CARTESIAN_POINT ( 'NONE',  ( -24.06787342886325121, -18.28917680027896608, 53.49999999999994316 ) ) ;
#34100=CARTESIAN_POINT ( 'NONE',  ( -14.19282086353638661, -8.542981675383003903, 71.01485553001869278 ) ) ;
#34101=AXIS2_PLACEMENT_3D ( 'NONE', #1850, #6021, #47399 ) ;
#34103=CARTESIAN_POINT ( 'NONE',  ( -10.35515617550548306, -17.16373074020370737, 61.34398415755805445 ) ) ;
#34104=CARTESIAN_POINT ( 'NONE',  ( -24.03160980685186487, -17.26750534774173929, 69.41339792588559021 ) ) ;
#34105=CARTESIAN_POINT ( 'NONE',  ( -13.15570000409499229, -9.198020586789933617, 67.38502599777598334 ) ) ;
#34107=VERTEX_POINT ( 'NONE', #11348 ) ;
#34108=FACE_BOUND ( 'NONE', #37151, .T. ) ;
#34109=CARTESIAN_POINT ( 'NONE',  ( -17.15134030326023051, -7.364115279526828317, 70.67531275522621570 ) ) ;
#34111=FACE_BOUND ( 'NONE', #18411, .T. ) ;
#34113=B_SPLINE_CURVE_WITH_KNOTS ( 'NONE', 1,
 ( #29648, #33557 ),
 .UNSPECIFIED., .F., .F.,
 ( 2, 2 ),
 ( 0.000000000000000000, 1.000000000000000000 ),
 .UNSPECIFIED. ) ;
#34114=EDGE_LOOP ( 'NONE', ( #1375, #37666, #13992, #27776, #28696 ) ) ;
#34115=CARTESIAN_POINT ( 'NONE',  ( -10.72530867274958233, -17.00760959713300480, 57.97288447305808745 ) ) ;
#34117=CARTESIAN_POINT ( 'NONE',  ( -23.54569203310520464, -19.05535937789667145, 65.93894149164137275 ) ) ;
#34118=FACE_OUTER_BOUND ( 'NONE', #29337, .T. ) ;
#34119=ORIENTED_EDGE ( 'NONE', *, *, #1837, .T. ) ;
#34120=DIRECTION ( 'NONE',  ( 0.1571515419521612722, -0.9875744999047174622, 7.433889655140131751E-08 ) ) ;
#34122=CARTESIAN_POINT ( 'NONE',  ( -12.28110100360571444, -10.05819353197068722, 64.21841333961458531 ) ) ;
#34124=CARTESIAN_POINT ( 'NONE',  ( -14.99706828511980916, -21.85287925006270626, 65.29092110561946072 ) ) ;
#34125=VERTEX_POINT ( 'NONE', #32428 ) ;
#34126=CARTESIAN_POINT ( 'NONE',  ( -13.41327373486474883, -20.54621981236622830, 58.04650078084816300 ) ) ;
#34128=ORIENTED_EDGE ( 'NONE', *, *, #15946, .F. ) ;
#34129=ORIENTED_EDGE ( 'NONE', *, *, #22863, .T. ) ;
#34131=CARTESIAN_POINT ( 'NONE',  ( -15.40811923343076906, -21.56513327689926030, 72.06047564147742435 ) ) ;
#34132=B_SPLINE_CURVE_WITH_KNOTS ( 'NONE', 3,
 ( #5727, #43142, #9665, #17262, #13319, #43397, #24679, #39683, #20973, #32305 ),
 .UNSPECIFIED., .F., .F.,
 ( 4, 2, 2, 2, 4 ),
 ( 0.1272669073658627692, 0.2522669073463418843, 0.3772669073268209994, 0.5022669073073000590, 0.6272669072877792296 ),
 .UNSPECIFIED. ) ;
#34133=LINE ( 'NONE', #3369, #26521 ) ;
#34134=CARTESIAN_POINT ( 'NONE',  ( -12.64201450438284624, -19.99346662158319887, 72.22142341168820678 ) ) ;
#34135=DIRECTION ( 'NONE',  ( 1.684279440454093594E-06, -5.535644408139047379E-06, 0.9999999999832598352 ) ) ;
#34136=CARTESIAN_POINT ( 'NONE',  ( -10.37588343406238067, -17.22313626567787992, 61.33555868484288709 ) ) ;
#34138=DIRECTION ( 'NONE',  ( -0.3478314405900310713, -0.9375570856950864451, 0.000000000000000000 ) ) ;
#34139=ORIENTED_EDGE ( 'NONE', *, *, #17312, .F. ) ;
#34140=ORIENTED_EDGE ( 'NONE', *, *, #31494, .F. ) ;
#34141=VECTOR ( 'NONE', #19247, 1000.000000000000227 ) ;
#34142=CARTESIAN_POINT ( 'NONE',  ( -17.92858306677455715, -7.769287621248931686, 63.69489771833700331 ) ) ;
#34143=CARTESIAN_POINT ( 'NONE',  ( -11.85153772408746065, -9.864590794909398497, 64.22925524624133686 ) ) ;
#34144=FACE_OUTER_BOUND ( 'NONE', #3680, .T. ) ;
#34145=CARTESIAN_POINT ( 'NONE',  ( -19.63983784775455987, -21.44940190450812167, 65.46486191127920051 ) ) ;
#34148=ADVANCED_FACE ( 'NONE', ( #47449 ), #6321, .F. ) ;
#34150=EDGE_CURVE ( 'NONE', #6133, #43308, #8754, .T. ) ;
#34151=EDGE_CURVE ( 'NONE', #38159, #36571, #8448, .T. ) ;
#34152=LINE ( 'NONE', #4609, #21738 ) ;
#34153=CARTESIAN_POINT ( 'NONE',  ( -12.22456126456390280, -19.57467567670336450, 61.81167242413056329 ) ) ;
#34154=DIRECTION ( 'NONE',  ( -1.259531062706796257E-05, 2.755480462148206820E-06, -0.9999999999168825981 ) ) ;
#34155=ORIENTED_EDGE ( 'NONE', *, *, #16484, .T. ) ;
#34156=CARTESIAN_POINT ( 'NONE',  ( -10.61330258792943226, -12.98832159324075874, 68.03832347271723791 ) ) ;
#34157=CARTESIAN_POINT ( 'NONE',  ( -11.21783165637758550, -18.93062460193366192, 64.93202459354702683 ) ) ;
#34158=ORIENTED_EDGE ( 'NONE', *, *, #48193, .T. ) ;
#34159=CARTESIAN_POINT ( 'NONE',  ( -10.43949455435184603, -13.84896052950683476, 57.46297163929641982 ) ) ;
#34160=( BOUNDED_CURVE ( )  B_SPLINE_CURVE ( 3, ( #46620, #31830, #1793, #15388 ),
 .UNSPECIFIED., .F., .F. ) 
 B_SPLINE_CURVE_WITH_KNOTS ( ( 4, 4 ),
 ( 0.000000000000000000, 0.4074455897393616244 ),
 .UNSPECIFIED. ) 
 CURVE ( )  GEOMETRIC_REPRESENTATION_ITEM ( )  RATIONAL_B_SPLINE_CURVE ( ( 1.000000000000000000, 0.4567392136813359094, 0.3561768502900317657, 0.6983129098260875134 ) ) 
 REPRESENTATION_ITEM ( '' )  );
#34161=CARTESIAN_POINT ( 'NONE',  ( -10.04821616988549593, -15.85811384580076933, 64.62276300976363075 ) ) ;
#34163=VERTEX_POINT ( 'NONE', #16482 ) ;
#34164=CARTESIAN_POINT ( 'NONE',  ( -11.18189852286175956, -11.63857423012741421, 71.31690716596565949 ) ) ;
#34165=ORIENTED_EDGE ( 'NONE', *, *, #14225, .F. ) ;
#34167=CARTESIAN_POINT ( 'NONE',  ( -10.16786014542261007, -13.12079378898483384, 71.25182636653194379 ) ) ;
#34168=CARTESIAN_POINT ( 'NONE',  ( -14.80072874354800305, -7.836285926156586257, 56.89354091526551116 ) ) ;
#34171=EDGE_CURVE ( 'NONE', #6304, #30207, #17582, .T. ) ;
#34172=AXIS2_PLACEMENT_3D ( 'NONE', #10878, #44876, #40200 ) ;
#34173=CARTESIAN_POINT ( 'NONE',  ( -11.08846142298070880, -18.82290330472913098, 54.27966884056657904 ) ) ;
#34175=FACE_OUTER_BOUND ( 'NONE', #16817, .T. ) ;
#34176=CARTESIAN_POINT ( 'NONE',  ( -10.63004074901718532, -12.92571453866564823, 67.75304464120749515 ) ) ;
#34177=PLANE ( 'NONE',  #10176 ) ;
#34178=VERTEX_POINT ( 'NONE', #38660 ) ;
#34179=CARTESIAN_POINT ( 'NONE',  ( -19.17551097150447603, -8.031399452544897954, 63.71472721929436034 ) ) ;
#34180=( BOUNDED_CURVE ( )  B_SPLINE_CURVE ( 3, ( #42331, #8604, #23867, #34433 ),
 .UNSPECIFIED., .F., .F. ) 
 B_SPLINE_CURVE_WITH_KNOTS ( ( 4, 4 ),
 ( 0.5000000000000000000, 0.9074455897393601811 ),
 .UNSPECIFIED. ) 
 CURVE ( )  GEOMETRIC_REPRESENTATION_ITEM ( )  RATIONAL_B_SPLINE_CURVE ( ( 1.000000000000003331, 0.4567392136813360204, 0.3561768502900293232, 0.6983129098260867362 ) ) 
 REPRESENTATION_ITEM ( '' )  );
#34181=CARTESIAN_POINT ( 'NONE',  ( -13.19964055691519533, -20.45787379516043814, 58.13830346053801890 ) ) ;
#34182=ADVANCED_FACE ( 'NONE', ( #13683 ), #1540, .T. ) ;
#34183=EDGE_LOOP ( 'NONE', ( #4532, #36812, #26613, #12841, #48671 ) ) ;
#34184=ORIENTED_EDGE ( 'NONE', *, *, #31100, .F. ) ;
#34185=CARTESIAN_POINT ( 'NONE',  ( -21.91034708787274710, -20.18261625685872218, 59.06442899735736773 ) ) ;
#34188=PLANE ( 'NONE',  #845 ) ;
#34191=CARTESIAN_POINT ( 'NONE',  ( -12.01932494161596487, -10.27783711031607261, 71.38381879606350822 ) ) ;
#34192=CARTESIAN_POINT ( 'NONE',  ( -23.12302852889637350, -18.95946475466559633, 62.65406880579606508 ) ) ;
#34193=CARTESIAN_POINT ( 'NONE',  ( -12.38096385557255807, -9.882601854136318309, 57.38375773230528409 ) ) ;
#34194=ORIENTED_EDGE ( 'NONE', *, *, #25081, .F. ) ;
#34195=CARTESIAN_POINT ( 'NONE',  ( -10.40888601095206134, -14.10966482229656194, 61.21821293885882653 ) ) ;
#34196=CARTESIAN_POINT ( 'NONE',  ( -10.37541943412130863, -14.96049300415475614, 75.08306784598362071 ) ) ;
#34198=ORIENTED_EDGE ( 'NONE', *, *, #42756, .T. ) ;
#34200=EDGE_LOOP ( 'NONE', ( #844, #920 ) ) ;
#34202=CARTESIAN_POINT ( 'NONE',  ( -19.85890256509918572, -21.37233786973231275, 68.95612130754568625 ) ) ;
#34203=CARTESIAN_POINT ( 'NONE',  ( -10.61357223164714902, -13.19155561173493219, 71.20828586568362084 ) ) ;
#34204=B_SPLINE_CURVE_WITH_KNOTS ( 'NONE', 3,
 ( #13362, #32574, #43678, #10180, #21507, #40443, #28410, #36718, #5765, #20770 ),
 .UNSPECIFIED., .F., .F.,
 ( 4, 2, 2, 2, 4 ),
 ( 0.000000000000000000, 0.2500000000000000000, 0.5000000000000000000, 0.7500000000000000000, 1.000000000000000000 ),
 .UNSPECIFIED. ) ;
#34205=CARTESIAN_POINT ( 'NONE',  ( -11.71852041784209497, -10.01868235693899933, 67.59922621222234795 ) ) ;
#34207=EDGE_LOOP ( 'NONE', ( #30681, #9460, #39673, #36159, #47464 ) ) ;
#34209=EDGE_CURVE ( 'NONE', #18111, #11672, #19953, .T. ) ;
#34210=ADVANCED_FACE ( 'NONE', ( #47681 ), #16637, .T. ) ;
#34211=CARTESIAN_POINT ( 'NONE',  ( -14.28913779072144230, -8.050817036395716997, 67.37479760520351135 ) ) ;
#34212=VERTEX_POINT ( 'NONE', #42619 ) ;
#34213=ADVANCED_FACE ( 'NONE', ( #8878 ), #21676, .T. ) ;
#34214=CARTESIAN_POINT ( 'NONE',  ( -22.92319755143357085, -10.39759026177046763, 63.37185995336191979 ) ) ;
#34215=EDGE_CURVE ( 'NONE', #39854, #11424, #3855, .T. ) ;
#34216=CARTESIAN_POINT ( 'NONE',  ( -23.64508914155128139, -11.49223708805166311, 66.72214503450521761 ) ) ;
#34217=VERTEX_POINT ( 'NONE', #44252 ) ;
#34218=CARTESIAN_POINT ( 'NONE',  ( -11.65643154663995595, -18.86968838501740109, 64.95526796013899684 ) ) ;
#34219=VERTEX_POINT ( 'NONE', #15145 ) ;
#34221=B_SPLINE_CURVE_WITH_KNOTS ( 'NONE', 3,
 ( #40389, #47776, #10118, #28594, #14016, #9878, #17247, #29067, #29309, #24896 ),
 .UNSPECIFIED., .F., .F.,
 ( 4, 2, 2, 2, 4 ),
 ( 0.6272669072878390706, 0.7522669073073260382, 0.8772669073268131168, 1.002266907346299973, 1.127266907365787052 ),
 .UNSPECIFIED. ) ;
#34222=CARTESIAN_POINT ( 'NONE',  ( -20.40573040493966772, -8.475905570818413892, 63.53794860803412092 ) ) ;
#34224=DIRECTION ( 'NONE',  ( 0.7300417127692488961, 0.6834025882427879894, 6.612978994660554254E-09 ) ) ;
#34226=EDGE_CURVE ( 'NONE', #20348, #13463, #6739, .T. ) ;
#34228=CARTESIAN_POINT ( 'NONE',  ( -22.66727108289645543, -10.09628893573625064, 70.01178520457129650 ) ) ;
#34229=CARTESIAN_POINT ( 'NONE',  ( -19.17247957453286844, -7.567181637230756763, 63.61584517348745038 ) ) ;
#34232=CARTESIAN_POINT ( 'NONE',  ( -15.22116837037893866, -21.50650591823945845, 68.59065000974109694 ) ) ;
#34233=DIRECTION ( 'NONE',  ( -5.731567514496413899E-31, -1.020425574103664789E-16, -1.000000000000000000 ) ) ;
#34236=CARTESIAN_POINT ( 'NONE',  ( -24.63822977646513834, -12.69227384653554047, 54.02312124697525064 ) ) ;
#34237=CARTESIAN_POINT ( 'NONE',  ( -16.06904075904983031, -7.890656793283918446, 63.97011029956862416 ) ) ;
#34238=ORIENTED_EDGE ( 'NONE', *, *, #39179, .T. ) ;
#34239=ORIENTED_EDGE ( 'NONE', *, *, #15939, .T. ) ;
#34240=CARTESIAN_POINT ( 'NONE',  ( -24.49361813620984663, -12.45866096502549603, 73.43563874794485002 ) ) ;
#34241=CARTESIAN_POINT ( 'NONE',  ( -14.73594855369633905, -7.860282982240396343, 60.50651534380390473 ) ) ;
#34242=VERTEX_POINT ( 'NONE', #10737 ) ;
#34243=CARTESIAN_POINT ( 'NONE',  ( -12.83178440107774065, -20.15853244757020590, 72.10093902957984824 ) ) ;
#34244=CARTESIAN_POINT ( 'NONE',  ( -15.75283589881223278, -7.548994832054173543, 67.32502661251716347 ) ) ;
#34246=CARTESIAN_POINT ( 'NONE',  ( -13.90805003106573068, -20.86209311441256986, 68.75625137331327608 ) ) ;
#34247=B_SPLINE_CURVE_WITH_KNOTS ( 'NONE', 1,
 ( #28456, #24992 ),
 .UNSPECIFIED., .F., .F.,
 ( 2, 2 ),
 ( 0.000000000000000000, 1.000000000000000000 ),
 .UNSPECIFIED. ) ;
#34248=CARTESIAN_POINT ( 'NONE',  ( -12.05615918852498680, -19.97535170061420828, 61.51183199568394144 ) ) ;
#34249=CARTESIAN_POINT ( 'NONE',  ( -18.50162202296811742, -21.72577595440482057, 72.28510940981611554 ) ) ;
#34250=CARTESIAN_POINT ( 'NONE',  ( -20.34472269902922292, -8.388554739717058339, 63.31121412747268096 ) ) ;
#34254=CARTESIAN_POINT ( 'NONE',  ( -10.51205449915416068, -13.40259651842557531, 71.20828329199629536 ) ) ;
#34255=( BOUNDED_CURVE ( )  B_SPLINE_CURVE ( 3, ( #35769, #13359, #10174, #17298 ),
 .UNSPECIFIED., .F., .F. ) 
 B_SPLINE_CURVE_WITH_KNOTS ( ( 4, 4 ),
 ( 0.5000000000000000000, 0.9074455897393680637 ),
 .UNSPECIFIED. ) 
 CURVE ( )  GEOMETRIC_REPRESENTATION_ITEM ( )  RATIONAL_B_SPLINE_CURVE ( ( 1.000000000000016653, 0.4567392136813376302, 0.3561768502900207745, 0.6983129098260839607 ) ) 
 REPRESENTATION_ITEM ( '' )  );
#34256=CARTESIAN_POINT ( 'NONE',  ( -13.90804716676048258, -20.86209139562971160, 68.45625137333186672 ) ) ;
#34261=EDGE_LOOP ( 'NONE', ( #10078, #27334, #3014, #36430, #19 ) ) ;
#34266=CARTESIAN_POINT ( 'NONE',  ( -16.47526054104836746, -21.74466271362331682, 61.77070513569444188 ) ) ;
#34267=VECTOR ( 'NONE', #31373, 1000.000000000000000 ) ;
#34268=CARTESIAN_POINT ( 'NONE',  ( -13.34343926350448584, -8.575967577738570213, 57.13001076993559479 ) ) ;
#34269=CARTESIAN_POINT ( 'NONE',  ( -16.77411572588129118, -21.83219480353551134, 72.58031927177887610 ) ) ;
#34270=ORIENTED_EDGE ( 'NONE', *, *, #36550, .F. ) ;
#34271=EDGE_CURVE ( 'NONE', #1779, #12574, #46077, .T. ) ;
#34272=CARTESIAN_POINT ( 'NONE',  ( -13.83248983650026709, -21.33638410845934885, 72.18253639678975730 ) ) ;
#34273=CARTESIAN_POINT ( 'NONE',  ( -17.55282127470103504, -7.360150197541120320, 63.71090416642158516 ) ) ;
#34274=EDGE_CURVE ( 'NONE', #2663, #25694, #41027, .T. ) ;
#34276=CARTESIAN_POINT ( 'NONE',  ( -11.96084830514426400, -9.743959610980004626, 60.74413522332266524 ) ) ;
#34277=B_SPLINE_CURVE_WITH_KNOTS ( 'NONE', 1,
 ( #38477, #19048 ),
 .UNSPECIFIED., .F., .F.,
 ( 2, 2 ),
 ( 0.000000000000000000, 1.000000000000000000 ),
 .UNSPECIFIED. ) ;
#34278=CARTESIAN_POINT ( 'NONE',  ( -10.37497030826117417, -14.69804335084345759, 71.32782692816427073 ) ) ;
#34279=ORIENTED_EDGE ( 'NONE', *, *, #27008, .T. ) ;
#34281=CARTESIAN_POINT ( 'NONE',  ( -24.47498361611929596, -14.63661054434306763, 59.12811639263489383 ) ) ;
#34282=CARTESIAN_POINT ( 'NONE',  ( -21.36420383812641077, -21.13211724076752773, 69.31096130815059553 ) ) ;
#34283=CARTESIAN_POINT ( 'NONE',  ( -17.85261197751258067, -25.23011165689956670, 54.58422952202461431 ) ) ;
#34284=VERTEX_POINT ( 'NONE', #37302 ) ;
#34285=CARTESIAN_POINT ( 'NONE',  ( -23.20384594580217552, -10.10819856274111039, 63.23219334867470565 ) ) ;
#34286=LINE ( 'NONE', #8215, #24978 ) ;
#34287=EDGE_CURVE ( 'NONE', #16467, #46532, #42105, .T. ) ;
#34288=CARTESIAN_POINT ( 'NONE',  ( -14.54176566789882585, -21.67913831930545854, 58.28122448549703449 ) ) ;
#34289=CARTESIAN_POINT ( 'NONE',  ( -21.06702863216100141, -20.84540773593991148, 65.86981821684420879 ) ) ;
#34291=CARTESIAN_POINT ( 'NONE',  ( -15.75283589881223278, -7.548994832054173543, 67.32502661251716347 ) ) ;
#34294=DIRECTION ( 'NONE',  ( 1.190035119058586791E-06, 1.172070126139376962E-06, 0.9999999999986050048 ) ) ;
#34298=CARTESIAN_POINT ( 'NONE',  ( -24.05059659118241555, -17.06519001246171996, 72.88336032079776317 ) ) ;
#34299=ORIENTED_EDGE ( 'NONE', *, *, #15208, .F. ) ;
#34300=CYLINDRICAL_SURFACE ( 'NONE', #44183, 0.1499999999999992173 ) ;
#34301=CARTESIAN_POINT ( 'NONE',  ( -22.98865682493615381, -9.855478938366896813, 70.12683207277369490 ) ) ;
#34302=CARTESIAN_POINT ( 'NONE',  ( -14.60831023476407786, -21.21965601727942996, 58.35544853774701579 ) ) ;
#34303=( BOUNDED_CURVE ( )  B_SPLINE_CURVE ( 3, ( #48347, #3298, #18545, #18297 ),
 .UNSPECIFIED., .F., .F. ) 
 B_SPLINE_CURVE_WITH_KNOTS ( ( 4, 4 ),
 ( 1.570796326794896558, 1.780235837034217727 ),
 .UNSPECIFIED. ) 
 CURVE ( )  GEOMETRIC_REPRESENTATION_ITEM ( )  RATIONAL_B_SPLINE_CURVE ( ( 1.000000000000000000, 0.9963479302455154896, 0.9963479302455154896, 1.000000000000000000 ) ) 
 REPRESENTATION_ITEM ( '' )  );
#34304=EDGE_LOOP ( 'NONE', ( #22337, #3656, #1486, #46421, #36645 ) ) ;
#34305=CARTESIAN_POINT ( 'NONE',  ( -18.39951258112534305, -22.19516185762106275, 69.00009993223443416 ) ) ;
#34308=CARTESIAN_POINT ( 'NONE',  ( -23.47609061619699844, -18.32690069530191579, 72.83656187062067033 ) ) ;
#34313=EDGE_CURVE ( 'NONE', #17093, #33155, #1399, .T. ) ;
#34314=CARTESIAN_POINT ( 'NONE',  ( -14.09575362490740602, -8.143965183153959231, 70.83683468466919919 ) ) ;
#34315=CARTESIAN_POINT ( 'NONE',  ( -13.50402399543905929, -9.009805505539487669, 57.16070831537086860 ) ) ;
#34316=B_SPLINE_CURVE_WITH_KNOTS ( 'NONE', 3,
 ( #35658, #1938, #23879, #38882, #31743, #5160, #24841, #35177, #46763, #16937 ),
 .UNSPECIFIED., .F., .F.,
 ( 4, 2, 2, 2, 4 ),
 ( 0.000000000000000000, 0.2500000000000000000, 0.5000000000000000000, 0.7500000000000000000, 1.000000000000000000 ),
 .UNSPECIFIED. ) ;
#34317=( BOUNDED_CURVE ( )  B_SPLINE_CURVE ( 3, ( #28991, #32683, #13475, #13223 ),
 .UNSPECIFIED., .F., .F. ) 
 B_SPLINE_CURVE_WITH_KNOTS ( ( 4, 4 ),
 ( 0.5000000000000000000, 0.9074455897393649551 ),
 .UNSPECIFIED. ) 
 CURVE ( )  GEOMETRIC_REPRESENTATION_ITEM ( )  RATIONAL_B_SPLINE_CURVE ( ( 1.000000000000004441, 0.4567392136813354098, 0.3561768502900284350, 0.6983129098260884016 ) ) 
 REPRESENTATION_ITEM ( '' )  );
#34318=ORIENTED_EDGE ( 'NONE', *, *, #14465, .F. ) ;
#34321=CARTESIAN_POINT ( 'NONE',  ( -22.99375746295947209, -9.861153455744265273, 70.13461618218333626 ) ) ;
#34322=CARTESIAN_POINT ( 'NONE',  ( -23.81024829756716343, -18.64597716098235836, 72.94863620959463901 ) ) ;
#34324=( BOUNDED_CURVE ( )  B_SPLINE_CURVE ( 3, ( #17852, #28953, #6312, #32874 ),
 .UNSPECIFIED., .F., .F. ) 
 B_SPLINE_CURVE_WITH_KNOTS ( ( 4, 4 ),
 ( 0.5000000000000000000, 0.9074455897393627346 ),
 .UNSPECIFIED. ) 
 CURVE ( )  GEOMETRIC_REPRESENTATION_ITEM ( )  RATIONAL_B_SPLINE_CURVE ( ( 1.000000000000033973, 0.4567392136813449577, 0.3561768502900111155, 0.6983129098260696388 ) ) 
 REPRESENTATION_ITEM ( '' )  );
#34326=CARTESIAN_POINT ( 'NONE',  ( -20.48833060507423909, -8.513735687714852673, 66.89177111435644463 ) ) ;
#34328=CARTESIAN_POINT ( 'NONE',  ( -9.982647249627337516, -14.45068338159927990, 68.11446040317247252 ) ) ;
#34330=EDGE_CURVE ( 'NONE', #28874, #44341, #10828, .T. ) ;
#34334=ADVANCED_FACE ( 'NONE', ( #8768 ), #30476, .T. ) ;
#34335=CARTESIAN_POINT ( 'NONE',  ( -13.00647906721701297, -9.304695462141918227, 64.06513368409466125 ) ) ;
#34336=CARTESIAN_POINT ( 'NONE',  ( -9.974999579213063683, -14.92872621805817879, 74.99053041033617717 ) ) ;
#34337=CARTESIAN_POINT ( 'NONE',  ( -12.57425161569036653, -9.153915111069411026, 74.42648864573870071 ) ) ;
#34338=CARTESIAN_POINT ( 'NONE',  ( -13.27770465421436619, -9.107456272842560097, 64.20946529204060482 ) ) ;
#34339=ORIENTED_EDGE ( 'NONE', *, *, #6886, .T. ) ;
#34340=CARTESIAN_POINT ( 'NONE',  ( -10.74573065459234478, -12.54952415110468422, 60.81325645027152405 ) ) ;
#34341=CARTESIAN_POINT ( 'NONE',  ( -10.78031428196279329, -11.32923628920978487, 47.99999999999994316 ) ) ;
#34344=CARTESIAN_POINT ( 'NONE',  ( -10.32984062102020850, -12.53399622812623448, 60.95886941719668073 ) ) ;
#34346=ORIENTED_EDGE ( 'NONE', *, *, #8322, .F. ) ;
#34347=DIRECTION ( 'NONE',  ( -0.3739781583979218671, -0.9274375111247652459, -6.296758467538797382E-09 ) ) ;
#34350=FACE_BOUND ( 'NONE', #16665, .T. ) ;
#34351=ORIENTED_EDGE ( 'NONE', *, *, #44845, .F. ) ;
#34352=CARTESIAN_POINT ( 'NONE',  ( -22.17032154447610282, -19.95442984834653188, 62.34325199807766182 ) ) ;
#34353=CARTESIAN_POINT ( 'NONE',  ( -18.11889201384288128, -21.82488578508536747, 65.34532159284481168 ) ) ;
#34354=CARTESIAN_POINT ( 'NONE',  ( -23.50612575731066656, -19.11299006986292071, 66.01044822673141255 ) ) ;
#34355=CARTESIAN_POINT ( 'NONE',  ( -15.73993337224566247, -7.955115359200574332, 63.82577855974437853 ) ) ;
#34356=ORIENTED_EDGE ( 'NONE', *, *, #31434, .F. ) ;
#34358=VERTEX_POINT ( 'NONE', #15885 ) ;
#34359=PLANE ( 'NONE',  #25038 ) ;
#34360=CARTESIAN_POINT ( 'NONE',  ( -20.03282965983824226, -21.84088468745754597, 77.49999999999994316 ) ) ;
#34361=ADVANCED_FACE ( 'NONE', ( #15382 ), #4335, .T. ) ;
#34362=VERTEX_POINT ( 'NONE', #38047 ) ;
#34364=CARTESIAN_POINT ( 'NONE',  ( -23.07130679197163659, -10.58859284808890422, 59.60763246093404177 ) ) ;
#34368=ORIENTED_EDGE ( 'NONE', *, *, #36048, .T. ) ;
#34369=CARTESIAN_POINT ( 'NONE',  ( -20.63628304827270199, -8.086446354347476273, 66.96759359044023086 ) ) ;
#34371=CARTESIAN_POINT ( 'NONE',  ( -21.21817610565444667, -20.69187580328668119, 69.33984775460822902 ) ) ;
#34372=CARTESIAN_POINT ( 'NONE',  ( -15.56465948913147557, -7.543361525925788236, 54.27966884056655061 ) ) ;
#34373=CARTESIAN_POINT ( 'NONE',  ( -24.13123319531394273, -12.80563922725783144, 66.49349849057904294 ) ) ;
#34374=CARTESIAN_POINT ( 'NONE',  ( -12.68381388925888587, -19.95990997655619381, 68.63657438305759229 ) ) ;
#34375=CARTESIAN_POINT ( 'NONE',  ( -22.37499513144005903, -19.83249348569362880, 73.05889139438880875 ) ) ;
#34377=AXIS2_PLACEMENT_3D ( 'NONE', #26181, #19511, #325 ) ;
#34378=ORIENTED_EDGE ( 'NONE', *, *, #16423, .T. ) ;
#34379=ORIENTED_EDGE ( 'NONE', *, *, #43969, .F. ) ;
#34380=CARTESIAN_POINT ( 'NONE',  ( -12.15425132636677219, -10.20155252404504331, 64.02914322084043874 ) ) ;
#34381=CARTESIAN_POINT ( 'NONE',  ( -14.09463846823036981, -8.088735815341543400, 53.49999999999994316 ) ) ;
#34382=FACE_OUTER_BOUND ( 'NONE', #37105, .T. ) ;
#34385=ORIENTED_EDGE ( 'NONE', *, *, #33812, .T. ) ;
#34387=EDGE_LOOP ( 'NONE', ( #21751, #13646, #22000, #5689, #30556 ) ) ;
#34388=CARTESIAN_POINT ( 'NONE',  ( -11.75774308769439003, -19.00384223356172697, 71.98685884781657762 ) ) ;
#34389=CARTESIAN_POINT ( 'NONE',  ( -10.50429924535250414, -16.15944446069506668, 71.46222527016213633 ) ) ;
#34390=CARTESIAN_POINT ( 'NONE',  ( -10.40511033146429831, -14.11732416830307280, 57.33336190745325212 ) ) ;
#34391=ORIENTED_EDGE ( 'NONE', *, *, #44535, .F. ) ;
#34393=PLANE ( 'NONE',  #13839 ) ;
#34394=CARTESIAN_POINT ( 'NONE',  ( -24.17607580446128068, -11.66038665607651836, 59.60422999760712059 ) ) ;
#34396=EDGE_LOOP ( 'NONE', ( #14726, #44619 ) ) ;
#34397=CARTESIAN_POINT ( 'NONE',  ( -24.47368665962210343, -14.70950332193510590, 62.72768537250228604 ) ) ;
#34401=CARTESIAN_POINT ( 'NONE',  ( -11.15769924256992951, -11.68856090084249999, 71.37244301326146001 ) ) ;
#34402=AXIS2_PLACEMENT_3D ( 'NONE', #21412, #36877, #17201 ) ;
#34404=ORIENTED_EDGE ( 'NONE', *, *, #41291, .T. ) ;
#34405=CARTESIAN_POINT ( 'NONE',  ( -10.16749015965427105, -13.12235144340169235, 71.39323866028058774 ) ) ;
#34406=CARTESIAN_POINT ( 'NONE',  ( -24.38111619087839799, -15.96880572012975286, 62.47839786477943136 ) ) ;
#34408=DIRECTION ( 'NONE',  ( -0.9998756790481366785, -0.01576789294826319923, -3.907472230461692677E-09 ) ) ;
#34409=CARTESIAN_POINT ( 'NONE',  ( -24.53780083649505173, -12.59584922708229904, 69.95738295622972203 ) ) ;
#34410=LINE ( 'NONE', #12503, #39129 ) ;
#34411=EDGE_LOOP ( 'NONE', ( #9330, #30127, #9995, #10133, #23316 ) ) ;
#34412=DIRECTION ( 'NONE',  ( -0.1186632576870824130, 0.9929345553837299887, 6.051931679537041823E-08 ) ) ;
#34413=AXIS2_PLACEMENT_3D ( 'NONE', #44921, #15322, #19042 ) ;
#34414=CARTESIAN_POINT ( 'NONE',  ( -10.67239429020883890, -12.76729606296974140, 68.03832549181448996 ) ) ;
#34415=CARTESIAN_POINT ( 'NONE',  ( -10.93882906647579922, -17.44414160026099125, 68.39721938813583790 ) ) ;
#34416=ORIENTED_EDGE ( 'NONE', *, *, #33265, .F. ) ;
#34419=CARTESIAN_POINT ( 'NONE',  ( -23.58390325158506329, -11.37972522600045089, 69.89770551021980793 ) ) ;
#34421=ADVANCED_FACE ( 'NONE', ( #24753 ), #16917, .T. ) ;
#34424=ORIENTED_EDGE ( 'NONE', *, *, #12866, .F. ) ;
#34427=FACE_OUTER_BOUND ( 'NONE', #42534, .T. ) ;
#34429=CARTESIAN_POINT ( 'NONE',  ( -10.55421158500719336, -13.20934456994658035, 67.73832145363171264 ) ) ;
#34430=B_SPLINE_CURVE_WITH_KNOTS ( 'NONE', 3,
 ( #8872, #35670, #16474, #39134, #34718, #1953, #1461, #43076, #47010, #38653 ),
 .UNSPECIFIED., .F., .F.,
 ( 4, 2, 2, 2, 4 ),
 ( 0.000000000000000000, 0.2500000000000000000, 0.5000000000000000000, 0.7500000000000000000, 1.000000000000000000 ),
 .UNSPECIFIED. ) ;
#34433=CARTESIAN_POINT ( 'NONE',  ( -23.80321479583337307, -17.81075880182941873, 59.30378417737342289 ) ) ;
#34434=ORIENTED_EDGE ( 'NONE', *, *, #31105, .T. ) ;
#34435=CARTESIAN_POINT ( 'NONE',  ( -22.89412281574421471, -9.750308782327882895, 70.12523226502652562 ) ) ;
#34436=SHAPE_REPRESENTATION_RELATIONSHIP ( 'NONE' , 'NONE' ,  #22625, #23202 ) ;
#34438=CARTESIAN_POINT ( 'NONE',  ( -24.53575672594257995, -12.58916661682799898, 69.89430231120414305 ) ) ;
#34439=CARTESIAN_POINT ( 'NONE',  ( -21.90064967531214890, -9.427635609301674435, 60.00705870275116638 ) ) ;
#34443=AXIS2_PLACEMENT_3D ( 'NONE', #20861, #21108, #13691 ) ;
#34444=VERTEX_POINT ( 'NONE', #1603 ) ;
#34445=EDGE_CURVE ( 'NONE', #41130, #14380, #33139, .T. ) ;
#34446=CARTESIAN_POINT ( 'NONE',  ( -21.41863048803932656, -8.999699081277377388, 73.61600897546567523 ) ) ;
#34448=CARTESIAN_POINT ( 'NONE',  ( -13.29262146975105274, -21.00882449603590985, 61.69459112368684117 ) ) ;
#34449=CARTESIAN_POINT ( 'NONE',  ( -10.17310289001843948, -13.09872099292910264, 71.40817355644446707 ) ) ;
#34451=B_SPLINE_CURVE_WITH_KNOTS ( 'NONE', 3,
 ( #44792, #22368, #26306, #25814, #19401, #22615, #37613, #48457, #11046, #225 ),
 .UNSPECIFIED., .F., .F.,
 ( 4, 2, 2, 2, 4 ),
 ( 0.1272669073658194150, 0.2522669073463100209, 0.3772669073268006823, 0.5022669073072912882, 0.6272669072877818941 ),
 .UNSPECIFIED. ) ;
#34454=CARTESIAN_POINT ( 'NONE',  ( -20.17037934351568751, -8.316057459223078041, 70.55100343557511167 ) ) ;
#34455=CARTESIAN_POINT ( 'NONE',  ( -13.46025101761997078, -8.974705932511858109, 64.00126803586600488 ) ) ;
#34456=ORIENTED_EDGE ( 'NONE', *, *, #39390, .F. ) ;
#34457=EDGE_CURVE ( 'NONE', #24815, #25854, #28445, .T. ) ;
#34458=CARTESIAN_POINT ( 'NONE',  ( -12.94403785604389867, -20.18778427150672883, 71.91539741676557185 ) ) ;
#34459=B_SPLINE_CURVE_WITH_KNOTS ( 'NONE', 3,
 ( #1903, #43526, #9305, #35626, #16906, #8831, #31943, #24804, #39813, #46957 ),
 .UNSPECIFIED., .F., .F.,
 ( 4, 2, 2, 2, 4 ),
 ( 0.000000000000000000, 0.2500000000000000000, 0.5000000000000000000, 0.7500000000000000000, 1.000000000000000000 ),
 .UNSPECIFIED. ) ;
#34461=CARTESIAN_POINT ( 'NONE',  ( -21.77428020737724523, -9.323007506576582060, 66.77223141407961293 ) ) ;
#34462=( BOUNDED_CURVE ( )  B_SPLINE_CURVE ( 3, ( #1634, #20602, #35599, #21568 ),
 .UNSPECIFIED., .F., .F. ) 
 B_SPLINE_CURVE_WITH_KNOTS ( ( 4, 4 ),
 ( 0.4074455897393726156, 0.5000000000000000000 ),
 .UNSPECIFIED. ) 
 CURVE ( )  GEOMETRIC_REPRESENTATION_ITEM ( )  RATIONAL_B_SPLINE_CURVE ( ( 0.6983129098261142698, 0.7760317562607251807, 0.8765941196520231626, 1.000000000000013989 ) ) 
 REPRESENTATION_ITEM ( '' )  );
#34463=ORIENTED_EDGE ( 'NONE', *, *, #30232, .T. ) ;
#34464=CARTESIAN_POINT ( 'NONE',  ( -24.53780051168580911, -12.59584816521350348, 69.95738404390658616 ) ) ;
#34465=CARTESIAN_POINT ( 'NONE',  ( -11.10300763040008398, -10.86615618544839457, 57.39398486019972268 ) ) ;
#34466=B_SPLINE_CURVE_WITH_KNOTS ( 'NONE', 3,
 ( #29320, #40397, #33223, #18219, #21688, #17969, #21924, #25615, #40628, #36928 ),
 .UNSPECIFIED., .F., .F.,
 ( 4, 2, 2, 2, 4 ),
 ( 0.1272669073658077854, 0.2522669073439209875, 0.3772669073220341618, 0.5022669073001474471, 0.6272669072782606214 ),
 .UNSPECIFIED. ) ;
#34467=ORIENTED_EDGE ( 'NONE', *, *, #7017, .T. ) ;
#34474=CARTESIAN_POINT ( 'NONE',  ( -21.70399976399352937, -9.206932529385648323, 66.66150014529212342 ) ) ;
#34476=CARTESIAN_POINT ( 'NONE',  ( -19.22579309969192707, -21.57336792462666253, 58.52507384993226225 ) ) ;
#34480=DIRECTION ( 'NONE',  ( 0.3636930986378154040, 0.9315188296557533887, -1.850371886801397658E-09 ) ) ;
#34481=CYLINDRICAL_SURFACE ( 'NONE', #44777, 0.1499999999999998002 ) ;
#34483=EDGE_CURVE ( 'NONE', #1731, #10912, #35475, .T. ) ;
#34484=ADVANCED_FACE ( 'NONE', ( #24027 ), #2330, .T. ) ;
#34485=ORIENTED_EDGE ( 'NONE', *, *, #18102, .T. ) ;
#34486=ORIENTED_EDGE ( 'NONE', *, *, #6952, .T. ) ;
#34487=CYLINDRICAL_SURFACE ( 'NONE', #14084, 0.1500000000000054068 ) ;
#34489=ORIENTED_EDGE ( 'NONE', *, *, #7793, .F. ) ;
#34490=CARTESIAN_POINT ( 'NONE',  ( -21.05967961157278268, -21.31196033385931443, 62.30745545902120597 ) ) ;
#34491=CARTESIAN_POINT ( 'NONE',  ( -15.12736151640637416, -21.89643440865206614, 68.69097607374993686 ) ) ;
#34495=CARTESIAN_POINT ( 'NONE',  ( -14.12328906776938631, -8.570644558479624919, 67.41542347112275024 ) ) ;
#34496=CARTESIAN_POINT ( 'NONE',  ( -10.86088752666615065, -11.28245350497684818, 67.80519939327926693 ) ) ;
#34497=LINE ( 'NONE', #22964, #30298 ) ;
#34498=B_SPLINE_CURVE_WITH_KNOTS ( 'NONE', 3,
 ( #21670, #10109, #32743, #36425, #2939, #2703, #36909, #40148, #25369, #36658 ),
 .UNSPECIFIED., .F., .F.,
 ( 4, 2, 2, 2, 4 ),
 ( 0.000000000000000000, 0.2500000000000000000, 0.5000000000000000000, 0.7500000000000000000, 1.000000000000000000 ),
 .UNSPECIFIED. ) ;
#34499=VERTEX_POINT ( 'NONE', #21046 ) ;
#34500=ADVANCED_FACE ( 'NONE', ( #35806 ), #2083, .T. ) ;
#34502=CARTESIAN_POINT ( 'NONE',  ( -22.50076973789108692, -19.70108052134635557, 72.64400543415067091 ) ) ;
#34503=CARTESIAN_POINT ( 'NONE',  ( -11.56046518335400286, -10.21343137625755482, 71.16167249782886017 ) ) ;
#34504=EDGE_CURVE ( 'NONE', #48202, #33991, #47140, .T. ) ;
#34505=CARTESIAN_POINT ( 'NONE',  ( -13.90805003106573068, -20.86209311441256986, 68.75625137331327608 ) ) ;
#34506=CARTESIAN_POINT ( 'NONE',  ( -12.80044327789678249, -20.06500310223181671, 71.80653684543825932 ) ) ;
#34507=CARTESIAN_POINT ( 'NONE',  ( -18.12432747636454877, -22.22630431188652977, 65.60178084401016463 ) ) ;
#34508=EDGE_LOOP ( 'NONE', ( #7958, #39789 ) ) ;
#34510=CARTESIAN_POINT ( 'NONE',  ( -20.04849592361258104, -21.35284569240296548, 72.69006679631316103 ) ) ;
#34511=VERTEX_POINT ( 'NONE', #13394 ) ;
#34512=EDGE_CURVE ( 'NONE', #12297, #29684, #26719, .T. ) ;
#34513=CARTESIAN_POINT ( 'NONE',  ( -12.01952932525029816, -9.681273877180114340, 60.69884694392221292 ) ) ;
#34515=CARTESIAN_POINT ( 'NONE',  ( -10.02995829593802668, -13.89786868041111667, 57.63320316755233819 ) ) ;
#34518=LINE ( 'NONE', #1517, #12485 ) ;
#34519=CARTESIAN_POINT ( 'NONE',  ( -11.30361347545239958, -11.41219030243732391, 64.14882039658046153 ) ) ;
#34520=CARTESIAN_POINT ( 'NONE',  ( -17.31415506352089650, -21.86632207739205569, 72.32110344861041540 ) ) ;
#34521=ORIENTED_EDGE ( 'NONE', *, *, #36383, .T. ) ;
#34522=CARTESIAN_POINT ( 'NONE',  ( -14.34827028450108344, -21.16170790896200060, 72.08174668229233362 ) ) ;
#34524=CARTESIAN_POINT ( 'NONE',  ( -19.67760665824181388, -21.48965406232008490, 65.75014118398131302 ) ) ;
#34526=CARTESIAN_POINT ( 'NONE',  ( -11.36856108582972702, -11.29517246406753195, 64.22052367023555064 ) ) ;
#34529=CARTESIAN_POINT ( 'NONE',  ( -16.84865286310842336, -21.83598151670433296, 68.98088545748413480 ) ) ;
#34530=DIRECTION ( 'NONE',  ( -0.04086606279947146980, -0.9938001236776475844, 0.1033986416233891037 ) ) ;
#34532=CARTESIAN_POINT ( 'NONE',  ( -23.20845821660187980, -10.11394778068016898, 63.19373217977586421 ) ) ;
#34533=CARTESIAN_POINT ( 'NONE',  ( -24.09286991228532315, -11.48796221018129238, 63.05879980478538727 ) ) ;
#34534=CARTESIAN_POINT ( 'NONE',  ( -18.35897211656709160, -21.79709577657633446, 69.10954899396081430 ) ) ;
#34535=CARTESIAN_POINT ( 'NONE',  ( -24.21281492007539526, -12.87834259335418530, 73.38658464541695992 ) ) ;
#34537=CARTESIAN_POINT ( 'NONE',  ( -12.23220206747518013, -19.57856285391799034, 58.22682373937799838 ) ) ;
#34538=CARTESIAN_POINT ( 'NONE',  ( -22.33041777183100507, -20.41561037748852669, 62.34943743628787161 ) ) ;
#34543=EDGE_CURVE ( 'NONE', #47823, #46955, #40505, .T. ) ;
#34547=CARTESIAN_POINT ( 'NONE',  ( -24.28028284729623465, -16.22112348152082362, 59.19620387435347197 ) ) ;
#34548=ORIENTED_EDGE ( 'NONE', *, *, #47400, .F. ) ;
#34549=DIRECTION ( 'NONE',  ( 0.9710973231077276724, -0.2386838684389877008, 7.431671637556431570E-08 ) ) ;
#34551=CARTESIAN_POINT ( 'NONE',  ( -23.24167040808332985, -10.15534690731836065, 63.27197199642595393 ) ) ;
#34552=CARTESIAN_POINT ( 'NONE',  ( -14.74690658000796439, -21.27702444416618732, 58.16617884968206198 ) ) ;
#34553=ORIENTED_EDGE ( 'NONE', *, *, #28959, .F. ) ;
#34554=CARTESIAN_POINT ( 'NONE',  ( -17.04978450098071718, -7.769001547375945727, 73.96578056985927674 ) ) ;
#34555=AXIS2_PLACEMENT_3D ( 'NONE', #33379, #45479, #7074 ) ;
#34556=CARTESIAN_POINT ( 'NONE',  ( -15.28291166272248169, -21.52618791248891128, 68.87592918174580348 ) ) ;
#34557=EDGE_CURVE ( 'NONE', #22030, #17855, #27234, .T. ) ;
#34558=CARTESIAN_POINT ( 'NONE',  ( -12.05749060505181269, -9.640721912800795934, 60.74573338552316670 ) ) ;
#34559=VERTEX_POINT ( 'NONE', #47873 ) ;
#34560=CARTESIAN_POINT ( 'NONE',  ( -18.60622205832422082, -22.16490843864383109, 72.47006330605313451 ) ) ;
#34561=ADVANCED_FACE ( 'NONE', ( #21539 ), #6994, .T. ) ;
#34562=VECTOR ( 'NONE', #17343, 1000.000000000000227 ) ;
#34565=CARTESIAN_POINT ( 'NONE',  ( -10.01440776720603765, -14.03439672543145988, 61.03325998023760235 ) ) ;
#34566=DIRECTION ( 'NONE',  ( 1.389773841562029912E-07, 3.718553644687884925E-07, -0.9999999999999211742 ) ) ;
#34567=CARTESIAN_POINT ( 'NONE',  ( -13.24129617563109740, -8.644154241298165786, 60.69596227262822907 ) ) ;
#34569=VERTEX_POINT ( 'NONE', #40970 ) ;
#34571=CARTESIAN_POINT ( 'NONE',  ( -24.40026719341414108, -15.82783281859430780, 69.53867305742785732 ) ) ;
#34572=CARTESIAN_POINT ( 'NONE',  ( -23.39840055413978348, -11.16100488844999994, 73.36193259119190202 ) ) ;
#34573=CARTESIAN_POINT ( 'NONE',  ( -11.46044050272623416, -11.04924139602722377, 57.20903212151935691 ) ) ;
#34574=CARTESIAN_POINT ( 'NONE',  ( -10.76542905790024385, -16.97361952088028758, 61.26816177302506361 ) ) ;
#34579=VERTEX_POINT ( 'NONE', #36520 ) ;
#34580=CARTESIAN_POINT ( 'NONE',  ( -21.89953879547803695, -8.853196296446007807, 66.70504049802050872 ) ) ;
#34581=AXIS2_PLACEMENT_3D ( 'NONE', #13417, #32157, #44226 ) ;
#34583=B_SPLINE_CURVE_WITH_KNOTS ( 'NONE', 1,
 ( #25318, #7090 ),
 .UNSPECIFIED., .F., .F.,
 ( 2, 2 ),
 ( 0.000000000000000000, 1.000000000000000000 ),
 .UNSPECIFIED. ) ;
#34586=PLANE ( 'NONE',  #19475 ) ;
#34587=CARTESIAN_POINT ( 'NONE',  ( -12.10131192688100299, -10.18592936015514816, 64.31442259820508411 ) ) ;
#34589=ORIENTED_EDGE ( 'NONE', *, *, #45271, .T. ) ;
#34590=CARTESIAN_POINT ( 'NONE',  ( -22.58065782673598676, -12.89613362149922438, 54.07175714974875547 ) ) ;
#34592=( BOUNDED_CURVE ( )  B_SPLINE_CURVE ( 3, ( #16932, #13001, #43315, #1932 ),
 .UNSPECIFIED., .F., .F. ) 
 B_SPLINE_CURVE_WITH_KNOTS ( ( 4, 4 ),
 ( 0.4074455897393606807, 0.5000000000000000000 ),
 .UNSPECIFIED. ) 
 CURVE ( )  GEOMETRIC_REPRESENTATION_ITEM ( )  RATIONAL_B_SPLINE_CURVE ( ( 0.6983129098260772993, 0.7760317562606969810, 0.8765941196520082856, 1.000000000000019762 ) ) 
 REPRESENTATION_ITEM ( '' )  );
#34593=ADVANCED_FACE ( 'NONE', ( #10685 ), #44436, .T. ) ;
#34594=CARTESIAN_POINT ( 'NONE',  ( -21.73099075187129614, -8.730192115828774746, 70.31627817507801126 ) ) ;
#34595=CARTESIAN_POINT ( 'NONE',  ( -20.90213356920466126, -8.220891710688713161, 59.94101618556534561 ) ) ;
#34596=VERTEX_POINT ( 'NONE', #3043 ) ;
#34597=CARTESIAN_POINT ( 'NONE',  ( -10.33743488275009526, -17.10781281734085724, 57.80947783183761146 ) ) ;
#34599=CARTESIAN_POINT ( 'NONE',  ( -23.81024772113315890, -18.64597811008791695, 72.94863512192290500 ) ) ;
#34600=CARTESIAN_POINT ( 'NONE',  ( -19.52100072682865672, -19.90831991051152627, 53.88362224778185805 ) ) ;
#34602=CARTESIAN_POINT ( 'NONE',  ( -22.81278634540432648, -10.26332246522033032, 66.54182271920811331 ) ) ;
#34603=CARTESIAN_POINT ( 'NONE',  ( -14.51638892016982219, -21.23572161159003713, 58.46617851441119029 ) ) ;
#34604=EDGE_LOOP ( 'NONE', ( #15471, #13684, #22161, #19549, #43122 ) ) ;
#34605=DIRECTION ( 'NONE',  ( -6.471065199890530885E-06, -1.909039593073236381E-06, 0.9999999999772404280 ) ) ;
#34606=ORIENTED_EDGE ( 'NONE', *, *, #19074, .T. ) ;
#34607=CARTESIAN_POINT ( 'NONE',  ( -22.79734292848665334, -10.24514101169484270, 66.84182257473257494 ) ) ;
#34608=CARTESIAN_POINT ( 'NONE',  ( -13.18108784799495936, -9.241582085570342997, 67.67942828295852564 ) ) ;
#34609=ORIENTED_EDGE ( 'NONE', *, *, #34982, .T. ) ;
#34610=( BOUNDED_CURVE ( )  B_SPLINE_CURVE ( 3, ( #36246, #9198, #39953, #9444 ),
 .UNSPECIFIED., .F., .F. ) 
 B_SPLINE_CURVE_WITH_KNOTS ( ( 4, 4 ),
 ( 0.4074455897393677306, 0.5000000000000000000 ),
 .UNSPECIFIED. ) 
 CURVE ( )  GEOMETRIC_REPRESENTATION_ITEM ( )  RATIONAL_B_SPLINE_CURVE ( ( 0.6983129098261039447, 0.7760317562607236264, 0.8765941196520269374, 1.000000000000025313 ) ) 
 REPRESENTATION_ITEM ( '' )  );
#34611=CARTESIAN_POINT ( 'NONE',  ( -24.71334378318632830, -13.26952680650525274, 59.47772536435775947 ) ) ;
#34612=FACE_BOUND ( 'NONE', #35969, .T. ) ;
#34613=VERTEX_POINT ( 'NONE', #29159 ) ;
#34614=ORIENTED_EDGE ( 'NONE', *, *, #46523, .T. ) ;
#34616=ADVANCED_FACE ( 'NONE', ( #2805 ), #7254, .T. ) ;
#34618=CARTESIAN_POINT ( 'NONE',  ( -10.46291082975850806, -15.97406517396614944, 61.19356052171543325 ) ) ;
#34619=AXIS2_PLACEMENT_3D ( 'NONE', #10922, #4031, #45389 ) ;
#34621=ADVANCED_FACE ( 'NONE', ( #29401 ), #48594, .T. ) ;
#34622=CARTESIAN_POINT ( 'NONE',  ( -24.34138173484705803, -16.17068648017255583, 62.59328676670276792 ) ) ;
#34623=CARTESIAN_POINT ( 'NONE',  ( -17.43166586245951422, -7.359124596637800053, 67.13544155391683432 ) ) ;
#34624=CARTESIAN_POINT ( 'NONE',  ( -11.81636632494307015, -9.904339708471926684, 64.15101585200166312 ) ) ;
#34625=CARTESIAN_POINT ( 'NONE',  ( -19.41839014062696123, -8.097970103967929489, 60.18922903702627281 ) ) ;
#34627=( BOUNDED_CURVE ( )  B_SPLINE_CURVE ( 3, ( #24498, #32588, #32113, #17559 ),
 .UNSPECIFIED., .F., .F. ) 
 B_SPLINE_CURVE_WITH_KNOTS ( ( 4, 4 ),
 ( 0.9074455897393698400, 1.000000000000000000 ),
 .UNSPECIFIED. ) 
 CURVE ( )  GEOMETRIC_REPRESENTATION_ITEM ( )  RATIONAL_B_SPLINE_CURVE ( ( 0.6983129098261089407, 0.7760317562607119690, 0.8765941196520089518, 1.000000000000000000 ) ) 
 REPRESENTATION_ITEM ( '' )  );
#34628=EDGE_LOOP ( 'NONE', ( #19474, #31028, #33017, #9686, #47839 ) ) ;
#34629=ORIENTED_EDGE ( 'NONE', *, *, #11857, .T. ) ;
#34632=CARTESIAN_POINT ( 'NONE',  ( -13.76849323099554567, -20.83774554052356009, 65.27156739751333703 ) ) ;
#34633=DIRECTION ( 'NONE',  ( -0.9501515917649785425, -0.3117883138709295898, 1.594035198720926202E-08 ) ) ;
#34635=CARTESIAN_POINT ( 'NONE',  ( -19.74220741432039716, -21.41423112065765011, 65.57372225646707875 ) ) ;
#34640=VERTEX_POINT ( 'NONE', #6518 ) ;
#34641=DIRECTION ( 'NONE',  ( -0.9774082387306984865, 0.2113602016968848529, -7.903122840838824810E-08 ) ) ;
#34642=CARTESIAN_POINT ( 'NONE',  ( -15.33758281339130036, -21.49113659546963362, 68.87592903483572115 ) ) ;
#34643=VECTOR ( 'NONE', #7606, 1000.000000000000000 ) ;
#34644=B_SPLINE_CURVE_WITH_KNOTS ( 'NONE', 1,
 ( #3149, #7352 ),
 .UNSPECIFIED., .F., .F.,
 ( 2, 2 ),
 ( 0.000000000000000000, 1.000000000000000000 ),
 .UNSPECIFIED. ) ;
#34645=CARTESIAN_POINT ( 'NONE',  ( -12.44661342226983969, -19.73288402143430886, 64.93845064584576221 ) ) ;
#34647=CARTESIAN_POINT ( 'NONE',  ( -23.34481426128875015, -18.63642081788813343, 69.29371984264746231 ) ) ;
#34649=CARTESIAN_POINT ( 'NONE',  ( -10.44881520703817479, -17.42631679175528703, 64.74244059074541724 ) ) ;
#34651=AXIS2_PLACEMENT_3D ( 'NONE', #5302, #38045, #35328 ) ;
#34653=CARTESIAN_POINT ( 'NONE',  ( -21.68499601416157674, -9.192516039336664946, 66.66149992327366647 ) ) ;
#34654=EDGE_CURVE ( 'NONE', #47654, #46361, #35511, .T. ) ;
#34655=CARTESIAN_POINT ( 'NONE',  ( -22.96484172783137012, -19.08706962207428504, 58.88410642316259214 ) ) ;
#34657=ORIENTED_EDGE ( 'NONE', *, *, #39803, .T. ) ;
#34658=B_SPLINE_CURVE_WITH_KNOTS ( 'NONE', 3,
 ( #37072, #22558, #26251, #29956, #3105, #3858, #18863, #30209, #11474, #26498 ),
 .UNSPECIFIED., .F., .F.,
 ( 4, 2, 2, 2, 4 ),
 ( 0.1272669073658397321, 0.2522669073463245093, 0.3772669073268092310, 0.5022669073072940638, 0.6272669072877787855 ),
 .UNSPECIFIED. ) ;
#34659=CARTESIAN_POINT ( 'NONE',  ( -22.51043027204183034, -20.25270558619591910, 65.85421731173748583 ) ) ;
#34661=VERTEX_POINT ( 'NONE', #26199 ) ;
#34662=FACE_OUTER_BOUND ( 'NONE', #31874, .T. ) ;
#34664=CARTESIAN_POINT ( 'NONE',  ( -14.79922921121938195, -7.836842249070715916, 57.03495322699122738 ) ) ;
#34665=VERTEX_POINT ( 'NONE', #37247 ) ;
#34666=CARTESIAN_POINT ( 'NONE',  ( -16.36675962830097930, -22.18387328577503581, 61.79922180027413958 ) ) ;
#34667=CARTESIAN_POINT ( 'NONE',  ( -23.84761967927745374, -12.02338244726358596, 59.67162711403931752 ) ) ;
#34670=CARTESIAN_POINT ( 'NONE',  ( -9.995124286023395754, -14.24916261073750334, 64.58142169135716415 ) ) ;
#34676=CARTESIAN_POINT ( 'NONE',  ( -19.22943505703176115, -8.044692082162882230, 63.50259577331515715 ) ) ;
#34677=DIRECTION ( 'NONE',  ( -5.731567514496413899E-31, -1.020425574103664789E-16, -1.000000000000000000 ) ) ;
#34679=ORIENTED_EDGE ( 'NONE', *, *, #2049, .T. ) ;
#34680=VERTEX_POINT ( 'NONE', #10216 ) ;
#34683=CARTESIAN_POINT ( 'NONE',  ( -10.42496409799848323, -14.69883155267435626, 71.62782692796884021 ) ) ;
#34685=CARTESIAN_POINT ( 'NONE',  ( -24.41160895735743352, -13.85031893932584701, 73.00782755091154286 ) ) ;
#34686=CARTESIAN_POINT ( 'NONE',  ( -11.60006141122767609, -10.16330251221877390, 71.08397807149754044 ) ) ;
#34687=CARTESIAN_POINT ( 'NONE',  ( -18.55956930788366677, -7.446158750330262421, 74.02559786541287679 ) ) ;
#34689=ORIENTED_EDGE ( 'NONE', *, *, #48623, .F. ) ;
#34690=EDGE_LOOP ( 'NONE', ( #16525, #34719, #6548, #31573, #30618 ) ) ;
#34692=CARTESIAN_POINT ( 'NONE',  ( -22.98865682493615381, -9.855478938366896813, 70.12683207277369490 ) ) ;
#34694=EDGE_CURVE ( 'NONE', #8655, #40234, #24366, .T. ) ;
#34696=CARTESIAN_POINT ( 'NONE',  ( -11.51319708992055801, -18.65819952746894472, 68.30869917720363560 ) ) ;
#34698=EDGE_CURVE ( 'NONE', #38602, #20878, #48417, .T. ) ;
#34699=CARTESIAN_POINT ( 'NONE',  ( -18.76715758977493209, -7.481188742717107765, 70.41422074109146934 ) ) ;
#34700=ORIENTED_EDGE ( 'NONE', *, *, #15305, .T. ) ;
#34701=EDGE_LOOP ( 'NONE', ( #41712, #28623, #32153, #36694, #26993 ) ) ;
#34702=CYLINDRICAL_SURFACE ( 'NONE', #33519, 0.1500000000000008826 ) ;
#34703=DIRECTION ( 'NONE',  ( 0.6043825497304157190, -0.7966942535134532433, 5.656674838975381179E-08 ) ) ;
#34705=CARTESIAN_POINT ( 'NONE',  ( -23.98984720795339243, -17.39877237835929691, 73.02768823732557735 ) ) ;
#34707=EDGE_CURVE ( 'NONE', #8636, #32302, #34277, .T. ) ;
#34708=ORIENTED_EDGE ( 'NONE', *, *, #8186, .T. ) ;
#34710=CARTESIAN_POINT ( 'NONE',  ( -10.53709656823301799, -16.06259630760735035, 68.27767780832155609 ) ) ;
#34715=CARTESIAN_POINT ( 'NONE',  ( -22.66727051383977809, -10.09628829486277546, 70.31178520457007153 ) ) ;
#34716=CARTESIAN_POINT ( 'NONE',  ( -17.56717507065399531, -7.360494836047319467, 63.73552460944732445 ) ) ;
#34717=VERTEX_POINT ( 'NONE', #22757 ) ;
#34718=CARTESIAN_POINT ( 'NONE',  ( -10.49991634527385287, -13.77081010382293158, 57.55898204955100539 ) ) ;
#34719=ORIENTED_EDGE ( 'NONE', *, *, #17763, .T. ) ;
#34720=CYLINDRICAL_SURFACE ( 'NONE', #14133, 0.1500000000000079881 ) ;
#34721=B_SPLINE_CURVE_WITH_KNOTS ( 'NONE', 3,
 ( #12858, #9183, #47341, #24200, #2512, #17515, #16787, #39209, #5738, #28127 ),
 .UNSPECIFIED., .F., .F.,
 ( 4, 2, 2, 2, 4 ),
 ( 0.6272669072877680163, 0.7522669073072806301, 0.8772669073267931328, 1.002266907346305747, 1.127266907365818360 ),
 .UNSPECIFIED. ) ;
#34723=CARTESIAN_POINT ( 'NONE',  ( -20.49049834636491596, -8.516442497579440385, 63.31121494938373928 ) ) ;
#34724=ORIENTED_EDGE ( 'NONE', *, *, #33578, .F. ) ;
#34726=PLANE ( 'NONE',  #43895 ) ;
#34728=DIRECTION ( 'NONE',  ( -0.8604039311673230550, -0.5096126717731922495, 7.110477544621476444E-08 ) ) ;
#34731=ORIENTED_EDGE ( 'NONE', *, *, #46092, .F. ) ;
#34732=CARTESIAN_POINT ( 'NONE',  ( -19.18784946220089083, -21.58347464219594514, 58.82507428380127834 ) ) ;
#34733=CARTESIAN_POINT ( 'NONE',  ( -18.19071170428347273, -21.76716127234782761, 65.36034592301929536 ) ) ;
#34734=CARTESIAN_POINT ( 'NONE',  ( -14.72744631621160494, -8.295007313424175521, 60.60524229057013201 ) ) ;
#34735=CARTESIAN_POINT ( 'NONE',  ( -18.53201708017407157, -7.846807123103141102, 74.14064401780551350 ) ) ;
#34736=CARTESIAN_POINT ( 'NONE',  ( -17.67903503446239455, -25.24601286685181023, 54.49999999999995026 ) ) ;
#34738=ORIENTED_EDGE ( 'NONE', *, *, #3210, .F. ) ;
#34740=DIRECTION ( 'NONE',  ( -3.084459869131082876E-06, 5.853393715878419656E-06, -0.9999999999781118420 ) ) ;
#34741=CARTESIAN_POINT ( 'NONE',  ( -12.03169470190467827, -10.26217700280571421, 71.06073263571943244 ) ) ;
#34743=CARTESIAN_POINT ( 'NONE',  ( -22.53655392111809164, -20.22829597721307948, 65.88917050827579658 ) ) ;
#34746=CARTESIAN_POINT ( 'NONE',  ( -11.07857854458970692, -11.73724703412850801, 71.08860870961423473 ) ) ;
#34747=CARTESIAN_POINT ( 'NONE',  ( -21.01123855637963089, -20.87838213191899683, 65.58453944497207999 ) ) ;
#34748=CARTESIAN_POINT ( 'NONE',  ( -15.73542338568409349, -8.015832264148292197, 70.60989886599207921 ) ) ;
#34750=ORIENTED_EDGE ( 'NONE', *, *, #27552, .F. ) ;
#34752=CARTESIAN_POINT ( 'NONE',  ( -24.38143503755601316, -15.58083059521001168, 73.30303748419844112 ) ) ;
#34754=CARTESIAN_POINT ( 'NONE',  ( -17.59211729576255934, -7.811223397794364587, 63.55057029380298417 ) ) ;
#34755=CARTESIAN_POINT ( 'NONE',  ( -19.94917705995926482, -8.226604131702123013, 74.00624557436877637 ) ) ;
#34756=( BOUNDED_SURFACE ( )  B_SPLINE_SURFACE ( 3, 1, ( 
 ( #30998, #477 ),
 ( #41845, #31236 ),
 ( #8118, #42324 ),
 ( #8592, #23134 ),
 ( #38124, #4904 ),
 ( #4401, #19915 ),
 ( #46259, #26326 ) ),
 .UNSPECIFIED., .T., .F., .F. ) 
 B_SPLINE_SURFACE_WITH_KNOTS ( ( 4, 3, 4 ),
 ( 2, 2 ),
 ( 0.000000000000000000, 0.5000000000000000000, 1.000000000000000000 ),
 ( 0.000000000000000000, 1.000000000000000000 ),
 .UNSPECIFIED. ) 
 GEOMETRIC_REPRESENTATION_ITEM ( )  RATIONAL_B_SPLINE_SURFACE ( (
 ( 1.000000000000000000, 1.000000000000000000),
 ( 0.3333333333333335369, 0.3333333333333330373),
 ( 0.3333333333333335369, 0.3333333333333330373),
 ( 1.000000000000000000, 1.000000000000000000),
 ( 0.3333333333333333703, 0.3333333333333333703),
 ( 0.3333333333333333703, 0.3333333333333333703),
 ( 1.000000000000000000, 1.000000000000000000) ) ) 
 REPRESENTATION_ITEM ( '' )  SURFACE ( )  );
#34757=CARTESIAN_POINT ( 'NONE',  ( -19.84080129957490612, -21.85712737670714390, 65.57830891090566183 ) ) ;
#34758=ORIENTED_EDGE ( 'NONE', *, *, #21891, .F. ) ;
#34760=CARTESIAN_POINT ( 'NONE',  ( -19.92776479198160189, -21.39998277484045275, 72.41950795000725805 ) ) ;
#34761=B_SPLINE_CURVE_WITH_KNOTS ( 'NONE', 3,
 ( #31499, #31018, #38385, #12782, #31745, #46039, #16940, #27316, #12061, #23384 ),
 .UNSPECIFIED., .F., .F.,
 ( 4, 2, 2, 2, 4 ),
 ( 0.1272669073658920791, 0.2522669073463494893, 0.3772669073268068995, 0.5022669073072643098, 0.6272669072877217200 ),
 .UNSPECIFIED. ) ;
#34762=ORIENTED_EDGE ( 'NONE', *, *, #26891, .F. ) ;
#34763=CARTESIAN_POINT ( 'NONE',  ( -17.25805186741143871, -7.753187986760909034, 63.70624286928425306 ) ) ;
#34765=CARTESIAN_POINT ( 'NONE',  ( -12.77013062424865630, -8.927826924028671840, 53.49999999999994316 ) ) ;
#34766=ORIENTED_EDGE ( 'NONE', *, *, #19621, .T. ) ;
#34767=( BOUNDED_CURVE ( )  B_SPLINE_CURVE ( 3, ( #2790, #18283, #21754, #3029 ),
 .UNSPECIFIED., .F., .F. ) 
 B_SPLINE_CURVE_WITH_KNOTS ( ( 4, 4 ),
 ( 4.712388980384690562, 4.921828490624010399 ),
 .UNSPECIFIED. ) 
 CURVE ( )  GEOMETRIC_REPRESENTATION_ITEM ( )  RATIONAL_B_SPLINE_CURVE ( ( 1.000000000000000000, 0.9963479302455154896, 0.9963479302455154896, 1.000000000000000000 ) ) 
 REPRESENTATION_ITEM ( '' )  );
#34768=EDGE_CURVE ( 'NONE', #37232, #21212, #18501, .T. ) ;
#34769=CARTESIAN_POINT ( 'NONE',  ( -10.43073325114686511, -14.50439929630985603, 68.15800126138398696 ) ) ;
#34770=CARTESIAN_POINT ( 'NONE',  ( -13.40918607372062610, -8.533554674359928427, 57.07693621075073054 ) ) ;
#34771=EDGE_CURVE ( 'NONE', #24347, #44341, #19648, .T. ) ;
#34772=EDGE_CURVE ( 'NONE', #25179, #27516, #31933, .T. ) ;
#34774=CARTESIAN_POINT ( 'NONE',  ( -17.75017200679030083, -21.85170198611075065, 58.70553379369455627 ) ) ;
#34775=B_SPLINE_CURVE_WITH_KNOTS ( 'NONE', 3,
 ( #20810, #24030, #9500, #35809, #39521, #28452, #27709, #43474, #9736, #31161 ),
 .UNSPECIFIED., .F., .F.,
 ( 4, 2, 2, 2, 4 ),
 ( 0.000000000000000000, 0.2500000000000000000, 0.5000000000000000000, 0.7500000000000000000, 1.000000000000000000 ),
 .UNSPECIFIED. ) ;
#34776=FACE_OUTER_BOUND ( 'NONE', #21737, .T. ) ;
#34777=ORIENTED_EDGE ( 'NONE', *, *, #36642, .F. ) ;
#34778=CARTESIAN_POINT ( 'NONE',  ( -11.36856035537877396, -11.29517376149446761, 64.37711966785748530 ) ) ;
#34780=EDGE_CURVE ( 'NONE', #1356, #3049, #26720, .T. ) ;
#34781=EDGE_CURVE ( 'NONE', #24975, #44310, #11912, .T. ) ;
#34782=CARTESIAN_POINT ( 'NONE',  ( -11.13656563017467782, -10.81292993477855902, 57.40241537293904628 ) ) ;
#34783=CARTESIAN_POINT ( 'NONE',  ( -22.23704373183037575, -20.49607752381679759, 58.90296374359631670 ) ) ;
#34784=CARTESIAN_POINT ( 'NONE',  ( -23.36965734407794670, -18.59798837310562902, 69.58812159897662752 ) ) ;
#34785=EDGE_LOOP ( 'NONE', ( #4952, #29833, #22080, #11163, #12789 ) ) ;
#34786=CARTESIAN_POINT ( 'NONE',  ( -11.04141120970326462, -11.93494789359697883, 74.55840195308121565 ) ) ;
#34787=CARTESIAN_POINT ( 'NONE',  ( -24.08597852354971280, -11.47399750213189407, 63.07405535103134753 ) ) ;
#34788=CARTESIAN_POINT ( 'NONE',  ( -16.15548939330727407, -7.924675066161051440, 63.95394534455144253 ) ) ;
#34791=CARTESIAN_POINT ( 'NONE',  ( -22.76771927571487453, -10.21026527410489138, 66.83622464935415053 ) ) ;
#34792=CARTESIAN_POINT ( 'NONE',  ( -17.59331747086620368, -7.761237804118464645, 63.85057029381061966 ) ) ;
#34797=DIRECTION ( 'NONE',  ( -0.1186632576870824130, 0.9929345553837299887, 6.051931679537041823E-08 ) ) ;
#34798=CARTESIAN_POINT ( 'NONE',  ( -10.44881481234349252, -17.42631575494719698, 64.74243950200344955 ) ) ;
#34799=ORIENTED_EDGE ( 'NONE', *, *, #5156, .F. ) ;
#34801=DIRECTION ( 'NONE',  ( 4.664556981411351282E-06, -8.285185778185610086E-06, 0.9999999999547987128 ) ) ;
#34802=CARTESIAN_POINT ( 'NONE',  ( -22.92319923916556235, -10.39759239192951235, 63.07185995337424345 ) ) ;
#34803=CARTESIAN_POINT ( 'NONE',  ( -14.62324711167149260, -21.22583875644025753, 58.39447665211296368 ) ) ;
#34804=EDGE_LOOP ( 'NONE', ( #40210, #32379, #24889, #36475, #35803 ) ) ;
#34805=CARTESIAN_POINT ( 'NONE',  ( -24.40666182452685362, -14.31463369505075001, 66.40966133397022020 ) ) ;
#34806=FACE_OUTER_BOUND ( 'NONE', #21549, .T. ) ;
#34807=CARTESIAN_POINT ( 'NONE',  ( -12.41791333049023116, -9.841008508234809327, 60.97406688302051947 ) ) ;
#34808=EDGE_LOOP ( 'NONE', ( #21782, #45755, #23053, #2837, #28969 ) ) ;
#34809=CARTESIAN_POINT ( 'NONE',  ( -11.43942668935558515, -18.54264994400395850, 57.80714389716341373 ) ) ;
#34811=CARTESIAN_POINT ( 'NONE',  ( -10.01424894596331505, -14.03598936870067782, 61.17467227907766869 ) ) ;
#34812=CARTESIAN_POINT ( 'NONE',  ( -21.73797167162284438, -8.735188488120728678, 70.23794211215633254 ) ) ;
#34813=DIRECTION ( 'NONE',  ( 0.9796876409582463419, -0.2005296141562635803, -7.890952368640937478E-08 ) ) ;
#34814=EDGE_LOOP ( 'NONE', ( #47510, #19979, #27381, #13706, #44897 ) ) ;
#34815=ORIENTED_EDGE ( 'NONE', *, *, #29887, .T. ) ;
#34817=CARTESIAN_POINT ( 'NONE',  ( -13.87406498055279158, -8.713951040527767589, 74.19954688782125629 ) ) ;
#34818=CARTESIAN_POINT ( 'NONE',  ( -23.41977742916776251, -11.19648202114625235, 73.66193302070908544 ) ) ;
#34819=CARTESIAN_POINT ( 'NONE',  ( -17.77920954038207668, -22.25082405446125122, 58.59048702730397196 ) ) ;
#34820=ADVANCED_FACE ( 'NONE', ( #30389 ), #1061, .T. ) ;
#34822=CARTESIAN_POINT ( 'NONE',  ( -20.20088676517873694, -8.325823464045813083, 74.13585170226248522 ) ) ;
#34823=B_SPLINE_CURVE_WITH_KNOTS ( 'NONE', 3,
 ( #30047, #18684, #47764, #48484, #32965, #14248, #37644, #10820, #7143, #36907 ),
 .UNSPECIFIED., .F., .F.,
 ( 4, 2, 2, 2, 4 ),
 ( 0.1272669073658264371, 0.2522669073439405274, 0.3772669073220545899, 0.5022669073001687634, 0.6272669072782828259 ),
 .UNSPECIFIED. ) ;
#34824=CARTESIAN_POINT ( 'NONE',  ( -17.78516316699992217, -21.85793681952389989, 65.48965078530844153 ) ) ;
#34826=CARTESIAN_POINT ( 'NONE',  ( -12.64995474452274138, -19.99670071527213366, 68.63657438322856308 ) ) ;
#34827=CARTESIAN_POINT ( 'NONE',  ( -10.47654091737289050, -16.00694475801543248, 67.97767859625193410 ) ) ;
#34829=EDGE_CURVE ( 'NONE', #35725, #21025, #23567, .T. ) ;
#34830=EDGE_CURVE ( 'NONE', #3552, #21656, #37335, .T. ) ;
#34833=VERTEX_POINT ( 'NONE', #34537 ) ;
#34834=CARTESIAN_POINT ( 'NONE',  ( -8.912481985338086332, -18.08067441140542186, 54.49999999999995026 ) ) ;
#34836=CARTESIAN_POINT ( 'NONE',  ( -11.97490362423377164, -10.33561459433851404, 67.78424783647008667 ) ) ;
#34839=CARTESIAN_POINT ( 'NONE',  ( -21.57995947450667984, -9.113990939708571659, 70.14604673427196246 ) ) ;
#34840=CARTESIAN_POINT ( 'NONE',  ( -24.47213906732331878, -17.22327966652203202, 72.98361780307556046 ) ) ;
#34843=CARTESIAN_POINT ( 'NONE',  ( -17.79333148728606417, -22.25021806323848494, 58.54406892197518886 ) ) ;
#34845=FACE_BOUND ( 'NONE', #6567, .T. ) ;
#34846=B_SPLINE_CURVE_WITH_KNOTS ( 'NONE', 1,
 ( #22789, #34322 ),
 .UNSPECIFIED., .F., .F.,
 ( 2, 2 ),
 ( 0.000000000000000000, 1.000000000000000000 ),
 .UNSPECIFIED. ) ;
#34848=CARTESIAN_POINT ( 'NONE',  ( -23.34611474887041282, -10.97735184451543589, 73.57013074316820678 ) ) ;
#34849=ADVANCED_FACE ( 'NONE', ( #9429 ), #46847, .T. ) ;
#34850=VECTOR ( 'NONE', #33599, 1000.000000000000227 ) ;
#34851=CARTESIAN_POINT ( 'NONE',  ( -14.51923423662272938, -21.23689935983381716, 58.25797845284014187 ) ) ;
#34855=CARTESIAN_POINT ( 'NONE',  ( -12.18170072908086965, -10.17053062278287889, 64.32914326641392222 ) ) ;
#34856=CARTESIAN_POINT ( 'NONE',  ( -16.79771060966972129, -22.23299631151009237, 68.85594001288120580 ) ) ;
#34859=FACE_BOUND ( 'NONE', #24574, .T. ) ;
#34860=ORIENTED_EDGE ( 'NONE', *, *, #36793, .F. ) ;
#34862=ORIENTED_EDGE ( 'NONE', *, *, #33432, .F. ) ;
#34865=CARTESIAN_POINT ( 'NONE',  ( -14.56922802208840828, -8.416425255985021892, 67.48804881135004052 ) ) ;
#34866=CARTESIAN_POINT ( 'NONE',  ( -11.86332896968958650, -9.851264934370021820, 64.13640162903247699 ) ) ;
#34867=CARTESIAN_POINT ( 'NONE',  ( -11.12358174778395714, -11.75903488045733347, 71.38860871064898106 ) ) ;
#34871=FACE_OUTER_BOUND ( 'NONE', #48633, .T. ) ;
#34873=DIRECTION ( 'NONE',  ( 5.854827030937197869E-31, 1.020425574103664912E-16, 1.000000000000000000 ) ) ;
#34875=EDGE_CURVE ( 'NONE', #40518, #22263, #33582, .T. ) ;
#34880=CARTESIAN_POINT ( 'NONE',  ( -19.11145557798581152, -7.964112677450091660, 63.73089235102099792 ) ) ;
#34883=( BOUNDED_CURVE ( )  B_SPLINE_CURVE ( 3, ( #18966, #34455, #15487, #30552 ),
 .UNSPECIFIED., .F., .F. ) 
 B_SPLINE_CURVE_WITH_KNOTS ( ( 4, 4 ),
 ( 0.5000000000000000000, 0.9074455897393663983 ),
 .UNSPECIFIED. ) 
 CURVE ( )  GEOMETRIC_REPRESENTATION_ITEM ( )  RATIONAL_B_SPLINE_CURVE ( ( 1.000000000000010658, 0.4567392136813307468, 0.3561768502900223843, 0.6983129098260969503 ) ) 
 REPRESENTATION_ITEM ( '' )  );
#34884=ORIENTED_EDGE ( 'NONE', *, *, #36789, .F. ) ;
#34885=CARTESIAN_POINT ( 'NONE',  ( -16.52316554273587101, -21.80170452179945073, 65.24036514508233608 ) ) ;
#34886=CARTESIAN_POINT ( 'NONE',  ( -21.61813339613238227, -8.651787399021619862, 73.71633365192373333 ) ) ;
#34887=CARTESIAN_POINT ( 'NONE',  ( -10.42892955798469323, -14.54578234806194992, 67.85800118616361942 ) ) ;
#34889=EDGE_CURVE ( 'NONE', #29740, #27105, #31748, .T. ) ;
#34891=CARTESIAN_POINT ( 'NONE',  ( -10.45256745270239307, -15.43993597667916795, 57.86792809192976961 ) ) ;
#34892=ADVANCED_FACE ( 'NONE', ( #24455 ), #35514, .T. ) ;
#34893=CARTESIAN_POINT ( 'NONE',  ( -21.34581862946232889, -20.66775363590295456, 72.52446429492310642 ) ) ;
#34894=CARTESIAN_POINT ( 'NONE',  ( -12.35838514372898800, -20.27197932131825198, 68.44383270345304027 ) ) ;
#34896=CARTESIAN_POINT ( 'NONE',  ( -10.02134419679888211, -13.96483583313674615, 61.10476640098193002 ) ) ;
#34897=( BOUNDED_CURVE ( )  B_SPLINE_CURVE ( 3, ( #12821, #34980, #12583, #20211 ),
 .UNSPECIFIED., .F., .F. ) 
 B_SPLINE_CURVE_WITH_KNOTS ( ( 4, 4 ),
 ( 0.5000000000000000000, 0.9074455897393671755 ),
 .UNSPECIFIED. ) 
 CURVE ( )  GEOMETRIC_REPRESENTATION_ITEM ( )  RATIONAL_B_SPLINE_CURVE ( ( 0.9999999999999841238, 0.4567392136813330783, 0.3561768502900416467, 0.6983129098260927314 ) ) 
 REPRESENTATION_ITEM ( '' )  );
#34898=VERTEX_POINT ( 'NONE', #28129 ) ;
#34900=CARTESIAN_POINT ( 'NONE',  ( -14.86477050248655551, -7.812526586475418533, 57.10645908473438226 ) ) ;
#34901=EDGE_CURVE ( 'NONE', #43456, #15655, #45985, .T. ) ;
#34903=CARTESIAN_POINT ( 'NONE',  ( -13.07136655094769750, -8.762923122256669473, 64.02451139116674028 ) ) ;
#34904=CARTESIAN_POINT ( 'NONE',  ( -18.32857646159318676, -22.20418385865972155, 68.93019298464047040 ) ) ;
#34906=DIRECTION ( 'NONE',  ( 2.210955087992717862E-06, -1.097707075699772489E-06, 0.9999999999969533260 ) ) ;
#34907=ORIENTED_EDGE ( 'NONE', *, *, #25702, .F. ) ;
#34908=CARTESIAN_POINT ( 'NONE',  ( -9.996284180359110039, -14.23299000612383303, 64.51086969714638997 ) ) ;
#34911=FACE_OUTER_BOUND ( 'NONE', #27703, .T. ) ;
#34912=CARTESIAN_POINT ( 'NONE',  ( -10.49189908542464700, -16.09426454567519116, 68.26295692486267797 ) ) ;
#34913=EDGE_LOOP ( 'NONE', ( #47161, #4626, #2907, #22362, #43325 ) ) ;
#34914=DIRECTION ( 'NONE',  ( 0.9271861211590526342, 0.3746009833543293421, -1.005599061620490611E-08 ) ) ;
#34916=CARTESIAN_POINT ( 'NONE',  ( -21.79997194174348607, -9.271457673084677609, 70.27565669584988939 ) ) ;
#34917=AXIS2_PLACEMENT_3D ( 'NONE', #29642, #37011, #18296 ) ;
#34919=ORIENTED_EDGE ( 'NONE', *, *, #40667, .F. ) ;
#34920=CARTESIAN_POINT ( 'NONE',  ( -22.80992383800762724, -10.33718617846504273, 66.82565708633600821 ) ) ;
#34921=CARTESIAN_POINT ( 'NONE',  ( -24.09792889798371007, -17.08130376423426000, 73.18336032035891492 ) ) ;
#34922=CARTESIAN_POINT ( 'NONE',  ( -11.22150886908280931, -18.16670198096008093, 58.22203402163793839 ) ) ;
#34924=CARTESIAN_POINT ( 'NONE',  ( -24.17899278864585355, -11.66673636667039027, 59.66731167108189737 ) ) ;
#34926=CARTESIAN_POINT ( 'NONE',  ( -19.70639647806698136, -21.90109437720271757, 65.57990800639531415 ) ) ;
#34927=CARTESIAN_POINT ( 'NONE',  ( -23.75797280549784318, -17.78947120508452429, 59.30378417803890301 ) ) ;
#34930=CARTESIAN_POINT ( 'NONE',  ( -11.25339550917664333, -11.39346175823023088, 60.56396915994215391 ) ) ;
#34931=( NAMED_UNIT ( * ) PLANE_ANGLE_UNIT ( ) SI_UNIT ( $, .RADIAN. ) );
#34933=CARTESIAN_POINT ( 'NONE',  ( -13.54792730259346456, -8.920061342218058797, 57.25495614889487683 ) ) ;
#34936=ORIENTED_EDGE ( 'NONE', *, *, #40027, .T. ) ;
#34938=CARTESIAN_POINT ( 'NONE',  ( -24.86242989439883289, -14.39095395922188558, 66.36788051138485400 ) ) ;
#34940=CARTESIAN_POINT ( 'NONE',  ( -15.83004105235379022, -7.531612319186171689, 67.26290417877635264 ) ) ;
#34941=EDGE_LOOP ( 'NONE', ( #11752, #40022, #43926, #6667, #6776 ) ) ;
#34942=CARTESIAN_POINT ( 'NONE',  ( -21.94242186726961208, -9.397052521110282441, 60.00699132926281010 ) ) ;
#34943=CARTESIAN_POINT ( 'NONE',  ( -19.30271816048872324, -8.014114901043837946, 60.26092997144683494 ) ) ;
#34945=ORIENTED_EDGE ( 'NONE', *, *, #1089, .F. ) ;
#34947=CARTESIAN_POINT ( 'NONE',  ( -14.63779949229408750, -10.05162950738736072, 53.69233794759168887 ) ) ;
#34948=CARTESIAN_POINT ( 'NONE',  ( -22.17450858901738897, -19.95071429852638545, 66.00421734751543568 ) ) ;
#34949=VERTEX_POINT ( 'NONE', #24921 ) ;
#34950=CARTESIAN_POINT ( 'NONE',  ( -13.11945872550529657, -9.225962324091906197, 67.67942785705487552 ) ) ;
#34951=ORIENTED_EDGE ( 'NONE', *, *, #42956, .F. ) ;
#34952=DIRECTION ( 'NONE',  ( 0.1571515419521612722, -0.9875744999047174622, 7.433889655140131751E-08 ) ) ;
#34955=ORIENTED_EDGE ( 'NONE', *, *, #20168, .T. ) ;
#34956=CARTESIAN_POINT ( 'NONE',  ( -23.80175822008580866, -17.82088921309938812, 62.88849600917846061 ) ) ;
#34959=CARTESIAN_POINT ( 'NONE',  ( -15.06075745000970834, -21.87520294740874149, 68.76248218113177302 ) ) ;
#34964=VERTEX_POINT ( 'NONE', #42681 ) ;
#34967=CARTESIAN_POINT ( 'NONE',  ( -14.60479643987598841, -7.913168514039711887, 60.50491717424539218 ) ) ;
#34968=CARTESIAN_POINT ( 'NONE',  ( -24.59325023630216833, -12.78233532962698682, 66.46280073947134781 ) ) ;
#34969=CARTESIAN_POINT ( 'NONE',  ( -12.55411140858086760, -19.90724249994213935, 65.15202838036978505 ) ) ;
#34971=VERTEX_POINT ( 'NONE', #28850 ) ;
#34972=CARTESIAN_POINT ( 'NONE',  ( -21.31800492490012999, -20.62620369199774117, 72.52446429884872714 ) ) ;
#34973=ORIENTED_EDGE ( 'NONE', *, *, #38886, .F. ) ;
#34974=CARTESIAN_POINT ( 'NONE',  ( -24.12651600458584511, -12.62191667979047338, 73.25697658996379857 ) ) ;
#34975=CARTESIAN_POINT ( 'NONE',  ( -15.19396558280303822, -21.91766586989539434, 68.61946996636811491 ) ) ;
#34976=CARTESIAN_POINT ( 'NONE',  ( -10.27127829932231862, -12.72555322402984146, 64.44552998452087422 ) ) ;
#34978=EDGE_CURVE ( 'NONE', #40830, #5810, #38644, .T. ) ;
#34979=CARTESIAN_POINT ( 'NONE',  ( -11.06939607882469190, -17.86905163984256006, 71.45229597776977926 ) ) ;
#34980=CARTESIAN_POINT ( 'NONE',  ( -10.89363166428750773, -17.47500997361330022, 71.65898155907456157 ) ) ;
#34981=DIRECTION ( 'NONE',  ( 0.9986807914369958405, -0.05134858142905002198, 1.286972170232540014E-09 ) ) ;
#34982=EDGE_CURVE ( 'NONE', #748, #36010, #41825, .T. ) ;
#34983=VECTOR ( 'NONE', #20410, 1000.000000000000114 ) ;
#34985=CARTESIAN_POINT ( 'NONE',  ( -22.68646401470678953, -20.08284273627726435, 69.35913316877790180 ) ) ;
#34986=EDGE_CURVE ( 'NONE', #26512, #29684, #23665, .T. ) ;
#34989=CARTESIAN_POINT ( 'NONE',  ( -22.51638425468451743, -9.928425624739869448, 70.21998462585445111 ) ) ;
#34990=CARTESIAN_POINT ( 'NONE',  ( -17.72591277652480812, -7.814435863317398479, 63.77886828924947338 ) ) ;
#34991=CARTESIAN_POINT ( 'NONE',  ( -17.39742496553465401, -7.759256980052345654, 67.02039592192090822 ) ) ;
#34992=B_SPLINE_CURVE_WITH_KNOTS ( 'NONE', 3,
 ( #17291, #24707, #32336, #9921, #42695, #2040, #6225, #1556, #32086, #12876 ),
 .UNSPECIFIED., .F., .F.,
 ( 4, 2, 2, 2, 4 ),
 ( 0.6272669072878003238, 0.7522669073073093848, 0.8772669073268185569, 1.002266907346327729, 1.127266907365836790 ),
 .UNSPECIFIED. ) ;
#34993=ORIENTED_EDGE ( 'NONE', *, *, #7623, .T. ) ;
#34994=ORIENTED_EDGE ( 'NONE', *, *, #3386, .F. ) ;
#34996=ORIENTED_EDGE ( 'NONE', *, *, #45905, .T. ) ;
#34997=B_SPLINE_CURVE_WITH_KNOTS ( 'NONE', 3,
 ( #24626, #31758, #20440, #42847, #36158, #47013, #28054, #2678, #39136, #5419 ),
 .UNSPECIFIED., .F., .F.,
 ( 4, 2, 2, 2, 4 ),
 ( 0.1272669073658367345, 0.2522669073463192357, 0.3772669073268017925, 0.5022669073072842938, 0.6272669072877667951 ),
 .UNSPECIFIED. ) ;
#34998=CARTESIAN_POINT ( 'NONE',  ( -11.17943887680513981, -18.87220427245064513, 65.00353025264104190 ) ) ;
#34999=CARTESIAN_POINT ( 'NONE',  ( -11.00006132919183521, -18.58228645891882280, 57.92901817424456112 ) ) ;
#35000=ORIENTED_EDGE ( 'NONE', *, *, #41291, .F. ) ;
#35002=CARTESIAN_POINT ( 'NONE',  ( -15.56465948913147557, -7.543361525925788236, 54.27966884056655061 ) ) ;
#35004=CARTESIAN_POINT ( 'NONE',  ( -14.11063322135152909, -21.03236308526469855, 72.21135587486895702 ) ) ;
#35007=CARTESIAN_POINT ( 'NONE',  ( -10.83683315258895519, -12.44108567723101899, 57.32857332099802505 ) ) ;
#35008=CARTESIAN_POINT ( 'NONE',  ( -13.54546414475118610, -21.17012168889900181, 65.14662202029667526 ) ) ;
#35009=B_SPLINE_CURVE_WITH_KNOTS ( 'NONE', 1,
 ( #21246, #18494 ),
 .UNSPECIFIED., .F., .F.,
 ( 2, 2 ),
 ( 0.000000000000000000, 1.000000000000000000 ),
 .UNSPECIFIED. ) ;
#35011=CARTESIAN_POINT ( 'NONE',  ( -23.08487763607990928, -19.01185175973044039, 62.36879011380454330 ) ) ;
#35012=CARTESIAN_POINT ( 'NONE',  ( -16.71957921250844592, -21.82421608262117729, 68.71032757591046902 ) ) ;
#35013=EDGE_CURVE ( 'NONE', #33357, #39181, #46846, .T. ) ;
#35014=CARTESIAN_POINT ( 'NONE',  ( -19.56272746357835501, -21.53536514712069305, 58.68074270823246508 ) ) ;
#35015=ORIENTED_EDGE ( 'NONE', *, *, #41247, .T. ) ;
#35018=CARTESIAN_POINT ( 'NONE',  ( -21.99213670719075253, -20.17946569659695655, 59.04970794435396897 ) ) ;
#35019=( BOUNDED_SURFACE ( )  B_SPLINE_SURFACE ( 3, 1, ( 
 ( #24333, #9566 ),
 ( #38355, #46506 ),
 ( #12984, #46970 ),
 ( #955, #16918 ),
 ( #5137, #20145 ),
 ( #46015, #13215 ),
 ( #27293, #4899 ) ),
 .UNSPECIFIED., .T., .F., .F. ) 
 B_SPLINE_SURFACE_WITH_KNOTS ( ( 4, 3, 4 ),
 ( 2, 2 ),
 ( 0.000000000000000000, 0.5000000000000000000, 1.000000000000000000 ),
 ( 0.000000000000000000, 1.000000000000000000 ),
 .UNSPECIFIED. ) 
 GEOMETRIC_REPRESENTATION_ITEM ( )  RATIONAL_B_SPLINE_SURFACE ( (
 ( 1.000000000000000000, 1.000000000000000000),
 ( 0.3333333333333335369, 0.3333333333333330373),
 ( 0.3333333333333335369, 0.3333333333333330373),
 ( 1.000000000000000000, 1.000000000000000000),
 ( 0.3333333333333333703, 0.3333333333333333703),
 ( 0.3333333333333333703, 0.3333333333333333703),
 ( 1.000000000000000000, 1.000000000000000000) ) ) 
 REPRESENTATION_ITEM ( '' )  SURFACE ( )  );
#35021=CARTESIAN_POINT ( 'NONE',  ( -24.08517543038346531, -12.49907855475201579, 73.52753481283211556 ) ) ;
#35024=CARTESIAN_POINT ( 'NONE',  ( -11.01197672498281044, -17.74032467813711733, 71.85246142747087106 ) ) ;
#35025=CARTESIAN_POINT ( 'NONE',  ( -12.07742570852865427, -19.41007429933622319, 58.22682412763990811 ) ) ;
#35028=EDGE_LOOP ( 'NONE', ( #5462, #3834, #43764, #33648, #29647 ) ) ;
#35030=CARTESIAN_POINT ( 'NONE',  ( -11.81042834955647258, -10.54382735031610174, 74.45357240259568243 ) ) ;
#35032=CARTESIAN_POINT ( 'NONE',  ( -23.27284462870851911, -18.74605969774991010, 66.10917289053097079 ) ) ;
#35033=CARTESIAN_POINT ( 'NONE',  ( -15.01062035279700346, -21.85762174227016885, 65.26630065318278184 ) ) ;
#35034=CARTESIAN_POINT ( 'NONE',  ( -21.39967327233876659, -20.63170314183283693, 72.80974286114339122 ) ) ;
#35035=CARTESIAN_POINT ( 'NONE',  ( -23.25220530991251167, -10.16847870644612328, 63.26524311255320043 ) ) ;
#35036=DIRECTION ( 'NONE',  ( 3.549360974554993999E-17, -6.371834667797928663E-18, -1.000000000000000000 ) ) ;
#35037=( BOUNDED_CURVE ( )  B_SPLINE_CURVE ( 3, ( #5197, #24152, #43359, #27836 ),
 .UNSPECIFIED., .F., .F. ) 
 B_SPLINE_CURVE_WITH_KNOTS ( ( 4, 4 ),
 ( 4.712388980384690562, 4.921828490624008623 ),
 .UNSPECIFIED. ) 
 CURVE ( )  GEOMETRIC_REPRESENTATION_ITEM ( )  RATIONAL_B_SPLINE_CURVE ( ( 1.000000000000000000, 0.9963479302455156006, 0.9963479302455156006, 1.000000000000000000 ) ) 
 REPRESENTATION_ITEM ( '' )  );
#35039=( BOUNDED_CURVE ( )  B_SPLINE_CURVE ( 3, ( #18407, #11521, #7361, #34159 ),
 .UNSPECIFIED., .F., .F. ) 
 B_SPLINE_CURVE_WITH_KNOTS ( ( 4, 4 ),
 ( 0.4074455897393624015, 0.5000000000000000000 ),
 .UNSPECIFIED. ) 
 CURVE ( )  GEOMETRIC_REPRESENTATION_ITEM ( )  RATIONAL_B_SPLINE_CURVE ( ( 0.6983129098260958401, 0.7760317562606984243, 0.8765941196519991818, 0.9999999999999965583 ) ) 
 REPRESENTATION_ITEM ( '' )  );
#35040=CARTESIAN_POINT ( 'NONE',  ( -23.71873315273824545, -11.74668173045760433, 63.25218284853021089 ) ) ;
#35041=EDGE_CURVE ( 'NONE', #45990, #46544, #7190, .T. ) ;
#35042=CARTESIAN_POINT ( 'NONE',  ( -20.70466284777608124, -8.568939270112290174, 60.14125232065403992 ) ) ;
#35043=CARTESIAN_POINT ( 'NONE',  ( -10.08184786930872789, -16.07202671437600117, 68.08493695327037187 ) ) ;
#35045=EDGE_CURVE ( 'NONE', #22219, #13885, #8181, .T. ) ;
#35046=ORIENTED_EDGE ( 'NONE', *, *, #3935, .T. ) ;
#35047=CARTESIAN_POINT ( 'NONE',  ( -23.96075626263749569, -17.45014286185010732, 66.24357239682277054 ) ) ;
#35049=CARTESIAN_POINT ( 'NONE',  ( -18.34560609025200861, -9.386954687716537293, 53.49999999999995026 ) ) ;
#35050=CARTESIAN_POINT ( 'NONE',  ( -10.13258936719380898, -16.33817337277914561, 71.63245765104117879 ) ) ;
#35052=( BOUNDED_CURVE ( )  B_SPLINE_CURVE ( 3, ( #3244, #7443, #7202, #3482 ),
 .UNSPECIFIED., .F., .F. ) 
 B_SPLINE_CURVE_WITH_KNOTS ( ( 4, 4 ),
 ( 0.4074455897279072869, 0.5000000000000000000 ),
 .UNSPECIFIED. ) 
 CURVE ( )  GEOMETRIC_REPRESENTATION_ITEM ( )  RATIONAL_B_SPLINE_CURVE ( ( 0.6983129097972519128, 0.7760317562358295396, 0.8765941196367486032, 1.000000000000016209 ) ) 
 REPRESENTATION_ITEM ( '' )  );
#35056=CARTESIAN_POINT ( 'NONE',  ( -19.85909577874797449, -21.37257635846961890, 72.46322212860958700 ) ) ;
#35057=DIRECTION ( 'NONE',  ( -0.6323592902076723421, -0.7746752403995151859, 4.984538757074985308E-08 ) ) ;
#35060=EDGE_CURVE ( 'NONE', #47966, #32808, #47431, .T. ) ;
#35061=CARTESIAN_POINT ( 'NONE',  ( -10.59656512619885227, -13.05092609425065220, 68.02360230423869325 ) ) ;
#35062=CARTESIAN_POINT ( 'NONE',  ( -13.91686182480500200, -8.236299899141551251, 74.31459327626868117 ) ) ;
#35063=CARTESIAN_POINT ( 'NONE',  ( -23.95986381193147707, -17.46034710541827906, 69.82828398331871256 ) ) ;
#35064=EDGE_LOOP ( 'NONE', ( #14328, #41265, #6880, #29855, #35828 ) ) ;
#35065=CARTESIAN_POINT ( 'NONE',  ( -24.12016595861979695, -18.07666464397348349, 59.19033703419022885 ) ) ;
#35066=CARTESIAN_POINT ( 'NONE',  ( -17.15681831196262408, -7.812702829301893637, 74.14945326254591862 ) ) ;
#35067=VERTEX_POINT ( 'NONE', #17517 ) ;
#35068=DIRECTION ( 'NONE',  ( -5.224165706511165539E-06, 4.853367013834837651E-07, 0.9999999999862362321 ) ) ;
#35072=CARTESIAN_POINT ( 'NONE',  ( -10.00186344861280396, -15.45246920467748275, 57.67518653529428718 ) ) ;
#35073=ADVANCED_FACE ( 'NONE', ( #6457 ), #25405, .T. ) ;
#35074=CARTESIAN_POINT ( 'NONE',  ( -21.69457540385530336, -9.196023516753362159, 70.54621400560100142 ) ) ;
#35075=CARTESIAN_POINT ( 'NONE',  ( -19.52323420048857372, -8.075080386471409355, 60.26093179093862062 ) ) ;
#35077=CARTESIAN_POINT ( 'NONE',  ( -18.60622096112062707, -22.16490860957766529, 72.47006221837980888 ) ) ;
#35079=DIRECTION ( 'NONE',  ( -0.9271861211590526342, -0.3746009833543293421, 1.005599061620507320E-08 ) ) ;
#35085=CARTESIAN_POINT ( 'NONE',  ( -17.33262245845742910, -7.759502110702281463, 67.30567542699309058 ) ) ;
#35088=CARTESIAN_POINT ( 'NONE',  ( -10.69329545470549547, -12.88639875208188634, 64.28338539888954983 ) ) ;
#35089=EDGE_LOOP ( 'NONE', ( #1078, #25116, #15230, #17457, #40334 ) ) ;
#35091=CARTESIAN_POINT ( 'NONE',  ( -13.18109041692693140, -9.241580129719441317, 67.37942828297590836 ) ) ;
#35092=ORIENTED_EDGE ( 'NONE', *, *, #2789, .T. ) ;
#35093=CARTESIAN_POINT ( 'NONE',  ( -22.88419851978063591, -10.42888047092867865, 63.07185995612697837 ) ) ;
#35094=FACE_BOUND ( 'NONE', #29243, .T. ) ;
#35095=ORIENTED_EDGE ( 'NONE', *, *, #15766, .T. ) ;
#35096=EDGE_CURVE ( 'NONE', #41338, #2641, #21311, .T. ) ;
#35098=EDGE_LOOP ( 'NONE', ( #3061, #13875 ) ) ;
#35099=ORIENTED_EDGE ( 'NONE', *, *, #2776, .F. ) ;
#35100=CARTESIAN_POINT ( 'NONE',  ( -10.03860189133040315, -15.79316336790978603, 61.15133701675058120 ) ) ;
#35101=DIRECTION ( 'NONE',  ( -0.4332512900281776380, 0.1108752438054599471, 0.8944271909999157444 ) ) ;
#35102=CARTESIAN_POINT ( 'NONE',  ( -22.82021534226488413, -10.26644114900146576, 70.31178585817200144 ) ) ;
#35103=CARTESIAN_POINT ( 'NONE',  ( -10.57136597998982985, -13.11950654315977793, 64.42403173677416817 ) ) ;
#35104=CARTESIAN_POINT ( 'NONE',  ( -13.34436364135905606, -9.120990523779875403, 60.63053345639304581 ) ) ;
#35107=EDGE_CURVE ( 'NONE', #43552, #2873, #42507, .T. ) ;
#35108=EDGE_CURVE ( 'NONE', #39476, #10157, #37687, .T. ) ;
#35110=EDGE_CURVE ( 'NONE', #8273, #33946, #22688, .T. ) ;
#35111=CARTESIAN_POINT ( 'NONE',  ( -22.61838138049972358, -19.58773617554900071, 69.32985287095068827 ) ) ;
#35112=CARTESIAN_POINT ( 'NONE',  ( -23.12302852889637705, -18.95946475466559633, 62.65406880579606508 ) ) ;
#35113=CYLINDRICAL_SURFACE ( 'NONE', #15097, 0.1499999999999991063 ) ;
#35114=EDGE_CURVE ( 'NONE', #13421, #23075, #2825, .T. ) ;
#35115=ORIENTED_EDGE ( 'NONE', *, *, #44212, .F. ) ;
#35118=AXIS2_PLACEMENT_3D ( 'NONE', #31799, #46818, #9876 ) ;
#35120=CARTESIAN_POINT ( 'NONE',  ( -23.08463366406817840, -10.68898790873936555, 59.83033381731064537 ) ) ;
#35121=EDGE_CURVE ( 'NONE', #29632, #188, #1314, .T. ) ;
#35122=CARTESIAN_POINT ( 'NONE',  ( -16.71957921250844592, -21.82421608262117729, 68.71032757591046902 ) ) ;
#35126=ORIENTED_EDGE ( 'NONE', *, *, #24414, .T. ) ;
#35127=CARTESIAN_POINT ( 'NONE',  ( -11.60677555321244547, -18.70493759839273906, 68.44519605431926834 ) ) ;
#35128=CARTESIAN_POINT ( 'NONE',  ( -22.76532612177806314, -10.19550891705927498, 73.62593845350987465 ) ) ;
#35129=CARTESIAN_POINT ( 'NONE',  ( -22.11926001268504294, -9.024814352312150234, 63.30658345311071855 ) ) ;
#35130=CARTESIAN_POINT ( 'NONE',  ( -12.05451961919647630, -9.643808529799599683, 57.20280282899455671 ) ) ;
#35132=CARTESIAN_POINT ( 'NONE',  ( -24.55871722839809834, -12.66422925090921225, 69.88747596251579353 ) ) ;
#35133=CARTESIAN_POINT ( 'NONE',  ( -24.83179309550701319, -15.60247978309782546, 73.19577886632693264 ) ) ;
#35134=CARTESIAN_POINT ( 'NONE',  ( -24.31823732957325745, -17.63313362019280106, 66.05861802595141796 ) ) ;
#35135=ORIENTED_EDGE ( 'NONE', *, *, #40586, .F. ) ;
#35136=CARTESIAN_POINT ( 'NONE',  ( -22.49805058420730219, -9.986866540729424813, 73.78161091687563555 ) ) ;
#35138=CARTESIAN_POINT ( 'NONE',  ( -19.24190894175819366, -7.584296403803404196, 63.54593838833191910 ) ) ;
#35140=ORIENTED_EDGE ( 'NONE', *, *, #6550, .F. ) ;
#35141=CARTESIAN_POINT ( 'NONE',  ( -16.36834346081282732, -22.18410778960565466, 61.94063409281806543 ) ) ;
#35143=CARTESIAN_POINT ( 'NONE',  ( -24.22177629109872399, -13.13842424187848934, 63.13264177643409880 ) ) ;
#35145=ORIENTED_EDGE ( 'NONE', *, *, #21868, .T. ) ;
#35147=CARTESIAN_POINT ( 'NONE',  ( -20.52762626839951210, -8.534807245883811788, 63.61121513079540080 ) ) ;
#35148=EDGE_CURVE ( 'NONE', #31941, #45590, #16002, .T. ) ;
#35149=CARTESIAN_POINT ( 'NONE',  ( -10.42257993575900876, -15.70014684107950842, 68.12200980565171449 ) ) ;
#35151=CARTESIAN_POINT ( 'NONE',  ( -12.83007281553047108, -20.09077549419061626, 71.80653676829817300 ) ) ;
#35153=B_SPLINE_CURVE_WITH_KNOTS ( 'NONE', 3,
 ( #7210, #33264, #14537, #41168, #18755, #10648, #44886, #3490, #21970, #45128 ),
 .UNSPECIFIED., .F., .F.,
 ( 4, 2, 2, 2, 4 ),
 ( 0.000000000000000000, 0.2500000000000000000, 0.5000000000000000000, 0.7500000000000000000, 1.000000000000000000 ),
 .UNSPECIFIED. ) ;
#35154=CARTESIAN_POINT ( 'NONE',  ( -21.78783678618839303, -8.770877803870156697, 70.38778484029896276 ) ) ;
#35155=ADVANCED_FACE ( 'NONE', ( #23176 ), #46062, .T. ) ;
#35156=ORIENTED_EDGE ( 'NONE', *, *, #14927, .T. ) ;
#35157=EDGE_LOOP ( 'NONE', ( #3518, #18207, #290, #17154, #10766 ) ) ;
#35158=CARTESIAN_POINT ( 'NONE',  ( -14.87246701381353198, -21.32764640494525210, 58.39291311840838006 ) ) ;
#35159=CARTESIAN_POINT ( 'NONE',  ( -20.04168780904239355, -21.30143565362524072, 72.41981212996954298 ) ) ;
#35163=CARTESIAN_POINT ( 'NONE',  ( -12.39467452642779044, -9.940348555453047297, 57.10438015346839791 ) ) ;
#35164=LINE ( 'NONE', #20649, #44044 ) ;
#35165=CARTESIAN_POINT ( 'NONE',  ( -17.28496127917699710, -14.43418371046636217, 56.49999999999994316 ) ) ;
#35167=VERTEX_POINT ( 'NONE', #38168 ) ;
#35168=EDGE_LOOP ( 'NONE', ( #3062, #33135, #16208, #36568, #45241 ) ) ;
#35169=CARTESIAN_POINT ( 'NONE',  ( -11.52915434062558120, -10.92788463621912420, 60.82318916367986361 ) ) ;
#35172=CARTESIAN_POINT ( 'NONE',  ( -12.60227155074094441, -19.95281705956671559, 68.35129494334645983 ) ) ;
#35173=CARTESIAN_POINT ( 'NONE',  ( -18.30726797983150789, -21.75326897020822514, 68.81514702557041119 ) ) ;
#35174=EDGE_CURVE ( 'NONE', #14220, #17691, #10128, .T. ) ;
#35175=( BOUNDED_CURVE ( )  B_SPLINE_CURVE ( 3, ( #15353, #14855, #38014, #33573 ),
 .UNSPECIFIED., .F., .F. ) 
 B_SPLINE_CURVE_WITH_KNOTS ( ( 4, 4 ),
 ( 0.5000000000000000000, 0.9074455897393662873 ),
 .UNSPECIFIED. ) 
 CURVE ( )  GEOMETRIC_REPRESENTATION_ITEM ( )  RATIONAL_B_SPLINE_CURVE ( ( 1.000000000000000666, 0.4567392136813310799, 0.3561768502900293232, 0.6983129098260962841 ) ) 
 REPRESENTATION_ITEM ( '' )  );
#35176=VERTEX_POINT ( 'NONE', #30816 ) ;
#35177=CARTESIAN_POINT ( 'NONE',  ( -14.99952990268716491, -21.37596734354964667, 61.92135132145442356 ) ) ;
#35178=CARTESIAN_POINT ( 'NONE',  ( -23.75068382698706770, -10.87373689121910658, 73.47537926597675551 ) ) ;
#35179=CARTESIAN_POINT ( 'NONE',  ( -17.39742496553465401, -7.759256980052345654, 67.02039592192090822 ) ) ;
#35180=CARTESIAN_POINT ( 'NONE',  ( -24.20601044598569374, -16.76383555912477874, 73.03903240339252534 ) ) ;
#35182=ORIENTED_EDGE ( 'NONE', *, *, #31418, .T. ) ;
#35183=( BOUNDED_SURFACE ( )  B_SPLINE_SURFACE ( 3, 1, ( 
 ( #3388, #33649 ),
 ( #3897, #22119 ),
 ( #18906, #29994 ),
 ( #37593, #10546 ),
 ( #40568, #26055 ),
 ( #29494, #36617 ),
 ( #40817, #17904 ) ),
 .UNSPECIFIED., .T., .F., .F. ) 
 B_SPLINE_SURFACE_WITH_KNOTS ( ( 4, 3, 4 ),
 ( 2, 2 ),
 ( 0.000000000000000000, 0.5000000000000000000, 1.000000000000000000 ),
 ( 0.000000000000000000, 1.000000000000000000 ),
 .UNSPECIFIED. ) 
 GEOMETRIC_REPRESENTATION_ITEM ( )  RATIONAL_B_SPLINE_SURFACE ( (
 ( 1.000000000000000000, 1.000000000000000000),
 ( 0.3333333333333335369, 0.3333333333333330373),
 ( 0.3333333333333335369, 0.3333333333333330373),
 ( 1.000000000000000000, 1.000000000000000000),
 ( 0.3333333333333333703, 0.3333333333333333703),
 ( 0.3333333333333333703, 0.3333333333333333703),
 ( 1.000000000000000000, 1.000000000000000000) ) ) 
 REPRESENTATION_ITEM ( '' )  SURFACE ( )  );
#35184=CARTESIAN_POINT ( 'NONE',  ( -20.13271805750754950, -8.299978134201072777, 70.53628287813307907 ) ) ;
#35185=VECTOR ( 'NONE', #41854, 1000.000000000000114 ) ;
#35186=CARTESIAN_POINT ( 'NONE',  ( -24.37817933763783529, -15.98629254845087466, 69.94796348494512017 ) ) ;
#35188=EDGE_LOOP ( 'NONE', ( #2147, #40449, #32281, #33819, #20212 ) ) ;
#35190=DIRECTION ( 'NONE',  ( -0.1261685609230672744, -0.9920088176193796459, -5.058037263227848996E-08 ) ) ;
#35191=CARTESIAN_POINT ( 'NONE',  ( -24.21863471429747250, -16.49938873345172397, 59.31259601734559794 ) ) ;
#35193=CARTESIAN_POINT ( 'NONE',  ( -14.09463846823036981, -8.088735815341543400, 53.49999999999994316 ) ) ;
#35195=EDGE_LOOP ( 'NONE', ( #37451, #11506, #45236, #2524, #41068 ) ) ;
#35197=CARTESIAN_POINT ( 'NONE',  ( -18.84068548446033731, -21.72355622379298978, 72.44077832767429470 ) ) ;
#35199=CARTESIAN_POINT ( 'NONE',  ( -15.18349748943555966, -8.120920323119461770, 56.94179993390997652 ) ) ;
#35200=CARTESIAN_POINT ( 'NONE',  ( -18.33016535318852291, -22.20398178282153623, 69.07160637178317586 ) ) ;
#35202=VERTEX_POINT ( 'NONE', #7927 ) ;
#35205=CARTESIAN_POINT ( 'NONE',  ( -10.61954745215241935, -11.77581898585687092, 74.75114390221474991 ) ) ;
#35206=CARTESIAN_POINT ( 'NONE',  ( -14.84927081153347039, -21.37251255130113137, 61.65072491673618771 ) ) ;
#35207=ORIENTED_EDGE ( 'NONE', *, *, #6395, .T. ) ;
#35208=CARTESIAN_POINT ( 'NONE',  ( -16.22920462672756159, -7.911818831816758824, 60.50028431019059383 ) ) ;
#35209=CARTESIAN_POINT ( 'NONE',  ( -11.81042834955647258, -10.54382735031610174, 74.45357240259568243 ) ) ;
#35211=CARTESIAN_POINT ( 'NONE',  ( -20.51563283865871057, -8.030886342657675314, 66.88765784730034625 ) ) ;
#35212=CARTESIAN_POINT ( 'NONE',  ( -12.65513433691805290, -20.00553804586020590, 64.75186297256590251 ) ) ;
#35214=VERTEX_POINT ( 'NONE', #37936 ) ;
#35215=CARTESIAN_POINT ( 'NONE',  ( -18.32882331211134286, -7.814473174497912566, 73.72575526123169709 ) ) ;
#35216=CARTESIAN_POINT ( 'NONE',  ( -11.00421863625541974, -17.72293202094342490, 71.86158434966563391 ) ) ;
#35217=ORIENTED_EDGE ( 'NONE', *, *, #17731, .T. ) ;
#35218=CARTESIAN_POINT ( 'NONE',  ( -15.82259747647940173, -7.533288219471245384, 67.25511999279136433 ) ) ;
#35221=CARTESIAN_POINT ( 'NONE',  ( -23.82760511577973617, -11.00139541567114421, 73.48476430283872673 ) ) ;
#35222=CARTESIAN_POINT ( 'NONE',  ( -10.84896266223257122, -17.37486770053218521, 71.71150890757306229 ) ) ;
#35225=EDGE_LOOP ( 'NONE', ( #22461, #46520 ) ) ;
#35228=CARTESIAN_POINT ( 'NONE',  ( -10.45582064790140464, -15.88054293009791706, 64.80211778324330396 ) ) ;
#35229=CARTESIAN_POINT ( 'NONE',  ( -19.83745867003831975, -21.38006599400703678, 68.94187494913028047 ) ) ;
#35230=DIRECTION ( 'NONE',  ( -0.6323592902076722311, -0.7746752403995150749, 4.984538757074984646E-08 ) ) ;
#35233=EDGE_LOOP ( 'NONE', ( #39447, #37182, #7849, #12837 ) ) ;
#35235=EDGE_CURVE ( 'NONE', #3060, #46704, #45377, .T. ) ;
#35237=CARTESIAN_POINT ( 'NONE',  ( -24.47697530877170990, -14.85041752174647733, 63.12785080464042409 ) ) ;
#35238=CARTESIAN_POINT ( 'NONE',  ( -24.11793993921729395, -12.76166543249827434, 70.07243002473258286 ) ) ;
#35239=EDGE_CURVE ( 'NONE', #16707, #18836, #43091, .T. ) ;
#35241=CARTESIAN_POINT ( 'NONE',  ( -10.82867520472564848, -11.34449427682889677, 67.73369198428547122 ) ) ;
#35242=CARTESIAN_POINT ( 'NONE',  ( -11.13733870171179596, -11.61806121328041996, 67.90392505421056057 ) ) ;
#35243=VERTEX_POINT ( 'NONE', #46563 ) ;
#35244=CARTESIAN_POINT ( 'NONE',  ( -20.95139844211411884, -8.247003834134126521, 59.96408367069768275 ) ) ;
#35245=CARTESIAN_POINT ( 'NONE',  ( -10.47144901298989694, -13.99582629904338127, 57.73359634450734745 ) ) ;
#35248=CARTESIAN_POINT ( 'NONE',  ( -19.86401518824997225, -21.42384811948916834, 69.22010401872219632 ) ) ;
#35249=CARTESIAN_POINT ( 'NONE',  ( -10.13336409668949400, -13.27690444941326042, 74.77843402251788518 ) ) ;
#35251=VECTOR ( 'NONE', #27764, 1000.000000000000227 ) ;
#35254=CARTESIAN_POINT ( 'NONE',  ( -24.47243858273885664, -15.17772250287404567, 59.38732937676161328 ) ) ;
#35255=CARTESIAN_POINT ( 'NONE',  ( -24.14679772577363437, -12.68507108172156705, 70.05770892828130059 ) ) ;
#35257=VERTEX_POINT ( 'NONE', #13036 ) ;
#35260=CARTESIAN_POINT ( 'NONE',  ( -24.08907074505709645, -11.48026357735065872, 63.13713704106291402 ) ) ;
#35263=CARTESIAN_POINT ( 'NONE',  ( -13.69528579949288982, -8.884502191640171631, 56.98584450146461222 ) ) ;
#35264=CARTESIAN_POINT ( 'NONE',  ( -22.79960237261627398, -9.650942640399760464, 73.66656521964461035 ) ) ;
#35265=CARTESIAN_POINT ( 'NONE',  ( -19.15893590421327985, -8.027528287274607877, 60.03381006258986474 ) ) ;
#35266=ORIENTED_EDGE ( 'NONE', *, *, #2116, .F. ) ;
#35268=CARTESIAN_POINT ( 'NONE',  ( -22.79734292848665334, -10.24514101169484448, 66.84182257473258915 ) ) ;
#35269=CARTESIAN_POINT ( 'NONE',  ( -24.86682742714664229, -14.47648176530652719, 66.34439218741853495 ) ) ;
#35270=CYLINDRICAL_SURFACE ( 'NONE', #48589, 0.1500000000000047407 ) ;
#35271=CARTESIAN_POINT ( 'NONE',  ( -24.86610167639389246, -14.46236660854407674, 66.29797298380238146 ) ) ;
#35273=ORIENTED_EDGE ( 'NONE', *, *, #21809, .T. ) ;
#35274=CARTESIAN_POINT ( 'NONE',  ( -15.40811923343077083, -21.56513327689926030, 72.06047564147742435 ) ) ;
#35276=ORIENTED_EDGE ( 'NONE', *, *, #30783, .F. ) ;
#35279=CARTESIAN_POINT ( 'NONE',  ( -17.96161316005734676, -22.23979900576015822, 62.07524705671683307 ) ) ;
#35280=CARTESIAN_POINT ( 'NONE',  ( -23.26642198590026211, -10.18619985444824572, 63.23332526816662380 ) ) ;
#35281=CARTESIAN_POINT ( 'NONE',  ( -16.26195973558533581, -21.76306465430365122, 58.57113428431811997 ) ) ;
#35285=CARTESIAN_POINT ( 'NONE',  ( -10.85164377074246289, -17.36018552090334310, 64.92179613810992578 ) ) ;
#35286=CARTESIAN_POINT ( 'NONE',  ( -12.13668540368383653, -10.14142895936130628, 60.44429485117178302 ) ) ;
#35287=EDGE_LOOP ( 'NONE', ( #22952, #26334 ) ) ;
#35289=B_SPLINE_CURVE_WITH_KNOTS ( 'NONE', 3,
 ( #46795, #31050, #8893, #19469, #770, #28069, #13039, #27593, #1484, #42132 ),
 .UNSPECIFIED., .F., .F.,
 ( 4, 2, 2, 2, 4 ),
 ( 0.1272669073657891059, 0.2522669073462849854, 0.3772669073267808093, 0.5022669073072767443, 0.6272669072877725682 ),
 .UNSPECIFIED. ) ;
#35290=CARTESIAN_POINT ( 'NONE',  ( -18.29367245688808552, -17.15309925898211318, 77.49999999999994316 ) ) ;
#35293=CARTESIAN_POINT ( 'NONE',  ( -13.80550519567689172, -20.80142258237229669, 65.00131257522635053 ) ) ;
#35294=CARTESIAN_POINT ( 'NONE',  ( -20.99070387547166661, -20.89051904145194527, 65.58453967743210455 ) ) ;
#35297=ORIENTED_EDGE ( 'NONE', *, *, #47404, .T. ) ;
#35300=EDGE_CURVE ( 'NONE', #38102, #21018, #4303, .T. ) ;
#35301=CARTESIAN_POINT ( 'NONE',  ( -18.68070144837527735, -7.415226739706412218, 47.99999999999994316 ) ) ;
#35303=DIRECTION ( 'NONE',  ( 6.385196549736874992E-06, -5.147825522337142951E-06, 0.9999999999663644612 ) ) ;
#35304=VECTOR ( 'NONE', #39575, 1000.000000000000000 ) ;
#35305=CARTESIAN_POINT ( 'NONE',  ( -22.97880759471717838, -10.54929209374549082, 59.60203382397228467 ) ) ;
#35307=FACE_OUTER_BOUND ( 'NONE', #44887, .T. ) ;
#35308=CARTESIAN_POINT ( 'NONE',  ( -18.45262242793555885, -21.79183460504582470, 65.50099240037707204 ) ) ;
#35310=ORIENTED_EDGE ( 'NONE', *, *, #6550, .T. ) ;
#35311=CARTESIAN_POINT ( 'NONE',  ( -22.37417161799345777, -19.75879703283636957, 69.17417994536339165 ) ) ;
#35312=ADVANCED_FACE ( 'NONE', ( #27588 ), #42627, .T. ) ;
#35315=ORIENTED_EDGE ( 'NONE', *, *, #14484, .F. ) ;
#35316=CARTESIAN_POINT ( 'NONE',  ( -10.60402983012795808, -16.62626367578652520, 57.83193508283319773 ) ) ;
#35318=ADVANCED_FACE ( 'NONE', ( #5435 ), #5909, .T. ) ;
#35319=ORIENTED_EDGE ( 'NONE', *, *, #39347, .T. ) ;
#35321=CARTESIAN_POINT ( 'NONE',  ( -13.88293547364789049, -20.90532801101632643, 68.75625136993008368 ) ) ;
#35323=CARTESIAN_POINT ( 'NONE',  ( -21.89264518680100835, -20.26253109894388160, 58.77915004610761684 ) ) ;
#35326=CARTESIAN_POINT ( 'NONE',  ( -21.79997194174348607, -9.271457673084677609, 70.27565669584988939 ) ) ;
#35327=ORIENTED_EDGE ( 'NONE', *, *, #10436, .F. ) ;
#35328=DIRECTION ( 'NONE',  ( -6.865757635625664415E-07, -1.412849153005328843E-06, -0.9999999999987663202 ) ) ;
#35330=( BOUNDED_SURFACE ( )  B_SPLINE_SURFACE ( 3, 1, ( 
 ( #28425, #31633 ),
 ( #9718, #35790 ),
 ( #42721, #46412 ),
 ( #16344, #31136 ),
 ( #38764, #16828 ),
 ( #35063, #13128 ),
 ( #46656, #5539 ) ),
 .UNSPECIFIED., .T., .F., .F. ) 
 B_SPLINE_SURFACE_WITH_KNOTS ( ( 4, 3, 4 ),
 ( 2, 2 ),
 ( 0.000000000000000000, 0.5000000000000000000, 1.000000000000000000 ),
 ( 0.000000000000000000, 1.000000000000000000 ),
 .UNSPECIFIED. ) 
 GEOMETRIC_REPRESENTATION_ITEM ( )  RATIONAL_B_SPLINE_SURFACE ( (
 ( 1.000000000000000000, 1.000000000000000000),
 ( 0.3333333333333335369, 0.3333333333333330373),
 ( 0.3333333333333335369, 0.3333333333333330373),
 ( 1.000000000000000000, 1.000000000000000000),
 ( 0.3333333333333333703, 0.3333333333333333703),
 ( 0.3333333333333333703, 0.3333333333333333703),
 ( 1.000000000000000000, 1.000000000000000000) ) ) 
 REPRESENTATION_ITEM ( '' )  SURFACE ( )  );
#35332=AXIS2_PLACEMENT_3D ( 'NONE', #21233, #36233, #17993 ) ;
#35333=CARTESIAN_POINT ( 'NONE',  ( -11.24322483140283069, -11.41063336453235166, 60.88705523236457395 ) ) ;
#35334=FACE_BOUND ( 'NONE', #21339, .T. ) ;
#35339=CARTESIAN_POINT ( 'NONE',  ( -23.71751471349159601, -11.63122711669449494, 63.23746208799618529 ) ) ;
#35341=ORIENTED_EDGE ( 'NONE', *, *, #35447, .T. ) ;
#35345=CARTESIAN_POINT ( 'NONE',  ( -19.97013658168673800, -21.81073013994861398, 68.97836559665680056 ) ) ;
#35347=CARTESIAN_POINT ( 'NONE',  ( -12.74071866071660075, -9.015263582886822391, 70.96429948631303830 ) ) ;
#35348=ORIENTED_EDGE ( 'NONE', *, *, #3044, .T. ) ;
#35349=EDGE_CURVE ( 'NONE', #37778, #6964, #44858, .T. ) ;
#35350=VERTEX_POINT ( 'NONE', #25349 ) ;
#35352=CARTESIAN_POINT ( 'NONE',  ( -10.51729497052148155, -16.22293520194095962, 71.74750383215044280 ) ) ;
#35353=CARTESIAN_POINT ( 'NONE',  ( -24.43851978893111365, -14.10038870526526722, 73.12831301160871078 ) ) ;
#35356=CARTESIAN_POINT ( 'NONE',  ( -13.34492810635830651, -9.120585717833787243, 60.54836177336171943 ) ) ;
#35358=VERTEX_POINT ( 'NONE', #25583 ) ;
#35360=CARTESIAN_POINT ( 'NONE',  ( -13.71338950266841650, -20.80363499509022773, 64.98628881289567971 ) ) ;
#35362=FACE_OUTER_BOUND ( 'NONE', #20187, .T. ) ;
#35363=FACE_OUTER_BOUND ( 'NONE', #34207, .T. ) ;
#35366=VERTEX_POINT ( 'NONE', #14464 ) ;
#35367=CARTESIAN_POINT ( 'NONE',  ( -10.93232766038821424, -17.55941949638709687, 68.38249893951126523 ) ) ;
#35368=FACE_OUTER_BOUND ( 'NONE', #20715, .T. ) ;
#35369=VERTEX_POINT ( 'NONE', #32494 ) ;
#35370=CARTESIAN_POINT ( 'NONE',  ( -11.71918404020638427, -18.95175453447548009, 71.70158022526054253 ) ) ;
#35371=CARTESIAN_POINT ( 'NONE',  ( -9.973354012397450674, -14.79738236791871664, 71.44127436690867228 ) ) ;
#35372=LINE ( 'NONE', #6064, #32064 ) ;
#35374=ADVANCED_FACE ( 'NONE', ( #7131 ), #47995, .T. ) ;
#35375=CARTESIAN_POINT ( 'NONE',  ( -22.43322805121811214, -20.32484237088842249, 65.89077003248591780 ) ) ;
#35377=CARTESIAN_POINT ( 'NONE',  ( -24.27331421978716364, -11.70866763410274913, 53.76227901944321275 ) ) ;
#35378=CARTESIAN_POINT ( 'NONE',  ( -20.12289019246589206, -7.865124395032225380, 73.90592041591946781 ) ) ;
#35380=PLANE ( 'NONE',  #33798 ) ;
#35381=ORIENTED_EDGE ( 'NONE', *, *, #34504, .T. ) ;
#35382=CARTESIAN_POINT ( 'NONE',  ( -18.50498591074712706, -7.838904286686645406, 70.57887743023405847 ) ) ;
#35383=EDGE_CURVE ( 'NONE', #18814, #35636, #24879, .T. ) ;
#35384=EDGE_CURVE ( 'NONE', #7607, #15639, #4922, .T. ) ;
#35385=CARTESIAN_POINT ( 'NONE',  ( -23.76104667403178894, -10.32500873748839787, 54.49999999999995026 ) ) ;
#35387=FACE_OUTER_BOUND ( 'NONE', #17791, .T. ) ;
#35388=CARTESIAN_POINT ( 'NONE',  ( -10.40181215838624240, -12.32098906055858478, 57.37211424251319158 ) ) ;
#35389=CARTESIAN_POINT ( 'NONE',  ( -24.20371252810814866, -12.87440185077122834, 66.58774614429587757 ) ) ;
#35390=AXIS2_PLACEMENT_3D ( 'NONE', #37117, #30505, #15691 ) ;
#35392=ORIENTED_EDGE ( 'NONE', *, *, #26898, .F. ) ;
#35393=CARTESIAN_POINT ( 'NONE',  ( -11.01197672498280866, -17.74032467813711378, 71.85246142747085685 ) ) ;
#35394=AXIS2_PLACEMENT_3D ( 'NONE', #43635, #25154, #35731 ) ;
#35395=CARTESIAN_POINT ( 'NONE',  ( -20.84966316371748363, -20.97445663613623523, 58.52986464729110594 ) ) ;
#35396=CARTESIAN_POINT ( 'NONE',  ( -10.53876648713876740, -16.36073154998923229, 68.13334680848100788 ) ) ;
#35397=ORIENTED_EDGE ( 'NONE', *, *, #43993, .T. ) ;
#35398=CARTESIAN_POINT ( 'NONE',  ( -15.75439910800316845, -7.548642891367095764, 67.18361323375314953 ) ) ;
#35400=CARTESIAN_POINT ( 'NONE',  ( -21.78913871579879569, -8.771809629715434653, 70.24637254705723421 ) ) ;
#35403=ORIENTED_EDGE ( 'NONE', *, *, #14205, .T. ) ;
#35404=CARTESIAN_POINT ( 'NONE',  ( -23.83724620116612058, -11.87385095858915207, 63.36706934938042934 ) ) ;
#35405=CARTESIAN_POINT ( 'NONE',  ( -20.04136243794045313, -21.30156843505427489, 72.69013421047081636 ) ) ;
#35406=CARTESIAN_POINT ( 'NONE',  ( -10.42707437396587800, -14.56501430223373106, 71.39952884310628178 ) ) ;
#35410=CARTESIAN_POINT ( 'NONE',  ( -12.36127418495607877, -19.64332424046381576, 57.99970467312913058 ) ) ;
#35411=CARTESIAN_POINT ( 'NONE',  ( -19.76620107553464933, -21.88153087662584895, 65.57147903976517966 ) ) ;
#35412=CARTESIAN_POINT ( 'NONE',  ( -16.78341213209640159, -22.23169296657789928, 68.88056055876903372 ) ) ;
#35413=ORIENTED_EDGE ( 'NONE', *, *, #34226, .F. ) ;
#35415=CARTESIAN_POINT ( 'NONE',  ( -12.34237343482028670, -20.25724347209099818, 68.49803924141983202 ) ) ;
#35417=CARTESIAN_POINT ( 'NONE',  ( -24.55871722839809834, -12.66422925090921225, 69.88747596251579353 ) ) ;
#35418=( BOUNDED_CURVE ( )  B_SPLINE_CURVE ( 3, ( #18608, #9853, #10088, #45238 ),
 .UNSPECIFIED., .F., .F. ) 
 B_SPLINE_CURVE_WITH_KNOTS ( ( 4, 4 ),
 ( 0.9074455897393695070, 1.000000000000000000 ),
 .UNSPECIFIED. ) 
 CURVE ( )  GEOMETRIC_REPRESENTATION_ITEM ( )  RATIONAL_B_SPLINE_CURVE ( ( 0.6983129098261139367, 0.7760317562607162989, 0.8765941196520116163, 1.000000000000000000 ) ) 
 REPRESENTATION_ITEM ( '' )  );
#35421=CARTESIAN_POINT ( 'NONE',  ( -19.92776479198160189, -21.39998277484045275, 72.41950795000725805 ) ) ;
#35423=VECTOR ( 'NONE', #34728, 1000.000000000000000 ) ;
#35428=CARTESIAN_POINT ( 'NONE',  ( -23.51785832295892931, -11.36449550514380036, 69.89210750611785272 ) ) ;
#35429=DIRECTION ( 'NONE',  ( -0.3478314405900307937, -0.9375570856950865561, 0.000000000000000000 ) ) ;
#35430=EDGE_CURVE ( 'NONE', #38940, #34024, #2555, .T. ) ;
#35431=CARTESIAN_POINT ( 'NONE',  ( -24.42401644153718721, -14.84212863923847081, 59.24300237020570137 ) ) ;
#35432=VECTOR ( 'NONE', #47180, 1000.000000000000000 ) ;
#35434=CARTESIAN_POINT ( 'NONE',  ( -24.25171796977671335, -16.35308120058899206, 59.42332432118549690 ) ) ;
#35436=FACE_OUTER_BOUND ( 'NONE', #15720, .T. ) ;
#35437=ORIENTED_EDGE ( 'NONE', *, *, #11263, .F. ) ;
#35438=ADVANCED_FACE ( 'NONE', ( #43837 ), #36891, .T. ) ;
#35439=CARTESIAN_POINT ( 'NONE',  ( -19.24931602816760190, -7.586122295205923294, 63.55372364550890296 ) ) ;
#35440=CARTESIAN_POINT ( 'NONE',  ( -18.76558283008973049, -7.480892646508040755, 70.55563411965815135 ) ) ;
#35441=ORIENTED_EDGE ( 'NONE', *, *, #37879, .F. ) ;
#35442=CARTESIAN_POINT ( 'NONE',  ( -13.88293403466071396, -20.90532716339074781, 68.60625136993937190 ) ) ;
#35444=EDGE_CURVE ( 'NONE', #1437, #45729, #33289, .T. ) ;
#35447=EDGE_CURVE ( 'NONE', #37610, #21448, #40131, .T. ) ;
#35448=CARTESIAN_POINT ( 'NONE',  ( -15.16478962180274870, -8.127860897350485558, 57.26488623981089177 ) ) ;
#35449=CARTESIAN_POINT ( 'NONE',  ( -13.49267557974227394, -8.956801037788498121, 60.45422421514565059 ) ) ;
#35452=CARTESIAN_POINT ( 'NONE',  ( -10.85841931818429629, -17.37798394237199062, 64.91267318220633342 ) ) ;
#35454=CARTESIAN_POINT ( 'NONE',  ( -21.15336808330806662, -20.73310000539657949, 69.35450185099439580 ) ) ;
#35455=CARTESIAN_POINT ( 'NONE',  ( -12.15299190543910512, -20.07505386821981119, 65.05330132703942070 ) ) ;
#35456=VERTEX_POINT ( 'NONE', #238 ) ;
#35457=ORIENTED_EDGE ( 'NONE', *, *, #6757, .T. ) ;
#35458=CARTESIAN_POINT ( 'NONE',  ( -24.11881394502254849, -17.01995806294775448, 73.16863963025599560 ) ) ;
#35459=VERTEX_POINT ( 'NONE', #7870 ) ;
#35460=CARTESIAN_POINT ( 'NONE',  ( -24.33993967182187035, -15.89175611583846681, 66.07827301765077266 ) ) ;
#35463=( BOUNDED_CURVE ( )  B_SPLINE_CURVE ( 3, ( #37379, #2696, #36898, #26325 ),
 .UNSPECIFIED., .F., .F. ) 
 B_SPLINE_CURVE_WITH_KNOTS ( ( 4, 4 ),
 ( 0.000000000000000000, 0.4074455897393662873 ),
 .UNSPECIFIED. ) 
 CURVE ( )  GEOMETRIC_REPRESENTATION_ITEM ( )  RATIONAL_B_SPLINE_CURVE ( ( 1.000000000000000000, 0.4567392136813298587, 0.3561768502900295452, 0.6983129098260991707 ) ) 
 REPRESENTATION_ITEM ( '' )  );
#35464=DIRECTION ( 'NONE',  ( -5.731567514496413899E-31, -1.020425574103664789E-16, -1.000000000000000000 ) ) ;
#35465=CYLINDRICAL_SURFACE ( 'NONE', #7407, 0.1500000000000010769 ) ;
#35467=EDGE_LOOP ( 'NONE', ( #9207, #24776, #2041, #39056, #39871 ) ) ;
#35468=CARTESIAN_POINT ( 'NONE',  ( -22.94346461125903147, -10.41716915086503725, 66.63362387568147938 ) ) ;
#35469=CARTESIAN_POINT ( 'NONE',  ( -13.00192122862099531, -8.813424762390464906, 64.06979850922034814 ) ) ;
#35470=AXIS2_PLACEMENT_3D ( 'NONE', #39180, #38702, #4983 ) ;
#35471=CARTESIAN_POINT ( 'NONE',  ( -24.03160971261424805, -17.26750559640275640, 69.71339792588547368 ) ) ;
#35472=CARTESIAN_POINT ( 'NONE',  ( -12.97018521796328017, -9.340428432532196013, 74.73411830381819243 ) ) ;
#35474=B_SPLINE_CURVE_WITH_KNOTS ( 'NONE', 3,
 ( #2632, #17405, #28505, #2144, #3111, #28741, #36827, #21364, #32438, #17145 ),
 .UNSPECIFIED., .F., .F.,
 ( 4, 2, 2, 2, 4 ),
 ( 0.000000000000000000, 0.2500000000000000000, 0.5000000000000000000, 0.7500000000000000000, 1.000000000000000000 ),
 .UNSPECIFIED. ) ;
#35475=( BOUNDED_CURVE ( )  B_SPLINE_CURVE ( 3, ( #42969, #35333, #21299, #28914 ),
 .UNSPECIFIED., .F., .F. ) 
 B_SPLINE_CURVE_WITH_KNOTS ( ( 4, 4 ),
 ( 0.000000000000000000, 0.4074455897393631787 ),
 .UNSPECIFIED. ) 
 CURVE ( )  GEOMETRIC_REPRESENTATION_ITEM ( )  RATIONAL_B_SPLINE_CURVE ( ( 1.000000000000000000, 0.4567392136813281378, 0.3561768502900288791, 0.6983129098261022794 ) ) 
 REPRESENTATION_ITEM ( '' )  );
#35476=ORIENTED_EDGE ( 'NONE', *, *, #27195, .F. ) ;
#35479=CARTESIAN_POINT ( 'NONE',  ( -23.28921155407422106, -22.22116534042542213, 53.49999999999995026 ) ) ;
#35480=AXIS2_PLACEMENT_3D ( 'NONE', #40296, #35852, #13195 ) ;
#35482=CARTESIAN_POINT ( 'NONE',  ( -21.74938187378823784, -9.305322344061284667, 63.47688388556134242 ) ) ;
#35483=B_SPLINE_CURVE_WITH_KNOTS ( 'NONE', 3,
 ( #10010, #16894, #14154, #47201, #20621, #10264, #6317, #2850, #39563, #46948 ),
 .UNSPECIFIED., .F., .F.,
 ( 4, 2, 2, 2, 4 ),
 ( 0.000000000000000000, 0.2500000000000000000, 0.5000000000000000000, 0.7500000000000000000, 1.000000000000000000 ),
 .UNSPECIFIED. ) ;
#35484=EDGE_CURVE ( 'NONE', #21822, #2374, #213, .T. ) ;
#35488=CARTESIAN_POINT ( 'NONE',  ( -10.42131017383741032, -15.64935787052201910, 57.45304097017945111 ) ) ;
#35490=B_SPLINE_CURVE_WITH_KNOTS ( 'NONE', 3,
 ( #25500, #40512, #43999, #40755, #47912, #40044, #6059, #6789, #33106, #6310 ),
 .UNSPECIFIED., .F., .F.,
 ( 4, 2, 2, 2, 4 ),
 ( 0.000000000000000000, 0.2500000000000000000, 0.5000000000000000000, 0.7500000000000000000, 1.000000000000000000 ),
 .UNSPECIFIED. ) ;
#35491=AXIS2_PLACEMENT_3D ( 'NONE', #42924, #34549, #833 ) ;
#35493=CARTESIAN_POINT ( 'NONE',  ( -23.78474285830518653, -17.73496384451835794, 62.70190779623644062 ) ) ;
#35494=ORIENTED_EDGE ( 'NONE', *, *, #33812, .F. ) ;
#35496=VERTEX_POINT ( 'NONE', #11796 ) ;
#35497=FACE_OUTER_BOUND ( 'NONE', #9254, .T. ) ;
#35498=ORIENTED_EDGE ( 'NONE', *, *, #44962, .F. ) ;
#35499=CARTESIAN_POINT ( 'NONE',  ( -24.87385082706414607, -14.87839859077033822, 59.49946141495512819 ) ) ;
#35501=CARTESIAN_POINT ( 'NONE',  ( -19.30706997687812887, -22.01740875295033462, 58.64012098774584558 ) ) ;
#35502=VERTEX_POINT ( 'NONE', #26566 ) ;
#35504=CARTESIAN_POINT ( 'NONE',  ( -24.70168866369219529, -16.40345363474641260, 59.28365756255518448 ) ) ;
#35505=EDGE_CURVE ( 'NONE', #16942, #38159, #17909, .T. ) ;
#35508=ADVANCED_FACE ( 'NONE', ( #11541 ), #33941, .T. ) ;
#35510=CARTESIAN_POINT ( 'NONE',  ( -10.46835785932885621, -15.59614926455694572, 61.03789074737235154 ) ) ;
#35511=B_SPLINE_CURVE_WITH_KNOTS ( 'NONE', 1,
 ( #32835, #22256 ),
 .UNSPECIFIED., .F., .F.,
 ( 2, 2 ),
 ( 0.000000000000000000, 1.000000000000000000 ),
 .UNSPECIFIED. ) ;
#35512=LINE ( 'NONE', #31824, #29783 ) ;
#35513=ORIENTED_EDGE ( 'NONE', *, *, #44427, .F. ) ;
#35514=PLANE ( 'NONE',  #23936 ) ;
#35515=CARTESIAN_POINT ( 'NONE',  ( -13.01616685277437568, -9.306763517318225709, 70.86397465682092900 ) ) ;
#35516=DIRECTION ( 'NONE',  ( -0.9893521221787096032, 0.1455416721783832079, 6.188545272020283923E-08 ) ) ;
#35518=EDGE_CURVE ( 'NONE', #39956, #15214, #35928, .T. ) ;
#35519=CARTESIAN_POINT ( 'NONE',  ( -19.97164353606484255, -21.81018995992316079, 69.11977899231902711 ) ) ;
#35521=AXIS2_PLACEMENT_3D ( 'NONE', #18477, #48281, #14283 ) ;
#35522=EDGE_LOOP ( 'NONE', ( #36590, #5935, #33274, #6621 ) ) ;
#35525=CARTESIAN_POINT ( 'NONE',  ( -11.52461732454066023, -18.67456722079397125, 68.63178522425482697 ) ) ;
#35528=CARTESIAN_POINT ( 'NONE',  ( -23.09608884140482132, -18.99645705127922923, 62.35966695639078239 ) ) ;
#35530=EDGE_CURVE ( 'NONE', #8372, #11939, #26531, .T. ) ;
#35531=VERTEX_POINT ( 'NONE', #12035 ) ;
#35532=CARTESIAN_POINT ( 'NONE',  ( -12.09375059738624714, -9.604167670197291784, 57.22789050401003408 ) ) ;
#35533=FACE_OUTER_BOUND ( 'NONE', #40742, .T. ) ;
#35534=VECTOR ( 'NONE', #22597, 1000.000000000000114 ) ;
#35536=EDGE_LOOP ( 'NONE', ( #8736, #4252, #39389, #4789, #21093 ) ) ;
#35537=CARTESIAN_POINT ( 'NONE',  ( -17.22121256223034536, -7.361891212656819228, 70.74681744497029001 ) ) ;
#35542=CARTESIAN_POINT ( 'NONE',  ( -20.95545100651803594, -20.91135505560678354, 65.59926067308570907 ) ) ;
#35543=ORIENTED_EDGE ( 'NONE', *, *, #25497, .F. ) ;
#35546=DIRECTION ( 'NONE',  ( 0.8603613874411337736, -0.3191920208248667512, 0.3973597071195127395 ) ) ;
#35547=CARTESIAN_POINT ( 'NONE',  ( -14.11518482969570876, -8.134170225034605295, 70.89104128859074194 ) ) ;
#35548=EDGE_CURVE ( 'NONE', #18372, #4771, #4815, .T. ) ;
#35549=PLANE ( 'NONE',  #46905 ) ;
#35550=CARTESIAN_POINT ( 'NONE',  ( -23.77487038158592014, -11.74745262826995429, 62.96690348473899235 ) ) ;
#35551=DIRECTION ( 'NONE',  ( -7.110378524392051906E-06, -9.728165310344191876E-06, 0.9999999999274027385 ) ) ;
#35552=EDGE_LOOP ( 'NONE', ( #4134, #27139, #4152, #8540, #4033 ) ) ;
#35554=CARTESIAN_POINT ( 'NONE',  ( -21.57946453887431204, -8.565578233975859490, 54.27966884056655061 ) ) ;
#35555=ORIENTED_EDGE ( 'NONE', *, *, #32635, .F. ) ;
#35556=CARTESIAN_POINT ( 'NONE',  ( -24.18037252889021005, -17.94870914462638822, 59.18873732074431615 ) ) ;
#35558=VERTEX_POINT ( 'NONE', #18671 ) ;
#35559=CARTESIAN_POINT ( 'NONE',  ( -17.63866254341385442, -7.362211269489866261, 63.66561597723832477 ) ) ;
#35560=CARTESIAN_POINT ( 'NONE',  ( -18.63519442141342353, -21.70370385402750912, 72.51184200825215953 ) ) ;
#35562=CARTESIAN_POINT ( 'NONE',  ( -18.19389434033494268, -22.21941471489327569, 65.53027570717884487 ) ) ;
#35563=ADVANCED_FACE ( 'NONE', ( #45539 ), #38336, .T. ) ;
#35564=CARTESIAN_POINT ( 'NONE',  ( -12.01648161716052776, -10.28590799842451098, 67.79896869921920199 ) ) ;
#35565=B_SPLINE_CURVE_WITH_KNOTS ( 'NONE', 3,
 ( #32802, #22221, #47831, #21729, #18013, #33033, #26645, #15290, #34503, #45618 ),
 .UNSPECIFIED., .F., .F.,
 ( 4, 2, 2, 2, 4 ),
 ( 0.1272669073658538319, 0.2522669073463332245, 0.3772669073268126727, 0.5022669073072920654, 0.6272669072877714580 ),
 .UNSPECIFIED. ) ;
#35566=B_SPLINE_CURVE_WITH_KNOTS ( 'NONE', 1,
 ( #5417, #23894 ),
 .UNSPECIFIED., .F., .F.,
 ( 2, 2 ),
 ( 0.000000000000000000, 1.000000000000000000 ),
 .UNSPECIFIED. ) ;
#35568=CARTESIAN_POINT ( 'NONE',  ( -8.039996143071578061, -9.893874759132541996, 53.49999999999995026 ) ) ;
#35569=ORIENTED_EDGE ( 'NONE', *, *, #12366, .T. ) ;
#35570=CARTESIAN_POINT ( 'NONE',  ( -10.62096356601691660, -12.92974252456203743, 60.95420737114066156 ) ) ;
#35572=CARTESIAN_POINT ( 'NONE',  ( -11.05863916172663330, -11.77843433669154827, 71.38301090529685666 ) ) ;
#35573=EDGE_CURVE ( 'NONE', #3501, #12328, #8977, .T. ) ;
#35574=CARTESIAN_POINT ( 'NONE',  ( -18.77534723317123877, -22.20510239617831516, 54.02312124697527906 ) ) ;
#35575=CARTESIAN_POINT ( 'NONE',  ( -22.04378365035703879, -20.13510231884741231, 62.24911246861644543 ) ) ;
#35577=VERTEX_POINT ( 'NONE', #41334 ) ;
#35581=B_SPLINE_CURVE_WITH_KNOTS ( 'NONE', 3,
 ( #12748, #15943, #944, #42793, #46245, #30986, #19898, #23118, #38346, #4390 ),
 .UNSPECIFIED., .F., .F.,
 ( 4, 2, 2, 2, 4 ),
 ( 0.6272669072878013230, 0.7522669073073041668, 0.8772669073268071216, 1.002266907346309965, 1.127266907365812809 ),
 .UNSPECIFIED. ) ;
#35582=VERTEX_POINT ( 'NONE', #44805 ) ;
#35583=CARTESIAN_POINT ( 'NONE',  ( -19.60932529797995727, -21.51514414075818493, 69.34971148877966129 ) ) ;
#35584=ORIENTED_EDGE ( 'NONE', *, *, #38689, .F. ) ;
#35589=CARTESIAN_POINT ( 'NONE',  ( -17.38444741023572959, -7.359303210311908927, 67.22028379401484699 ) ) ;
#35591=CARTESIAN_POINT ( 'NONE',  ( -17.04413539470109740, -21.84925844046378174, 72.45071136019464575 ) ) ;
#35592=CARTESIAN_POINT ( 'NONE',  ( -23.48344415125163565, -18.41350569598871090, 73.04896097104848707 ) ) ;
#35597=EDGE_CURVE ( 'NONE', #31055, #7816, #25389, .T. ) ;
#35598=CARTESIAN_POINT ( 'NONE',  ( -21.48052744822966531, -21.05892743585564375, 72.71101825924023387 ) ) ;
#35599=CARTESIAN_POINT ( 'NONE',  ( -12.61628475940923089, -19.96571365470544990, 68.34217200571772821 ) ) ;
#35600=( BOUNDED_CURVE ( )  B_SPLINE_CURVE ( 3, ( #28915, #2806, #28447, #32836 ),
 .UNSPECIFIED., .F., .F. ) 
 B_SPLINE_CURVE_WITH_KNOTS ( ( 4, 4 ),
 ( 0.4074455897393610138, 0.5000000000000000000 ),
 .UNSPECIFIED. ) 
 CURVE ( )  GEOMETRIC_REPRESENTATION_ITEM ( )  RATIONAL_B_SPLINE_CURVE ( ( 0.6983129098260827394, 0.7760317562607027542, 0.8765941196520123935, 1.000000000000021316 ) ) 
 REPRESENTATION_ITEM ( '' )  );
#35603=FACE_OUTER_BOUND ( 'NONE', #524, .T. ) ;
#35605=DIRECTION ( 'NONE',  ( 0.8017593358536257986, 0.5976470257363775129, -1.209213344958501974E-07 ) ) ;
#35607=CARTESIAN_POINT ( 'NONE',  ( -11.73051513911133981, -18.96706119963912940, 71.69245704744217562 ) ) ;
#35608=( BOUNDED_SURFACE ( )  B_SPLINE_SURFACE ( 3, 1, ( 
 ( #427, #48187 ),
 ( #14417, #41288 ),
 ( #7573, #29478 ),
 ( #44508, #12224 ),
 ( #23562, #45741 ),
 ( #19865, #27001 ),
 ( #15904, #27244 ) ),
 .UNSPECIFIED., .T., .F., .F. ) 
 B_SPLINE_SURFACE_WITH_KNOTS ( ( 4, 3, 4 ),
 ( 2, 2 ),
 ( 0.000000000000000000, 0.5000000000000000000, 1.000000000000000000 ),
 ( 0.000000000000000000, 1.000000000000000000 ),
 .UNSPECIFIED. ) 
 GEOMETRIC_REPRESENTATION_ITEM ( )  RATIONAL_B_SPLINE_SURFACE ( (
 ( 1.000000000000000000, 1.000000000000000000),
 ( 0.3333333333333335369, 0.3333333333333330373),
 ( 0.3333333333333335369, 0.3333333333333330373),
 ( 1.000000000000000000, 1.000000000000000000),
 ( 0.3333333333333333703, 0.3333333333333333703),
 ( 0.3333333333333333703, 0.3333333333333333703),
 ( 1.000000000000000000, 1.000000000000000000) ) ) 
 REPRESENTATION_ITEM ( '' )  SURFACE ( )  );
#35609=CARTESIAN_POINT ( 'NONE',  ( -10.37821464302998109, -14.49231327520767465, 71.74271303568544056 ) ) ;
#35610=CARTESIAN_POINT ( 'NONE',  ( -10.41531639268335496, -14.04517892474411589, 60.93293405735092705 ) ) ;
#35612=AXIS2_PLACEMENT_3D ( 'NONE', #15874, #11706, #46173 ) ;
#35614=CARTESIAN_POINT ( 'NONE',  ( -10.92750425249182022, -11.16255029878774252, 64.26386639478288032 ) ) ;
#35615=B_SPLINE_CURVE_WITH_KNOTS ( 'NONE', 3,
 ( #24125, #28546, #5664, #35668, #35909, #25747, #1951, #16948, #17194, #31994 ),
 .UNSPECIFIED., .F., .F.,
 ( 4, 2, 2, 2, 4 ),
 ( 0.000000000000000000, 0.2500000000000000000, 0.5000000000000000000, 0.7500000000000000000, 1.000000000000000000 ),
 .UNSPECIFIED. ) ;
#35616=DIRECTION ( 'NONE',  ( 0.8083598999316399247, 0.5886886037477750966, 6.671815825018553389E-08 ) ) ;
#35617=ORIENTED_EDGE ( 'NONE', *, *, #44602, .F. ) ;
#35621=CARTESIAN_POINT ( 'NONE',  ( -9.974346092350561577, -14.73447246694985147, 71.44969959282907723 ) ) ;
#35622=CARTESIAN_POINT ( 'NONE',  ( -9.982343128696857804, -14.45766102835504263, 68.05138424084104543 ) ) ;
#35623=EDGE_LOOP ( 'NONE', ( #17292, #46663 ) ) ;
#35624=EDGE_CURVE ( 'NONE', #16796, #39956, #26421, .T. ) ;
#35625=CARTESIAN_POINT ( 'NONE',  ( -10.68602809008750576, -16.88409676349039046, 57.70232650191087487 ) ) ;
#35626=CARTESIAN_POINT ( 'NONE',  ( -21.80761086145510674, -20.26839064256230571, 58.83613193677467734 ) ) ;
#35629=ORIENTED_EDGE ( 'NONE', *, *, #4482, .F. ) ;
#35630=CARTESIAN_POINT ( 'NONE',  ( -10.90176001668674743, -17.49323270848192635, 71.98206789237249836 ) ) ;
#35632=CARTESIAN_POINT ( 'NONE',  ( -15.17160733334415212, -8.120315110694912519, 74.23552617732688930 ) ) ;
#35634=CARTESIAN_POINT ( 'NONE',  ( -17.62621216070176544, -7.758391551400871222, 67.32039556304484051 ) ) ;
#35636=VERTEX_POINT ( 'NONE', #42801 ) ;
#35638=CARTESIAN_POINT ( 'NONE',  ( -24.45634967269333160, -15.35895078922937529, 73.00303538218732058 ) ) ;
#35639=CARTESIAN_POINT ( 'NONE',  ( -19.96994574550859980, -21.32983827578761193, 72.40478737306770540 ) ) ;
#35640=CARTESIAN_POINT ( 'NONE',  ( -11.35719102664687874, -18.40077844947705543, 58.09242476654641507 ) ) ;
#35643=CARTESIAN_POINT ( 'NONE',  ( -13.08938031007640213, -9.312742571539336822, 67.66477384774475468 ) ) ;
#35644=EDGE_CURVE ( 'NONE', #3562, #39905, #27533, .T. ) ;
#35648=CARTESIAN_POINT ( 'NONE',  ( -10.96921284960095555, -11.97350354382807680, 74.84368195529052059 ) ) ;
#35649=ADVANCED_FACE ( 'NONE', ( #2148 ), #7598, .T. ) ;
#35650=EDGE_CURVE ( 'NONE', #21669, #44245, #11326, .T. ) ;
#35653=CARTESIAN_POINT ( 'NONE',  ( -12.12786991918758339, -13.32596279628197600, 53.49899999999994549 ) ) ;
#35654=CARTESIAN_POINT ( 'NONE',  ( -22.48114103837971101, -19.64927616005747879, 72.64400547034465205 ) ) ;
#35656=B_SPLINE_CURVE_WITH_KNOTS ( 'NONE', 3,
 ( #15081, #45392, #16053, #571, #11647, #26924, #19778, #335, #4034, #41437 ),
 .UNSPECIFIED., .F., .F.,
 ( 4, 2, 2, 2, 4 ),
 ( 0.000000000000000000, 0.2500000000000000000, 0.5000000000000000000, 0.7500000000000000000, 1.000000000000000000 ),
 .UNSPECIFIED. ) ;
#35657=ORIENTED_EDGE ( 'NONE', *, *, #18818, .F. ) ;
#35658=CARTESIAN_POINT ( 'NONE',  ( -14.92764478915313653, -21.34891159457319532, 61.63600440564275829 ) ) ;
#35659=CARTESIAN_POINT ( 'NONE',  ( -23.99713630548045273, -11.30230610301594574, 66.52876207254645635 ) ) ;
#35661=CARTESIAN_POINT ( 'NONE',  ( -24.11881394502254849, -17.01995806294775448, 73.16863963025599560 ) ) ;
#35662=ORIENTED_EDGE ( 'NONE', *, *, #33942, .T. ) ;
#35664=CARTESIAN_POINT ( 'NONE',  ( -22.20390354280803180, -19.99167827517580420, 65.70981500101784434 ) ) ;
#35665=CARTESIAN_POINT ( 'NONE',  ( -10.78978129071826686, -12.42417052737942917, 57.32857332104949677 ) ) ;
#35668=CARTESIAN_POINT ( 'NONE',  ( -23.45033742471730420, -11.24757414297479663, 69.96498761153686985 ) ) ;
#35670=CARTESIAN_POINT ( 'NONE',  ( -10.48584418858393796, -13.88064117961823563, 57.44825077271759284 ) ) ;
#35673=CARTESIAN_POINT ( 'NONE',  ( -21.19428927390184114, -8.848463597801222491, 73.48639860482715847 ) ) ;
#35674=VERTEX_POINT ( 'NONE', #35151 ) ;
#35678=ORIENTED_EDGE ( 'NONE', *, *, #1758, .T. ) ;
#35679=CARTESIAN_POINT ( 'NONE',  ( -15.22116837037893866, -21.50650591823945845, 68.59065000974109694 ) ) ;
#35680=CARTESIAN_POINT ( 'NONE',  ( -24.05845762361657947, -12.57644656616312773, 73.24225570276865938 ) ) ;
#35684=CARTESIAN_POINT ( 'NONE',  ( -10.44881520703817479, -17.42631679175528703, 64.74244059074541724 ) ) ;
#35688=ORIENTED_EDGE ( 'NONE', *, *, #1712, .T. ) ;
#35690=CARTESIAN_POINT ( 'NONE',  ( -21.00588228679873382, -20.88502978299158741, 69.46939052609951659 ) ) ;
#35691=VERTEX_POINT ( 'NONE', #1421 ) ;
#35692=CARTESIAN_POINT ( 'NONE',  ( -22.28468842640968006, -19.91619389767071269, 65.98949666203347419 ) ) ;
#35693=CARTESIAN_POINT ( 'NONE',  ( -10.47425561207849753, -17.49314520081206936, 64.81234810402725088 ) ) ;
#35695=CARTESIAN_POINT ( 'NONE',  ( -13.05080691482932487, -8.777874379507830227, 64.10957736189999423 ) ) ;
#35699=CARTESIAN_POINT ( 'NONE',  ( -22.94545718403308854, -10.41951498227516204, 66.84182396041623520 ) ) ;
#35701=CARTESIAN_POINT ( 'NONE',  ( -19.04853579327176760, -7.948602568230340282, 63.71617106789811658 ) ) ;
#35702=B_SPLINE_CURVE_WITH_KNOTS ( 'NONE', 3,
 ( #30111, #34017, #29859, #19013, #30596, #41174, #33771, #14789, #7703, #37712 ),
 .UNSPECIFIED., .F., .F.,
 ( 4, 2, 2, 2, 4 ),
 ( 0.6272669072877665730, 0.7522669073072862922, 0.8772669073268060114, 1.002266907346325731, 1.127266907365845450 ),
 .UNSPECIFIED. ) ;
#35703=CARTESIAN_POINT ( 'NONE',  ( -12.83007325466668114, -20.09077588727113550, 72.10653676829758751 ) ) ;
#35704=CARTESIAN_POINT ( 'NONE',  ( -12.63291411399994146, -9.103221862242449447, 74.50578369661835154 ) ) ;
#35705=CARTESIAN_POINT ( 'NONE',  ( -10.82867520472564848, -11.34449427682889677, 67.73369198428547122 ) ) ;
#35709=EDGE_CURVE ( 'NONE', #11362, #39854, #13169, .T. ) ;
#35710=EDGE_CURVE ( 'NONE', #28414, #15343, #46516, .T. ) ;
#35711=ORIENTED_EDGE ( 'NONE', *, *, #15939, .F. ) ;
#35712=CARTESIAN_POINT ( 'NONE',  ( -10.86332160119170354, -12.36740434215989737, 57.34473927219137579 ) ) ;
#35715=EDGE_CURVE ( 'NONE', #26003, #19831, #9533, .T. ) ;
#35716=CARTESIAN_POINT ( 'NONE',  ( -16.43987971142158599, -21.73979382505777735, 62.05568083039364780 ) ) ;
#35719=CARTESIAN_POINT ( 'NONE',  ( -22.79734409636068904, -10.24514240368273477, 66.54182257473807738 ) ) ;
#35720=CARTESIAN_POINT ( 'NONE',  ( -10.37255316239921044, -15.11044245508572459, 57.71225695896244190 ) ) ;
#35722=ORIENTED_EDGE ( 'NONE', *, *, #33024, .F. ) ;
#35723=CARTESIAN_POINT ( 'NONE',  ( -10.62531315016929767, -17.85539008243733861, 71.66694575197517736 ) ) ;
#35725=VERTEX_POINT ( 'NONE', #25771 ) ;
#35728=CARTESIAN_POINT ( 'NONE',  ( -11.93522140360746064, -14.45952210441258501, 53.49999999999995026 ) ) ;
#35730=CARTESIAN_POINT ( 'NONE',  ( -16.02567528876233993, -7.491550372963335924, 63.92656979170173059 ) ) ;
#35731=DIRECTION ( 'NONE',  ( 5.104528489711356381E-07, 5.317498756133547718E-07, 0.9999999999997283284 ) ) ;
#35732=CARTESIAN_POINT ( 'NONE',  ( -19.23951954158338751, -22.03540154427634334, 58.71162761787055473 ) ) ;
#35733=ORIENTED_EDGE ( 'NONE', *, *, #9269, .F. ) ;
#35734=CARTESIAN_POINT ( 'NONE',  ( -22.58065782673598676, -12.89613362149922260, 53.49899999999994549 ) ) ;
#35736=FACE_OUTER_BOUND ( 'NONE', #16844, .T. ) ;
#35737=( BOUNDED_CURVE ( )  B_SPLINE_CURVE ( 3, ( #16544, #13803, #46842, #13328 ),
 .UNSPECIFIED., .F., .F. ) 
 B_SPLINE_CURVE_WITH_KNOTS ( ( 4, 4 ),
 ( 0.000000000000000000, 0.4074455897393627901 ),
 .UNSPECIFIED. ) 
 CURVE ( )  GEOMETRIC_REPRESENTATION_ITEM ( )  RATIONAL_B_SPLINE_CURVE ( ( 1.000000000000000000, 0.4567392136813325787, 0.3561768502900305444, 0.6983129098260937306 ) ) 
 REPRESENTATION_ITEM ( '' )  );
#35738=LINE ( 'NONE', #32316, #3063 ) ;
#35739=DIRECTION ( 'NONE',  ( 0.8705373987491421550, -0.4921022631314296847, 4.758021987246392719E-08 ) ) ;
#35743=CARTESIAN_POINT ( 'NONE',  ( -11.77745829805909850, -9.948221969229217976, 67.68552175396945358 ) ) ;
#35744=CARTESIAN_POINT ( 'NONE',  ( -10.37541943412130863, -14.96049300415475614, 75.08306784598362071 ) ) ;
#35753=ORIENTED_EDGE ( 'NONE', *, *, #23650, .F. ) ;
#35754=CARTESIAN_POINT ( 'NONE',  ( -11.67943375510494697, -18.89645239624664441, 68.50217487844219022 ) ) ;
#35755=DIRECTION ( 'NONE',  ( 3.549360974554993999E-17, -6.371834667797928663E-18, -1.000000000000000000 ) ) ;
#35756=CARTESIAN_POINT ( 'NONE',  ( -23.07906255732286738, -9.958937815627702861, 66.72677557046061736 ) ) ;
#35757=CARTESIAN_POINT ( 'NONE',  ( -22.80481760130283675, -10.24931098477615166, 70.42667203218238114 ) ) ;
#35760=VERTEX_POINT ( 'NONE', #40790 ) ;
#35761=CARTESIAN_POINT ( 'NONE',  ( -24.80650529658183956, -15.81082447850069883, 69.63969160935214120 ) ) ;
#35762=( BOUNDED_CURVE ( )  B_SPLINE_CURVE ( 3, ( #46787, #1732, #38904, #5183 ),
 .UNSPECIFIED., .F., .F. ) 
 B_SPLINE_CURVE_WITH_KNOTS ( ( 4, 4 ),
 ( 0.9074455897393619574, 1.000000000000000000 ),
 .UNSPECIFIED. ) 
 CURVE ( )  GEOMETRIC_REPRESENTATION_ITEM ( )  RATIONAL_B_SPLINE_CURVE ( ( 0.6983129098260971723, 0.7760317562607017550, 0.8765941196520027345, 1.000000000000000000 ) ) 
 REPRESENTATION_ITEM ( '' )  );
#35763=DIRECTION ( 'NONE',  ( 3.549360974554993999E-17, -6.371834667797928663E-18, -1.000000000000000000 ) ) ;
#35764=B_SPLINE_CURVE_WITH_KNOTS ( 'NONE', 3,
 ( #34655, #43016, #31207, #9054, #4624, #24072, #31695, #16417, #19649, #27512 ),
 .UNSPECIFIED., .F., .F.,
 ( 4, 2, 2, 2, 4 ),
 ( 0.000000000000000000, 0.2500000000000000000, 0.5000000000000000000, 0.7500000000000000000, 1.000000000000000000 ),
 .UNSPECIFIED. ) ;
#35769=CARTESIAN_POINT ( 'NONE',  ( -15.74783386771837890, -7.961078896070159061, 70.62461975990308360 ) ) ;
#35770=B_SPLINE_CURVE_WITH_KNOTS ( 'NONE', 1,
 ( #10498, #7047 ),
 .UNSPECIFIED., .F., .F.,
 ( 2, 2 ),
 ( 0.000000000000000000, 1.000000000000000000 ),
 .UNSPECIFIED. ) ;
#35771=LINE ( 'NONE', #43433, #42900 ) ;
#35772=CARTESIAN_POINT ( 'NONE',  ( -24.59748878097435210, -12.79772186451832994, 66.34600794915635902 ) ) ;
#35773=CARTESIAN_POINT ( 'NONE',  ( -10.42334091404133645, -15.64104667191196185, 61.33789045260130024 ) ) ;
#35778=CARTESIAN_POINT ( 'NONE',  ( -10.66160677810301038, -13.00123309306513697, 67.73832347541063825 ) ) ;
#35779=EDGE_CURVE ( 'NONE', #5540, #19035, #27718, .T. ) ;
#35780=B_SPLINE_CURVE_WITH_KNOTS ( 'NONE', 1,
 ( #31823, #43890 ),
 .UNSPECIFIED., .F., .F.,
 ( 2, 2 ),
 ( 0.000000000000000000, 1.000000000000000000 ),
 .UNSPECIFIED. ) ;
#35781=CARTESIAN_POINT ( 'NONE',  ( -15.56465948913147557, -7.543361525925788236, 53.49999999999994316 ) ) ;
#35782=ADVANCED_FACE ( 'NONE', ( #32901 ), #22991, .T. ) ;
#35784=EDGE_CURVE ( 'NONE', #8895, #6650, #13464, .T. ) ;
#35787=AXIS2_PLACEMENT_3D ( 'NONE', #46185, #42974, #12442 ) ;
#35788=ORIENTED_EDGE ( 'NONE', *, *, #40411, .T. ) ;
#35789=CARTESIAN_POINT ( 'NONE',  ( -10.99586697244644640, -11.04334986774487781, 60.86381167495338929 ) ) ;
#35790=CARTESIAN_POINT ( 'NONE',  ( -24.44334717380189659, -17.30795561478116085, 69.52684539094292404 ) ) ;
#35791=EDGE_CURVE ( 'NONE', #17461, #31125, #31452, .T. ) ;
#35792=ORIENTED_EDGE ( 'NONE', *, *, #47526, .F. ) ;
#35794=CARTESIAN_POINT ( 'NONE',  ( -17.04628566472521811, -7.819299315193825706, 73.96018289602247364 ) ) ;
#35796=CARTESIAN_POINT ( 'NONE',  ( -10.43949455435184603, -13.84896052950683476, 57.46297163929641982 ) ) ;
#35797=CARTESIAN_POINT ( 'NONE',  ( -11.30759946633453339, -18.32231678669580077, 61.36891081969880446 ) ) ;
#35798=ORIENTED_EDGE ( 'NONE', *, *, #15106, .T. ) ;
#35799=CARTESIAN_POINT ( 'NONE',  ( -17.79108452803360763, -21.84994637594637723, 58.69081321602850920 ) ) ;
#35800=CARTESIAN_POINT ( 'NONE',  ( -10.00891317999088592, -15.53039051438984863, 57.72826173703180075 ) ) ;
#35802=CARTESIAN_POINT ( 'NONE',  ( -11.08752838525962048, -17.78389909896315402, 71.79391619061119911 ) ) ;
#35803=ORIENTED_EDGE ( 'NONE', *, *, #7655, .F. ) ;
#35804=CARTESIAN_POINT ( 'NONE',  ( -22.11801181964649388, -9.023811091936513762, 63.44799684341401047 ) ) ;
#35805=CARTESIAN_POINT ( 'NONE',  ( -10.75331649400429868, -16.93069871048427544, 57.68760548944693056 ) ) ;
#35806=FACE_OUTER_BOUND ( 'NONE', #2201, .T. ) ;
#35807=DIRECTION ( 'NONE',  ( 0.8394943004421986377, -0.3114503813636534946, -0.4452504682462426477 ) ) ;
#35809=CARTESIAN_POINT ( 'NONE',  ( -11.46947365556686371, -11.12676018782347320, 60.75056137761610842 ) ) ;
#35810=CARTESIAN_POINT ( 'NONE',  ( -10.00439786467154057, -15.48048233825869424, 57.71792808022589583 ) ) ;
#35811=CARTESIAN_POINT ( 'NONE',  ( -12.16327279079253820, -10.11041878036023967, 67.79896963893753536 ) ) ;
#35813=CARTESIAN_POINT ( 'NONE',  ( -13.85393650630732054, -8.270265118416840977, 74.38450092284953996 ) ) ;
#35815=CARTESIAN_POINT ( 'NONE',  ( -13.38108913796246746, -20.52371920327048826, 58.04650125921649817 ) ) ;
#35816=EDGE_CURVE ( 'NONE', #47755, #19754, #20124, .T. ) ;
#35817=VERTEX_POINT ( 'NONE', #46382 ) ;
#35818=LINE ( 'NONE', #25244, #44389 ) ;
#35819=AXIS2_PLACEMENT_3D ( 'NONE', #44892, #40215, #44174 ) ;
#35821=ORIENTED_EDGE ( 'NONE', *, *, #16746, .T. ) ;
#35822=VERTEX_POINT ( 'NONE', #31352 ) ;
#35824=CARTESIAN_POINT ( 'NONE',  ( -12.90354087724769272, -8.887350501024684490, 67.49447389996370816 ) ) ;
#35825=FACE_OUTER_BOUND ( 'NONE', #17606, .T. ) ;
#35828=ORIENTED_EDGE ( 'NONE', *, *, #12608, .F. ) ;
#35831=EDGE_CURVE ( 'NONE', #35760, #46816, #24789, .T. ) ;
#35832=CARTESIAN_POINT ( 'NONE',  ( -21.00380416015782004, -21.34292312329482399, 62.22976100777699315 ) ) ;
#35833=FACE_OUTER_BOUND ( 'NONE', #8586, .T. ) ;
#35834=ADVANCED_FACE ( 'NONE', ( #29966 ), #16336, .T. ) ;
#35837=ADVANCED_FACE ( 'NONE', ( #11004 ), #8461, .T. ) ;
#35839=CARTESIAN_POINT ( 'NONE',  ( -10.85841931818429629, -17.37798394237198707, 64.91267318220633342 ) ) ;
#35841=EDGE_CURVE ( 'NONE', #22864, #6140, #36462, .T. ) ;
#35842=EDGE_LOOP ( 'NONE', ( #36820, #44403, #15678, #48437 ) ) ;
#35843=CARTESIAN_POINT ( 'NONE',  ( -11.66088694488815314, -18.78249085348093672, 68.51689682890159361 ) ) ;
#35845=CARTESIAN_POINT ( 'NONE',  ( -10.65515204393805959, -12.82555568974835580, 61.00673515780317757 ) ) ;
#35846=CARTESIAN_POINT ( 'NONE',  ( -11.25385002771267473, -18.98553936430136702, 68.40345028533118921 ) ) ;
#35848=VERTEX_POINT ( 'NONE', #27413 ) ;
#35849=DIRECTION ( 'NONE',  ( 0.9942595023566571655, -0.1069955231469582047, 3.800058679842194246E-08 ) ) ;
#35851=CARTESIAN_POINT ( 'NONE',  ( -11.73296596577226936, -10.64774513788296417, 74.72412863062541533 ) ) ;
#35852=DIRECTION ( 'NONE',  ( 0.6043825497304157190, -0.7966942535134532433, 5.656674838975381179E-08 ) ) ;
#35855=EDGE_CURVE ( 'NONE', #5832, #18426, #23745, .T. ) ;
#35856=VERTEX_POINT ( 'NONE', #33376 ) ;
#35858=CARTESIAN_POINT ( 'NONE',  ( -14.65075332640449091, -7.894636944940137901, 60.42022027453841559 ) ) ;
#35859=ORIENTED_EDGE ( 'NONE', *, *, #2974, .F. ) ;
#35860=CARTESIAN_POINT ( 'NONE',  ( -10.42546210075913748, -12.25520342886974845, 57.44361899967025664 ) ) ;
#35862=CARTESIAN_POINT ( 'NONE',  ( -17.01436944207222624, -7.370403393205478437, 74.21664194825545735 ) ) ;
#35863=B_SPLINE_CURVE_WITH_KNOTS ( 'NONE', 3,
 ( #39619, #22059, #28045, #1948, #43071, #31992, #47005, #11705, #8040, #14878 ),
 .UNSPECIFIED., .F., .F.,
 ( 4, 2, 2, 2, 4 ),
 ( 0.000000000000000000, 0.2500000000000000000, 0.5000000000000000000, 0.7500000000000000000, 1.000000000000000000 ),
 .UNSPECIFIED. ) ;
#35865=ORIENTED_EDGE ( 'NONE', *, *, #270, .F. ) ;
#35866=CARTESIAN_POINT ( 'NONE',  ( -17.00410623003636346, -7.771727578618798482, 74.11018273220987851 ) ) ;
#35868=CARTESIAN_POINT ( 'NONE',  ( -10.09291371782238045, -16.13494220690481384, 68.16263107114907882 ) ) ;
#35869=ORIENTED_EDGE ( 'NONE', *, *, #33585, .T. ) ;
#35871=CARTESIAN_POINT ( 'NONE',  ( -24.19028598586675116, -12.80082241304059210, 62.98831023884616798 ) ) ;
#35872=VERTEX_POINT ( 'NONE', #48419 ) ;
#35873=ORIENTED_EDGE ( 'NONE', *, *, #11049, .T. ) ;
#35874=CARTESIAN_POINT ( 'NONE',  ( -20.46655431664719060, -21.17292242669622837, 58.73655241890688927 ) ) ;
#35875=DIRECTION ( 'NONE',  ( 0.8324837747691379297, 0.5540494244615070674, 4.550593720660606642E-17 ) ) ;
#35878=CARTESIAN_POINT ( 'NONE',  ( -18.77178190320302775, -7.889067033164298692, 70.37627854585417708 ) ) ;
#35879=CARTESIAN_POINT ( 'NONE',  ( -19.54417908753315558, -21.48049550124873619, 62.22176935888264637 ) ) ;
#35880=( BOUNDED_SURFACE ( )  B_SPLINE_SURFACE ( 3, 1, ( 
 ( #198, #27010 ),
 ( #26042, #30481 ),
 ( #37339, #45496 ),
 ( #3626, #33641 ),
 ( #48682, #14926 ),
 ( #29983, #41295 ),
 ( #7581, #3885 ) ),
 .UNSPECIFIED., .T., .F., .F. ) 
 B_SPLINE_SURFACE_WITH_KNOTS ( ( 4, 3, 4 ),
 ( 2, 2 ),
 ( 0.000000000000000000, 0.5000000000000000000, 1.000000000000000000 ),
 ( 0.000000000000000000, 1.000000000000000000 ),
 .UNSPECIFIED. ) 
 GEOMETRIC_REPRESENTATION_ITEM ( )  RATIONAL_B_SPLINE_SURFACE ( (
 ( 1.000000000000000000, 1.000000000000000000),
 ( 0.3333333333333335369, 0.3333333333333330373),
 ( 0.3333333333333335369, 0.3333333333333330373),
 ( 1.000000000000000000, 1.000000000000000000),
 ( 0.3333333333333333703, 0.3333333333333333703),
 ( 0.3333333333333333703, 0.3333333333333333703),
 ( 1.000000000000000000, 1.000000000000000000) ) ) 
 REPRESENTATION_ITEM ( '' )  SURFACE ( )  );
#35881=CARTESIAN_POINT ( 'NONE',  ( -12.32124988467013615, -19.60105808195379140, 58.21217042357060478 ) ) ;
#35882=DIRECTION ( 'NONE',  ( -0.7670373483544791204, -0.6416024518573234525, 2.496223344567222868E-08 ) ) ;
#35886=ORIENTED_EDGE ( 'NONE', *, *, #21141, .F. ) ;
#35888=LINE ( 'NONE', #35653, #1587 ) ;
#35889=FACE_OUTER_BOUND ( 'NONE', #8804, .T. ) ;
#35890=CARTESIAN_POINT ( 'NONE',  ( -13.88419686192642111, -8.703135698866935499, 57.11400917758039952 ) ) ;
#35893=( BOUNDED_CURVE ( )  B_SPLINE_CURVE ( 3, ( #21969, #22457, #3002, #36965 ),
 .UNSPECIFIED., .F., .F. ) 
 B_SPLINE_CURVE_WITH_KNOTS ( ( 4, 4 ),
 ( 0.5000000000000000000, 0.9074455897393716164 ),
 .UNSPECIFIED. ) 
 CURVE ( )  GEOMETRIC_REPRESENTATION_ITEM ( )  RATIONAL_B_SPLINE_CURVE ( ( 1.000000000000037081, 0.4567392136813289705, 0.3561768502900032329, 0.6983129098260999479 ) ) 
 REPRESENTATION_ITEM ( '' )  );
#35894=ORIENTED_EDGE ( 'NONE', *, *, #37987, .F. ) ;
#35895=ADVANCED_FACE ( 'NONE', ( #7326 ), #21400, .T. ) ;
#35896=CARTESIAN_POINT ( 'NONE',  ( -20.03518388220226143, -21.78744935781895009, 72.59133997248245862 ) ) ;
#35897=CARTESIAN_POINT ( 'NONE',  ( -19.92776479198160189, -21.39998277484045275, 72.41950795000725805 ) ) ;
#35898=EDGE_CURVE ( 'NONE', #18094, #43051, #34610, .T. ) ;
#35900=CARTESIAN_POINT ( 'NONE',  ( -18.18535082455230523, -22.22026082442155115, 65.45193850245834710 ) ) ;
#35902=CARTESIAN_POINT ( 'NONE',  ( -10.13608973233657196, -13.26381535464663131, 74.87155958832882163 ) ) ;
#35904=CARTESIAN_POINT ( 'NONE',  ( -13.76849323099554567, -20.83774554052356365, 65.27156739751333703 ) ) ;
#35905=CARTESIAN_POINT ( 'NONE',  ( -12.81585776823299483, -9.539872998625803291, 74.31922966058063196 ) ) ;
#35907=CARTESIAN_POINT ( 'NONE',  ( -18.97054302448013985, -7.521389842619064403, 67.08567168106696954 ) ) ;
#35908=B_SPLINE_CURVE_WITH_KNOTS ( 'NONE', 1,
 ( #9019, #31413 ),
 .UNSPECIFIED., .F., .F.,
 ( 2, 2 ),
 ( 0.000000000000000000, 1.000000000000000000 ),
 .UNSPECIFIED. ) ;
#35909=CARTESIAN_POINT ( 'NONE',  ( -23.44282052155508111, -11.23500321550520731, 70.00096727704672617 ) ) ;
#35911=CARTESIAN_POINT ( 'NONE',  ( -20.92516765556211666, -8.685814626085017309, 59.93305413929914494 ) ) ;
#35912=ORIENTED_EDGE ( 'NONE', *, *, #13950, .F. ) ;
#35915=AXIS2_PLACEMENT_3D ( 'NONE', #44096, #40599, #10349 ) ;
#35917=CARTESIAN_POINT ( 'NONE',  ( -11.68335550665270794, -18.81469308649876737, 68.21689631955439381 ) ) ;
#35918=CARTESIAN_POINT ( 'NONE',  ( -10.22391373207313237, -12.89608419319863053, 67.93821120038428774 ) ) ;
#35920=EDGE_CURVE ( 'NONE', #45327, #28927, #3055, .T. ) ;
#35921=EDGE_CURVE ( 'NONE', #31348, #12784, #15342, .T. ) ;
#35922=ADVANCED_FACE ( 'NONE', ( #9689 ), #26137, .T. ) ;
#35924=ORIENTED_EDGE ( 'NONE', *, *, #34889, .T. ) ;
#35925=CARTESIAN_POINT ( 'NONE',  ( -15.19548991633585011, -21.91815178685365595, 68.76088227238139439 ) ) ;
#35928=B_SPLINE_CURVE_WITH_KNOTS ( 'NONE', 1,
 ( #38353, #41586 ),
 .UNSPECIFIED., .F., .F.,
 ( 2, 2 ),
 ( 0.000000000000000000, 1.000000000000000000 ),
 .UNSPECIFIED. ) ;
#35929=FACE_OUTER_BOUND ( 'NONE', #43984, .T. ) ;
#35930=ORIENTED_EDGE ( 'NONE', *, *, #8484, .T. ) ;
#35932=CARTESIAN_POINT ( 'NONE',  ( -11.73296596577226936, -10.64774513788296240, 74.72412863062541533 ) ) ;
#35933=CARTESIAN_POINT ( 'NONE',  ( -18.30727046116018286, -21.75326869042403288, 69.11514702556002021 ) ) ;
#35935=ORIENTED_EDGE ( 'NONE', *, *, #42902, .T. ) ;
#35936=ORIENTED_EDGE ( 'NONE', *, *, #201, .T. ) ;
#35937=CARTESIAN_POINT ( 'NONE',  ( -23.81420843745974381, -18.63945674058080826, 72.94085094053922091 ) ) ;
#35938=CARTESIAN_POINT ( 'NONE',  ( -21.36284888653444725, -21.13297021396988384, 69.16954901539321554 ) ) ;
#35939=ORIENTED_EDGE ( 'NONE', *, *, #44042, .F. ) ;
#35940=CARTESIAN_POINT ( 'NONE',  ( -10.63483715323753565, -17.87674169505483235, 71.75213630217804450 ) ) ;
#35941=CARTESIAN_POINT ( 'NONE',  ( -10.68008709410406354, -12.75422072778657601, 64.27395902318073695 ) ) ;
#35945=CARTESIAN_POINT ( 'NONE',  ( -15.62100938680255524, -7.580606089661849012, 70.72494556531428600 ) ) ;
#35947=DIRECTION ( 'NONE',  ( -0.8017593358536256876, -0.5976470257363775129, 1.209213344977627448E-07 ) ) ;
#35949=CARTESIAN_POINT ( 'NONE',  ( -19.17247957453286844, -7.567181637230756763, 63.61584517348745038 ) ) ;
#35951=CARTESIAN_POINT ( 'NONE',  ( -10.82516083999262690, -11.35126292582506302, 67.72590458424124904 ) ) ;
#35955=ORIENTED_EDGE ( 'NONE', *, *, #29318, .F. ) ;
#35956=CARTESIAN_POINT ( 'NONE',  ( -12.56172001024846452, -20.45377019276184427, 71.99149100736865137 ) ) ;
#35957=CARTESIAN_POINT ( 'NONE',  ( -14.08076552632586420, -21.02024474708484192, 68.45624882270347200 ) ) ;
#35959=CARTESIAN_POINT ( 'NONE',  ( -10.71125836907356543, -12.65457585138356400, 61.09293791546713948 ) ) ;
#35960=AXIS2_PLACEMENT_3D ( 'NONE', #21470, #9671, #14281 ) ;
#35961=EDGE_LOOP ( 'NONE', ( #26796, #433 ) ) ;
#35964=VERTEX_POINT ( 'NONE', #15037 ) ;
#35965=CARTESIAN_POINT ( 'NONE',  ( -10.60881404221464663, -17.81840116198948820, 71.67444023447058044 ) ) ;
#35966=CARTESIAN_POINT ( 'NONE',  ( -19.76711226259482856, -21.88123280879678134, 65.65760363486209883 ) ) ;
#35967=VERTEX_POINT ( 'NONE', #18495 ) ;
#35968=CARTESIAN_POINT ( 'NONE',  ( -23.04402284766838349, -19.06632961612601918, 59.16938527523783620 ) ) ;
#35969=EDGE_LOOP ( 'NONE', ( #33053, #40154 ) ) ;
#35970=CARTESIAN_POINT ( 'NONE',  ( -10.61357140615669792, -13.19155887971477448, 71.50828586566468914 ) ) ;
#35971=VERTEX_POINT ( 'NONE', #40663 ) ;
#35972=CARTESIAN_POINT ( 'NONE',  ( -20.35208293893518672, -8.450992964911224092, 67.08104082230126153 ) ) ;
#35973=CARTESIAN_POINT ( 'NONE',  ( -22.83095763869631512, -19.93459457198476770, 72.82895875648904394 ) ) ;
#35974=CARTESIAN_POINT ( 'NONE',  ( -20.89788161767221197, -20.94431024770144489, 62.39999296070408974 ) ) ;
#35976=CARTESIAN_POINT ( 'NONE',  ( -13.41271538705132116, -9.007285817396986971, 57.17787480142766299 ) ) ;
#35977=EDGE_CURVE ( 'NONE', #25499, #9944, #29577, .T. ) ;
#35979=CARTESIAN_POINT ( 'NONE',  ( -24.04021708909630206, -12.36549076622675791, 73.12736853451067986 ) ) ;
#35980=CYLINDRICAL_SURFACE ( 'NONE', #3747, 0.1499999999999994948 ) ;
#35981=VECTOR ( 'NONE', #17264, 1000.000000000000227 ) ;
#35982=CARTESIAN_POINT ( 'NONE',  ( -13.75553675855627134, -8.845634611387561463, 57.15894934091076607 ) ) ;
#35983=CARTESIAN_POINT ( 'NONE',  ( -13.49145512112739276, -18.65424914341562967, 53.49999999999995026 ) ) ;
#35984=CARTESIAN_POINT ( 'NONE',  ( -19.24944996930525676, -8.051263618916641107, 60.26092964427753884 ) ) ;
#35985=EDGE_LOOP ( 'NONE', ( #43486, #38550, #18023, #17783, #42552 ) ) ;
#35989=CARTESIAN_POINT ( 'NONE',  ( -16.78411497196904278, -21.83009869597352903, 68.69560651670111895 ) ) ;
#35990=FACE_OUTER_BOUND ( 'NONE', #18912, .T. ) ;
#35991=EDGE_CURVE ( 'NONE', #5827, #40125, #47117, .T. ) ;
#35992=EDGE_CURVE ( 'NONE', #45391, #43613, #14198, .T. ) ;
#35993=CARTESIAN_POINT ( 'NONE',  ( -13.13238435621759237, -20.89891265215350913, 58.15375942484206462 ) ) ;
#35995=ORIENTED_EDGE ( 'NONE', *, *, #10613, .F. ) ;
#35996=CARTESIAN_POINT ( 'NONE',  ( -21.24554520941113367, -21.20453976546471608, 65.76949229983627276 ) ) ;
#35997=DIRECTION ( 'NONE',  ( -2.027460363947684990E-06, -1.195255637520530846E-05, 0.9999999999265128947 ) ) ;
#36001=CARTESIAN_POINT ( 'NONE',  ( -14.62687819956926027, -8.392386103536567887, 64.08978840643771946 ) ) ;
#36003=CARTESIAN_POINT ( 'NONE',  ( -12.10131192688100477, -10.18592936015514638, 64.31442259820508411 ) ) ;
#36005=ORIENTED_EDGE ( 'NONE', *, *, #15666, .F. ) ;
#36006=CARTESIAN_POINT ( 'NONE',  ( -16.50258162057404832, -20.23145840177225807, 53.49999999999995026 ) ) ;
#36008=CARTESIAN_POINT ( 'NONE',  ( -20.81696265954430558, -20.93198702957875668, 62.11471400680572685 ) ) ;
#36010=VERTEX_POINT ( 'NONE', #25182 ) ;
#36012=CARTESIAN_POINT ( 'NONE',  ( -13.41535183621916438, -9.069180408055801834, 64.13776496077019829 ) ) ;
#36013=CARTESIAN_POINT ( 'NONE',  ( -20.88270815654435353, -21.40782497263450068, 58.82970582236164603 ) ) ;
#36014=CARTESIAN_POINT ( 'NONE',  ( -23.44980260057077714, -18.46889688393208218, 72.76368236443251192 ) ) ;
#36015=ORIENTED_EDGE ( 'NONE', *, *, #34150, .T. ) ;
#36018=CARTESIAN_POINT ( 'NONE',  ( -13.18702109819586710, -9.237203801506172596, 64.01832437545327537 ) ) ;
#36019=AXIS2_PLACEMENT_3D ( 'NONE', #4334, #20319, #38783 ) ;
#36020=CARTESIAN_POINT ( 'NONE',  ( -12.06140467229625912, -20.05244645202335008, 53.49999999999994316 ) ) ;
#36024=CARTESIAN_POINT ( 'NONE',  ( -22.91174631722474686, -10.46344187337216169, 59.79306521909829542 ) ) ;
#36025=LINE ( 'NONE', #17315, #27750 ) ;
#36030=VERTEX_POINT ( 'NONE', #18004 ) ;
#36031=( BOUNDED_CURVE ( )  B_SPLINE_CURVE ( 3, ( #293, #18483, #4452, #41890 ),
 .UNSPECIFIED., .F., .F. ) 
 B_SPLINE_CURVE_WITH_KNOTS ( ( 4, 4 ),
 ( 0.000000000000000000, 0.4074455897393691739 ),
 .UNSPECIFIED. ) 
 CURVE ( )  GEOMETRIC_REPRESENTATION_ITEM ( )  RATIONAL_B_SPLINE_CURVE ( ( 1.000000000000000000, 0.4567392136813293035, 0.3561768502900293232, 0.6983129098261000589 ) ) 
 REPRESENTATION_ITEM ( '' )  );
#36032=CARTESIAN_POINT ( 'NONE',  ( -23.04367457972577427, -10.55211693511195215, 59.75203429192391269 ) ) ;
#36033=CARTESIAN_POINT ( 'NONE',  ( -11.91076409904084699, -14.84341972694825884, 53.69233794759168177 ) ) ;
#36034=ORIENTED_EDGE ( 'NONE', *, *, #47664, .F. ) ;
#36035=PLANE ( 'NONE',  #18160 ) ;
#36038=CARTESIAN_POINT ( 'NONE',  ( -17.52077441883401576, -21.86154573861348283, 58.82041992746825798 ) ) ;
#36039=ADVANCED_FACE ( 'NONE', ( #29352 ), #33258, .F. ) ;
#36040=CARTESIAN_POINT ( 'NONE',  ( -24.42668993457695592, -13.99045928592870958, 73.40799407547365263 ) ) ;
#36042=CARTESIAN_POINT ( 'NONE',  ( -24.69524243360033111, -13.18581942010154506, 59.50121368153175183 ) ) ;
#36043=VERTEX_POINT ( 'NONE', #44384 ) ;
#36044=FACE_OUTER_BOUND ( 'NONE', #40935, .T. ) ;
#36047=( BOUNDED_SURFACE ( )  B_SPLINE_SURFACE ( 3, 1, ( 
 ( #4519, #27175 ),
 ( #2279, #13342 ),
 ( #47357, #39708 ),
 ( #16799, #28861 ),
 ( #43905, #32556 ),
 ( #5973, #24465 ),
 ( #20996, #17287 ) ),
 .UNSPECIFIED., .T., .F., .F. ) 
 B_SPLINE_SURFACE_WITH_KNOTS ( ( 4, 3, 4 ),
 ( 2, 2 ),
 ( 0.000000000000000000, 0.5000000000000000000, 1.000000000000000000 ),
 ( 0.000000000000000000, 1.000000000000000000 ),
 .UNSPECIFIED. ) 
 GEOMETRIC_REPRESENTATION_ITEM ( )  RATIONAL_B_SPLINE_SURFACE ( (
 ( 1.000000000000000000, 1.000000000000000000),
 ( 0.3333333333333335369, 0.3333333333333330373),
 ( 0.3333333333333335369, 0.3333333333333330373),
 ( 1.000000000000000000, 1.000000000000000000),
 ( 0.3333333333333333703, 0.3333333333333333703),
 ( 0.3333333333333333703, 0.3333333333333333703),
 ( 1.000000000000000000, 1.000000000000000000) ) ) 
 REPRESENTATION_ITEM ( '' )  SURFACE ( )  );
#36048=EDGE_CURVE ( 'NONE', #22956, #14468, #43109, .T. ) ;
#36053=DIRECTION ( 'NONE',  ( -6.651268172957068788E-06, -3.577353461959433263E-06, -0.9999999999714815901 ) ) ;
#36054=ORIENTED_EDGE ( 'NONE', *, *, #305, .F. ) ;
#36055=CARTESIAN_POINT ( 'NONE',  ( -13.84130163926618451, -8.277085044245813705, 74.35988050052598908 ) ) ;
#36057=CARTESIAN_POINT ( 'NONE',  ( -13.49145512112739631, -18.65424914341562612, 54.07175714974879099 ) ) ;
#36059=ORIENTED_EDGE ( 'NONE', *, *, #7034, .F. ) ;
#36060=CARTESIAN_POINT ( 'NONE',  ( -23.74619265052512418, -11.68934008440959893, 62.95218278636777143 ) ) ;
#36063=ORIENTED_EDGE ( 'NONE', *, *, #18242, .F. ) ;
#36064=VERTEX_POINT ( 'NONE', #22210 ) ;
#36065=EDGE_LOOP ( 'NONE', ( #17125, #47327 ) ) ;
#36066=CARTESIAN_POINT ( 'NONE',  ( -14.07761835836965858, -20.95746660330474143, 72.22607703844037985 ) ) ;
#36067=VECTOR ( 'NONE', #11176, 1000.000000000000114 ) ;
#36068=CARTESIAN_POINT ( 'NONE',  ( -23.76771070410665132, -11.84943609209516424, 59.48235735874851571 ) ) ;
#36073=ORIENTED_EDGE ( 'NONE', *, *, #32649, .T. ) ;
#36075=CARTESIAN_POINT ( 'NONE',  ( -18.46801905451614445, -7.836623195388688679, 74.12592262855558545 ) ) ;
#36076=CARTESIAN_POINT ( 'NONE',  ( -11.77193539988124371, -19.02301398277157318, 71.98685856039797670 ) ) ;
#36079=CARTESIAN_POINT ( 'NONE',  ( -15.41904748403203484, -7.634001509309876532, 74.19490257054667381 ) ) ;
#36081=CARTESIAN_POINT ( 'NONE',  ( -24.87421550414592986, -14.80086288727809141, 59.42017156831820301 ) ) ;
#36086=AXIS2_PLACEMENT_3D ( 'NONE', #11600, #26629, #18737 ) ;
#36087=VECTOR ( 'NONE', #12088, 1000.000000000000227 ) ;
#36090=CARTESIAN_POINT ( 'NONE',  ( -16.28253830925437384, -21.71555932027983715, 58.57120154339385465 ) ) ;
#36091=CARTESIAN_POINT ( 'NONE',  ( -18.97054410961560578, -7.521390078327941708, 67.08567059339527816 ) ) ;
#36093=VECTOR ( 'NONE', #41637, 1000.000000000000000 ) ;
#36094=CARTESIAN_POINT ( 'NONE',  ( -19.37484727228654080, -7.619050864103940057, 60.14588289477547534 ) ) ;
#36095=CARTESIAN_POINT ( 'NONE',  ( -23.12535468111908443, -10.01343724238356359, 66.65686954956312604 ) ) ;
#36096=CARTESIAN_POINT ( 'NONE',  ( -20.18941624216641273, -7.891347737435665977, 73.83601159825586535 ) ) ;
#36097=ORIENTED_EDGE ( 'NONE', *, *, #5511, .F. ) ;
#36098=CYLINDRICAL_SURFACE ( 'NONE', #12620, 0.1499999999999986067 ) ;
#36099=CARTESIAN_POINT ( 'NONE',  ( -24.45714095472541771, -14.31630891555218987, 69.66747352629326429 ) ) ;
#36100=EDGE_LOOP ( 'NONE', ( #47536, #36059, #13228, #34049 ) ) ;
#36101=CARTESIAN_POINT ( 'NONE',  ( -13.45889463159840282, -8.979947265385323618, 60.43950308547118766 ) ) ;
#36103=ORIENTED_EDGE ( 'NONE', *, *, #39276, .F. ) ;
#36104=CARTESIAN_POINT ( 'NONE',  ( -20.19053640067075506, -7.838066347919499854, 53.49999999999994316 ) ) ;
#36106=CARTESIAN_POINT ( 'NONE',  ( -24.46506355971582991, -17.24406257311080992, 72.99840714145864240 ) ) ;
#36107=ADVANCED_FACE ( 'NONE', ( #1018 ), #23189, .T. ) ;
#36109=ORIENTED_EDGE ( 'NONE', *, *, #493, .T. ) ;
#36110=CARTESIAN_POINT ( 'NONE',  ( -23.44980356754079054, -18.46889531339634871, 72.91368236442116313 ) ) ;
#36111=EDGE_CURVE ( 'NONE', #29137, #656, #24177, .T. ) ;
#36113=CARTESIAN_POINT ( 'NONE',  ( -24.93953149451673568, -10.04808947811604902, 53.49999999999995026 ) ) ;
#36114=EDGE_LOOP ( 'NONE', ( #28895, #6036 ) ) ;
#36115=ADVANCED_FACE ( 'NONE', ( #38681 ), #31170, .T. ) ;
#36116=CARTESIAN_POINT ( 'NONE',  ( -17.92193035392797285, -21.84160718002658541, 61.87535923543195793 ) ) ;
#36117=B_SPLINE_CURVE_WITH_KNOTS ( 'NONE', 1,
 ( #18097, #44243 ),
 .UNSPECIFIED., .F., .F.,
 ( 2, 2 ),
 ( 0.000000000000000000, 1.000000000000000000 ),
 .UNSPECIFIED. ) ;
#36118=ORIENTED_EDGE ( 'NONE', *, *, #7851, .T. ) ;
#36120=CARTESIAN_POINT ( 'NONE',  ( -10.37497031247464463, -14.69804315800203476, 71.62782692816419683 ) ) ;
#36123=CARTESIAN_POINT ( 'NONE',  ( -10.02024861317775262, -15.63870305697176377, 61.19935569097407324 ) ) ;
#36124=( BOUNDED_SURFACE ( )  B_SPLINE_SURFACE ( 3, 1, ( 
 ( #29051, #47533 ),
 ( #13767, #25364 ),
 ( #32737, #7140 ),
 ( #14245, #25592 ),
 ( #36183, #28811 ),
 ( #26094, #17944 ),
 ( #10583, #44098 ) ),
 .UNSPECIFIED., .T., .F., .F. ) 
 B_SPLINE_SURFACE_WITH_KNOTS ( ( 4, 3, 4 ),
 ( 2, 2 ),
 ( 0.000000000000000000, 0.5000000000000000000, 1.000000000000000000 ),
 ( 0.000000000000000000, 1.000000000000000000 ),
 .UNSPECIFIED. ) 
 GEOMETRIC_REPRESENTATION_ITEM ( )  RATIONAL_B_SPLINE_SURFACE ( (
 ( 1.000000000000000000, 1.000000000000000000),
 ( 0.3333333333333335369, 0.3333333333333330373),
 ( 0.3333333333333335369, 0.3333333333333330373),
 ( 1.000000000000000000, 1.000000000000000000),
 ( 0.3333333333333333703, 0.3333333333333333703),
 ( 0.3333333333333333703, 0.3333333333333333703),
 ( 1.000000000000000000, 1.000000000000000000) ) ) 
 REPRESENTATION_ITEM ( '' )  SURFACE ( )  );
#36126=DIRECTION ( 'NONE',  ( -0.6105870317843965500, -0.7919491628991826015, 6.540688078712152548E-08 ) ) ;
#36127=CARTESIAN_POINT ( 'NONE',  ( -23.89279295945009096, -11.11331726805715725, 69.93564813258274171 ) ) ;
#36128=EDGE_CURVE ( 'NONE', #2367, #48136, #27137, .T. ) ;
#36129=CARTESIAN_POINT ( 'NONE',  ( -14.93036884410937937, -8.267093201351965348, 60.39166468221263528 ) ) ;
#36130=CARTESIAN_POINT ( 'NONE',  ( -12.24887892415898172, -20.16835215658221969, 65.05949058504921823 ) ) ;
#36131=VECTOR ( 'NONE', #44321, 1000.000000000000114 ) ;
#36134=FACE_OUTER_BOUND ( 'NONE', #23066, .T. ) ;
#36135=CARTESIAN_POINT ( 'NONE',  ( -23.06991199560340533, -9.948164920181065796, 66.68035737299506138 ) ) ;
#36136=LINE ( 'NONE', #2421, #44116 ) ;
#36138=FACE_OUTER_BOUND ( 'NONE', #7060, .T. ) ;
#36139=CARTESIAN_POINT ( 'NONE',  ( -20.48427295952909688, -21.16374346551129548, 59.05963865090804887 ) ) ;
#36141=VERTEX_POINT ( 'NONE', #19735 ) ;
#36142=CARTESIAN_POINT ( 'NONE',  ( -10.44881481234349252, -17.42631575494719698, 64.74243950200344955 ) ) ;
#36143=CARTESIAN_POINT ( 'NONE',  ( -22.82423354248128078, -9.676858997600051637, 73.63161091602947295 ) ) ;
#36144=CARTESIAN_POINT ( 'NONE',  ( -23.44980260057077714, -18.46889688393208573, 72.76368236443251192 ) ) ;
#36146=ORIENTED_EDGE ( 'NONE', *, *, #45364, .T. ) ;
#36151=FACE_OUTER_BOUND ( 'NONE', #23209, .T. ) ;
#36152=EDGE_LOOP ( 'NONE', ( #28616, #2944, #21850, #46035, #28997 ) ) ;
#36153=ADVANCED_FACE ( 'NONE', ( #31291 ), #46074, .T. ) ;
#36154=DIRECTION ( 'NONE',  ( 8.560949391518745609E-06, -2.380493834460222846E-06, 0.9999999999605218015 ) ) ;
#36156=EDGE_LOOP ( 'NONE', ( #27855, #34589 ) ) ;
#36157=CARTESIAN_POINT ( 'NONE',  ( -22.25476733894167580, -19.94415178569153468, 66.00421729349081090 ) ) ;
#36158=CARTESIAN_POINT ( 'NONE',  ( -10.01510117332873584, -14.02744298369021969, 61.09634062789294973 ) ) ;
#36159=ORIENTED_EDGE ( 'NONE', *, *, #27818, .F. ) ;
#36160=CARTESIAN_POINT ( 'NONE',  ( -12.71302066933910524, -9.037873161084162277, 70.99925350880062069 ) ) ;
#36164=( BOUNDED_SURFACE ( )  B_SPLINE_SURFACE ( 3, 1, ( 
 ( #44409, #10663 ),
 ( #25927, #40940 ),
 ( #6969, #36983 ),
 ( #32813, #17311 ),
 ( #43685, #47844 ),
 ( #29133, #40451 ),
 ( #38198, #41188 ) ),
 .UNSPECIFIED., .T., .F., .F. ) 
 B_SPLINE_SURFACE_WITH_KNOTS ( ( 4, 3, 4 ),
 ( 2, 2 ),
 ( 0.000000000000000000, 0.5000000000000000000, 1.000000000000000000 ),
 ( 0.000000000000000000, 1.000000000000000000 ),
 .UNSPECIFIED. ) 
 GEOMETRIC_REPRESENTATION_ITEM ( )  RATIONAL_B_SPLINE_SURFACE ( (
 ( 1.000000000000000000, 1.000000000000000000),
 ( 0.3333333333333335369, 0.3333333333333330373),
 ( 0.3333333333333335369, 0.3333333333333330373),
 ( 1.000000000000000000, 1.000000000000000000),
 ( 0.3333333333333333703, 0.3333333333333333703),
 ( 0.3333333333333333703, 0.3333333333333333703),
 ( 1.000000000000000000, 1.000000000000000000) ) ) 
 REPRESENTATION_ITEM ( '' )  SURFACE ( )  );
#36165=CARTESIAN_POINT ( 'NONE',  ( -20.00946503018472811, -8.250368534377352958, 73.72096600125085786 ) ) ;
#36166=FACE_OUTER_BOUND ( 'NONE', #17010, .T. ) ;
#36168=CARTESIAN_POINT ( 'NONE',  ( -13.47245400663725690, -21.12492667118925382, 65.10133491818508844 ) ) ;
#36170=EDGE_CURVE ( 'NONE', #30487, #40380, #36186, .T. ) ;
#36171=CARTESIAN_POINT ( 'NONE',  ( -11.32604004198825365, -11.37209441256710463, 60.86988868631853933 ) ) ;
#36172=CARTESIAN_POINT ( 'NONE',  ( -22.91943239076679006, -10.38811108791941429, 59.48714571049892896 ) ) ;
#36173=ORIENTED_EDGE ( 'NONE', *, *, #30849, .F. ) ;
#36175=ORIENTED_EDGE ( 'NONE', *, *, #44201, .T. ) ;
#36177=CARTESIAN_POINT ( 'NONE',  ( -23.79811132998510459, -18.66596081585729650, 72.86344597896119524 ) ) ;
#36179=ORIENTED_EDGE ( 'NONE', *, *, #10619, .T. ) ;
#36180=CARTESIAN_POINT ( 'NONE',  ( -20.75149224175378748, -8.143498925893005946, 63.50459817289195996 ) ) ;
#36183=CARTESIAN_POINT ( 'NONE',  ( -23.89460186926044472, -11.99007647016461320, 63.09651074612323640 ) ) ;
#36185=CARTESIAN_POINT ( 'NONE',  ( -15.61945779041031201, -7.581001026129836617, 70.86635785818099009 ) ) ;
#36186=( BOUNDED_CURVE ( )  B_SPLINE_CURVE ( 3, ( #42387, #8657, #26385, #41400 ),
 .UNSPECIFIED., .F., .F. ) 
 B_SPLINE_CURVE_WITH_KNOTS ( ( 4, 4 ),
 ( 0.000000000000000000, 0.4074455897393690629 ),
 .UNSPECIFIED. ) 
 CURVE ( )  GEOMETRIC_REPRESENTATION_ITEM ( )  RATIONAL_B_SPLINE_CURVE ( ( 1.000000000000000000, 0.4567392136813264170, 0.3561768502900282130, 0.6983129098261053880 ) ) 
 REPRESENTATION_ITEM ( '' )  );
#36187=VERTEX_POINT ( 'NONE', #41653 ) ;
#36189=B_SPLINE_CURVE_WITH_KNOTS ( 'NONE', 3,
 ( #24412, #5214, #35229, #1504 ),
 .UNSPECIFIED., .F., .F.,
 ( 4, 4 ),
 ( 0.000000000000000000, 0.1735808155647264317 ),
 .UNSPECIFIED. ) ;
#36191=CARTESIAN_POINT ( 'NONE',  ( -22.80485643099853021, -9.656470841191969967, 73.67435257262538073 ) ) ;
#36192=CARTESIAN_POINT ( 'NONE',  ( -16.58312381330344110, -22.21171629078730092, 65.40281258638998452 ) ) ;
#36194=AXIS2_PLACEMENT_3D ( 'NONE', #40681, #41414, #37458 ) ;
#36195=EDGE_CURVE ( 'NONE', #25586, #42260, #12611, .T. ) ;
#36196=ORIENTED_EDGE ( 'NONE', *, *, #7241, .T. ) ;
#36197=( BOUNDED_CURVE ( )  B_SPLINE_CURVE ( 3, ( #38026, #44466, #37285, #25992 ),
 .UNSPECIFIED., .F., .F. ) 
 B_SPLINE_CURVE_WITH_KNOTS ( ( 4, 4 ),
 ( 0.5000000000000000000, 0.9074455897393720605 ),
 .UNSPECIFIED. ) 
 CURVE ( )  GEOMETRIC_REPRESENTATION_ITEM ( )  RATIONAL_B_SPLINE_CURVE ( ( 0.9999999999999906741, 0.4567392136813236414, 0.3561768502900335420, 0.6983129098261104950 ) ) 
 REPRESENTATION_ITEM ( '' )  );
#36198=ORIENTED_EDGE ( 'NONE', *, *, #42706, .F. ) ;
#36201=CARTESIAN_POINT ( 'NONE',  ( -10.85011828021597857, -12.40413123133334850, 57.32857331434495052 ) ) ;
#36202=CARTESIAN_POINT ( 'NONE',  ( -22.60238019587661995, -10.09889146956836825, 70.31178508704351771 ) ) ;
#36206=B_SPLINE_CURVE_WITH_KNOTS ( 'NONE', 3,
 ( #4165, #26555, #12259, #230, #42308, #34667, #15443, #30515, #38605, #19897 ),
 .UNSPECIFIED., .F., .F.,
 ( 4, 2, 2, 2, 4 ),
 ( 0.000000000000000000, 0.2500000000000000000, 0.5000000000000000000, 0.7500000000000000000, 1.000000000000000000 ),
 .UNSPECIFIED. ) ;
#36207=CARTESIAN_POINT ( 'NONE',  ( -16.16063032598464133, -7.467038112641824377, 60.38523865926408263 ) ) ;
#36208=CARTESIAN_POINT ( 'NONE',  ( -12.57881008754452345, -9.149975892475048056, 74.57568945445216002 ) ) ;
#36209=CIRCLE ( 'NONE', #5595, 7.000000000000000888 ) ;
#36210=EDGE_LOOP ( 'NONE', ( #43734, #7828, #20954, #46386, #10609 ) ) ;
#36211=CARTESIAN_POINT ( 'NONE',  ( -10.99655682251556144, -18.57624055219563175, 57.99209882808910521 ) ) ;
#36212=CARTESIAN_POINT ( 'NONE',  ( -12.52433193127781408, -20.42124925782731992, 71.90679425634165511 ) ) ;
#36213=CARTESIAN_POINT ( 'NONE',  ( -15.88656107989463706, -7.980151544674868980, 67.14007279409138107 ) ) ;
#36214=ORIENTED_EDGE ( 'NONE', *, *, #24685, .F. ) ;
#36215=CARTESIAN_POINT ( 'NONE',  ( -24.16181610925939793, -12.90510579204740083, 69.96170108456067283 ) ) ;
#36216=ORIENTED_EDGE ( 'NONE', *, *, #15879, .T. ) ;
#36217=CARTESIAN_POINT ( 'NONE',  ( -24.34442481654545176, -17.56831618823577301, 65.98711337262309939 ) ) ;
#36219=DIRECTION ( 'NONE',  ( 0.6172023957221189905, 0.7799807200343574776, 0.1033986416233889649 ) ) ;
#36220=ORIENTED_EDGE ( 'NONE', *, *, #21553, .F. ) ;
#36221=PLANE ( 'NONE',  #41186 ) ;
#36223=CARTESIAN_POINT ( 'NONE',  ( -10.48245863704348579, -16.06162050378864592, 64.50771356773347520 ) ) ;
#36224=CARTESIAN_POINT ( 'NONE',  ( -14.60689786731817286, -8.346551761976032324, 63.93978840692965093 ) ) ;
#36228=CARTESIAN_POINT ( 'NONE',  ( -20.52513420828390878, -21.08626482067204577, 58.87305014468301323 ) ) ;
#36229=ORIENTED_EDGE ( 'NONE', *, *, #9829, .T. ) ;
#36232=CARTESIAN_POINT ( 'NONE',  ( -11.64187585391237612, -10.11031112578646152, 67.61241562450165077 ) ) ;
#36233=DIRECTION ( 'NONE',  ( -0.9753750245375039096, -0.2205528542287732985, -7.244220463057848842E-08 ) ) ;
#36234=CARTESIAN_POINT ( 'NONE',  ( -13.35818949714929360, -21.05197827947291955, 61.70141596610112344 ) ) ;
#36236=CARTESIAN_POINT ( 'NONE',  ( -23.88415217903648369, -17.63235132829416685, 62.77360984996715842 ) ) ;
#36238=VERTEX_POINT ( 'NONE', #47294 ) ;
#36241=LINE ( 'NONE', #21242, #3789 ) ;
#36242=VERTEX_POINT ( 'NONE', #35693 ) ;
#36243=CARTESIAN_POINT ( 'NONE',  ( -11.76008542200333018, -19.01204350050032232, 68.10200740694565980 ) ) ;
#36244=CARTESIAN_POINT ( 'NONE',  ( -10.47603521207407518, -16.02136065384195973, 71.86239274348770323 ) ) ;
#36246=CARTESIAN_POINT ( 'NONE',  ( -11.64235026963700470, -18.84330375823651949, 68.21689631561287115 ) ) ;
#36247=DIRECTION ( 'NONE',  ( -1.474291233076046698E-06, -1.298191854940810726E-06, 0.9999999999980706544 ) ) ;
#36248=DIRECTION ( 'NONE',  ( -0.9939059412784551073, -0.1102314832132140487, -5.576311684675194245E-08 ) ) ;
#36249=ORIENTED_EDGE ( 'NONE', *, *, #25297, .T. ) ;
#36250=FACE_BOUND ( 'NONE', #46870, .T. ) ;
#36251=CARTESIAN_POINT ( 'NONE',  ( -23.88506662780487133, -17.50400919611850270, 65.95973823122339752 ) ) ;
#36253=CARTESIAN_POINT ( 'NONE',  ( -20.73422126667899690, -8.581213913796407411, 63.72610227039507436 ) ) ;
#36254=ORIENTED_EDGE ( 'NONE', *, *, #10036, .T. ) ;
#36256=CARTESIAN_POINT ( 'NONE',  ( -11.02370713164636129, -10.86456322469730118, 54.02312124697527906 ) ) ;
#36257=CARTESIAN_POINT ( 'NONE',  ( -18.73538018142495432, -21.73996178052156836, 72.28510691925902165 ) ) ;
#36258=CARTESIAN_POINT ( 'NONE',  ( -16.93941734680482725, -7.775588144984237005, 74.24546186738449194 ) ) ;
#36259=CARTESIAN_POINT ( 'NONE',  ( -24.20371252810814866, -12.87440185077122834, 66.58774614429587757 ) ) ;
#36260=FACE_OUTER_BOUND ( 'NONE', #7376, .T. ) ;
#36261=DIRECTION ( 'NONE',  ( -0.1464579420318390945, 0.9892168979631277281, 7.284849527811297202E-08 ) ) ;
#36262=EDGE_CURVE ( 'NONE', #8500, #27898, #17625, .T. ) ;
#36264=ORIENTED_EDGE ( 'NONE', *, *, #46851, .F. ) ;
#36266=EDGE_CURVE ( 'NONE', #13505, #34212, #38876, .T. ) ;
#36267=ADVANCED_FACE ( 'NONE', ( #46325 ), #42640, .T. ) ;
#36268=DIRECTION ( 'NONE',  ( -5.731567514496413899E-31, -1.020425574103664789E-16, -1.000000000000000000 ) ) ;
#36270=DIRECTION ( 'NONE',  ( -0.9998756790481366785, -0.01576789294826319923, -3.907472230461692677E-09 ) ) ;
#36271=AXIS2_PLACEMENT_3D ( 'NONE', #2494, #21213, #17497 ) ;
#36272=EDGE_CURVE ( 'NONE', #22946, #32101, #19514, .T. ) ;
#36273=EDGE_CURVE ( 'NONE', #1406, #19538, #42978, .T. ) ;
#36274=CARTESIAN_POINT ( 'NONE',  ( -24.59706333651279664, -12.79617740830267891, 66.48742133194130588 ) ) ;
#36275=CARTESIAN_POINT ( 'NONE',  ( -24.31823732957325745, -17.63313362019280106, 66.05861802595141796 ) ) ;
#36276=EDGE_LOOP ( 'NONE', ( #37560, #29099 ) ) ;
#36277=CARTESIAN_POINT ( 'NONE',  ( -19.30706890485013005, -22.01740903849647069, 58.64011989901568711 ) ) ;
#36278=CARTESIAN_POINT ( 'NONE',  ( -20.89788161767221197, -20.94431024770144489, 62.39999296070408974 ) ) ;
#36280=CARTESIAN_POINT ( 'NONE',  ( -17.93641254378128025, -22.24158300746090333, 61.97561672547572442 ) ) ;
#36282=ORIENTED_EDGE ( 'NONE', *, *, #10169, .F. ) ;
#36284=CARTESIAN_POINT ( 'NONE',  ( -10.42310822017611649, -15.66923192643957385, 57.77612719067403191 ) ) ;
#36285=ORIENTED_EDGE ( 'NONE', *, *, #45972, .F. ) ;
#36286=CARTESIAN_POINT ( 'NONE',  ( -20.20256548602924696, -7.896530927994315441, 73.88243076186758174 ) ) ;
#36288=AXIS2_PLACEMENT_3D ( 'NONE', #20742, #35739, #47569 ) ;
#36289=CARTESIAN_POINT ( 'NONE',  ( -24.44334717380189659, -17.30795561478116085, 69.52684539094292404 ) ) ;
#36290=CARTESIAN_POINT ( 'NONE',  ( -16.59344707466788549, -21.75974795715521282, 65.52564390620075585 ) ) ;
#36292=PLANE ( 'NONE',  #27383 ) ;
#36293=CARTESIAN_POINT ( 'NONE',  ( -24.26384900572966075, -13.06773595597165460, 69.91676003018049812 ) ) ;
#36294=CARTESIAN_POINT ( 'NONE',  ( -12.37139604325248499, -19.73008851950320519, 57.81193715039307079 ) ) ;
#36295=AXIS2_PLACEMENT_3D ( 'NONE', #44235, #47907, #33340 ) ;
#36298=CARTESIAN_POINT ( 'NONE',  ( -23.11971029740161754, -18.96910916387263768, 66.23878312252503520 ) ) ;
#36300=CARTESIAN_POINT ( 'NONE',  ( -13.91015139505516984, -8.239921989797695190, 74.30680484912956274 ) ) ;
#36301=CARTESIAN_POINT ( 'NONE',  ( -18.55453542384412557, -21.76813569768954792, 72.57951126079657911 ) ) ;
#36302=CARTESIAN_POINT ( 'NONE',  ( -10.00346675491595683, -15.47019071557144443, 57.76804009592240874 ) ) ;
#36303=ORIENTED_EDGE ( 'NONE', *, *, #3993, .T. ) ;
#36305=ORIENTED_EDGE ( 'NONE', *, *, #14808, .F. ) ;
#36306=ORIENTED_EDGE ( 'NONE', *, *, #2479, .F. ) ;
#36307=ORIENTED_EDGE ( 'NONE', *, *, #1089, .T. ) ;
#36308=CARTESIAN_POINT ( 'NONE',  ( -18.82836516733858900, -7.492696928432808434, 70.47793897115684558 ) ) ;
#36311=CARTESIAN_POINT ( 'NONE',  ( -17.43166586245951422, -7.359124596637800053, 67.13544155391683432 ) ) ;
#36312=DIRECTION ( 'NONE',  ( -0.7847243476406478013, -0.6198448985189424221, 4.433022207822356401E-08 ) ) ;
#36316=ADVANCED_FACE ( 'NONE', ( #23830 ), #975, .T. ) ;
#36318=CARTESIAN_POINT ( 'NONE',  ( -21.84079957929829874, -9.314189696129254514, 63.19153755727187161 ) ) ;
#36319=( BOUNDED_CURVE ( )  B_SPLINE_CURVE ( 3, ( #1844, #39998, #32832, #2324 ),
 .UNSPECIFIED., .F., .F. ) 
 B_SPLINE_CURVE_WITH_KNOTS ( ( 4, 4 ),
 ( 0.000000000000000000, 0.4074455897393609582 ),
 .UNSPECIFIED. ) 
 CURVE ( )  GEOMETRIC_REPRESENTATION_ITEM ( )  RATIONAL_B_SPLINE_CURVE ( ( 1.000000000000000000, 0.4567392136813415160, 0.3561768502900338196, 0.6983129098260768552 ) ) 
 REPRESENTATION_ITEM ( '' )  );
#36321=B_SPLINE_CURVE_WITH_KNOTS ( 'NONE', 1,
 ( #42684, #35271 ),
 .UNSPECIFIED., .F., .F.,
 ( 2, 2 ),
 ( 0.000000000000000000, 1.000000000000000000 ),
 .UNSPECIFIED. ) ;
#36325=CARTESIAN_POINT ( 'NONE',  ( -10.99490523303392742, -17.71099535734608210, 68.09721976853542458 ) ) ;
#36326=EDGE_CURVE ( 'NONE', #33012, #15747, #41231, .T. ) ;
#36330=ORIENTED_EDGE ( 'NONE', *, *, #15512, .F. ) ;
#36332=( BOUNDED_CURVE ( )  B_SPLINE_CURVE ( 3, ( #12754, #28262, #32202, #16676 ),
 .UNSPECIFIED., .F., .F. ) 
 B_SPLINE_CURVE_WITH_KNOTS ( ( 4, 4 ),
 ( 0.5000000000000000000, 0.9074455897393691739 ),
 .UNSPECIFIED. ) 
 CURVE ( )  GEOMETRIC_REPRESENTATION_ITEM ( )  RATIONAL_B_SPLINE_CURVE ( ( 1.000000000000011324, 0.4567392136813279158, 0.3561768502900207189, 0.6983129098261022794 ) ) 
 REPRESENTATION_ITEM ( '' )  );
#36336=CARTESIAN_POINT ( 'NONE',  ( -18.98390459359973548, -7.933620001262258192, 66.91543923465638954 ) ) ;
#36338=EDGE_LOOP ( 'NONE', ( #42404, #19862 ) ) ;
#36339=LINE ( 'NONE', #28722, #47806 ) ;
#36340=LINE ( 'NONE', #39804, #20344 ) ;
#36341=CARTESIAN_POINT ( 'NONE',  ( -21.06702863216100496, -20.84540773593990792, 65.86981821684420879 ) ) ;
#36344=CARTESIAN_POINT ( 'NONE',  ( -24.43574572327428740, -14.04659777256190623, 69.53786587444344036 ) ) ;
#36345=EDGE_LOOP ( 'NONE', ( #13064, #15319, #27324, #12057, #31070 ) ) ;
#36347=CARTESIAN_POINT ( 'NONE',  ( -24.28619334359350290, -16.42731978468327014, 59.13804568661029037 ) ) ;
#36348=ORIENTED_EDGE ( 'NONE', *, *, #1997, .F. ) ;
#36349=CARTESIAN_POINT ( 'NONE',  ( -10.35650339757981442, -17.16777133705972602, 57.80105215977741295 ) ) ;
#36350=CARTESIAN_POINT ( 'NONE',  ( -27.30749335439299585, -15.43885699713180770, 53.49999999999995026 ) ) ;
#36351=CARTESIAN_POINT ( 'NONE',  ( -24.48810873059073856, -17.17637193698283582, 73.06831349224263761 ) ) ;
#36352=CARTESIAN_POINT ( 'NONE',  ( -22.71955294612819998, -10.22924750400738070, 70.24008358658993245 ) ) ;
#36356=CARTESIAN_POINT ( 'NONE',  ( -21.55251373718371966, -8.607551109076327478, 73.77845607332120892 ) ) ;
#36357=ORIENTED_EDGE ( 'NONE', *, *, #32715, .F. ) ;
#36358=CARTESIAN_POINT ( 'NONE',  ( -10.37795889460693033, -14.56696403379599403, 68.14328054657653411 ) ) ;
#36359=CARTESIAN_POINT ( 'NONE',  ( -12.00862336911722927, -9.692924116444773475, 60.81563991731260188 ) ) ;
#36360=ORIENTED_EDGE ( 'NONE', *, *, #32912, .F. ) ;
#36362=CARTESIAN_POINT ( 'NONE',  ( -10.66160677810301038, -13.00123309306513697, 67.73832347541063825 ) ) ;
#36365=CARTESIAN_POINT ( 'NONE',  ( -23.81133579610617090, -11.82462377160084799, 59.77675971422009127 ) ) ;
#36366=CARTESIAN_POINT ( 'NONE',  ( -19.45050378258324741, -7.639967419432419860, 60.13905765641194989 ) ) ;
#36367=EDGE_CURVE ( 'NONE', #31856, #2275, #4258, .T. ) ;
#36370=CARTESIAN_POINT ( 'NONE',  ( -20.43185948505062299, -8.432683554863363184, 66.79576150497511833 ) ) ;
#36373=DIRECTION ( 'NONE',  ( -8.226841962295982234E-06, 2.386003339349608660E-06, 0.9999999999633130132 ) ) ;
#36376=CARTESIAN_POINT ( 'NONE',  ( -19.77435985551070274, -21.87886194922281646, 65.64981515446680760 ) ) ;
#36377=CARTESIAN_POINT ( 'NONE',  ( -18.95651257885568342, -7.518342207144577571, 67.06105106039149177 ) ) ;
#36378=CARTESIAN_POINT ( 'NONE',  ( -20.12289019246589206, -7.865124395032225380, 73.90592041591946781 ) ) ;
#36380=ORIENTED_EDGE ( 'NONE', *, *, #31301, .F. ) ;
#36381=CARTESIAN_POINT ( 'NONE',  ( -12.64995474452274138, -19.99670071527213366, 68.63657438322856308 ) ) ;
#36383=EDGE_CURVE ( 'NONE', #11500, #32302, #25360, .T. ) ;
#36385=CARTESIAN_POINT ( 'NONE',  ( -18.12273401612753077, -22.22646211661374593, 65.46036745194116691 ) ) ;
#36386=EDGE_CURVE ( 'NONE', #31760, #8273, #39935, .T. ) ;
#36387=ORIENTED_EDGE ( 'NONE', *, *, #34901, .T. ) ;
#36388=ADVANCED_FACE ( 'NONE', ( #16658 ), #38061, .T. ) ;
#36389=CARTESIAN_POINT ( 'NONE',  ( -10.58210918802064526, -16.28842348006157081, 71.46252756767603387 ) ) ;
#36390=CARTESIAN_POINT ( 'NONE',  ( -17.77594409791816688, -7.367433943401969998, 60.26556080592736464 ) ) ;
#36393=DIRECTION ( 'NONE',  ( 0.3926557917762825145, -0.9196855055857631189, -5.808111619717074757E-09 ) ) ;
#36395=CARTESIAN_POINT ( 'NONE',  ( -23.01149708753333201, -19.02605167522872520, 59.16945258677317554 ) ) ;
#36396=ORIENTED_EDGE ( 'NONE', *, *, #38450, .T. ) ;
#36397=CARTESIAN_POINT ( 'NONE',  ( -15.09544305450467938, -21.46351983957133669, 65.40596681500470311 ) ) ;
#36399=ORIENTED_EDGE ( 'NONE', *, *, #35505, .F. ) ;
#36400=CARTESIAN_POINT ( 'NONE',  ( -20.39466380231803200, -8.415554760933066092, 66.78104085373595922 ) ) ;
#36402=ORIENTED_EDGE ( 'NONE', *, *, #17029, .T. ) ;
#36404=( BOUNDED_CURVE ( )  B_SPLINE_CURVE ( 3, ( #1754, #24408, #28344, #20950 ),
 .UNSPECIFIED., .F., .F. ) 
 B_SPLINE_CURVE_WITH_KNOTS ( ( 4, 4 ),
 ( 0.9074455897393640669, 1.000000000000000000 ),
 .UNSPECIFIED. ) 
 CURVE ( )  GEOMETRIC_REPRESENTATION_ITEM ( )  RATIONAL_B_SPLINE_CURVE ( ( 0.6983129098260925094, 0.7760317562606977582, 0.8765941196520002920, 1.000000000000000000 ) ) 
 REPRESENTATION_ITEM ( '' )  );
#36405=CARTESIAN_POINT ( 'NONE',  ( -19.84080129957490612, -21.85712737670714390, 65.57830891090566183 ) ) ;
#36407=ORIENTED_EDGE ( 'NONE', *, *, #44912, .F. ) ;
#36408=CARTESIAN_POINT ( 'NONE',  ( -13.33151401730585306, -20.55006798877650454, 58.06122216312902395 ) ) ;
#36409=CARTESIAN_POINT ( 'NONE',  ( -17.13503149044196405, -7.764836982087095052, 70.77563787455143540 ) ) ;
#36410=B_SPLINE_CURVE_WITH_KNOTS ( 'NONE', 3,
 ( #42989, #1369, #12461, #9028, #24047, #31908, #27245, #15906, #42271, #1624 ),
 .UNSPECIFIED., .F., .F.,
 ( 4, 2, 2, 2, 4 ),
 ( 0.000000000000000000, 0.2500000000000000000, 0.5000000000000000000, 0.7500000000000000000, 1.000000000000000000 ),
 .UNSPECIFIED. ) ;
#36411=CARTESIAN_POINT ( 'NONE',  ( -24.16575376147897458, -12.74704232990201547, 69.77243002240838621 ) ) ;
#36412=DIRECTION ( 'NONE',  ( -7.166348394334737576E-06, 1.030346079289304524E-05, 0.9999999999212411117 ) ) ;
#36415=ORIENTED_EDGE ( 'NONE', *, *, #10297, .T. ) ;
#36416=CARTESIAN_POINT ( 'NONE',  ( -11.76162984098805708, -18.92470629761549006, 68.28977573079643548 ) ) ;
#36418=ORIENTED_EDGE ( 'NONE', *, *, #11192, .F. ) ;
#36419=CARTESIAN_POINT ( 'NONE',  ( -20.77205709590035454, -8.153671001013822917, 63.45088146699718834 ) ) ;
#36424=ORIENTED_EDGE ( 'NONE', *, *, #28049, .T. ) ;
#36425=CARTESIAN_POINT ( 'NONE',  ( -10.54479291434905797, -13.51458092965912705, 74.75105665847443959 ) ) ;
#36426=CARTESIAN_POINT ( 'NONE',  ( -14.16498672988215191, -8.109065889264286398, 70.91612917212019340 ) ) ;
#36427=LINE ( 'NONE', #2706, #9894 ) ;
#36430=ORIENTED_EDGE ( 'NONE', *, *, #40392, .T. ) ;
#36431=CARTESIAN_POINT ( 'NONE',  ( -17.02294265308554344, -7.369891754266058470, 74.13831026345251018 ) ) ;
#36432=DIRECTION ( 'NONE',  ( 0.04108628546905852136, 0.9991556020692448081, -1.019563928860402442E-16 ) ) ;
#36433=ADVANCED_FACE ( 'NONE', ( #20369 ), #45005, .T. ) ;
#36434=CARTESIAN_POINT ( 'NONE',  ( -10.01222935355948529, -14.05624259999535042, 61.01847049672689138 ) ) ;
#36435=CARTESIAN_POINT ( 'NONE',  ( -11.51240771850610933, -10.27427218717217627, 71.08237763624090633 ) ) ;
#36437=CARTESIAN_POINT ( 'NONE',  ( -24.23620318903103410, -13.19799477795856824, 59.43555865750501965 ) ) ;
#36439=CARTESIAN_POINT ( 'NONE',  ( -10.89357934009856521, -11.22367372050276302, 64.19236096111531253 ) ) ;
#36441=ORIENTED_EDGE ( 'NONE', *, *, #1758, .F. ) ;
#36442=CARTESIAN_POINT ( 'NONE',  ( -10.96149970135419061, -18.51576062833312974, 58.06360531077050524 ) ) ;
#36444=CARTESIAN_POINT ( 'NONE',  ( -19.75127562985729313, -21.88641334670167282, 65.66474991182012388 ) ) ;
#36445=( BOUNDED_CURVE ( )  B_SPLINE_CURVE ( 3, ( #2699, #32735, #20940, #10099 ),
 .UNSPECIFIED., .F., .F. ) 
 B_SPLINE_CURVE_WITH_KNOTS ( ( 4, 4 ),
 ( 0.9074455897393601811, 1.000000000000000000 ),
 .UNSPECIFIED. ) 
 CURVE ( )  GEOMETRIC_REPRESENTATION_ITEM ( )  RATIONAL_B_SPLINE_CURVE ( ( 0.6983129098260881795, 0.7760317562606939834, 0.8765941196519979606, 1.000000000000000000 ) ) 
 REPRESENTATION_ITEM ( '' )  );
#36448=CARTESIAN_POINT ( 'NONE',  ( -19.81036900135710965, -9.838928235415560053, 53.88362224778186516 ) ) ;
#36450=LINE ( 'NONE', #19155, #34643 ) ;
#36451=CARTESIAN_POINT ( 'NONE',  ( -22.56207008003183745, -19.63703213565221262, 72.92928497383269359 ) ) ;
#36452=DIRECTION ( 'NONE',  ( 0.2479245821708705166, 0.9687793358424813261, 2.626836608334030890E-18 ) ) ;
#36453=ORIENTED_EDGE ( 'NONE', *, *, #42489, .T. ) ;
#36454=FACE_OUTER_BOUND ( 'NONE', #21607, .T. ) ;
#36455=FACE_OUTER_BOUND ( 'NONE', #45837, .T. ) ;
#36457=EDGE_CURVE ( 'NONE', #28688, #47772, #11844, .T. ) ;
#36458=CARTESIAN_POINT ( 'NONE',  ( -10.77704936818085812, -17.00411804736975085, 57.70262972533568302 ) ) ;
#36462=( BOUNDED_CURVE ( )  B_SPLINE_CURVE ( 3, ( #37565, #16070, #12391, #3364 ),
 .UNSPECIFIED., .F., .F. ) 
 B_SPLINE_CURVE_WITH_KNOTS ( ( 4, 4 ),
 ( 0.9074455897393681747, 1.000000000000000000 ),
 .UNSPECIFIED. ) 
 CURVE ( )  GEOMETRIC_REPRESENTATION_ITEM ( )  RATIONAL_B_SPLINE_CURVE ( ( 0.6983129098261009471, 0.7760317562607050856, 0.8765941196520047329, 1.000000000000000000 ) ) 
 REPRESENTATION_ITEM ( '' )  );
#36463=CARTESIAN_POINT ( 'NONE',  ( -24.87123160714014958, -14.59964084223042491, 62.89791924484052998 ) ) ;
#36465=DIRECTION ( 'NONE',  ( 0.04287186434519785205, 0.9990805789562555717, -2.806673972535357682E-09 ) ) ;
#36466=DIRECTION ( 'NONE',  ( -0.3739781583979218116, -0.9274375111247651349, -6.296758467538796555E-09 ) ) ;
#36467=FACE_OUTER_BOUND ( 'NONE', #42341, .T. ) ;
#36468=DIRECTION ( 'NONE',  ( 6.885933443815673122E-06, -1.077603661396111343E-05, 0.9999999999182304089 ) ) ;
#36469=EDGE_CURVE ( 'NONE', #45223, #3454, #41526, .T. ) ;
#36474=CARTESIAN_POINT ( 'NONE',  ( -22.07022430586338402, -11.86582892075562334, 53.49899999999994549 ) ) ;
#36475=ORIENTED_EDGE ( 'NONE', *, *, #40837, .F. ) ;
#36476=CARTESIAN_POINT ( 'NONE',  ( -20.66848101912799862, -8.549761622307149977, 60.12653141481577990 ) ) ;
#36478=CARTESIAN_POINT ( 'NONE',  ( -23.19494370299929287, -18.77118727246694263, 65.82389430425217824 ) ) ;
#36479=CARTESIAN_POINT ( 'NONE',  ( -13.76436681951595098, -7.422085961289871747, 53.49999999999995026 ) ) ;
#36480=DIRECTION ( 'NONE',  ( -0.3478314405900309603, -0.9375570856950864451, 0.000000000000000000 ) ) ;
#36481=CARTESIAN_POINT ( 'NONE',  ( -23.85820692815676480, -17.57049044119773029, 66.05430223995341521 ) ) ;
#36482=DIRECTION ( 'NONE',  ( -0.6771828760946863035, 0.7358147540815750398, -3.419290845356464001E-09 ) ) ;
#36483=( BOUNDED_CURVE ( )  B_SPLINE_CURVE ( 3, ( #16280, #34774, #1045, #26913 ),
 .UNSPECIFIED., .F., .F. ) 
 B_SPLINE_CURVE_WITH_KNOTS ( ( 4, 4 ),
 ( 0.9074455897393621795, 1.000000000000000000 ),
 .UNSPECIFIED. ) 
 CURVE ( )  GEOMETRIC_REPRESENTATION_ITEM ( )  RATIONAL_B_SPLINE_CURVE ( ( 0.6983129098260796308, 0.7760317562606866559, 0.8765941196519934087, 1.000000000000000000 ) ) 
 REPRESENTATION_ITEM ( '' )  );
#36484=CARTESIAN_POINT ( 'NONE',  ( -20.49170831689750827, -8.461258797198503601, 63.59649424907591708 ) ) ;
#36485=ORIENTED_EDGE ( 'NONE', *, *, #42074, .T. ) ;
#36487=CARTESIAN_POINT ( 'NONE',  ( -10.63004074901718532, -12.92571453866564646, 67.75304464120749515 ) ) ;
#36489=CARTESIAN_POINT ( 'NONE',  ( -24.18362101178863455, -17.94180522593430283, 59.18095321646488571 ) ) ;
#36490=CARTESIAN_POINT ( 'NONE',  ( -24.08517543038346531, -12.49907855475201579, 73.52753481283211556 ) ) ;
#36491=DIRECTION ( 'NONE',  ( -0.3478314405900309603, -0.9375570856950864451, 0.000000000000000000 ) ) ;
#36492=VERTEX_POINT ( 'NONE', #19595 ) ;
#36496=CARTESIAN_POINT ( 'NONE',  ( -13.24492651052040415, -9.193567913827360272, 63.92448906866182767 ) ) ;
#36497=CARTESIAN_POINT ( 'NONE',  ( -11.68672781637937419, -10.05669048882576533, 67.68392176937598492 ) ) ;
#36498=EDGE_CURVE ( 'NONE', #32446, #4358, #46578, .T. ) ;
#36499=CARTESIAN_POINT ( 'NONE',  ( -24.59908880092032035, -12.80353012418438396, 66.49520876175452599 ) ) ;
#36500=DIRECTION ( 'NONE',  ( 0.4846961512978548159, 0.8746825943832683414, 4.196010046976493442E-08 ) ) ;
#36501=ORIENTED_EDGE ( 'NONE', *, *, #36262, .F. ) ;
#36502=EDGE_CURVE ( 'NONE', #14412, #8372, #26984, .T. ) ;
#36505=ORIENTED_EDGE ( 'NONE', *, *, #35921, .F. ) ;
#36506=DIRECTION ( 'NONE',  ( -3.395770065602591412E-06, -1.105252671792169116E-06, 0.9999999999936236561 ) ) ;
#36507=VECTOR ( 'NONE', #10020, 1000.000000000000227 ) ;
#36508=ORIENTED_EDGE ( 'NONE', *, *, #3571, .F. ) ;
#36509=CARTESIAN_POINT ( 'NONE',  ( -19.44142144650348314, -21.98165757830647138, 62.18158996068683564 ) ) ;
#36510=CARTESIAN_POINT ( 'NONE',  ( -10.03904597514415009, -13.82694077737217242, 57.56329639008353638 ) ) ;
#36511=CARTESIAN_POINT ( 'NONE',  ( -14.78754745127378634, -8.270772244812137686, 60.61996282000563241 ) ) ;
#36512=VERTEX_POINT ( 'NONE', #41513 ) ;
#36515=CARTESIAN_POINT ( 'NONE',  ( -24.46950595589296285, -14.38832865607273703, 73.26704460715303924 ) ) ;
#36516=CARTESIAN_POINT ( 'NONE',  ( -24.86288141285521647, -20.97301237610655988, 54.50428052266514101 ) ) ;
#36517=CARTESIAN_POINT ( 'NONE',  ( -11.04811567812601680, -17.69860408370704263, 71.56718199152911097 ) ) ;
#36518=ORIENTED_EDGE ( 'NONE', *, *, #30628, .T. ) ;
#36520=CARTESIAN_POINT ( 'NONE',  ( -17.70776835051902864, -22.25388969026799657, 58.52057945155585372 ) ) ;
#36522=ADVANCED_FACE ( 'NONE', ( #45231 ), #4573, .T. ) ;
#36526=CARTESIAN_POINT ( 'NONE',  ( -15.93106588071581697, -7.910958181831522218, 60.35595345230024833 ) ) ;
#36527=CARTESIAN_POINT ( 'NONE',  ( -23.54569203310520464, -19.05535937789667145, 65.93894149164137275 ) ) ;
#36529=CARTESIAN_POINT ( 'NONE',  ( -18.44790534074380517, -7.884421568168953343, 73.85566781112635226 ) ) ;
#36531=CARTESIAN_POINT ( 'NONE',  ( -18.20082364030551503, -7.794104720362528660, 73.99631248270939921 ) ) ;
#36535=ORIENTED_EDGE ( 'NONE', *, *, #37983, .F. ) ;
#36537=CARTESIAN_POINT ( 'NONE',  ( -19.82413079548422274, -21.27835043604049048, 75.49999999999994316 ) ) ;
#36538=FACE_OUTER_BOUND ( 'NONE', #259, .T. ) ;
#36539=CARTESIAN_POINT ( 'NONE',  ( -15.81235419205221504, -7.945607373518417837, 67.42535135806457447 ) ) ;
#36540=ORIENTED_EDGE ( 'NONE', *, *, #12934, .T. ) ;
#36546=CARTESIAN_POINT ( 'NONE',  ( -10.75396668955334256, -17.10360140286105590, 64.92739389533053895 ) ) ;
#36547=CARTESIAN_POINT ( 'NONE',  ( -10.86061992081550365, -17.24265423301508449, 61.38416481539552194 ) ) ;
#36549=ORIENTED_EDGE ( 'NONE', *, *, #15208, .T. ) ;
#36550=EDGE_CURVE ( 'NONE', #8569, #18139, #18206, .T. ) ;
#36553=CARTESIAN_POINT ( 'NONE',  ( -24.87417962317557496, -14.80849170857717567, 59.42795673386487465 ) ) ;
#36555=CYLINDRICAL_SURFACE ( 'NONE', #22662, 0.1499999999999988565 ) ;
#36556=ORIENTED_EDGE ( 'NONE', *, *, #3440, .F. ) ;
#36558=CARTESIAN_POINT ( 'NONE',  ( -24.83666526594744184, -14.06169473043846629, 73.28418025887795295 ) ) ;
#36560=ORIENTED_EDGE ( 'NONE', *, *, #35300, .F. ) ;
#36562=CARTESIAN_POINT ( 'NONE',  ( -23.12431869989520550, -10.01221758024046338, 66.79828185159925624 ) ) ;
#36564=ORIENTED_EDGE ( 'NONE', *, *, #12502, .F. ) ;
#36565=DIRECTION ( 'NONE',  ( 9.352133743349324758E-06, 6.779811746737758835E-06, 0.9999999999332858103 ) ) ;
#36566=CARTESIAN_POINT ( 'NONE',  ( -21.64297170217681554, -9.150934564753532285, 73.74561934610416358 ) ) ;
#36567=CARTESIAN_POINT ( 'NONE',  ( -10.70629277777140942, -11.58826885910880478, 71.28135027068064744 ) ) ;
#36568=ORIENTED_EDGE ( 'NONE', *, *, #17512, .F. ) ;
#36570=CARTESIAN_POINT ( 'NONE',  ( -13.82836502510361854, -20.88256612802230450, 61.67213144371572042 ) ) ;
#36571=VERTEX_POINT ( 'NONE', #41267 ) ;
#36573=ADVANCED_FACE ( 'NONE', ( #46910 ), #24568, .T. ) ;
#36574=FACE_OUTER_BOUND ( 'NONE', #37552, .T. ) ;
#36575=DIRECTION ( 'NONE',  ( 0.3926557917762824590, -0.9196855055857630079, -5.808111619717073930E-09 ) ) ;
#36581=( BOUNDED_CURVE ( )  B_SPLINE_CURVE ( 3, ( #32335, #43169, #35528, #24706 ),
 .UNSPECIFIED., .F., .F. ) 
 B_SPLINE_CURVE_WITH_KNOTS ( ( 4, 4 ),
 ( 0.4074455897393678416, 0.5000000000000000000 ),
 .UNSPECIFIED. ) 
 CURVE ( )  GEOMETRIC_REPRESENTATION_ITEM ( )  RATIONAL_B_SPLINE_CURVE ( ( 0.6983129098260949519, 0.7760317562607005337, 0.8765941196520024015, 1.000000000000001110 ) ) 
 REPRESENTATION_ITEM ( '' )  );
#36583=CARTESIAN_POINT ( 'NONE',  ( -15.41904641700715217, -7.634001813009263060, 74.19490365927923392 ) ) ;
#36584=ORIENTED_EDGE ( 'NONE', *, *, #39048, .F. ) ;
#36585=CARTESIAN_POINT ( 'NONE',  ( -10.36617775085144899, -14.83726598580069300, 68.01367321887373407 ) ) ;
#36586=EDGE_CURVE ( 'NONE', #30331, #35502, #32740, .T. ) ;
#36588=CYLINDRICAL_SURFACE ( 'NONE', #6270, 0.1499999999999999667 ) ;
#36590=ORIENTED_EDGE ( 'NONE', *, *, #9661, .F. ) ;
#36591=ADVANCED_FACE ( 'NONE', ( #16615 ), #43226, .T. ) ;
#36593=CARTESIAN_POINT ( 'NONE',  ( -13.43773910423563400, -20.62433115109003268, 58.33177939114180788 ) ) ;
#36594=CARTESIAN_POINT ( 'NONE',  ( -11.54557276264065280, -18.70100022596745859, 65.04707046112368118 ) ) ;
#36595=B_SPLINE_CURVE_WITH_KNOTS ( 'NONE', 1,
 ( #45937, #23780 ),
 .UNSPECIFIED., .F., .F.,
 ( 2, 2 ),
 ( 0.000000000000000000, 1.000000000000000000 ),
 .UNSPECIFIED. ) ;
#36596=CARTESIAN_POINT ( 'NONE',  ( -12.77796340496265692, -17.75258416873320400, 54.07175714974880520 ) ) ;
#36597=( BOUNDED_CURVE ( )  B_SPLINE_CURVE ( 3, ( #41012, #18578, #620, #37051 ),
 .UNSPECIFIED., .F., .F. ) 
 B_SPLINE_CURVE_WITH_KNOTS ( ( 4, 4 ),
 ( 1.570796326794896780, 1.780235837034217505 ),
 .UNSPECIFIED. ) 
 CURVE ( )  GEOMETRIC_REPRESENTATION_ITEM ( )  RATIONAL_B_SPLINE_CURVE ( ( 1.000000000000000000, 0.9963479302455154896, 0.9963479302455154896, 1.000000000000000000 ) ) 
 REPRESENTATION_ITEM ( '' )  );
#36599=CARTESIAN_POINT ( 'NONE',  ( -22.06352374043166265, -8.980015506435984562, 63.37649162950052784 ) ) ;
#36600=CARTESIAN_POINT ( 'NONE',  ( -22.73317970229575025, -20.03675580610048712, 72.83055794290764595 ) ) ;
#36602=VERTEX_POINT ( 'NONE', #12689 ) ;
#36603=CARTESIAN_POINT ( 'NONE',  ( -22.92319755143357085, -10.39759026177046763, 63.37185995336191979 ) ) ;
#36604=EDGE_CURVE ( 'NONE', #14795, #12703, #34775, .T. ) ;
#36605=B_SPLINE_CURVE_WITH_KNOTS ( 'NONE', 3,
 ( #27203, #42230, #6007, #24968, #21029, #2069, #3028, #32821, #39504, #9950 ),
 .UNSPECIFIED., .F., .F.,
 ( 4, 2, 2, 2, 4 ),
 ( 0.000000000000000000, 0.2500000000000000000, 0.5000000000000000000, 0.7500000000000000000, 1.000000000000000000 ),
 .UNSPECIFIED. ) ;
#36606=CARTESIAN_POINT ( 'NONE',  ( -21.41863048803932656, -8.999699081277377388, 73.61600897546567523 ) ) ;
#36609=DIRECTION ( 'NONE',  ( -2.699622400625883127E-06, 1.161037828378819543E-05, 0.9999999999289554964 ) ) ;
#36610=ORIENTED_EDGE ( 'NONE', *, *, #27947, .T. ) ;
#36611=B_SPLINE_CURVE_WITH_KNOTS ( 'NONE', 1,
 ( #6713, #20767 ),
 .UNSPECIFIED., .F., .F.,
 ( 2, 2 ),
 ( 0.000000000000000000, 1.000000000000000000 ),
 .UNSPECIFIED. ) ;
#36613=( BOUNDED_CURVE ( )  B_SPLINE_CURVE ( 3, ( #10027, #9797, #6088, #40070 ),
 .UNSPECIFIED., .F., .F. ) 
 B_SPLINE_CURVE_WITH_KNOTS ( ( 4, 4 ),
 ( 0.4074455897393624570, 0.5000000000000000000 ),
 .UNSPECIFIED. ) 
 CURVE ( )  GEOMETRIC_REPRESENTATION_ITEM ( )  RATIONAL_B_SPLINE_CURVE ( ( 0.6983129098260902889, 0.7760317562606902086, 0.8765941196519916323, 0.9999999999999910072 ) ) 
 REPRESENTATION_ITEM ( '' )  );
#36615=VERTEX_POINT ( 'NONE', #42499 ) ;
#36616=CARTESIAN_POINT ( 'NONE',  ( -12.68362485313667598, -20.02768789089244805, 68.63097676073942921 ) ) ;
#36617=CARTESIAN_POINT ( 'NONE',  ( -11.91452160938943550, -19.82401263394628543, 58.18328287794685139 ) ) ;
#36618=FACE_OUTER_BOUND ( 'NONE', #26289, .T. ) ;
#36619=CARTESIAN_POINT ( 'NONE',  ( -10.44503168371052837, -15.82779754136115002, 68.39256704124431963 ) ) ;
#36620=ORIENTED_EDGE ( 'NONE', *, *, #16330, .F. ) ;
#36621=DIRECTION ( 'NONE',  ( -0.9990515194385546360, -0.04354378839186318767, 1.103613758316041215E-08 ) ) ;
#36622=CARTESIAN_POINT ( 'NONE',  ( -17.84735332803204599, -7.371153730986438113, 60.19565454701680807 ) ) ;
#36624=LINE ( 'NONE', #13735, #10225 ) ;
#36625=ORIENTED_EDGE ( 'NONE', *, *, #9945, .T. ) ;
#36626=CARTESIAN_POINT ( 'NONE',  ( -14.76715853668754797, -21.76932111121406521, 61.78600440926723536 ) ) ;
#36628=CARTESIAN_POINT ( 'NONE',  ( -23.88415222675040184, -17.63235122089636775, 62.47360984996718258 ) ) ;
#36632=CARTESIAN_POINT ( 'NONE',  ( -10.97888661679622047, -11.94317331668165671, 71.08860792922808969 ) ) ;
#36633=CARTESIAN_POINT ( 'NONE',  ( -12.45502217426375680, -20.36096218193827667, 71.99308960123012469 ) ) ;
#36635=LINE ( 'NONE', #39872, #40947 ) ;
#36637=CARTESIAN_POINT ( 'NONE',  ( -23.66263630406368534, -11.51900531544784911, 70.30699535439772774 ) ) ;
#36638=ORIENTED_EDGE ( 'NONE', *, *, #27445, .F. ) ;
#36641=AXIS2_PLACEMENT_3D ( 'NONE', #30246, #22859, #12238 ) ;
#36642=EDGE_CURVE ( 'NONE', #36141, #15790, #12896, .T. ) ;
#36643=CARTESIAN_POINT ( 'NONE',  ( -11.33476867595667770, -19.10151316506851416, 68.40185013497388411 ) ) ;
#36644=CARTESIAN_POINT ( 'NONE',  ( -23.34092642400682038, -10.28208056094584677, 59.78698708435513254 ) ) ;
#36645=ORIENTED_EDGE ( 'NONE', *, *, #9469, .F. ) ;
#36646=ORIENTED_EDGE ( 'NONE', *, *, #37401, .F. ) ;
#36647=ADVANCED_FACE ( 'NONE', ( #12922 ), #16116, .T. ) ;
#36648=CARTESIAN_POINT ( 'NONE',  ( -22.67603917253425294, -10.10156321767594179, 73.89649722025401957 ) ) ;
#36649=CARTESIAN_POINT ( 'NONE',  ( -11.83910118423700553, -10.58927088369822300, 71.15996259575267402 ) ) ;
#36653=DIRECTION ( 'NONE',  ( 0.9840843158728909135, -0.1445225939547943317, 0.1033986416233889927 ) ) ;
#36654=DIRECTION ( 'NONE',  ( 0.2573866790907599622, 0.9663084897829603559, 6.714855467380900338E-08 ) ) ;
#36655=CARTESIAN_POINT ( 'NONE',  ( -23.66133310609451712, -18.88359296917171903, 69.40876596050124192 ) ) ;
#36657=EDGE_LOOP ( 'NONE', ( #41148, #47287, #34351, #36845 ) ) ;
#36658=CARTESIAN_POINT ( 'NONE',  ( -10.57110035550071103, -13.38215360593666325, 74.97817647590578360 ) ) ;
#36659=CARTESIAN_POINT ( 'NONE',  ( -24.87351451566537364, -14.94990356866029657, 59.42955486997114178 ) ) ;
#36660=EDGE_CURVE ( 'NONE', #2205, #15682, #40600, .T. ) ;
#36661=ORIENTED_EDGE ( 'NONE', *, *, #36859, .T. ) ;
#36662=ORIENTED_EDGE ( 'NONE', *, *, #33234, .T. ) ;
#36663=LINE ( 'NONE', #41122, #39054 ) ;
#36664=CARTESIAN_POINT ( 'NONE',  ( -23.35152121466412467, -19.32258585407967999, 59.02264109267150616 ) ) ;
#36665=DIRECTION ( 'NONE',  ( -2.696738946685428783E-06, -1.002714487109772720E-05, -0.9999999999460920108 ) ) ;
#36666=EDGE_LOOP ( 'NONE', ( #16086, #3862, #47505, #45511, #10756 ) ) ;
#36667=VECTOR ( 'NONE', #16153, 1000.000000000000114 ) ;
#36668=CARTESIAN_POINT ( 'NONE',  ( -23.77561729583671379, -17.75197182879437463, 59.30378408728073225 ) ) ;
#36669=ORIENTED_EDGE ( 'NONE', *, *, #4295, .F. ) ;
#36670=CARTESIAN_POINT ( 'NONE',  ( -22.34365193135296579, -19.87012687442179981, 62.39006291346853317 ) ) ;
#36673=CARTESIAN_POINT ( 'NONE',  ( -24.87289997924709439, -14.67112824012948202, 62.82801159608117558 ) ) ;
#36675=ADVANCED_FACE ( 'NONE', ( #47406 ), #39655, .T. ) ;
#36676=ORIENTED_EDGE ( 'NONE', *, *, #41520, .T. ) ;
#36677=CARTESIAN_POINT ( 'NONE',  ( -20.47136568995129480, -10.23054578351414001, 53.49999999999995026 ) ) ;
#36680=CARTESIAN_POINT ( 'NONE',  ( -17.42409385541300892, -14.80920654474439324, 77.49999999999994316 ) ) ;
#36683=CARTESIAN_POINT ( 'NONE',  ( -19.42896492416523913, -21.56812594671148275, 61.99503644571810668 ) ) ;
#36686=DIRECTION ( 'NONE',  ( 1.143861049860740968E-05, -2.837703139598260652E-06, 0.9999999999305527743 ) ) ;
#36688=CARTESIAN_POINT ( 'NONE',  ( -24.87090184113336733, -14.58551080922006271, 62.85150006646590981 ) ) ;
#36689=CARTESIAN_POINT ( 'NONE',  ( -9.995738364564658696, -14.24060042610175358, 64.50308557176904856 ) ) ;
#36690=CARTESIAN_POINT ( 'NONE',  ( -14.47983227664519212, -7.965588925009814858, 63.90483403727078837 ) ) ;
#36691=CARTESIAN_POINT ( 'NONE',  ( -13.12613380977788147, -20.89454282643029259, 58.16154686733092660 ) ) ;
#36692=CARTESIAN_POINT ( 'NONE',  ( -16.16221656818315466, -22.15164012088281709, 58.32939616168999208 ) ) ;
#36693=CARTESIAN_POINT ( 'NONE',  ( -24.21189024148803171, -13.09820213895421759, 62.83264126992417431 ) ) ;
#36694=ORIENTED_EDGE ( 'NONE', *, *, #8938, .F. ) ;
#36698=CARTESIAN_POINT ( 'NONE',  ( -20.67810541806404956, -8.031554304750532225, 54.02312124697527196 ) ) ;
#36700=CARTESIAN_POINT ( 'NONE',  ( -23.96044199021409327, -11.23292130238350772, 66.53559200982742539 ) ) ;
#36703=CARTESIAN_POINT ( 'NONE',  ( -10.27345454978659944, -12.71824136398891980, 64.45331520391344782 ) ) ;
#36704=ADVANCED_FACE ( 'NONE', ( #29646 ), #6026, .T. ) ;
#36705=CARTESIAN_POINT ( 'NONE',  ( -14.67242798431547968, -21.73322265534233111, 58.27962637798393786 ) ) ;
#36706=DIRECTION ( 'NONE',  ( -5.731567514496413899E-31, -1.020425574103664789E-16, -1.000000000000000000 ) ) ;
#36707=CARTESIAN_POINT ( 'NONE',  ( -12.12013830951134885, -9.577504261232970606, 57.18911913778111256 ) ) ;
#36708=AXIS2_PLACEMENT_3D ( 'NONE', #27481, #27242, #11989 ) ;
#36709=CARTESIAN_POINT ( 'NONE',  ( -11.44360937317491711, -19.25177985856723595, 71.78662246600895003 ) ) ;
#36710=AXIS2_PLACEMENT_3D ( 'NONE', #5663, #40345, #25567 ) ;
#36711=EDGE_CURVE ( 'NONE', #44664, #47803, #16045, .T. ) ;
#36712=CARTESIAN_POINT ( 'NONE',  ( -23.69410982483307038, -17.92519756231842720, 59.11451459836140288 ) ) ;
#36713=VERTEX_POINT ( 'NONE', #43961 ) ;
#36715=CARTESIAN_POINT ( 'NONE',  ( -13.18904211892902367, -11.30002761096173280, 53.49899999999994549 ) ) ;
#36716=AXIS2_PLACEMENT_3D ( 'NONE', #7781, #22800, #4088 ) ;
#36717=CARTESIAN_POINT ( 'NONE',  ( -24.26595340233995302, -13.32969406988797623, 59.36267925071750540 ) ) ;
#36718=CARTESIAN_POINT ( 'NONE',  ( -21.08710664733760609, -20.77481365697375182, 69.33833681463573839 ) ) ;
#36719=ADVANCED_FACE ( 'NONE', ( #18298 ), #33069, .T. ) ;
#36723=ORIENTED_EDGE ( 'NONE', *, *, #41377, .T. ) ;
#36727=CARTESIAN_POINT ( 'NONE',  ( -17.05929182965467916, -21.79975568072098469, 72.45077872430272237 ) ) ;
#36729=AXIS2_PLACEMENT_3D ( 'NONE', #1177, #17092, #36053 ) ;
#36730=( BOUNDED_CURVE ( )  B_SPLINE_CURVE ( 3, ( #5944, #12360, #27380, #42416 ),
 .UNSPECIFIED., .F., .F. ) 
 B_SPLINE_CURVE_WITH_KNOTS ( ( 4, 4 ),
 ( 0.000000000000000000, 0.4074455897393696735 ),
 .UNSPECIFIED. ) 
 CURVE ( )  GEOMETRIC_REPRESENTATION_ITEM ( )  RATIONAL_B_SPLINE_CURVE ( ( 1.000000000000000000, 0.4567392136813298587, 0.3561768502900295452, 0.6983129098260991707 ) ) 
 REPRESENTATION_ITEM ( '' )  );
#36731=CARTESIAN_POINT ( 'NONE',  ( -15.43285674489986903, -7.630071079539528789, 74.21952314256675720 ) ) ;
#36733=ORIENTED_EDGE ( 'NONE', *, *, #305, .T. ) ;
#36734=LINE ( 'NONE', #33789, #42598 ) ;
#36735=ORIENTED_EDGE ( 'NONE', *, *, #5398, .F. ) ;
#36736=CARTESIAN_POINT ( 'NONE',  ( -17.97727801652185065, -22.23869005747018335, 61.98197623854611749 ) ) ;
#36737=EDGE_CURVE ( 'NONE', #31355, #46961, #679, .T. ) ;
#36738=( BOUNDED_SURFACE ( )  B_SPLINE_SURFACE ( 3, 1, ( 
 ( #41425, #7717 ),
 ( #34520, #22983 ),
 ( #30858, #15303 ),
 ( #37970, #45869 ),
 ( #4256, #19266 ),
 ( #34269, #3840 ),
 ( #14151, #32876 ) ),
 .UNSPECIFIED., .T., .F., .F. ) 
 B_SPLINE_SURFACE_WITH_KNOTS ( ( 4, 3, 4 ),
 ( 2, 2 ),
 ( 0.000000000000000000, 0.5000000000000000000, 1.000000000000000000 ),
 ( 0.000000000000000000, 1.000000000000000000 ),
 .UNSPECIFIED. ) 
 GEOMETRIC_REPRESENTATION_ITEM ( )  RATIONAL_B_SPLINE_SURFACE ( (
 ( 1.000000000000000000, 1.000000000000000000),
 ( 0.3333333333333335369, 0.3333333333333330373),
 ( 0.3333333333333335369, 0.3333333333333330373),
 ( 1.000000000000000000, 1.000000000000000000),
 ( 0.3333333333333333703, 0.3333333333333333703),
 ( 0.3333333333333333703, 0.3333333333333333703),
 ( 1.000000000000000000, 1.000000000000000000) ) ) 
 REPRESENTATION_ITEM ( '' )  SURFACE ( )  );
#36741=AXIS2_PLACEMENT_3D ( 'NONE', #19460, #513, #30566 ) ;
#36742=EDGE_LOOP ( 'NONE', ( #27158, #39920, #41385, #46742, #420 ) ) ;
#36743=CARTESIAN_POINT ( 'NONE',  ( -10.52422472645684870, -17.61911478008853749, 68.21226617000660042 ) ) ;
#36744=CARTESIAN_POINT ( 'NONE',  ( -10.72530867274958233, -17.00760959713300480, 57.97288447305808745 ) ) ;
#36745=CARTESIAN_POINT ( 'NONE',  ( -23.08280660609100465, -10.60377317445056811, 59.61675562601556067 ) ) ;
#36746=VERTEX_POINT ( 'NONE', #2746 ) ;
#36747=CARTESIAN_POINT ( 'NONE',  ( -20.12998554757678704, -7.867921253476878540, 73.91370774657193010 ) ) ;
#36748=CARTESIAN_POINT ( 'NONE',  ( -24.82002243867330549, -13.90704071453223456, 73.23616177064057808 ) ) ;
#36750=CARTESIAN_POINT ( 'NONE',  ( -24.38570565625541064, -13.64691002463509939, 59.50701104079105619 ) ) ;
#36751=CARTESIAN_POINT ( 'NONE',  ( -22.17130319910813085, -20.55096425825585982, 58.87947600183965591 ) ) ;
#36753=CYLINDRICAL_SURFACE ( 'NONE', #16404, 0.1499999999999990508 ) ;
#36755=AXIS2_PLACEMENT_3D ( 'NONE', #42865, #24398, #9136 ) ;
#36757=CARTESIAN_POINT ( 'NONE',  ( -23.66133370835450833, -18.88359203746988868, 69.40876704922922613 ) ) ;
#36758=CARTESIAN_POINT ( 'NONE',  ( -14.25068826455714621, -8.513811653308138716, 70.87957628655816222 ) ) ;
#36759=CARTESIAN_POINT ( 'NONE',  ( -24.22122181710478017, -12.92668648255967234, 62.71775301689540782 ) ) ;
#36760=ORIENTED_EDGE ( 'NONE', *, *, #8665, .T. ) ;
#36761=CARTESIAN_POINT ( 'NONE',  ( -10.70313322336788175, -12.85206431338615118, 64.56836087214048803 ) ) ;
#36763=CARTESIAN_POINT ( 'NONE',  ( -10.44916039635137217, -15.83526825291551177, 64.50771589744864798 ) ) ;
#36765=ORIENTED_EDGE ( 'NONE', *, *, #48322, .F. ) ;
#36769=ORIENTED_EDGE ( 'NONE', *, *, #43177, .T. ) ;
#36770=EDGE_LOOP ( 'NONE', ( #41491, #20628, #17564, #29817, #25820 ) ) ;
#36773=EDGE_CURVE ( 'NONE', #18567, #27537, #4719, .T. ) ;
#36774=CARTESIAN_POINT ( 'NONE',  ( -11.06793303470118950, -10.92167721944563397, 60.86541164553911187 ) ) ;
#36775=VECTOR ( 'NONE', #35036, 1000.000000000000000 ) ;
#36777=FACE_OUTER_BOUND ( 'NONE', #10277, .T. ) ;
#36778=AXIS2_PLACEMENT_3D ( 'NONE', #16550, #30633, #19531 ) ;
#36780=VERTEX_POINT ( 'NONE', #17752 ) ;
#36781=VERTEX_POINT ( 'NONE', #32075 ) ;
#36783=B_SPLINE_CURVE_WITH_KNOTS ( 'NONE', 3,
 ( #2453, #46309, #24864, #5430, #32007, #39397, #20193, #12565, #35205, #20690 ),
 .UNSPECIFIED., .F., .F.,
 ( 4, 2, 2, 2, 4 ),
 ( 0.1272669073658869721, 0.2522669073439838816, 0.3772669073220807912, 0.5022669073001777562, 0.6272669072782746102 ),
 .UNSPECIFIED. ) ;
#36787=B_SPLINE_CURVE_WITH_KNOTS ( 'NONE', 1,
 ( #12439, #8769 ),
 .UNSPECIFIED., .F., .F.,
 ( 2, 2 ),
 ( 0.000000000000000000, 1.000000000000000000 ),
 .UNSPECIFIED. ) ;
#36789=EDGE_CURVE ( 'NONE', #33324, #39625, #27993, .T. ) ;
#36790=EDGE_CURVE ( 'NONE', #17249, #46845, #1891, .T. ) ;
#36793=EDGE_CURVE ( 'NONE', #34024, #32237, #24241, .T. ) ;
#36794=EDGE_CURVE ( 'NONE', #48564, #13641, #43, .T. ) ;
#36796=CARTESIAN_POINT ( 'NONE',  ( -24.87413924702786971, -14.81707641383176721, 59.34961947317660957 ) ) ;
#36798=ORIENTED_EDGE ( 'NONE', *, *, #48071, .F. ) ;
#36799=CYLINDRICAL_SURFACE ( 'NONE', #43914, 0.1500000000000005218 ) ;
#36800=ORIENTED_EDGE ( 'NONE', *, *, #32943, .F. ) ;
#36801=CARTESIAN_POINT ( 'NONE',  ( -22.39330545970614850, -9.879000042779363611, 73.67264350515011984 ) ) ;
#36802=B_SPLINE_CURVE_WITH_KNOTS ( 'NONE', 3,
 ( #45161, #48336, #3288, #26676, #22995, #44423, #7978, #25940, #11168, #40957 ),
 .UNSPECIFIED., .F., .F.,
 ( 4, 2, 2, 2, 4 ),
 ( 0.000000000000000000, 0.2500000000000000000, 0.5000000000000000000, 0.7500000000000000000, 1.000000000000000000 ),
 .UNSPECIFIED. ) ;
#36803=CARTESIAN_POINT ( 'NONE',  ( -18.22959801979823879, -21.76314743224078185, 69.09898171275015955 ) ) ;
#36804=CARTESIAN_POINT ( 'NONE',  ( -10.59051903643958958, -13.04363995460383663, 74.82250634059326444 ) ) ;
#36806=ORIENTED_EDGE ( 'NONE', *, *, #18789, .F. ) ;
#36807=CARTESIAN_POINT ( 'NONE',  ( -19.04074625787506037, -7.997132879027503805, 67.12901749300219478 ) ) ;
#36809=CARTESIAN_POINT ( 'NONE',  ( -24.21483728131241975, -11.74476288741533914, 59.62202341653743076 ) ) ;
#36810=CARTESIAN_POINT ( 'NONE',  ( -19.37484620200115160, -7.619050568204919216, 60.14588398245204814 ) ) ;
#36811=DIRECTION ( 'NONE',  ( -5.731567514496413899E-31, -1.020425574103664789E-16, -1.000000000000000000 ) ) ;
#36812=ORIENTED_EDGE ( 'NONE', *, *, #13481, .F. ) ;
#36814=CARTESIAN_POINT ( 'NONE',  ( -21.34582186320181307, -20.66775149956831115, 72.82446429489806405 ) ) ;
#36818=EDGE_LOOP ( 'NONE', ( #12086, #29289, #31486, #46294 ) ) ;
#36819=CARTESIAN_POINT ( 'NONE',  ( -13.29845860553889203, -21.01266621750898267, 61.63151044148704472 ) ) ;
#36820=ORIENTED_EDGE ( 'NONE', *, *, #1151, .T. ) ;
#36822=CARTESIAN_POINT ( 'NONE',  ( -23.78500256881436314, -11.88707711785523635, 59.48235732566631384 ) ) ;
#36823=EDGE_CURVE ( 'NONE', #3056, #1995, #6000, .T. ) ;
#36824=CARTESIAN_POINT ( 'NONE',  ( -24.08517543038346531, -12.49907855475201579, 73.52753481283211556 ) ) ;
#36825=CARTESIAN_POINT ( 'NONE',  ( -23.21026474594941291, -18.83721105783783401, 65.82949252296415921 ) ) ;
#36827=CARTESIAN_POINT ( 'NONE',  ( -22.06133437076497827, -9.563835992883470638, 59.95001055572075899 ) ) ;
#36829=EDGE_LOOP ( 'NONE', ( #28658, #42887, #11903, #29505, #36760 ) ) ;
#36830=CARTESIAN_POINT ( 'NONE',  ( -14.77006348030517380, -21.34072373105164999, 58.46058126903869834 ) ) ;
#36831=ORIENTED_EDGE ( 'NONE', *, *, #11817, .T. ) ;
#36833=CARTESIAN_POINT ( 'NONE',  ( -11.91307475890685552, -9.794993484201089728, 60.67262835395951015 ) ) ;
#36835=ORIENTED_EDGE ( 'NONE', *, *, #12942, .F. ) ;
#36836=CARTESIAN_POINT ( 'NONE',  ( -14.86359179994916246, -21.80616968373489684, 65.29251951080507865 ) ) ;
#36839=CARTESIAN_POINT ( 'NONE',  ( -23.47153285936109413, -19.16039112161479352, 62.47594094552156463 ) ) ;
#36840=FACE_OUTER_BOUND ( 'NONE', #46644, .T. ) ;
#36842=DIRECTION ( 'NONE',  ( -0.8017593358536259096, -0.5976470257363776240, 1.209213344977627713E-07 ) ) ;
#36843=CARTESIAN_POINT ( 'NONE',  ( -20.57278596605185683, -8.057205637650621810, 66.89608763938375091 ) ) ;
#36844=ORIENTED_EDGE ( 'NONE', *, *, #39968, .F. ) ;
#36845=ORIENTED_EDGE ( 'NONE', *, *, #33315, .T. ) ;
#36849=CARTESIAN_POINT ( 'NONE',  ( -21.07890896836238781, -21.30130458668023508, 62.27504751322158683 ) ) ;
#36850=DIRECTION ( 'NONE',  ( 0.9372362738803844406, 0.3486949482324239735, -5.386914174890154601E-09 ) ) ;
#36851=CARTESIAN_POINT ( 'NONE',  ( -24.42398663107514523, -15.65075326911586906, 73.01775867260030850 ) ) ;
#36852=PRODUCT_DEFINITION_FORMATION_WITH_SPECIFIED_SOURCE ( 'ANY', '', #45689, .NOT_KNOWN. ) ;
#36853=ORIENTED_EDGE ( 'NONE', *, *, #45438, .T. ) ;
#36856=VECTOR ( 'NONE', #7902, 1000.000000000000114 ) ;
#36857=ORIENTED_EDGE ( 'NONE', *, *, #9392, .F. ) ;
#36859=EDGE_CURVE ( 'NONE', #24381, #23558, #23634, .T. ) ;
#36861=CARTESIAN_POINT ( 'NONE',  ( -10.20197030601470090, -12.78660143320473175, 54.27966884056655061 ) ) ;
#36863=CARTESIAN_POINT ( 'NONE',  ( -18.14458250172319609, -22.22429833870308613, 65.44557911879493872 ) ) ;
#36864=AXIS2_PLACEMENT_3D ( 'NONE', #15265, #31219, #12749 ) ;
#36866=EDGE_CURVE ( 'NONE', #2066, #43726, #38777, .T. ) ;
#36867=EDGE_CURVE ( 'NONE', #5915, #10474, #37636, .T. ) ;
#36868=FACE_OUTER_BOUND ( 'NONE', #31818, .T. ) ;
#36869=CARTESIAN_POINT ( 'NONE',  ( -24.23636277187043220, -17.82529184948975498, 62.58865552117998021 ) ) ;
#36870=ORIENTED_EDGE ( 'NONE', *, *, #27733, .T. ) ;
#36871=CYLINDRICAL_SURFACE ( 'NONE', #22613, 0.1500000000000060452 ) ;
#36872=( BOUNDED_CURVE ( )  B_SPLINE_CURVE ( 3, ( #4579, #24274, #5314, #23795 ),
 .UNSPECIFIED., .F., .F. ) 
 B_SPLINE_CURVE_WITH_KNOTS ( ( 4, 4 ),
 ( 0.000000000000000000, 0.4074455897393652326 ),
 .UNSPECIFIED. ) 
 CURVE ( )  GEOMETRIC_REPRESENTATION_ITEM ( )  RATIONAL_B_SPLINE_CURVE ( ( 1.000000000000000000, 0.4567392136813419046, 0.3561768502900339861, 0.6983129098260761891 ) ) 
 REPRESENTATION_ITEM ( '' )  );
#36873=FACE_OUTER_BOUND ( 'NONE', #31702, .T. ) ;
#36875=DIRECTION ( 'NONE',  ( -2.083496777882594458E-06, 1.347747145367441676E-07, 0.9999999999978204102 ) ) ;
#36876=EDGE_LOOP ( 'NONE', ( #43095, #29627, #32777, #9582, #47743 ) ) ;
#36877=DIRECTION ( 'NONE',  ( -0.1922068328301544116, -0.9813544382196450755, 7.804899501296266931E-08 ) ) ;
#36878=CARTESIAN_POINT ( 'NONE',  ( -17.63866254341385442, -7.362211269489866261, 63.66561597723832477 ) ) ;
#36879=ORIENTED_EDGE ( 'NONE', *, *, #41189, .T. ) ;
#36880=CARTESIAN_POINT ( 'NONE',  ( -22.42594789675818845, -19.77792426076253918, 69.45945937764655298 ) ) ;
#36881=EDGE_CURVE ( 'NONE', #33555, #22004, #41154, .T. ) ;
#36882=CARTESIAN_POINT ( 'NONE',  ( -20.57117620866707242, -8.500566317031267971, 63.31121523393445472 ) ) ;
#36886=CARTESIAN_POINT ( 'NONE',  ( -11.10019564437503448, -18.74767688259557730, 61.38372506178604482 ) ) ;
#36887=( BOUNDED_CURVE ( )  B_SPLINE_CURVE ( 3, ( #21172, #43088, #24634, #39636 ),
 .UNSPECIFIED., .F., .F. ) 
 B_SPLINE_CURVE_WITH_KNOTS ( ( 4, 4 ),
 ( 0.4074455897393687853, 0.5000000000000000000 ),
 .UNSPECIFIED. ) 
 CURVE ( )  GEOMETRIC_REPRESENTATION_ITEM ( )  RATIONAL_B_SPLINE_CURVE ( ( 0.6983129098261063872, 0.7760317562606898756, 0.8765941196519819734, 0.9999999999999684697 ) ) 
 REPRESENTATION_ITEM ( '' )  );
#36888=CARTESIAN_POINT ( 'NONE',  ( -24.86497429546398763, -14.44044012822152467, 66.28318476119724778 ) ) ;
#36890=( BOUNDED_CURVE ( )  B_SPLINE_CURVE ( 3, ( #17560, #3282, #10198, #47619 ),
 .UNSPECIFIED., .F., .F. ) 
 B_SPLINE_CURVE_WITH_KNOTS ( ( 4, 4 ),
 ( 1.570796326794896780, 1.780235837034218616 ),
 .UNSPECIFIED. ) 
 CURVE ( )  GEOMETRIC_REPRESENTATION_ITEM ( )  RATIONAL_B_SPLINE_CURVE ( ( 1.000000000000000000, 0.9963479302455153785, 0.9963479302455153785, 1.000000000000000000 ) ) 
 REPRESENTATION_ITEM ( '' )  );
#36891=CYLINDRICAL_SURFACE ( 'NONE', #23971, 0.1500000000000014655 ) ;
#36894=CARTESIAN_POINT ( 'NONE',  ( -11.96004319712522168, -10.43380364626374579, 67.60782902827304497 ) ) ;
#36895=FACE_OUTER_BOUND ( 'NONE', #459, .T. ) ;
#36896=ORIENTED_EDGE ( 'NONE', *, *, #8960, .T. ) ;
#36898=CARTESIAN_POINT ( 'NONE',  ( -22.54258147833521875, -19.66265161326780486, 69.17418017405046271 ) ) ;
#36899=DIRECTION ( 'NONE',  ( -1.568615307090388417E-06, -3.599470258889626763E-09, 0.9999999999987696508 ) ) ;
#36900=CARTESIAN_POINT ( 'NONE',  ( -19.20719371956520050, -7.575738887753711737, 63.58089232527501622 ) ) ;
#36901=AXIS2_PLACEMENT_3D ( 'NONE', #43227, #9502, #2090 ) ;
#36903=FACE_OUTER_BOUND ( 'NONE', #1985, .T. ) ;
#36905=CARTESIAN_POINT ( 'NONE',  ( -15.48563737764182591, -8.027819004131977465, 70.49500973495348433 ) ) ;
#36906=( BOUNDED_CURVE ( )  B_SPLINE_CURVE ( 3, ( #43880, #26358, #41368, #26861 ),
 .UNSPECIFIED., .F., .F. ) 
 B_SPLINE_CURVE_WITH_KNOTS ( ( 4, 4 ),
 ( 0.9074455897393596260, 1.000000000000000000 ),
 .UNSPECIFIED. ) 
 CURVE ( )  GEOMETRIC_REPRESENTATION_ITEM ( )  RATIONAL_B_SPLINE_CURVE ( ( 0.6983129098260846268, 0.7760317562606909858, 0.8765941196519960732, 1.000000000000000000 ) ) 
 REPRESENTATION_ITEM ( '' )  );
#36907=CARTESIAN_POINT ( 'NONE',  ( -16.57554889599778747, -22.21081103083016117, 65.41059783760971413 ) ) ;
#36908=ORIENTED_EDGE ( 'NONE', *, *, #23834, .F. ) ;
#36909=CARTESIAN_POINT ( 'NONE',  ( -10.54472383408941205, -13.51494001709767723, 74.90490956355360197 ) ) ;
#36910=CARTESIAN_POINT ( 'NONE',  ( -17.39742520082695165, -7.759256980592265762, 67.17039592192074338 ) ) ;
#36913=ORIENTED_EDGE ( 'NONE', *, *, #10375, .F. ) ;
#36915=EDGE_CURVE ( 'NONE', #20377, #7647, #28231, .T. ) ;
#36917=CARTESIAN_POINT ( 'NONE',  ( -24.44757306576362410, -14.11227934896924374, 66.33859978849633876 ) ) ;
#36919=DIRECTION ( 'NONE',  ( -0.2737502900231350011, -0.9618007999124593699, 5.400150802763565900E-08 ) ) ;
#36920=DIRECTION ( 'NONE',  ( -0.6205284308219183309, -0.7841839494287597967, -1.702810348471078804E-17 ) ) ;
#36921=ORIENTED_EDGE ( 'NONE', *, *, #40487, .T. ) ;
#36923=CARTESIAN_POINT ( 'NONE',  ( -13.60238289842205894, -8.884932333444998775, 57.26967755503795132 ) ) ;
#36924=EDGE_CURVE ( 'NONE', #36746, #42977, #35289, .T. ) ;
#36925=CARTESIAN_POINT ( 'NONE',  ( -12.52591726580351228, -9.195683270288645517, 74.50418291613799227 ) ) ;
#36926=ORIENTED_EDGE ( 'NONE', *, *, #336, .F. ) ;
#36927=ADVANCED_FACE ( 'NONE', ( #19966 ), #42380, .T. ) ;
#36928=CARTESIAN_POINT ( 'NONE',  ( -13.71293426195967413, -21.26916566922604801, 68.64120525947689089 ) ) ;
#36929=CARTESIAN_POINT ( 'NONE',  ( -24.87123163304818974, -14.59964195235338735, 62.89791815715346956 ) ) ;
#36930=ADVANCED_FACE ( 'NONE', ( #4957 ), #30821, .F. ) ;
#36931=ORIENTED_EDGE ( 'NONE', *, *, #7541, .T. ) ;
#36932=FACE_OUTER_BOUND ( 'NONE', #33865, .T. ) ;
#36933=VERTEX_POINT ( 'NONE', #20200 ) ;
#36934=CARTESIAN_POINT ( 'NONE',  ( -23.78676187654788521, -10.93361199230012559, 73.54688693628270357 ) ) ;
#36935=FACE_OUTER_BOUND ( 'NONE', #36100, .T. ) ;
#36936=VERTEX_POINT ( 'NONE', #42631 ) ;
#36937=CARTESIAN_POINT ( 'NONE',  ( -24.16075099676623950, -17.99041029048389717, 59.20389616614811956 ) ) ;
#36939=EDGE_CURVE ( 'NONE', #14865, #8232, #8649, .T. ) ;
#36942=CARTESIAN_POINT ( 'NONE',  ( -10.76587724080305541, -16.97019452347059953, 57.98760522221959945 ) ) ;
#36943=CARTESIAN_POINT ( 'NONE',  ( -16.50258162057404832, -20.23145840177225452, 54.07175714974879099 ) ) ;
#36944=ORIENTED_EDGE ( 'NONE', *, *, #19563, .T. ) ;
#36945=CARTESIAN_POINT ( 'NONE',  ( -24.87290000513101873, -14.67112934921935974, 62.82801050733710468 ) ) ;
#36946=CARTESIAN_POINT ( 'NONE',  ( -22.98355915621633372, -9.849807724373423667, 70.11904361266189767 ) ) ;
#36948=DIRECTION ( 'NONE',  ( -0.8459089628457130416, -0.5333273165489313961, 7.771812504399801304E-08 ) ) ;
#36953=CARTESIAN_POINT ( 'NONE',  ( -11.24997143734453076, -18.22902874506724302, 61.42143955951387113 ) ) ;
#36954=CARTESIAN_POINT ( 'NONE',  ( -21.14277848257653503, -8.274947154434103780, 53.76227901944321275 ) ) ;
#36956=CARTESIAN_POINT ( 'NONE',  ( -19.30128557755455532, -21.60500301973953086, 58.81035253397666196 ) ) ;
#36958=CARTESIAN_POINT ( 'NONE',  ( -11.29272682956604967, -18.18986319395907714, 57.99641719428725395 ) ) ;
#36960=CARTESIAN_POINT ( 'NONE',  ( -12.55420354710856223, -9.778633195358828800, 57.20008522322477518 ) ) ;
#36962=CARTESIAN_POINT ( 'NONE',  ( -24.74075702715665770, -16.21285080831185965, 62.77823949964436423 ) ) ;
#36964=AXIS2_PLACEMENT_3D ( 'NONE', #27494, #20352, #9522 ) ;
#36965=CARTESIAN_POINT ( 'NONE',  ( -23.44980453451080749, -18.46889374286061525, 73.06368236440982855 ) ) ;
#36968=DIRECTION ( 'NONE',  ( 0.1186632576870824268, -0.9929345553837299887, -6.051931680293946494E-08 ) ) ;
#36969=LINE ( 'NONE', #36715, #22732 ) ;
#36971=FACE_OUTER_BOUND ( 'NONE', #15422, .T. ) ;
#36973=ADVANCED_FACE ( 'NONE', ( #12327 ), #33005, .T. ) ;
#36974=CARTESIAN_POINT ( 'NONE',  ( -13.71293330176565384, -21.26916511146244915, 68.64120417180296840 ) ) ;
#36975=DIRECTION ( 'NONE',  ( -1.184681380772507928E-05, -1.827615836447136132E-06, 0.9999999999281563579 ) ) ;
#36979=ORIENTED_EDGE ( 'NONE', *, *, #18327, .T. ) ;
#36981=CARTESIAN_POINT ( 'NONE',  ( -17.34602462345121410, -7.359448551298330088, 67.15893111912230040 ) ) ;
#36982=B_SPLINE_CURVE_WITH_KNOTS ( 'NONE', 1,
 ( #21084, #36079 ),
 .UNSPECIFIED., .F., .F.,
 ( 2, 2 ),
 ( 0.000000000000000000, 1.000000000000000000 ),
 .UNSPECIFIED. ) ;
#36983=CARTESIAN_POINT ( 'NONE',  ( -18.97210877009940688, -7.521729958488855061, 66.94425830142937173 ) ) ;
#36984=( BOUNDED_CURVE ( )  B_SPLINE_CURVE ( 3, ( #47106, #20999, #39955, #35281 ),
 .UNSPECIFIED., .F., .F. ) 
 B_SPLINE_CURVE_WITH_KNOTS ( ( 4, 4 ),
 ( 0.9074455897393605142, 1.000000000000000000 ),
 .UNSPECIFIED. ) 
 CURVE ( )  GEOMETRIC_REPRESENTATION_ITEM ( )  RATIONAL_B_SPLINE_CURVE ( ( 0.6983129098260913992, 0.7760317562606968700, 0.8765941196519997369, 1.000000000000000000 ) ) 
 REPRESENTATION_ITEM ( '' )  );
#36985=CARTESIAN_POINT ( 'NONE',  ( -22.75923480142028055, -10.27751027444597653, 66.84182257657300852 ) ) ;
#36986=CARTESIAN_POINT ( 'NONE',  ( -9.975950761882481643, -15.00625170120774321, 74.91123542948268721 ) ) ;
#36987=ORIENTED_EDGE ( 'NONE', *, *, #6979, .T. ) ;
#36988=EDGE_CURVE ( 'NONE', #9191, #42180, #43503, .T. ) ;
#36993=ORIENTED_EDGE ( 'NONE', *, *, #14251, .F. ) ;
#36995=AXIS2_PLACEMENT_3D ( 'NONE', #680, #38089, #15190 ) ;
#36997=ORIENTED_EDGE ( 'NONE', *, *, #15489, .T. ) ;
#36998=ADVANCED_FACE ( 'NONE', ( #19727 ), #16006, .T. ) ;
#36999=CYLINDRICAL_SURFACE ( 'NONE', #4014, 0.1500000000000050460 ) ;
#37000=CARTESIAN_POINT ( 'NONE',  ( -21.23484681875272884, -20.74088929683185611, 69.33978048267414351 ) ) ;
#37001=CARTESIAN_POINT ( 'NONE',  ( -23.34092642400682038, -10.28208056094584677, 59.78698708435513254 ) ) ;
#37002=EDGE_LOOP ( 'NONE', ( #48227, #22478, #46829, #18130, #19644 ) ) ;
#37003=CARTESIAN_POINT ( 'NONE',  ( -11.96697528417469236, -19.88111336767673976, 58.10399280105138331 ) ) ;
#37005=AXIS2_PLACEMENT_3D ( 'NONE', #3888, #15178, #42279 ) ;
#37006=ADVANCED_FACE ( 'NONE', ( #28567 ), #10576, .T. ) ;
#37007=CARTESIAN_POINT ( 'NONE',  ( -14.98563576580806789, -21.37212005543727855, 65.33426489834504025 ) ) ;
#37008=CARTESIAN_POINT ( 'NONE',  ( -23.96921983750137031, -17.29140838963852289, 66.13460527988867454 ) ) ;
#37010=PLANE ( 'NONE',  #32878 ) ;
#37011=DIRECTION ( 'NONE',  ( -0.4780674886490097197, 0.8783231047267436864, 5.292596395488306339E-08 ) ) ;
#37012=DIRECTION ( 'NONE',  ( -7.381188794381864007E-06, -5.670466972807880762E-06, -0.9999999999566818731 ) ) ;
#37013=DIRECTION ( 'NONE',  ( 2.210955087992717862E-06, -1.097707075699772489E-06, 0.9999999999969533260 ) ) ;
#37015=ORIENTED_EDGE ( 'NONE', *, *, #30763, .T. ) ;
#37016=CARTESIAN_POINT ( 'NONE',  ( -24.65023673758593148, -12.99629830290576038, 63.01759453279318279 ) ) ;
#37018=ORIENTED_EDGE ( 'NONE', *, *, #27685, .F. ) ;
#37019=CARTESIAN_POINT ( 'NONE',  ( -11.34285589096144697, -19.11310387458220816, 68.35543075210530617 ) ) ;
#37020=DIRECTION ( 'NONE',  ( 0.3688590060343663324, -0.9294853595766526810, 9.484706316669550371E-17 ) ) ;
#37021=EDGE_LOOP ( 'NONE', ( #48510, #13894, #40172, #40636, #8106 ) ) ;
#37024=ORIENTED_EDGE ( 'NONE', *, *, #39616, .F. ) ;
#37025=EDGE_LOOP ( 'NONE', ( #47235, #8802, #3730, #13435, #45209 ) ) ;
#37028=CARTESIAN_POINT ( 'NONE',  ( -14.30826096781649426, -8.540783494585491908, 71.02957638424210529 ) ) ;
#37029=CARTESIAN_POINT ( 'NONE',  ( -11.77169895589660520, -10.59578386207264700, 74.43885051664024388 ) ) ;
#37030=( BOUNDED_CURVE ( )  B_SPLINE_CURVE ( 3, ( #26158, #33029, #40923, #18504 ),
 .UNSPECIFIED., .F., .F. ) 
 B_SPLINE_CURVE_WITH_KNOTS ( ( 4, 4 ),
 ( 0.000000000000000000, 0.4074455897393634562 ),
 .UNSPECIFIED. ) 
 CURVE ( )  GEOMETRIC_REPRESENTATION_ITEM ( )  RATIONAL_B_SPLINE_CURVE ( ( 1.000000000000000000, 0.4567392136813276937, 0.3561768502900287126, 0.6983129098261030565 ) ) 
 REPRESENTATION_ITEM ( '' )  );
#37032=CARTESIAN_POINT ( 'NONE',  ( -14.10256395084115866, -8.140532207465255965, 70.84462205307964666 ) ) ;
#37033=CARTESIAN_POINT ( 'NONE',  ( -13.49267557974227394, -8.956801037788498121, 60.45422421514565059 ) ) ;
#37035=ORIENTED_EDGE ( 'NONE', *, *, #31774, .F. ) ;
#37036=ORIENTED_EDGE ( 'NONE', *, *, #30819, .T. ) ;
#37038=CARTESIAN_POINT ( 'NONE',  ( -11.42962470904260464, -10.38539412368214521, 74.62380407152070916 ) ) ;
#37039=VECTOR ( 'NONE', #16090, 1000.000000000000227 ) ;
#37040=LINE ( 'NONE', #48375, #5645 ) ;
#37043=( BOUNDED_CURVE ( )  B_SPLINE_CURVE ( 3, ( #14507, #10852, #14038, #33477 ),
 .UNSPECIFIED., .F., .F. ) 
 B_SPLINE_CURVE_WITH_KNOTS ( ( 4, 4 ),
 ( 0.9074455897393643999, 1.000000000000000000 ),
 .UNSPECIFIED. ) 
 CURVE ( )  GEOMETRIC_REPRESENTATION_ITEM ( )  RATIONAL_B_SPLINE_CURVE ( ( 0.6983129098261049439, 0.7760317562607085273, 0.8765941196520068424, 1.000000000000000000 ) ) 
 REPRESENTATION_ITEM ( '' )  );
#37044=ORIENTED_EDGE ( 'NONE', *, *, #25231, .T. ) ;
#37045=LINE ( 'NONE', #40508, #46552 ) ;
#37048=CARTESIAN_POINT ( 'NONE',  ( -10.49189908542464522, -16.09426454567519116, 68.26295692486267797 ) ) ;
#37049=CARTESIAN_POINT ( 'NONE',  ( -16.26195973558533581, -21.76306465430365122, 58.57113428431811997 ) ) ;
#37050=EDGE_LOOP ( 'NONE', ( #46694, #8539, #11986, #39434, #20820 ) ) ;
#37051=CARTESIAN_POINT ( 'NONE',  ( -10.00368807899092971, -15.89896712085359098, 54.27966884056655061 ) ) ;
#37052=ORIENTED_EDGE ( 'NONE', *, *, #2479, .T. ) ;
#37053=ADVANCED_FACE ( 'NONE', ( #28802 ), #48135, .T. ) ;
#37054=VECTOR ( 'NONE', #36432, 1000.000000000000000 ) ;
#37056=CARTESIAN_POINT ( 'NONE',  ( -24.83515304063678286, -14.04764234229505959, 73.23776096988058271 ) ) ;
#37058=CARTESIAN_POINT ( 'NONE',  ( -10.39648919455610709, -12.33579563135258361, 57.46710844504804072 ) ) ;
#37061=CARTESIAN_POINT ( 'NONE',  ( -11.14114473067313682, -10.80566704772025233, 57.32407823191172014 ) ) ;
#37062=CARTESIAN_POINT ( 'NONE',  ( -11.77169715766437008, -10.59578624409953207, 74.58885051661056309 ) ) ;
#37063=EDGE_CURVE ( 'NONE', #37232, #38712, #43840, .T. ) ;
#37064=CARTESIAN_POINT ( 'NONE',  ( -12.21606489183646715, -19.56099602313843988, 57.92682377985823194 ) ) ;
#37065=CARTESIAN_POINT ( 'NONE',  ( -11.02242957576233451, -11.85532881267382166, 74.57312195644870201 ) ) ;
#37067=DIRECTION ( 'NONE',  ( -0.1648596854219664953, -0.9863170302304249404, 7.074492695208252801E-08 ) ) ;
#37069=FACE_BOUND ( 'NONE', #15241, .T. ) ;
#37070=B_SPLINE_CURVE_WITH_KNOTS ( 'NONE', 3,
 ( #32786, #2522, #29101, #28394, #9684, #2034, #9193, #47584, #24210, #20519 ),
 .UNSPECIFIED., .F., .F.,
 ( 4, 2, 2, 2, 4 ),
 ( 0.000000000000000000, 0.2500000000000000000, 0.5000000000000000000, 0.7500000000000000000, 1.000000000000000000 ),
 .UNSPECIFIED. ) ;
#37072=CARTESIAN_POINT ( 'NONE',  ( -13.12613380977788147, -20.89454282643029259, 58.16154686733092660 ) ) ;
#37073=CARTESIAN_POINT ( 'NONE',  ( -14.17292126938155761, -21.07377676424729884, 68.61192020317307083 ) ) ;
#37076=DIRECTION ( 'NONE',  ( 0.9968684284758859704, -0.07907803935364898784, 1.831731161803828914E-08 ) ) ;
#37079=DIRECTION ( 'NONE',  ( -1.205044182522204318E-05, -2.694341353802685858E-06, -0.9999999999237636494 ) ) ;
#37080=CARTESIAN_POINT ( 'NONE',  ( -15.81671074304997582, -7.936704070960259649, 74.22418700304095296 ) ) ;
#37082=ORIENTED_EDGE ( 'NONE', *, *, #16821, .T. ) ;
#37083=CARTESIAN_POINT ( 'NONE',  ( -10.37182134788606369, -14.70778158825885207, 67.74311464738552502 ) ) ;
#37084=ADVANCED_FACE ( 'NONE', ( #47999 ), #2693, .T. ) ;
#37085=CARTESIAN_POINT ( 'NONE',  ( -16.98261326800368209, -21.79527086262147861, 72.16543221550985265 ) ) ;
#37087=EDGE_LOOP ( 'NONE', ( #36806, #952 ) ) ;
#37088=ORIENTED_EDGE ( 'NONE', *, *, #41730, .F. ) ;
#37090=CARTESIAN_POINT ( 'NONE',  ( -20.06838235508133650, -8.265300555148282768, 66.93671294127740623 ) ) ;
#37091=CARTESIAN_POINT ( 'NONE',  ( -20.19231670334047735, -8.325423520194950910, 70.40100341277891971 ) ) ;
#37092=CARTESIAN_POINT ( 'NONE',  ( -10.60168030567061415, -13.23530239299793365, 74.78890765637994775 ) ) ;
#37094=CARTESIAN_POINT ( 'NONE',  ( -14.21691894016960411, -8.585707489940052284, 74.42784435416010069 ) ) ;
#37095=CARTESIAN_POINT ( 'NONE',  ( -14.80708969572697775, -21.78456432865329973, 61.75787710153574039 ) ) ;
#37096=VERTEX_POINT ( 'NONE', #13274 ) ;
#37097=ORIENTED_EDGE ( 'NONE', *, *, #39826, .F. ) ;
#37103=VERTEX_POINT ( 'NONE', #43354 ) ;
#37105=EDGE_LOOP ( 'NONE', ( #34862, #39680, #13469, #23357, #13699 ) ) ;
#37106=CARTESIAN_POINT ( 'NONE',  ( -16.97946104448713101, -21.84517140583366057, 72.46543221429990922 ) ) ;
#37107=PLANE ( 'NONE',  #5670 ) ;
#37109=ORIENTED_EDGE ( 'NONE', *, *, #15376, .F. ) ;
#37111=CARTESIAN_POINT ( 'NONE',  ( -24.82475127085388422, -15.66597259679895693, 73.11808347143848152 ) ) ;
#37112=CARTESIAN_POINT ( 'NONE',  ( -21.59336496936327165, -9.186214804599407202, 66.94684602522839612 ) ) ;
#37113=ORIENTED_EDGE ( 'NONE', *, *, #16079, .T. ) ;
#37114=CARTESIAN_POINT ( 'NONE',  ( -17.66159697976433307, -21.85550285805611637, 58.42025434932890704 ) ) ;
#37115=CARTESIAN_POINT ( 'NONE',  ( -10.11824970337647223, -16.26811690260224452, 71.56254994910038647 ) ) ;
#37116=ORIENTED_EDGE ( 'NONE', *, *, #32978, .F. ) ;
#37117=CARTESIAN_POINT ( 'NONE',  ( -24.77132058643702450, -16.04239701017138131, 66.21324923524157668 ) ) ;
#37118=ORIENTED_EDGE ( 'NONE', *, *, #35239, .F. ) ;
#37119=CARTESIAN_POINT ( 'NONE',  ( -24.45577199812615632, -12.20047074031916168, 54.27966884056650088 ) ) ;
#37120=CARTESIAN_POINT ( 'NONE',  ( -11.55269001482513325, -18.62078876646939563, 65.04707126775019788 ) ) ;
#37121=ORIENTED_EDGE ( 'NONE', *, *, #21406, .T. ) ;
#37122=CARTESIAN_POINT ( 'NONE',  ( -13.06813783877040969, -9.265530354883374287, 67.66470656304637998 ) ) ;
#37123=CARTESIAN_POINT ( 'NONE',  ( -20.17268404433175633, -8.371407854712250796, 70.55100341248845552 ) ) ;
#37124=VERTEX_POINT ( 'NONE', #39642 ) ;
#37125=DIRECTION ( 'NONE',  ( -1.070267892829395584E-05, -6.715522050485540099E-06, 0.9999999999201771850 ) ) ;
#37126=CARTESIAN_POINT ( 'NONE',  ( -11.06712629860931152, -18.69414434431124761, 61.39215439313597500 ) ) ;
#37127=LINE ( 'NONE', #3174, #21974 ) ;
#37128=ORIENTED_EDGE ( 'NONE', *, *, #8088, .T. ) ;
#37129=DIRECTION ( 'NONE',  ( 1.474291235753705251E-06, 1.298191845539703006E-06, -0.9999999999980705434 ) ) ;
#37131=PLANE ( 'NONE',  #16449 ) ;
#37135=EDGE_LOOP ( 'NONE', ( #47987, #8259, #39287, #23868, #3433 ) ) ;
#37136=ORIENTED_EDGE ( 'NONE', *, *, #38457, .F. ) ;
#37137=DIRECTION ( 'NONE',  ( -0.4749924142254752235, -0.8799898899579782219, -8.916637576350563827E-09 ) ) ;
#37138=CARTESIAN_POINT ( 'NONE',  ( -24.31477923169101629, -16.30090137217950641, 59.40860294853779777 ) ) ;
#37139=CYLINDRICAL_SURFACE ( 'NONE', #11542, 0.1499999999999998834 ) ;
#37141=DIRECTION ( 'NONE',  ( 0.6990986543038555379, 0.7150252244155714809, 2.907955489811387718E-17 ) ) ;
#37142=CARTESIAN_POINT ( 'NONE',  ( -14.11063322135152909, -21.03236308526469855, 72.21135587486895702 ) ) ;
#37143=CARTESIAN_POINT ( 'NONE',  ( -24.37121093718953446, -17.50201705633955740, 66.05701994492248730 ) ) ;
#37144=CARTESIAN_POINT ( 'NONE',  ( -14.69865306246719960, -8.361098061448752006, 64.07362231527311280 ) ) ;
#37145=EDGE_LOOP ( 'NONE', ( #15488, #17687, #32625, #24417, #11330 ) ) ;
#37148=CARTESIAN_POINT ( 'NONE',  ( -18.24929096724884658, -21.81104555038653103, 68.82986815895560540 ) ) ;
#37149=CYLINDRICAL_SURFACE ( 'NONE', #24488, 0.1500000000000020206 ) ;
#37150=ORIENTED_EDGE ( 'NONE', *, *, #48159, .T. ) ;
#37151=EDGE_LOOP ( 'NONE', ( #32668, #7032 ) ) ;
#37152=EDGE_CURVE ( 'NONE', #29452, #37416, #1249, .T. ) ;
#37153=CARTESIAN_POINT ( 'NONE',  ( -17.03030002819346933, -7.369452674228779365, 74.09984905828893886 ) ) ;
#37155=CARTESIAN_POINT ( 'NONE',  ( -15.71420658305500240, -7.965879067615756703, 74.37985862309683682 ) ) ;
#37156=CARTESIAN_POINT ( 'NONE',  ( -23.16117746674104438, -18.90708040007733359, 62.63934749780565880 ) ) ;
#37157=( BOUNDED_CURVE ( )  B_SPLINE_CURVE ( 3, ( #33025, #18007, #3251, #48067 ),
 .UNSPECIFIED., .F., .F. ) 
 B_SPLINE_CURVE_WITH_KNOTS ( ( 4, 4 ),
 ( 0.5000000000000000000, 0.9074455897393687298 ),
 .UNSPECIFIED. ) 
 CURVE ( )  GEOMETRIC_REPRESENTATION_ITEM ( )  RATIONAL_B_SPLINE_CURVE ( ( 0.9999999999999878986, 0.4567392136813231973, 0.3561768502900354294, 0.6983129098261112722 ) ) 
 REPRESENTATION_ITEM ( '' )  );
#37158=ORIENTED_EDGE ( 'NONE', *, *, #21050, .F. ) ;
#37159=CARTESIAN_POINT ( 'NONE',  ( -24.31126627854681743, -17.82450373576648417, 53.76227901944321275 ) ) ;
#37160=CARTESIAN_POINT ( 'NONE',  ( -13.88293547364789404, -20.90532801101632643, 68.75625136993008368 ) ) ;
#37162=LINE ( 'NONE', #44841, #38635 ) ;
#37165=LINE ( 'NONE', #45326, #28102 ) ;
#37167=ORIENTED_EDGE ( 'NONE', *, *, #7034, .T. ) ;
#37168=( BOUNDED_SURFACE ( )  B_SPLINE_SURFACE ( 3, 1, ( 
 ( #23698, #12828 ),
 ( #38932, #20710 ),
 ( #16984, #19982 ),
 ( #12346, #16259 ),
 ( #46334, #27366 ),
 ( #1027, #5458 ),
 ( #13055, #38691 ) ),
 .UNSPECIFIED., .T., .F., .F. ) 
 B_SPLINE_SURFACE_WITH_KNOTS ( ( 4, 3, 4 ),
 ( 2, 2 ),
 ( 0.000000000000000000, 0.5000000000000000000, 1.000000000000000000 ),
 ( 0.000000000000000000, 1.000000000000000000 ),
 .UNSPECIFIED. ) 
 GEOMETRIC_REPRESENTATION_ITEM ( )  RATIONAL_B_SPLINE_SURFACE ( (
 ( 1.000000000000000000, 1.000000000000000000),
 ( 0.3333333333333335369, 0.3333333333333330373),
 ( 0.3333333333333335369, 0.3333333333333330373),
 ( 1.000000000000000000, 1.000000000000000000),
 ( 0.3333333333333333703, 0.3333333333333333703),
 ( 0.3333333333333333703, 0.3333333333333333703),
 ( 1.000000000000000000, 1.000000000000000000) ) ) 
 REPRESENTATION_ITEM ( '' )  SURFACE ( )  );
#37169=CARTESIAN_POINT ( 'NONE',  ( -12.55411140858086760, -19.90724249994213935, 65.15202838036978505 ) ) ;
#37170=VERTEX_POINT ( 'NONE', #14706 ) ;
#37171=CARTESIAN_POINT ( 'NONE',  ( -10.45785868539726593, -17.45007275320745421, 64.82750577911360779 ) ) ;
#37172=CARTESIAN_POINT ( 'NONE',  ( -23.68653687815194786, -11.57061008776568123, 66.43686604568146947 ) ) ;
#37175=CYLINDRICAL_SURFACE ( 'NONE', #16338, 0.1500000000000063782 ) ;
#37176=CIRCLE ( 'NONE', #45076, 0.4000000000000006883 ) ;
#37179=CARTESIAN_POINT ( 'NONE',  ( -10.77693834736609979, -17.00378654741047413, 57.97295180822617056 ) ) ;
#37182=ORIENTED_EDGE ( 'NONE', *, *, #2469, .F. ) ;
#37183=CARTESIAN_POINT ( 'NONE',  ( -16.91157668238500733, -22.24167941632281753, 72.34355973887613800 ) ) ;
#37184=( BOUNDED_CURVE ( )  B_SPLINE_CURVE ( 3, ( #38214, #42904, #5484, #45648 ),
 .UNSPECIFIED., .F., .F. ) 
 B_SPLINE_CURVE_WITH_KNOTS ( ( 4, 4 ),
 ( 0.5000000000000000000, 0.9074455897393647330 ),
 .UNSPECIFIED. ) 
 CURVE ( )  GEOMETRIC_REPRESENTATION_ITEM ( )  RATIONAL_B_SPLINE_CURVE ( ( 1.000000000000008882, 0.4567392136813313019, 0.3561768502900237165, 0.6983129098260958401 ) ) 
 REPRESENTATION_ITEM ( '' )  );
#37185=CARTESIAN_POINT ( 'NONE',  ( -10.38752013045322009, -14.36951432065623635, 64.67331771650336236 ) ) ;
#37186=CARTESIAN_POINT ( 'NONE',  ( -22.93125612490430143, -9.791620008186384894, 70.17211892575356558 ) ) ;
#37187=CARTESIAN_POINT ( 'NONE',  ( -11.93195840498443516, -10.38844327383712773, 70.98365212470247343 ) ) ;
#37188=CARTESIAN_POINT ( 'NONE',  ( -10.78527694652531288, -12.58937498152797474, 61.09853578751868497 ) ) ;
#37189=CARTESIAN_POINT ( 'NONE',  ( -17.05117351117937474, -7.819147136050148994, 70.68139120385312424 ) ) ;
#37190=EDGE_CURVE ( 'NONE', #35176, #33854, #44701, .T. ) ;
#37191=ORIENTED_EDGE ( 'NONE', *, *, #30494, .T. ) ;
#37192=ORIENTED_EDGE ( 'NONE', *, *, #33591, .F. ) ;
#37193=CARTESIAN_POINT ( 'NONE',  ( -9.974576530078440584, -14.71985993733158793, 71.52056861311223201 ) ) ;
#37195=CARTESIAN_POINT ( 'NONE',  ( -19.26171524298325011, -21.61554300578126231, 58.82507358300556888 ) ) ;
#37196=CARTESIAN_POINT ( 'NONE',  ( -14.07466585761016198, -21.01278620474601411, 72.22607682806530249 ) ) ;
#37198=CARTESIAN_POINT ( 'NONE',  ( -12.28060247932822691, -9.983304365141403736, 64.44402973226354447 ) ) ;
#37199=CARTESIAN_POINT ( 'NONE',  ( -10.16748990304072464, -13.12235252378331651, 71.39323974795351546 ) ) ;
#37200=B_SPLINE_CURVE_WITH_KNOTS ( 'NONE', 3,
 ( #22826, #15391, #7319, #22319, #33370, #23067, #3602, #18605, #37821, #14901 ),
 .UNSPECIFIED., .F., .F.,
 ( 4, 2, 2, 2, 4 ),
 ( 0.000000000000000000, 0.2500000000000000000, 0.5000000000000000000, 0.7500000000000000000, 1.000000000000000000 ),
 .UNSPECIFIED. ) ;
#37201=FACE_BOUND ( 'NONE', #13170, .T. ) ;
#37202=CARTESIAN_POINT ( 'NONE',  ( -10.79646186035629540, -11.40653701787342200, 67.66218675276181216 ) ) ;
#37204=EDGE_CURVE ( 'NONE', #3868, #36187, #2420, .T. ) ;
#37205=ADVANCED_FACE ( 'NONE', ( #36895 ), #16126, .T. ) ;
#37206=CARTESIAN_POINT ( 'NONE',  ( -10.20197030601470090, -12.78660143320473352, 47.99999999999994316 ) ) ;
#37207=VERTEX_POINT ( 'NONE', #3178 ) ;
#37208=CARTESIAN_POINT ( 'NONE',  ( -14.04913797814320375, -8.615409903819811532, 70.93777579550457801 ) ) ;
#37209=CARTESIAN_POINT ( 'NONE',  ( -10.52668521080748398, -13.31230368787681506, 67.89399308012602319 ) ) ;
#37211=CARTESIAN_POINT ( 'NONE',  ( -17.31415506352089650, -21.86632207739205569, 72.32110344861041540 ) ) ;
#37212=EDGE_CURVE ( 'NONE', #1174, #45729, #41336, .T. ) ;
#37213=DIRECTION ( 'NONE',  ( -0.9584484254710481377, -0.2852658684667118139, 3.516456354099036190E-08 ) ) ;
#37214=CARTESIAN_POINT ( 'NONE',  ( -24.61605428079846547, -12.86511719609775284, 66.41751453275240635 ) ) ;
#37216=CARTESIAN_POINT ( 'NONE',  ( -18.18338144371267617, -21.81849904615365432, 65.63060065626805795 ) ) ;
#37217=ORIENTED_EDGE ( 'NONE', *, *, #38120, .T. ) ;
#37220=VERTEX_POINT ( 'NONE', #48475 ) ;
#37221=B_SPLINE_CURVE_WITH_KNOTS ( 'NONE', 3,
 ( #37722, #3272, #3505, #11387, #18026, #26410, #22473, #14323, #48568, #37466 ),
 .UNSPECIFIED., .F., .F.,
 ( 4, 2, 2, 2, 4 ),
 ( 0.1272669073657611005, 0.2522669073438869036, 0.3772669073220126235, 0.5022669073001384543, 0.6272669072782641742 ),
 .UNSPECIFIED. ) ;
#37222=ADVANCED_FACE ( 'NONE', ( #18673 ), #26320, .T. ) ;
#37223=CARTESIAN_POINT ( 'NONE',  ( -17.02395368709362344, -21.79788336522463155, 72.16543205089590174 ) ) ;
#37224=VECTOR ( 'NONE', #22070, 1000.000000000000000 ) ;
#37225=CARTESIAN_POINT ( 'NONE',  ( -11.68775437312510235, -10.05546324315060858, 67.54250946422081370 ) ) ;
#37226=B_SPLINE_CURVE_WITH_KNOTS ( 'NONE', 3,
 ( #6527, #9742, #39525, #9505, #47643, #40014, #32145, #28457, #5806, #13404 ),
 .UNSPECIFIED., .F., .F.,
 ( 4, 2, 2, 2, 4 ),
 ( 0.1272669073658128924, 0.2522669073463100209, 0.3772669073268071216, 0.5022669073073042778, 0.6272669072878014340 ),
 .UNSPECIFIED. ) ;
#37228=CARTESIAN_POINT ( 'NONE',  ( -16.09337608010665477, -22.13948405174236811, 58.40090292489767876 ) ) ;
#37229=ORIENTED_EDGE ( 'NONE', *, *, #38895, .F. ) ;
#37230=FACE_OUTER_BOUND ( 'NONE', #17257, .T. ) ;
#37231=CARTESIAN_POINT ( 'NONE',  ( -18.83586040784625126, -7.494106175837369044, 70.48572642001049360 ) ) ;
#37232=VERTEX_POINT ( 'NONE', #33680 ) ;
#37233=CARTESIAN_POINT ( 'NONE',  ( -23.82366785274684418, -10.99486113721019009, 73.47697904737684382 ) ) ;
#37236=LINE ( 'NONE', #18534, #46411 ) ;
#37239=CARTESIAN_POINT ( 'NONE',  ( -10.67250920137991521, -11.65805311173287961, 71.20205571017048385 ) ) ;
#37240=CARTESIAN_POINT ( 'NONE',  ( -23.01899735208242248, -19.09874304491667019, 59.18410621858622278 ) ) ;
#37242=CARTESIAN_POINT ( 'NONE',  ( -14.98563567286690379, -21.37212002227751029, 65.17766890071607122 ) ) ;
#37243=CARTESIAN_POINT ( 'NONE',  ( -21.65477688667505518, -9.232350752012335349, 66.66149992610201025 ) ) ;
#37244=ORIENTED_EDGE ( 'NONE', *, *, #31712, .T. ) ;
#37245=CARTESIAN_POINT ( 'NONE',  ( -11.79630000206883977, -19.05592701419838519, 71.97213747039440079 ) ) ;
#37247=CARTESIAN_POINT ( 'NONE',  ( -16.23116076413911557, -7.455249184188991407, 60.31533086125586607 ) ) ;
#37248=CARTESIAN_POINT ( 'NONE',  ( -10.39060893342343839, -14.27672657784476584, 67.94980160461363994 ) ) ;
#37249=VECTOR ( 'NONE', #27832, 1000.000000000000227 ) ;
#37251=EDGE_CURVE ( 'NONE', #38159, #31450, #34063, .T. ) ;
#37254=CARTESIAN_POINT ( 'NONE',  ( -24.25486363958986757, -13.06355980472538292, 63.11792038370487035 ) ) ;
#37255=CYLINDRICAL_SURFACE ( 'NONE', #37533, 0.1500000000000022704 ) ;
#37257=CARTESIAN_POINT ( 'NONE',  ( -11.29385027892729987, -19.04286830487734861, 68.33194243210506613 ) ) ;
#37258=CARTESIAN_POINT ( 'NONE',  ( -22.60138648290591235, -10.09559422629491898, 73.59234105511633572 ) ) ;
#37259=CARTESIAN_POINT ( 'NONE',  ( -10.57110035550071103, -13.38215360593666325, 74.97817647590578360 ) ) ;
#37262=FACE_OUTER_BOUND ( 'NONE', #42303, .T. ) ;
#37263=ORIENTED_EDGE ( 'NONE', *, *, #40257, .F. ) ;
#37269=CARTESIAN_POINT ( 'NONE',  ( -22.78678303852979425, -9.565966637465477262, 54.27966884056655061 ) ) ;
#37276=CARTESIAN_POINT ( 'NONE',  ( -10.02191625022346955, -15.65273779443635327, 61.15293638507743168 ) ) ;
#37277=DIRECTION ( 'NONE',  ( -0.9848822020395749943, 0.1732254256905498002, 7.367703375004543066E-08 ) ) ;
#37278=EDGE_CURVE ( 'NONE', #33406, #7220, #25265, .T. ) ;
#37280=AXIS2_PLACEMENT_3D ( 'NONE', #28686, #6286, #32621 ) ;
#37282=DIRECTION ( 'NONE',  ( -0.9959323210854038599, 0.09010444948746665350, 2.601165157765156148E-08 ) ) ;
#37285=CARTESIAN_POINT ( 'NONE',  ( -22.21713244587612834, -19.98430316242970406, 69.47417961646398510 ) ) ;
#37286=CARTESIAN_POINT ( 'NONE',  ( -11.71665266943325534, -18.96132379659194100, 64.90273906658698877 ) ) ;
#37289=ORIENTED_EDGE ( 'NONE', *, *, #32703, .T. ) ;
#37290=CARTESIAN_POINT ( 'NONE',  ( -13.54893327507986456, -8.910214905335239521, 64.05379690000981441 ) ) ;
#37292=DIRECTION ( 'NONE',  ( 0.8967515337576290602, -0.4425343904188011046, 9.546469656967254525E-09 ) ) ;
#37293=ORIENTED_EDGE ( 'NONE', *, *, #43461, .T. ) ;
#37294=CARTESIAN_POINT ( 'NONE',  ( -10.37840828709523322, -12.38598989307629061, 60.98508858522948373 ) ) ;
#37295=CARTESIAN_POINT ( 'NONE',  ( -22.78745088117329942, -19.98005169855493079, 72.83738836787418336 ) ) ;
#37296=ADVANCED_FACE ( 'NONE', ( #20088 ), #23799, .F. ) ;
#37298=CYLINDRICAL_SURFACE ( 'NONE', #5633, 0.1500000000000032419 ) ;
#37299=ORIENTED_EDGE ( 'NONE', *, *, #10485, .F. ) ;
#37300=CARTESIAN_POINT ( 'NONE',  ( -19.50174133129179666, -21.96376507711987003, 62.17316415538206087 ) ) ;
#37301=CARTESIAN_POINT ( 'NONE',  ( -17.17470792286161441, -7.363371476440942587, 70.59012221026488021 ) ) ;
#37302=CARTESIAN_POINT ( 'NONE',  ( -22.37985683132060188, -19.82347751554591397, 69.47417989525710880 ) ) ;
#37303=VERTEX_POINT ( 'NONE', #1614 ) ;
#37304=FACE_BOUND ( 'NONE', #1119, .T. ) ;
#37306=B_SPLINE_CURVE_WITH_KNOTS ( 'NONE', 3,
 ( #10772, #40329, #18391, #29251, #29737, #25075, #13720, #2422, #40096, #17433 ),
 .UNSPECIFIED., .F., .F.,
 ( 4, 2, 2, 2, 4 ),
 ( 0.000000000000000000, 0.2500000000000000000, 0.5000000000000000000, 0.7500000000000000000, 1.000000000000000000 ),
 .UNSPECIFIED. ) ;
#37308=DIRECTION ( 'NONE',  ( 6.516572649233546247E-06, -8.834921932032007089E-06, -0.9999999999397393147 ) ) ;
#37310=B_SPLINE_CURVE_WITH_KNOTS ( 'NONE', 3,
 ( #48059, #18742, #29587, #14297, #33753, #48293, #10637, #44618, #37193, #44381 ),
 .UNSPECIFIED., .F., .F.,
 ( 4, 2, 2, 2, 4 ),
 ( 0.1272669073657781147, 0.2522669073462887601, 0.3772669073267994611, 0.5022669073073100510, 0.6272669072878207519 ),
 .UNSPECIFIED. ) ;
#37311=CARTESIAN_POINT ( 'NONE',  ( -21.55884032038934350, -8.611816057827914150, 73.78624026056009200 ) ) ;
#37312=VERTEX_POINT ( 'NONE', #35093 ) ;
#37313=CARTESIAN_POINT ( 'NONE',  ( -10.45004451964941872, -15.89438299218807771, 71.59183561948579211 ) ) ;
#37314=ORIENTED_EDGE ( 'NONE', *, *, #18088, .T. ) ;
#37315=CARTESIAN_POINT ( 'NONE',  ( -10.70566809389435647, -16.94585225683366048, 57.68760548748760186 ) ) ;
#37316=CARTESIAN_POINT ( 'NONE',  ( -17.15134141312287852, -7.364115244199362920, 70.67531166753866501 ) ) ;
#37317=( BOUNDED_SURFACE ( )  B_SPLINE_SURFACE ( 3, 1, ( 
 ( #10346, #44557 ),
 ( #3669, #10813 ),
 ( #11068, #18428 ),
 ( #44326, #25833 ),
 ( #7136, #41339 ),
 ( #36648, #25588 ),
 ( #10579, #22153 ) ),
 .UNSPECIFIED., .T., .F., .F. ) 
 B_SPLINE_SURFACE_WITH_KNOTS ( ( 4, 3, 4 ),
 ( 2, 2 ),
 ( 0.000000000000000000, 0.5000000000000000000, 1.000000000000000000 ),
 ( 0.000000000000000000, 1.000000000000000000 ),
 .UNSPECIFIED. ) 
 GEOMETRIC_REPRESENTATION_ITEM ( )  RATIONAL_B_SPLINE_SURFACE ( (
 ( 1.000000000000000000, 1.000000000000000000),
 ( 0.3333333333333335369, 0.3333333333333330373),
 ( 0.3333333333333335369, 0.3333333333333330373),
 ( 1.000000000000000000, 1.000000000000000000),
 ( 0.3333333333333333703, 0.3333333333333333703),
 ( 0.3333333333333333703, 0.3333333333333333703),
 ( 1.000000000000000000, 1.000000000000000000) ) ) 
 REPRESENTATION_ITEM ( '' )  SURFACE ( )  );
#37320=CARTESIAN_POINT ( 'NONE',  ( -16.10088536661951153, -22.14081006509091054, 58.39311438780030983 ) ) ;
#37322=CARTESIAN_POINT ( 'NONE',  ( -18.31433346867779832, -22.20599535381256118, 68.95481354857830070 ) ) ;
#37325=ORIENTED_EDGE ( 'NONE', *, *, #9046, .T. ) ;
#37328=EDGE_CURVE ( 'NONE', #5083, #35202, #30607, .T. ) ;
#37329=CARTESIAN_POINT ( 'NONE',  ( -21.18844016355402715, -20.71102104569741087, 69.35450135975200681 ) ) ;
#37330=EDGE_CURVE ( 'NONE', #19106, #13753, #16626, .T. ) ;
#37331=CARTESIAN_POINT ( 'NONE',  ( -20.69652669518947263, -8.116311108972663391, 63.35475588450814399 ) ) ;
#37332=CARTESIAN_POINT ( 'NONE',  ( -10.39374096550114857, -17.27431698850577391, 61.35731899298346548 ) ) ;
#37333=FACE_OUTER_BOUND ( 'NONE', #37145, .T. ) ;
#37334=CARTESIAN_POINT ( 'NONE',  ( -14.81376595223554737, -21.78711290537215461, 61.77453959052536447 ) ) ;
#37335=( BOUNDED_CURVE ( )  B_SPLINE_CURVE ( 3, ( #8447, #45888, #27402, #39211 ),
 .UNSPECIFIED., .F., .F. ) 
 B_SPLINE_CURVE_WITH_KNOTS ( ( 4, 4 ),
 ( 0.4074455897393666204, 0.5000000000000000000 ),
 .UNSPECIFIED. ) 
 CURVE ( )  GEOMETRIC_REPRESENTATION_ITEM ( )  RATIONAL_B_SPLINE_CURVE ( ( 0.6983129098261150469, 0.7760317562607207398, 0.8765941196520169454, 1.000000000000005773 ) ) 
 REPRESENTATION_ITEM ( '' )  );
#37339=CARTESIAN_POINT ( 'NONE',  ( -16.05890242020153380, -7.889590739215661230, 60.08539615417584656 ) ) ;
#37340=CARTESIAN_POINT ( 'NONE',  ( -13.75230030363714206, -20.82772173381313863, 65.28069058648037526 ) ) ;
#37341=DIRECTION ( 'NONE',  ( -0.7847243476406478013, -0.6198448985189424221, 4.433022207822356401E-08 ) ) ;
#37344=VERTEX_POINT ( 'NONE', #28460 ) ;
#37346=ORIENTED_EDGE ( 'NONE', *, *, #33642, .F. ) ;
#37347=CARTESIAN_POINT ( 'NONE',  ( -22.17130234749883044, -20.55096496926394778, 58.87947491310501391 ) ) ;
#37348=CARTESIAN_POINT ( 'NONE',  ( -13.54792730259346456, -8.920061342218058797, 57.25495614889487683 ) ) ;
#37349=CARTESIAN_POINT ( 'NONE',  ( -15.15518219298508740, -21.43299249554696218, 68.68665981031909951 ) ) ;
#37350=B_SPLINE_CURVE_WITH_KNOTS ( 'NONE', 1,
 ( #2249, #13789 ),
 .UNSPECIFIED., .F., .F.,
 ( 2, 2 ),
 ( 0.000000000000000000, 1.000000000000000000 ),
 .UNSPECIFIED. ) ;
#37351=EDGE_CURVE ( 'NONE', #47871, #1499, #38800, .T. ) ;
#37352=ORIENTED_EDGE ( 'NONE', *, *, #6886, .F. ) ;
#37354=EDGE_CURVE ( 'NONE', #40867, #25757, #39394, .T. ) ;
#37355=CARTESIAN_POINT ( 'NONE',  ( -15.75283589881223278, -7.548994832054173543, 67.32502661251716347 ) ) ;
#37357=EDGE_LOOP ( 'NONE', ( #4970, #28987 ) ) ;
#37358=CARTESIAN_POINT ( 'NONE',  ( -17.19980212172655953, -7.762775302065857197, 70.79035839668001984 ) ) ;
#37360=CARTESIAN_POINT ( 'NONE',  ( -10.05862335131466700, -15.92885902279982524, 64.69266873560974318 ) ) ;
#37361=CARTESIAN_POINT ( 'NONE',  ( -19.17437844398820701, -7.979623566120205957, 63.44561363416070776 ) ) ;
#37362=ORIENTED_EDGE ( 'NONE', *, *, #38312, .F. ) ;
#37365=CARTESIAN_POINT ( 'NONE',  ( -10.20016939456313843, -12.98476690782802834, 71.39483965270750332 ) ) ;
#37366=LINE ( 'NONE', #7368, #43747 ) ;
#37367=ORIENTED_EDGE ( 'NONE', *, *, #16286, .T. ) ;
#37371=CARTESIAN_POINT ( 'NONE',  ( -11.25989573505624364, -11.38792594226331190, 64.14882039369129529 ) ) ;
#37374=ORIENTED_EDGE ( 'NONE', *, *, #31363, .F. ) ;
#37376=CARTESIAN_POINT ( 'NONE',  ( -24.34138173484706158, -16.17068648017255583, 62.59328676670276792 ) ) ;
#37379=CARTESIAN_POINT ( 'NONE',  ( -22.42594789675818845, -19.77792426076253918, 69.45945937764655298 ) ) ;
#37380=CARTESIAN_POINT ( 'NONE',  ( -11.93102524044397938, -10.47028995287008257, 71.26893105764186487 ) ) ;
#37381=CARTESIAN_POINT ( 'NONE',  ( -14.25068793291388225, -8.513811817964199946, 71.02957628655769895 ) ) ;
#37382=CARTESIAN_POINT ( 'NONE',  ( -24.64621740481133116, -16.83181165628401033, 53.49999999999994316 ) ) ;
#37384=CARTESIAN_POINT ( 'NONE',  ( -20.44655245503490448, -7.999037100505644204, 70.43755594487680582 ) ) ;
#37385=B_SPLINE_CURVE_WITH_KNOTS ( 'NONE', 1,
 ( #38217, #27159 ),
 .UNSPECIFIED., .F., .F.,
 ( 2, 2 ),
 ( 0.000000000000000000, 1.000000000000000000 ),
 .UNSPECIFIED. ) ;
#37386=CARTESIAN_POINT ( 'NONE',  ( -12.30133590797630738, -20.21947593564565793, 68.52312695590214275 ) ) ;
#37388=VECTOR ( 'NONE', #22275, 1000.000000000000114 ) ;
#37390=EDGE_CURVE ( 'NONE', #23075, #25499, #4415, .T. ) ;
#37391=CARTESIAN_POINT ( 'NONE',  ( -10.40245588357037043, -14.17414831712846990, 61.20349182037644198 ) ) ;
#37392=EDGE_CURVE ( 'NONE', #31125, #3060, #32392, .T. ) ;
#37394=CARTESIAN_POINT ( 'NONE',  ( -10.53147947836020215, -13.32716033773700381, 74.68377445404198056 ) ) ;
#37396=ORIENTED_EDGE ( 'NONE', *, *, #6056, .T. ) ;
#37398=CARTESIAN_POINT ( 'NONE',  ( -10.63166550887824791, -13.11538008670639321, 71.49212078082935307 ) ) ;
#37399=CARTESIAN_POINT ( 'NONE',  ( -23.34481533081060434, -18.63641918517796370, 69.44371984263474928 ) ) ;
#37401=EDGE_CURVE ( 'NONE', #16467, #4162, #46682, .T. ) ;
#37402=VERTEX_POINT ( 'NONE', #42749 ) ;
#37403=ADVANCED_FACE ( 'NONE', ( #9018 ), #37776, .T. ) ;
#37405=CARTESIAN_POINT ( 'NONE',  ( -14.22441598498101989, -8.081217260141077219, 67.44470407312981308 ) ) ;
#37408=EDGE_CURVE ( 'NONE', #36043, #26347, #35818, .T. ) ;
#37409=ORIENTED_EDGE ( 'NONE', *, *, #48211, .T. ) ;
#37410=DIRECTION ( 'NONE',  ( -5.731567514496413899E-31, -1.020425574103664789E-16, -1.000000000000000000 ) ) ;
#37411=CARTESIAN_POINT ( 'NONE',  ( -24.34278085428046268, -16.17909949234452682, 66.47813813521833026 ) ) ;
#37413=CARTESIAN_POINT ( 'NONE',  ( -12.65513433691805290, -20.00553804586020590, 64.75186297256590251 ) ) ;
#37415=AXIS2_PLACEMENT_3D ( 'NONE', #11813, #33700, #26837 ) ;
#37416=VERTEX_POINT ( 'NONE', #9977 ) ;
#37417=FACE_OUTER_BOUND ( 'NONE', #46487, .T. ) ;
#37419=ORIENTED_EDGE ( 'NONE', *, *, #24161, .F. ) ;
#37421=DIRECTION ( 'NONE',  ( -0.8447509909909737269, 0.5351595679979644915, -5.460905094113873772E-17 ) ) ;
#37424=CARTESIAN_POINT ( 'NONE',  ( -10.06071315540565791, -15.94306492381650564, 64.66804923369144831 ) ) ;
#37426=CARTESIAN_POINT ( 'NONE',  ( -25.93570572548787467, -11.53773867808332199, 54.49999999999995026 ) ) ;
#37427=ORIENTED_EDGE ( 'NONE', *, *, #45521, .T. ) ;
#37428=CARTESIAN_POINT ( 'NONE',  ( -10.43906464568624060, -14.34976906838038779, 64.38803843031173813 ) ) ;
#37430=CARTESIAN_POINT ( 'NONE',  ( -18.19036405266678713, -21.76720106350623851, 65.63066800548942581 ) ) ;
#37431=FACE_OUTER_BOUND ( 'NONE', #30394, .T. ) ;
#37435=VERTEX_POINT ( 'NONE', #14357 ) ;
#37436=VERTEX_POINT ( 'NONE', #3310 ) ;
#37437=CARTESIAN_POINT ( 'NONE',  ( -23.56005053104643210, -11.33143871826892912, 66.30725794404830253 ) ) ;
#37438=CARTESIAN_POINT ( 'NONE',  ( -14.86281067640541664, -8.294554978430625169, 56.92322698856733609 ) ) ;
#37440=B_SPLINE_CURVE_WITH_KNOTS ( 'NONE', 3,
 ( #12521, #724, #31483, #39106, #42814, #23628, #23371, #38365, #42588, #30775 ),
 .UNSPECIFIED., .F., .F.,
 ( 4, 2, 2, 2, 4 ),
 ( 0.000000000000000000, 0.2500000000000000000, 0.5000000000000000000, 0.7500000000000000000, 1.000000000000000000 ),
 .UNSPECIFIED. ) ;
#37442=CARTESIAN_POINT ( 'NONE',  ( -24.43827367352892210, -15.52193379869737200, 73.28831629023289906 ) ) ;
#37443=CARTESIAN_POINT ( 'NONE',  ( -15.28291166272248347, -21.52618791248891128, 68.87592918174580348 ) ) ;
#37444=CARTESIAN_POINT ( 'NONE',  ( -12.54283214832790350, -9.790123402769298266, 57.31765315075176659 ) ) ;
#37445=CARTESIAN_POINT ( 'NONE',  ( -12.41310947992116098, -19.76871611099698001, 61.68206578716802113 ) ) ;
#37446=CARTESIAN_POINT ( 'NONE',  ( -24.74075702715665770, -16.21285080831185965, 62.77823949964436423 ) ) ;
#37447=CARTESIAN_POINT ( 'NONE',  ( -23.01870635325979109, -6.403053727051749355, 54.54971261817296835 ) ) ;
#37450=CARTESIAN_POINT ( 'NONE',  ( -24.38600339462866629, -15.53964004551538203, 73.30303710393928895 ) ) ;
#37451=ORIENTED_EDGE ( 'NONE', *, *, #4177, .T. ) ;
#37452=CARTESIAN_POINT ( 'NONE',  ( -24.09244580564493177, -11.48710279877582785, 63.14492440366687021 ) ) ;
#37456=DIRECTION ( 'NONE',  ( 3.084459863448555673E-06, -5.853393718798201518E-06, 0.9999999999781119531 ) ) ;
#37457=( BOUNDED_CURVE ( )  B_SPLINE_CURVE ( 3, ( #3791, #18801, #107, #25954 ),
 .UNSPECIFIED., .F., .F. ) 
 B_SPLINE_CURVE_WITH_KNOTS ( ( 4, 4 ),
 ( 4.712388980384689674, 4.921828490624009511 ),
 .UNSPECIFIED. ) 
 CURVE ( )  GEOMETRIC_REPRESENTATION_ITEM ( )  RATIONAL_B_SPLINE_CURVE ( ( 1.000000000000000000, 0.9963479302455154896, 0.9963479302455154896, 1.000000000000000000 ) ) 
 REPRESENTATION_ITEM ( '' )  );
#37458=DIRECTION ( 'NONE',  ( -7.340779737911174687E-07, 8.195271841582110202E-07, -0.9999999999993947064 ) ) ;
#37459=CARTESIAN_POINT ( 'NONE',  ( -18.05440415122280484, -21.83127237841607027, 65.36004252941745563 ) ) ;
#37462=EDGE_LOOP ( 'NONE', ( #42654, #1935, #37082, #314, #11274 ) ) ;
#37465=ORIENTED_EDGE ( 'NONE', *, *, #37848, .T. ) ;
#37466=CARTESIAN_POINT ( 'NONE',  ( -23.58616520728616806, -18.99640775243969060, 66.00884813586510802 ) ) ;
#37468=AXIS2_PLACEMENT_3D ( 'NONE', #13436, #28484, #10254 ) ;
#37469=( BOUNDED_CURVE ( )  B_SPLINE_CURVE ( 3, ( #1254, #31791, #35228, #16514 ),
 .UNSPECIFIED., .F., .F. ) 
 B_SPLINE_CURVE_WITH_KNOTS ( ( 4, 4 ),
 ( 0.9074455897393680637, 1.000000000000000000 ),
 .UNSPECIFIED. ) 
 CURVE ( )  GEOMETRIC_REPRESENTATION_ITEM ( )  RATIONAL_B_SPLINE_CURVE ( ( 0.6983129098260993928, 0.7760317562607036423, 0.8765941196520038448, 1.000000000000000000 ) ) 
 REPRESENTATION_ITEM ( '' )  );
#37470=CARTESIAN_POINT ( 'NONE',  ( -13.34963310073524312, -8.571971970645527961, 57.09154962634697483 ) ) ;
#37471=EDGE_CURVE ( 'NONE', #39973, #18340, #7008, .T. ) ;
#37473=CARTESIAN_POINT ( 'NONE',  ( -17.84735332803204599, -7.371153730986438113, 60.19565454701680807 ) ) ;
#37475=CARTESIAN_POINT ( 'NONE',  ( -24.38143469521110518, -15.58083332675401067, 73.00303748421107741 ) ) ;
#37476=FACE_OUTER_BOUND ( 'NONE', #47898, .T. ) ;
#37477=EDGE_LOOP ( 'NONE', ( #22744, #7709 ) ) ;
#37478=CARTESIAN_POINT ( 'NONE',  ( -15.12355705037926334, -21.47721786961508528, 61.63600470926916586 ) ) ;
#37480=( BOUNDED_SURFACE ( )  B_SPLINE_SURFACE ( 3, 1, ( 
 ( #39388, #21588 ),
 ( #12556, #5671 ),
 ( #35673, #16954 ),
 ( #6569, #8876 ),
 ( #36566, #23897 ),
 ( #14158, #4943 ),
 ( #19951, #1222 ) ),
 .UNSPECIFIED., .T., .F., .F. ) 
 B_SPLINE_SURFACE_WITH_KNOTS ( ( 4, 3, 4 ),
 ( 2, 2 ),
 ( 0.000000000000000000, 0.5000000000000000000, 1.000000000000000000 ),
 ( 0.000000000000000000, 1.000000000000000000 ),
 .UNSPECIFIED. ) 
 GEOMETRIC_REPRESENTATION_ITEM ( )  RATIONAL_B_SPLINE_SURFACE ( (
 ( 1.000000000000000000, 1.000000000000000000),
 ( 0.3333333333333335369, 0.3333333333333330373),
 ( 0.3333333333333335369, 0.3333333333333330373),
 ( 1.000000000000000000, 1.000000000000000000),
 ( 0.3333333333333333703, 0.3333333333333333703),
 ( 0.3333333333333333703, 0.3333333333333333703),
 ( 1.000000000000000000, 1.000000000000000000) ) ) 
 REPRESENTATION_ITEM ( '' )  SURFACE ( )  );
#37484=CARTESIAN_POINT ( 'NONE',  ( -19.75048190521760461, -21.47275536819973141, 62.15070614013394135 ) ) ;
#37486=DIRECTION ( 'NONE',  ( -0.3739781583979218116, -0.9274375111247651349, -6.296758467538796555E-09 ) ) ;
#37487=ORIENTED_EDGE ( 'NONE', *, *, #34901, .F. ) ;
#37488=CARTESIAN_POINT ( 'NONE',  ( -12.76273281506171919, -20.09846992828358125, 71.81213450582208679 ) ) ;
#37489=CYLINDRICAL_SURFACE ( 'NONE', #14700, 0.1500000000000072387 ) ;
#37490=CARTESIAN_POINT ( 'NONE',  ( -15.03805467426947828, -21.39046384358795194, 65.12213282899359967 ) ) ;
#37491=CARTESIAN_POINT ( 'NONE',  ( -23.91439695282944200, -17.43141281116713515, 66.24357239631997629 ) ) ;
#37492=ORIENTED_EDGE ( 'NONE', *, *, #18327, .F. ) ;
#37493=CARTESIAN_POINT ( 'NONE',  ( -10.61641629527463770, -11.78277212779517136, 74.74335553404092991 ) ) ;
#37494=FACE_OUTER_BOUND ( 'NONE', #30524, .T. ) ;
#37495=CARTESIAN_POINT ( 'NONE',  ( -15.34011606297474195, -21.49348192942642655, 72.15648571357043295 ) ) ;
#37498=CARTESIAN_POINT ( 'NONE',  ( -11.07857854458970692, -11.73724703412850801, 71.08860870961423473 ) ) ;
#37502=CARTESIAN_POINT ( 'NONE',  ( -13.51659408464697698, -24.65568926594394128, 53.49999999999995026 ) ) ;
#37503=FACE_OUTER_BOUND ( 'NONE', #5123, .T. ) ;
#37504=ORIENTED_EDGE ( 'NONE', *, *, #3192, .T. ) ;
#37507=CARTESIAN_POINT ( 'NONE',  ( -11.73260704738458671, -10.00184175524024610, 67.61401452035728710 ) ) ;
#37508=ORIENTED_EDGE ( 'NONE', *, *, #44753, .F. ) ;
#37510=DIRECTION ( 'NONE',  ( -0.3478314405900341799, -0.9375570856950852239, 0.000000000000000000 ) ) ;
#37513=CARTESIAN_POINT ( 'NONE',  ( -12.84086788549150704, -8.935670915691353855, 67.55659650341593192 ) ) ;
#37514=CARTESIAN_POINT ( 'NONE',  ( -10.89849601230814713, -17.47747223720621434, 68.09721941041966886 ) ) ;
#37515=CARTESIAN_POINT ( 'NONE',  ( -16.13432406759100601, -21.74052631579560568, 58.30057715624173653 ) ) ;
#37516=B_SPLINE_CURVE_WITH_KNOTS ( 'NONE', 1,
 ( #22663, #30309 ),
 .UNSPECIFIED., .F., .F.,
 ( 2, 2 ),
 ( 0.000000000000000000, 1.000000000000000000 ),
 .UNSPECIFIED. ) ;
#37517=CARTESIAN_POINT ( 'NONE',  ( -10.78898398081525301, -17.19290454168847404, 61.44271037915215317 ) ) ;
#37518=EDGE_LOOP ( 'NONE', ( #1477, #3358 ) ) ;
#37519=ORIENTED_EDGE ( 'NONE', *, *, #22841, .T. ) ;
#37521=CARTESIAN_POINT ( 'NONE',  ( -10.45863951484398946, -14.11462368554138536, 60.91821294131582931 ) ) ;
#37527=EDGE_CURVE ( 'NONE', #3166, #21687, #17048, .T. ) ;
#37528=CARTESIAN_POINT ( 'NONE',  ( -18.72680909822608797, -7.880611277284092608, 70.52068030200462090 ) ) ;
#37529=CARTESIAN_POINT ( 'NONE',  ( -14.01837044221388595, -8.636059239884618322, 74.48482605064899076 ) ) ;
#37531=ORIENTED_EDGE ( 'NONE', *, *, #27878, .T. ) ;
#37532=FACE_OUTER_BOUND ( 'NONE', #17067, .T. ) ;
#37533=AXIS2_PLACEMENT_3D ( 'NONE', #7261, #11189, #22767 ) ;
#37534=ORIENTED_EDGE ( 'NONE', *, *, #47511, .F. ) ;
#37535=EDGE_CURVE ( 'NONE', #20491, #21857, #46473, .T. ) ;
#37536=DIRECTION ( 'NONE',  ( 5.297746385098606630E-06, 8.914243324979344743E-06, 0.9999999999462350075 ) ) ;
#37537=CARTESIAN_POINT ( 'NONE',  ( -18.22959580818018566, -21.76314769987743603, 68.83131364167647348 ) ) ;
#37539=LINE ( 'NONE', #29688, #34850 ) ;
#37541=ORIENTED_EDGE ( 'NONE', *, *, #18126, .T. ) ;
#37542=CARTESIAN_POINT ( 'NONE',  ( -17.98657259272421172, -21.83703102787368167, 62.16063850355641307 ) ) ;
#37543=CARTESIAN_POINT ( 'NONE',  ( -15.37055318500739354, -21.97060318045666705, 72.24564236423489660 ) ) ;
#37545=CARTESIAN_POINT ( 'NONE',  ( -10.98557804775572144, -17.68114217416224321, 71.71718193507115302 ) ) ;
#37546=CARTESIAN_POINT ( 'NONE',  ( -19.86401518824997581, -21.42384811948916479, 69.22010401872219632 ) ) ;
#37548=DIRECTION ( 'NONE',  ( -5.731567514496413899E-31, -1.020425574103664789E-16, -1.000000000000000000 ) ) ;
#37549=CARTESIAN_POINT ( 'NONE',  ( -17.21518928061367859, -7.362082935544761675, 70.59761670184047944 ) ) ;
#37550=CARTESIAN_POINT ( 'NONE',  ( -18.76558392140857023, -7.480892851696864021, 70.55563303198719893 ) ) ;
#37551=FACE_BOUND ( 'NONE', #23762, .T. ) ;
#37552=EDGE_LOOP ( 'NONE', ( #45994, #36015, #39801, #44549, #3969 ) ) ;
#37553=LINE ( 'NONE', #11723, #6168 ) ;
#37554=CARTESIAN_POINT ( 'NONE',  ( -10.55840381512346049, -16.17443265670291197, 71.44750434600322819 ) ) ;
#37555=CARTESIAN_POINT ( 'NONE',  ( -16.97945985512182787, -21.84517132341290591, 72.16543221430227106 ) ) ;
#37556=VECTOR ( 'NONE', #37486, 1000.000000000000114 ) ;
#37557=CARTESIAN_POINT ( 'NONE',  ( -24.85076376908920537, -14.22007681150577518, 69.80275272707126533 ) ) ;
#37558=VERTEX_POINT ( 'NONE', #10946 ) ;
#37559=CARTESIAN_POINT ( 'NONE',  ( -10.50429924535250414, -16.15944446069507023, 71.46222527016213633 ) ) ;
#37560=ORIENTED_EDGE ( 'NONE', *, *, #4620, .F. ) ;
#37561=CARTESIAN_POINT ( 'NONE',  ( -12.67941281020567068, -9.065306902972979586, 71.02642229240572647 ) ) ;
#37564=ORIENTED_EDGE ( 'NONE', *, *, #46898, .T. ) ;
#37565=CARTESIAN_POINT ( 'NONE',  ( -10.78978130820344994, -12.42417047965500565, 57.62857332104950103 ) ) ;
#37567=VECTOR ( 'NONE', #40179, 1000.000000000000227 ) ;
#37568=CARTESIAN_POINT ( 'NONE',  ( -18.39194801826630510, -22.19612395633120627, 69.00788843400852102 ) ) ;
#37570=EDGE_LOOP ( 'NONE', ( #34860, #27958, #19027, #17261, #14033 ) ) ;
#37572=CARTESIAN_POINT ( 'NONE',  ( -15.27269024242438533, -21.52607325516635939, 72.46064223565690554 ) ) ;
#37573=CARTESIAN_POINT ( 'NONE',  ( -18.05440415122280839, -21.83127237841607027, 65.36004252941745563 ) ) ;
#37574=VECTOR ( 'NONE', #5246, 1000.000000000000000 ) ;
#37575=CARTESIAN_POINT ( 'NONE',  ( -21.95523322170430092, -8.895446802377390938, 66.77654591769551473 ) ) ;
#37576=CARTESIAN_POINT ( 'NONE',  ( -20.73422126667899690, -8.581213913796407411, 63.72610227039507436 ) ) ;
#37577=CARTESIAN_POINT ( 'NONE',  ( -21.76912952166680881, -20.36565426623231190, 58.85623051144766293 ) ) ;
#37578=CYLINDRICAL_SURFACE ( 'NONE', #26305, 0.1500000000000050737 ) ;
#37579=CARTESIAN_POINT ( 'NONE',  ( -23.46260370332432288, -11.17067683354235719, 73.66193301755811262 ) ) ;
#37580=VECTOR ( 'NONE', #16922, 1000.000000000000000 ) ;
#37582=ORIENTED_EDGE ( 'NONE', *, *, #43862, .F. ) ;
#37583=CARTESIAN_POINT ( 'NONE',  ( -17.49728986656368335, -7.358816873484950172, 63.66401766577892118 ) ) ;
#37585=CARTESIAN_POINT ( 'NONE',  ( -14.84927081153347039, -21.37251255130113137, 61.65072491673618771 ) ) ;
#37586=LINE ( 'NONE', #18631, #18947 ) ;
#37588=ADVANCED_FACE ( 'NONE', ( #10471 ), #40984, .T. ) ;
#37590=B_SPLINE_CURVE_WITH_KNOTS ( 'NONE', 3,
 ( #33949, #23364, #27297, #42323, #46258, #8591, #243, #15221, #38619, #41591 ),
 .UNSPECIFIED., .F., .F.,
 ( 4, 2, 2, 2, 4 ),
 ( 0.000000000000000000, 0.2500000000000000000, 0.5000000000000000000, 0.7500000000000000000, 1.000000000000000000 ),
 .UNSPECIFIED. ) ;
#37591=ORIENTED_EDGE ( 'NONE', *, *, #31976, .F. ) ;
#37593=CARTESIAN_POINT ( 'NONE',  ( -12.18836193727821460, -19.53083876418623532, 57.94154444592973618 ) ) ;
#37594=AXIS2_PLACEMENT_3D ( 'NONE', #1343, #31397, #26979 ) ;
#37595=CARTESIAN_POINT ( 'NONE',  ( -10.45740709548926262, -13.70915569549963031, 57.86313879094461754 ) ) ;
#37596=AXIS2_PLACEMENT_3D ( 'NONE', #24470, #36248, #43425 ) ;
#37597=ORIENTED_EDGE ( 'NONE', *, *, #39048, .T. ) ;
#37600=VECTOR ( 'NONE', #4110, 1000.000000000000227 ) ;
#37601=CARTESIAN_POINT ( 'NONE',  ( -10.38752013045322009, -14.36951432065623813, 64.67331771650336236 ) ) ;
#37602=CARTESIAN_POINT ( 'NONE',  ( -21.65477468606848532, -9.232349032746775208, 66.96149992608901869 ) ) ;
#37603=EDGE_CURVE ( 'NONE', #42912, #33146, #23271, .T. ) ;
#37605=CARTESIAN_POINT ( 'NONE',  ( -24.26499789074519597, -17.75976756996305639, 62.65856417960095825 ) ) ;
#37606=EDGE_CURVE ( 'NONE', #46221, #46252, #13883, .T. ) ;
#37607=( BOUNDED_SURFACE ( )  B_SPLINE_SURFACE ( 3, 1, ( 
 ( #29334, #15019 ),
 ( #44366, #3719 ),
 ( #30082, #6924 ),
 ( #33240, #21944 ),
 ( #3228, #11352 ),
 ( #48280, #29573 ),
 ( #10859, #14759 ) ),
 .UNSPECIFIED., .T., .F., .F. ) 
 B_SPLINE_SURFACE_WITH_KNOTS ( ( 4, 3, 4 ),
 ( 2, 2 ),
 ( 0.000000000000000000, 0.5000000000000000000, 1.000000000000000000 ),
 ( 0.000000000000000000, 1.000000000000000000 ),
 .UNSPECIFIED. ) 
 GEOMETRIC_REPRESENTATION_ITEM ( )  RATIONAL_B_SPLINE_SURFACE ( (
 ( 1.000000000000000000, 1.000000000000000000),
 ( 0.3333333333333335369, 0.3333333333333330373),
 ( 0.3333333333333335369, 0.3333333333333330373),
 ( 1.000000000000000000, 1.000000000000000000),
 ( 0.3333333333333333703, 0.3333333333333333703),
 ( 0.3333333333333333703, 0.3333333333333333703),
 ( 1.000000000000000000, 1.000000000000000000) ) ) 
 REPRESENTATION_ITEM ( '' )  SURFACE ( )  );
#37609=LINE ( 'NONE', #47793, #14227 ) ;
#37610=VERTEX_POINT ( 'NONE', #33826 ) ;
#37611=CARTESIAN_POINT ( 'NONE',  ( -11.14069362286655718, -11.72368817214407599, 71.08860884459858198 ) ) ;
#37612=ORIENTED_EDGE ( 'NONE', *, *, #37911, .T. ) ;
#37613=CARTESIAN_POINT ( 'NONE',  ( -10.32134938064561247, -17.05723401094961034, 57.88771750990810006 ) ) ;
#37614=CARTESIAN_POINT ( 'NONE',  ( -11.49187621880558119, -18.52825149122186943, 64.93634258412723170 ) ) ;
#37616=VERTEX_POINT ( 'NONE', #30650 ) ;
#37617=CARTESIAN_POINT ( 'NONE',  ( -12.85387012802420514, -9.430729208696401855, 67.53509681483876648 ) ) ;
#37619=LINE ( 'NONE', #33190, #47778 ) ;
#37620=ORIENTED_EDGE ( 'NONE', *, *, #18837, .T. ) ;
#37622=ADVANCED_FACE ( 'NONE', ( #45185 ), #45672, .F. ) ;
#37623=CARTESIAN_POINT ( 'NONE',  ( -19.61601503992405071, -21.50980213996393786, 65.76486213821364402 ) ) ;
#37624=CARTESIAN_POINT ( 'NONE',  ( -12.00971705810820467, -9.691755786776280246, 60.67422651510300113 ) ) ;
#37626=DIRECTION ( 'NONE',  ( -3.289814948237356682E-07, -7.277561423860909391E-07, 0.9999999999996810329 ) ) ;
#37627=( BOUNDED_CURVE ( )  B_SPLINE_CURVE ( 3, ( #1812, #8970, #42935, #1567 ),
 .UNSPECIFIED., .F., .F. ) 
 B_SPLINE_CURVE_WITH_KNOTS ( ( 4, 4 ),
 ( 0.4074455897393643999, 0.5000000000000000000 ),
 .UNSPECIFIED. ) 
 CURVE ( )  GEOMETRIC_REPRESENTATION_ITEM ( )  RATIONAL_B_SPLINE_CURVE ( ( 0.6983129098260837386, 0.7760317562606962039, 0.8765941196520034007, 1.000000000000009548 ) ) 
 REPRESENTATION_ITEM ( '' )  );
#37628=CARTESIAN_POINT ( 'NONE',  ( -21.73719165441269396, -8.734630208819112340, 70.32406670146895067 ) ) ;
#37630=ORIENTED_EDGE ( 'NONE', *, *, #46108, .T. ) ;
#37631=ORIENTED_EDGE ( 'NONE', *, *, #12010, .F. ) ;
#37633=CARTESIAN_POINT ( 'NONE',  ( -10.73080526501584941, -11.53763522125388086, 71.19586713194442495 ) ) ;
#37635=CARTESIAN_POINT ( 'NONE',  ( -23.50857174774670355, -19.10953103619692328, 62.46751498843644157 ) ) ;
#37636=B_SPLINE_CURVE_WITH_KNOTS ( 'NONE', 3,
 ( #41645, #48288, #523, #30579, #25891, #37189, #22202, #18485, #33491, #26143 ),
 .UNSPECIFIED., .F., .F.,
 ( 4, 2, 2, 2, 4 ),
 ( 0.000000000000000000, 0.2500000000000000000, 0.5000000000000000000, 0.7500000000000000000, 1.000000000000000000 ),
 .UNSPECIFIED. ) ;
#37639=CARTESIAN_POINT ( 'NONE',  ( -12.50924672071177923, -19.79360999578536351, 61.50564738844418144 ) ) ;
#37640=COLOUR_RGB ( '', 0.66274510, 0.83137255, 0.94901961) ;
#37641=CARTESIAN_POINT ( 'NONE',  ( -12.10369268100898132, -9.594121713099781346, 57.27430968559156810 ) ) ;
#37642=CARTESIAN_POINT ( 'NONE',  ( -24.34502386579654498, -17.56683345968398768, 66.12852568699506151 ) ) ;
#37644=CARTESIAN_POINT ( 'NONE',  ( -16.52978676676487169, -22.20534210804297715, 65.42575595334410821 ) ) ;
#37646=CARTESIAN_POINT ( 'NONE',  ( -11.49688049385020960, -18.62690763749001732, 64.76179218520603342 ) ) ;
#37651=EDGE_CURVE ( 'NONE', #30489, #27713, #28300, .T. ) ;
#37654=CARTESIAN_POINT ( 'NONE',  ( -21.61813339613238227, -8.651787399021619862, 73.71633365192373333 ) ) ;
#37655=CARTESIAN_POINT ( 'NONE',  ( -9.974654501588993583, -14.90060059298426864, 74.94778899347312517 ) ) ;
#37656=CARTESIAN_POINT ( 'NONE',  ( -13.28665195206506766, -21.00489563950134553, 61.67792873707563928 ) ) ;
#37657=CARTESIAN_POINT ( 'NONE',  ( -13.83862390296875056, -21.33972285065757291, 72.11946018631711297 ) ) ;
#37659=ADVANCED_FACE ( 'NONE', ( #38005 ), #8237, .T. ) ;
#37660=CYLINDRICAL_SURFACE ( 'NONE', #8559, 0.1499999999999993838 ) ;
#37661=CARTESIAN_POINT ( 'NONE',  ( -24.43113031232903865, -15.58634216689856800, 73.30303748141028564 ) ) ;
#37662=ORIENTED_EDGE ( 'NONE', *, *, #44136, .T. ) ;
#37666=ORIENTED_EDGE ( 'NONE', *, *, #43293, .T. ) ;
#37667=CARTESIAN_POINT ( 'NONE',  ( -24.77723877343947478, -16.00713684962007122, 66.24820200538215431 ) ) ;
#37668=VERTEX_POINT ( 'NONE', #34068 ) ;
#37671=EDGE_LOOP ( 'NONE', ( #10154, #28205, #35935, #48583, #11926 ) ) ;
#37672=CARTESIAN_POINT ( 'NONE',  ( -11.19819527566065887, -18.90074491542570456, 64.89707073357136835 ) ) ;
#37673=B_SPLINE_CURVE_WITH_KNOTS ( 'NONE', 3,
 ( #470, #11303, #37881, #26562, #18669, #12265, #14962, #42315, #34415, #42071 ),
 .UNSPECIFIED., .F., .F.,
 ( 4, 2, 2, 2, 4 ),
 ( 0.000000000000000000, 0.2500000000000000000, 0.5000000000000000000, 0.7500000000000000000, 1.000000000000000000 ),
 .UNSPECIFIED. ) ;
#37674=EDGE_CURVE ( 'NONE', #22263, #27202, #43410, .T. ) ;
#37675=CARTESIAN_POINT ( 'NONE',  ( -11.14029015952437263, -10.80702246001832023, 57.46549161190092292 ) ) ;
#37677=CARTESIAN_POINT ( 'NONE',  ( -13.32057209662121267, -9.066726955530414855, 57.12534593251891124 ) ) ;
#37678=CARTESIAN_POINT ( 'NONE',  ( -10.39679176622870038, -14.24023819782134481, 64.40275955115841100 ) ) ;
#37681=AXIS2_PLACEMENT_3D ( 'NONE', #22261, #18807, #6999 ) ;
#37682=EDGE_CURVE ( 'NONE', #24279, #18615, #9757, .T. ) ;
#37683=DIRECTION ( 'NONE',  ( 0.9118114225829225816, 0.4106092176842893182, 5.589476759239149737E-08 ) ) ;
#37684=CARTESIAN_POINT ( 'NONE',  ( -22.23024899390505027, -9.116745682064513190, 59.82832910242247237 ) ) ;
#37685=CARTESIAN_POINT ( 'NONE',  ( -13.42146604834728763, -8.525632923396102569, 57.14780542301615185 ) ) ;
#37687=LINE ( 'NONE', #4221, #8197 ) ;
#37688=DIRECTION ( 'NONE',  ( -0.9441784275685841665, 0.3294345108122634369, 1.993146885055994800E-08 ) ) ;
#37689=FACE_OUTER_BOUND ( 'NONE', #47482, .T. ) ;
#37690=CARTESIAN_POINT ( 'NONE',  ( -22.39476240126155560, -20.35875292466404574, 62.39472529595067840 ) ) ;
#37691=CARTESIAN_POINT ( 'NONE',  ( -24.18834572025230401, -13.00761457142965938, 62.90552128796598907 ) ) ;
#37694=FACE_OUTER_BOUND ( 'NONE', #872, .T. ) ;
#37695=CARTESIAN_POINT ( 'NONE',  ( -22.91296630721855365, -15.15889098507617128, 53.49999999999995026 ) ) ;
#37697=CARTESIAN_POINT ( 'NONE',  ( -21.01131272606871292, -21.33876233430101621, 62.30809711058548572 ) ) ;
#37698=CARTESIAN_POINT ( 'NONE',  ( -16.38232541403072773, -22.18617787627378846, 61.89421581153325747 ) ) ;
#37700=CARTESIAN_POINT ( 'NONE',  ( -17.27965118537360212, -7.810258991196201706, 70.77419234192039710 ) ) ;
#37701=ADVANCED_FACE ( 'NONE', ( #33564 ), #14439, .T. ) ;
#37702=LINE ( 'NONE', #34747, #14074 ) ;
#37703=CARTESIAN_POINT ( 'NONE',  ( -19.52948875563194875, -21.95553444029042467, 62.09529400939659638 ) ) ;
#37704=EDGE_CURVE ( 'NONE', #27713, #29708, #11035, .T. ) ;
#37706=CARTESIAN_POINT ( 'NONE',  ( -16.43317471172368016, -9.385549587026176255, 53.88362224778186516 ) ) ;
#37708=ADVANCED_FACE ( 'NONE', ( #30890 ), #38495, .F. ) ;
#37712=CARTESIAN_POINT ( 'NONE',  ( -12.05615918852498680, -19.97535170061420828, 61.51183199568394144 ) ) ;
#37713=( BOUNDED_CURVE ( )  B_SPLINE_CURVE ( 3, ( #16925, #36594, #25782, #47951 ),
 .UNSPECIFIED., .F., .F. ) 
 B_SPLINE_CURVE_WITH_KNOTS ( ( 4, 4 ),
 ( 0.9074455897393651771, 1.000000000000000000 ),
 .UNSPECIFIED. ) 
 CURVE ( )  GEOMETRIC_REPRESENTATION_ITEM ( )  RATIONAL_B_SPLINE_CURVE ( ( 0.6983129098260764112, 0.7760317562606838804, 0.8765941196519917433, 1.000000000000000000 ) ) 
 REPRESENTATION_ITEM ( '' )  );
#37715=CARTESIAN_POINT ( 'NONE',  ( -13.01353307917097268, -8.804980454159759162, 64.09441913135431435 ) ) ;
#37718=ORIENTED_EDGE ( 'NONE', *, *, #4183, .F. ) ;
#37719=ORIENTED_EDGE ( 'NONE', *, *, #44562, .T. ) ;
#37721=ORIENTED_EDGE ( 'NONE', *, *, #29601, .T. ) ;
#37722=CARTESIAN_POINT ( 'NONE',  ( -23.54569140518488624, -19.05536029250058050, 65.93894040291287695 ) ) ;
#37723=CARTESIAN_POINT ( 'NONE',  ( -16.39887994223181167, -21.73372354711506560, 61.75568132718285597 ) ) ;
#37725=DIRECTION ( 'NONE',  ( -0.5420872618288282707, -0.8403222004463035688, 7.592316861452269267E-08 ) ) ;
#37727=ORIENTED_EDGE ( 'NONE', *, *, #27008, .F. ) ;
#37728=DIRECTION ( 'NONE',  ( -0.9132646967824438189, 0.4073666574609055568, -8.344532079829881716E-09 ) ) ;
#37729=CARTESIAN_POINT ( 'NONE',  ( -17.63103806674120833, -7.362028203752553068, 63.65782862784570284 ) ) ;
#37734=CARTESIAN_POINT ( 'NONE',  ( -23.46741908093438767, -19.16603997859080266, 62.53902161361033052 ) ) ;
#37735=CARTESIAN_POINT ( 'NONE',  ( -21.42336286209559759, -21.09487474236010485, 69.23945462178221533 ) ) ;
#37736=EDGE_CURVE ( 'NONE', #13753, #14422, #11141, .T. ) ;
#37737=CARTESIAN_POINT ( 'NONE',  ( -17.23043714677651295, -7.361597588792181845, 70.61318921025367956 ) ) ;
#37738=ORIENTED_EDGE ( 'NONE', *, *, #20604, .F. ) ;
#37739=CARTESIAN_POINT ( 'NONE',  ( -10.73142062415649711, -12.58174813459350538, 64.36016235006516695 ) ) ;
#37741=AXIS2_PLACEMENT_3D ( 'NONE', #19707, #9357, #23655 ) ;
#37743=CARTESIAN_POINT ( 'NONE',  ( -24.24394117090890788, -12.99133827687660059, 59.51834745271546723 ) ) ;
#37745=EDGE_LOOP ( 'NONE', ( #19722, #14043, #41782, #19370, #42670 ) ) ;
#37746=CARTESIAN_POINT ( 'NONE',  ( -24.69852180232685157, -16.41745880042978101, 59.30827708941524889 ) ) ;
#37748=VECTOR ( 'NONE', #22333, 1000.000000000000227 ) ;
#37750=PLANE ( 'NONE',  #47045 ) ;
#37751=CARTESIAN_POINT ( 'NONE',  ( -20.93476986463577916, -20.86527884399460220, 62.34144714227700490 ) ) ;
#37752=CARTESIAN_POINT ( 'NONE',  ( -21.20554785340111081, -20.76353671134526380, 65.79273731141989856 ) ) ;
#37755=CARTESIAN_POINT ( 'NONE',  ( -24.65061889199765233, -12.99785316138012270, 62.87618224063605510 ) ) ;
#37756=FACE_OUTER_BOUND ( 'NONE', #1456, .T. ) ;
#37760=CARTESIAN_POINT ( 'NONE',  ( -24.44055745662519641, -14.11932379769929113, 73.13743607903229815 ) ) ;
#37761=CARTESIAN_POINT ( 'NONE',  ( -18.03441950114640235, -20.28875745248266327, 53.69233794759168887 ) ) ;
#37762=( BOUNDED_CURVE ( )  B_SPLINE_CURVE ( 3, ( #6138, #25338, #14221, #43578 ),
 .UNSPECIFIED., .F., .F. ) 
 B_SPLINE_CURVE_WITH_KNOTS ( ( 4, 4 ),
 ( 0.4074455897393596815, 0.5000000000000000000 ),
 .UNSPECIFIED. ) 
 CURVE ( )  GEOMETRIC_REPRESENTATION_ITEM ( )  RATIONAL_B_SPLINE_CURVE ( ( 0.6983129098260858481, 0.7760317562606769970, 0.8765941196519771994, 0.9999999999999761302 ) ) 
 REPRESENTATION_ITEM ( '' )  );
#37764=CARTESIAN_POINT ( 'NONE',  ( -18.64625997845222116, -21.76055708611507100, 68.97081679896227513 ) ) ;
#37766=CARTESIAN_POINT ( 'NONE',  ( -10.40035142239662669, -15.50347837920617167, 64.65204674534754758 ) ) ;
#37767=CARTESIAN_POINT ( 'NONE',  ( -23.48338609245114483, -18.31419979820022448, 72.87254147078147071 ) ) ;
#37769=EDGE_CURVE ( 'NONE', #42856, #25718, #31111, .T. ) ;
#37772=CARTESIAN_POINT ( 'NONE',  ( -14.39270380832417295, -8.498217223279159072, 70.80127861885151219 ) ) ;
#37773=CARTESIAN_POINT ( 'NONE',  ( -13.27770617114843965, -9.107455183738579763, 64.05946529205222362 ) ) ;
#37774=CARTESIAN_POINT ( 'NONE',  ( -24.85414368999009938, -14.26268454367973781, 69.83088022027575903 ) ) ;
#37775=CARTESIAN_POINT ( 'NONE',  ( -16.97945985512182787, -21.84517132341290591, 72.16543221430227106 ) ) ;
#37776=( BOUNDED_SURFACE ( )  B_SPLINE_SURFACE ( 3, 1, ( 
 ( #20336, #24278 ),
 ( #42983, #9255 ),
 ( #39288, #35345 ),
 ( #2097, #5571 ),
 ( #6035, #20586 ),
 ( #35583, #13407 ),
 ( #43483, #12451 ) ),
 .UNSPECIFIED., .T., .F., .F. ) 
 B_SPLINE_SURFACE_WITH_KNOTS ( ( 4, 3, 4 ),
 ( 2, 2 ),
 ( 0.000000000000000000, 0.5000000000000000000, 1.000000000000000000 ),
 ( 0.000000000000000000, 1.000000000000000000 ),
 .UNSPECIFIED. ) 
 GEOMETRIC_REPRESENTATION_ITEM ( )  RATIONAL_B_SPLINE_SURFACE ( (
 ( 1.000000000000000000, 1.000000000000000000),
 ( 0.3333333333333335369, 0.3333333333333330373),
 ( 0.3333333333333335369, 0.3333333333333330373),
 ( 1.000000000000000000, 1.000000000000000000),
 ( 0.3333333333333333703, 0.3333333333333333703),
 ( 0.3333333333333333703, 0.3333333333333333703),
 ( 1.000000000000000000, 1.000000000000000000) ) ) 
 REPRESENTATION_ITEM ( '' )  SURFACE ( )  );
#37778=VERTEX_POINT ( 'NONE', #20281 ) ;
#37781=AXIS2_PLACEMENT_3D ( 'NONE', #18106, #33124, #48163 ) ;
#37783=CARTESIAN_POINT ( 'NONE',  ( -13.46747565276156422, -9.034678650756244878, 60.73950277887485072 ) ) ;
#37786=( BOUNDED_SURFACE ( )  B_SPLINE_SURFACE ( 3, 1, ( 
 ( #37917, #46223 ),
 ( #24065, #1393 ),
 ( #8813, #33974 ),
 ( #5350, #39316 ),
 ( #35128, #16410 ),
 ( #4202, #19209 ),
 ( #15249, #272 ) ),
 .UNSPECIFIED., .T., .F., .F. ) 
 B_SPLINE_SURFACE_WITH_KNOTS ( ( 4, 3, 4 ),
 ( 2, 2 ),
 ( 0.000000000000000000, 0.5000000000000000000, 1.000000000000000000 ),
 ( 0.000000000000000000, 1.000000000000000000 ),
 .UNSPECIFIED. ) 
 GEOMETRIC_REPRESENTATION_ITEM ( )  RATIONAL_B_SPLINE_SURFACE ( (
 ( 1.000000000000000000, 1.000000000000000000),
 ( 0.3333333333333335369, 0.3333333333333330373),
 ( 0.3333333333333335369, 0.3333333333333330373),
 ( 1.000000000000000000, 1.000000000000000000),
 ( 0.3333333333333333703, 0.3333333333333333703),
 ( 0.3333333333333333703, 0.3333333333333333703),
 ( 1.000000000000000000, 1.000000000000000000) ) ) 
 REPRESENTATION_ITEM ( '' )  SURFACE ( )  );
#37788=EDGE_CURVE ( 'NONE', #32695, #32895, #39909, .T. ) ;
#37789=CARTESIAN_POINT ( 'NONE',  ( -10.69992066440855361, -12.66433694503948004, 67.88265386532016521 ) ) ;
#37791=AXIS2_PLACEMENT_3D ( 'NONE', #7344, #2888, #22590 ) ;
#37792=CARTESIAN_POINT ( 'NONE',  ( -23.77562434277295367, -17.86939608417919345, 59.01850491586762359 ) ) ;
#37793=ORIENTED_EDGE ( 'NONE', *, *, #48471, .F. ) ;
#37796=CARTESIAN_POINT ( 'NONE',  ( -12.57352595576265308, -9.154542183914287534, 74.51261323680796522 ) ) ;
#37797=CARTESIAN_POINT ( 'NONE',  ( -12.56341008138639026, -9.163283831748978869, 74.41948763787014798 ) ) ;
#37798=CARTESIAN_POINT ( 'NONE',  ( -11.36918367646109651, -19.26602422791083669, 53.76227901944321275 ) ) ;
#37800=ORIENTED_EDGE ( 'NONE', *, *, #23270, .T. ) ;
#37801=CARTESIAN_POINT ( 'NONE',  ( -17.84478125091072087, -22.24806977446377942, 62.06191208170499607 ) ) ;
#37802=CARTESIAN_POINT ( 'NONE',  ( -24.20525988284104457, -11.72391474569057124, 59.67574024123567256 ) ) ;
#37804=CYLINDRICAL_SURFACE ( 'NONE', #111, 0.1499999999999956923 ) ;
#37805=ORIENTED_EDGE ( 'NONE', *, *, #12701, .T. ) ;
#37807=FACE_OUTER_BOUND ( 'NONE', #14902, .T. ) ;
#37808=B_SPLINE_CURVE_WITH_KNOTS ( 'NONE', 3,
 ( #44909, #23220, #34273, #11162, #11636, #563, #22739, #41928, #37729, #26668 ),
 .UNSPECIFIED., .F., .F.,
 ( 4, 2, 2, 2, 4 ),
 ( 0.6272669072976760907, 0.7522669073147278951, 0.8772669073317798105, 1.002266907348831726, 1.127266907365883419 ),
 .UNSPECIFIED. ) ;
#37810=FACE_BOUND ( 'NONE', #35098, .T. ) ;
#37812=B_SPLINE_CURVE_WITH_KNOTS ( 'NONE', 3,
 ( #28101, #2000, #9156, #1765, #43127, #47063, #13300, #35482, #16760, #42411 ),
 .UNSPECIFIED., .F., .F.,
 ( 4, 2, 2, 2, 4 ),
 ( 0.000000000000000000, 0.2500000000000000000, 0.5000000000000000000, 0.7500000000000000000, 1.000000000000000000 ),
 .UNSPECIFIED. ) ;
#37813=EDGE_LOOP ( 'NONE', ( #7481, #17802, #46775, #18288, #3688 ) ) ;
#37815=FACE_OUTER_BOUND ( 'NONE', #11127, .T. ) ;
#37817=CARTESIAN_POINT ( 'NONE',  ( -23.62573085457600541, -18.93877797592854506, 65.93734031310268051 ) ) ;
#37820=ORIENTED_EDGE ( 'NONE', *, *, #29619, .T. ) ;
#37821=CARTESIAN_POINT ( 'NONE',  ( -10.44483699753067718, -14.26928449077156813, 64.68803882970183849 ) ) ;
#37822=VERTEX_POINT ( 'NONE', #12643 ) ;
#37824=LINE ( 'NONE', #4119, #19623 ) ;
#37825=ORIENTED_EDGE ( 'NONE', *, *, #44769, .F. ) ;
#37826=CARTESIAN_POINT ( 'NONE',  ( -18.33709340422855050, -22.20310063599641381, 69.00853016400594697 ) ) ;
#37828=ADVANCED_FACE ( 'NONE', ( #16567 ), #46866, .T. ) ;
#37830=EDGE_LOOP ( 'NONE', ( #14835, #42503, #42138, #10635, #26833 ) ) ;
#37831=CARTESIAN_POINT ( 'NONE',  ( -18.29367245688808552, -17.15309925898211318, 75.49999999999994316 ) ) ;
#37832=CARTESIAN_POINT ( 'NONE',  ( -22.86572475812252847, -14.01004878893095196, 53.49999999999995026 ) ) ;
#37835=FACE_OUTER_BOUND ( 'NONE', #34785, .T. ) ;
#37836=CARTESIAN_POINT ( 'NONE',  ( -24.17271927670314113, -12.95015993349377048, 66.30246741691458112 ) ) ;
#37837=CARTESIAN_POINT ( 'NONE',  ( -14.09914604623946488, -8.649277798895779412, 74.19954655170327840 ) ) ;
#37838=CARTESIAN_POINT ( 'NONE',  ( -12.50249420765911701, -20.40225435000794008, 71.98466421126660464 ) ) ;
#37839=EDGE_LOOP ( 'NONE', ( #40325, #29359, #5502, #29458, #20308 ) ) ;
#37840=EDGE_LOOP ( 'NONE', ( #25552, #15338, #41551, #18632, #2989 ) ) ;
#37841=EDGE_CURVE ( 'NONE', #17387, #18626, #48420, .T. ) ;
#37842=EDGE_CURVE ( 'NONE', #10553, #10266, #45780, .T. ) ;
#37843=CARTESIAN_POINT ( 'NONE',  ( -12.09292629619409531, -10.27274204020369197, 64.25587718757367384 ) ) ;
#37847=CARTESIAN_POINT ( 'NONE',  ( -10.52991701743181174, -16.02177613136639067, 67.97767831076122036 ) ) ;
#37848=EDGE_CURVE ( 'NONE', #48456, #39905, #6428, .T. ) ;
#37851=ORIENTED_EDGE ( 'NONE', *, *, #1831, .F. ) ;
#37852=VECTOR ( 'NONE', #33705, 1000.000000000000227 ) ;
#37853=CARTESIAN_POINT ( 'NONE',  ( -16.20683463515880973, -21.70255690700738782, 58.28585572422844052 ) ) ;
#37855=CARTESIAN_POINT ( 'NONE',  ( -15.42745694218142027, -21.51847616057531809, 68.80266276951817872 ) ) ;
#37857=CARTESIAN_POINT ( 'NONE',  ( -15.29809632361469873, -21.47854941203162937, 68.57592918283285144 ) ) ;
#37858=ORIENTED_EDGE ( 'NONE', *, *, #33209, .T. ) ;
#37860=CARTESIAN_POINT ( 'NONE',  ( -15.76027622468541978, -7.547319663497244591, 67.33281406147084169 ) ) ;
#37861=CARTESIAN_POINT ( 'NONE',  ( -12.10369346210734243, -9.594120923840563364, 57.27430859790474926 ) ) ;
#37862=ORIENTED_EDGE ( 'NONE', *, *, #11299, .T. ) ;
#37863=VECTOR ( 'NONE', #30910, 1000.000000000000114 ) ;
#37864=FACE_OUTER_BOUND ( 'NONE', #28250, .T. ) ;
#37865=B_SPLINE_CURVE_WITH_KNOTS ( 'NONE', 1,
 ( #8071, #23080 ),
 .UNSPECIFIED., .F., .F.,
 ( 2, 2 ),
 ( 0.000000000000000000, 1.000000000000000000 ),
 .UNSPECIFIED. ) ;
#37867=DIRECTION ( 'NONE',  ( 0.9893874368562762811, -0.1453014101478983522, 1.482692748682355818E-17 ) ) ;
#37869=CARTESIAN_POINT ( 'NONE',  ( -10.50466007945005487, -15.86899602918702001, 64.80771547851877301 ) ) ;
#37870=ORIENTED_EDGE ( 'NONE', *, *, #13422, .F. ) ;
#37871=CARTESIAN_POINT ( 'NONE',  ( -14.77897477670383353, -8.270997283837589364, 56.73511376018900876 ) ) ;
#37872=ORIENTED_EDGE ( 'NONE', *, *, #25817, .F. ) ;
#37874=CARTESIAN_POINT ( 'NONE',  ( -24.55824875695236287, -12.66269769826935310, 70.02888935069151444 ) ) ;
#37876=CARTESIAN_POINT ( 'NONE',  ( -11.46780417137699004, -10.33417537808259823, 74.54610936257664378 ) ) ;
#37877=VERTEX_POINT ( 'NONE', #17768 ) ;
#37878=CARTESIAN_POINT ( 'NONE',  ( -22.11926001268504294, -9.024814352312150234, 63.30658345311071855 ) ) ;
#37879=EDGE_CURVE ( 'NONE', #22956, #31810, #3252, .T. ) ;
#37880=LINE ( 'NONE', #30990, #771 ) ;
#37881=CARTESIAN_POINT ( 'NONE',  ( -10.92393591598462166, -17.40806730853362794, 68.11338529727301250 ) ) ;
#37883=CARTESIAN_POINT ( 'NONE',  ( -19.24513076412772961, -8.048561166981372139, 63.54162403522450830 ) ) ;
#37884=CARTESIAN_POINT ( 'NONE',  ( -18.76558283008973049, -7.480892646508040755, 70.55563411965815135 ) ) ;
#37888=EDGE_LOOP ( 'NONE', ( #26547, #5575 ) ) ;
#37892=DIRECTION ( 'NONE',  ( -9.352133734048191489E-06, -6.779811745274577181E-06, -0.9999999999332859213 ) ) ;
#37895=CARTESIAN_POINT ( 'NONE',  ( -10.59656512619885227, -13.05092609425065397, 68.02360230423870746 ) ) ;
#37896=CARTESIAN_POINT ( 'NONE',  ( -12.35277413765887999, -20.26681541663451114, 68.45162113748973809 ) ) ;
#37898=CARTESIAN_POINT ( 'NONE',  ( -17.65006842549283306, -20.30456235612524196, 53.49999999999995026 ) ) ;
#37899=ORIENTED_EDGE ( 'NONE', *, *, #1140, .F. ) ;
#37900=CYLINDRICAL_SURFACE ( 'NONE', #21070, 0.1500000000000019651 ) ;
#37903=CARTESIAN_POINT ( 'NONE',  ( -21.95938932932862642, -9.477124872050278981, 60.02171213236835712 ) ) ;
#37905=EDGE_LOOP ( 'NONE', ( #37229, #41500 ) ) ;
#37906=EDGE_CURVE ( 'NONE', #28606, #26764, #14724, .T. ) ;
#37908=DIRECTION ( 'NONE',  ( 0.4433615477241707459, -0.8963428685495451465, 2.661652803430218851E-08 ) ) ;
#37909=CARTESIAN_POINT ( 'NONE',  ( -13.30562964713168306, -21.01738586623506677, 61.70984649199183991 ) ) ;
#37910=DIRECTION ( 'NONE',  ( -0.1453014101478919129, -0.9893874368562773913, 2.030021817369025738E-16 ) ) ;
#37911=EDGE_CURVE ( 'NONE', #5353, #4057, #28752, .T. ) ;
#37912=( BOUNDED_SURFACE ( )  B_SPLINE_SURFACE ( 3, 1, ( 
 ( #36040, #29151 ),
 ( #47394, #36748 ),
 ( #21038, #3037 ),
 ( #3292, #17569 ),
 ( #36515, #24977 ),
 ( #21292, #2322 ),
 ( #10679, #28906 ) ),
 .UNSPECIFIED., .T., .F., .F. ) 
 B_SPLINE_SURFACE_WITH_KNOTS ( ( 4, 3, 4 ),
 ( 2, 2 ),
 ( 0.000000000000000000, 0.5000000000000000000, 1.000000000000000000 ),
 ( 0.000000000000000000, 1.000000000000000000 ),
 .UNSPECIFIED. ) 
 GEOMETRIC_REPRESENTATION_ITEM ( )  RATIONAL_B_SPLINE_SURFACE ( (
 ( 1.000000000000000000, 1.000000000000000000),
 ( 0.3333333333333335369, 0.3333333333333330373),
 ( 0.3333333333333335369, 0.3333333333333330373),
 ( 1.000000000000000000, 1.000000000000000000),
 ( 0.3333333333333333703, 0.3333333333333333703),
 ( 0.3333333333333333703, 0.3333333333333333703),
 ( 1.000000000000000000, 1.000000000000000000) ) ) 
 REPRESENTATION_ITEM ( '' )  SURFACE ( )  );
#37914=CARTESIAN_POINT ( 'NONE',  ( -24.47354778464749003, -12.39902454472287197, 73.42720984402279782 ) ) ;
#37915=CARTESIAN_POINT ( 'NONE',  ( -14.48548941065490148, -8.400516866317895293, 67.27447142263336843 ) ) ;
#37917=CARTESIAN_POINT ( 'NONE',  ( -22.48964968825576705, -9.905448439006629968, 73.76689030015370463 ) ) ;
#37918=CARTESIAN_POINT ( 'NONE',  ( -24.45320359087931550, -14.22178767528806276, 66.39112731077266005 ) ) ;
#37919=CARTESIAN_POINT ( 'NONE',  ( -11.96181431063714484, -19.87549516500596525, 58.11177798925346139 ) ) ;
#37922=( BOUNDED_CURVE ( )  B_SPLINE_CURVE ( 3, ( #36851, #6603, #18148, #47963 ),
 .UNSPECIFIED., .F., .F. ) 
 B_SPLINE_CURVE_WITH_KNOTS ( ( 4, 4 ),
 ( 0.5000000000000000000, 0.9074455897393689519 ),
 .UNSPECIFIED. ) 
 CURVE ( )  GEOMETRIC_REPRESENTATION_ITEM ( )  RATIONAL_B_SPLINE_CURVE ( ( 0.9999999999999958922, 0.4567392136813261949, 0.3561768502900309885, 0.6983129098261057210 ) ) 
 REPRESENTATION_ITEM ( '' )  );
#37924=DIRECTION ( 'NONE',  ( -1.295331064632368052E-06, 6.890485867068654572E-07, 0.9999999999989236388 ) ) ;
#37927=CARTESIAN_POINT ( 'NONE',  ( -13.35550522631041837, -8.568183888810063209, 57.15463030501995689 ) ) ;
#37928=CARTESIAN_POINT ( 'NONE',  ( -24.32420487361504868, -13.34567816304479848, 62.92444446668879721 ) ) ;
#37930=DIRECTION ( 'NONE',  ( -8.563106570025498363E-06, 6.519502999113576510E-06, -0.9999999999420846608 ) ) ;
#37931=EDGE_CURVE ( 'NONE', #39283, #7665, #8799, .T. ) ;
#37933=CARTESIAN_POINT ( 'NONE',  ( -24.43827367352892210, -15.52193379869737200, 73.28831629023289906 ) ) ;
#37934=CARTESIAN_POINT ( 'NONE',  ( -13.41559485503361948, -8.529420403834853559, 57.08472365561223683 ) ) ;
#37935=EDGE_LOOP ( 'NONE', ( #13979, #32190, #7300, #22171, #26651 ) ) ;
#37936=CARTESIAN_POINT ( 'NONE',  ( -11.79792781917550570, -18.97409009807959279, 71.68685885149984927 ) ) ;
#37937=CARTESIAN_POINT ( 'NONE',  ( -13.10977233404386944, -20.39504592733330313, 58.19083229533344337 ) ) ;
#37938=PLANE ( 'NONE',  #45486 ) ;
#37940=CARTESIAN_POINT ( 'NONE',  ( -23.79763979734637402, -18.66673721458791491, 72.96357004385932044 ) ) ;
#37943=CARTESIAN_POINT ( 'NONE',  ( -18.86321414053259105, -7.899510124550229051, 73.98497555292401273 ) ) ;
#37945=ORIENTED_EDGE ( 'NONE', *, *, #46096, .F. ) ;
#37946=CARTESIAN_POINT ( 'NONE',  ( -24.00225416124087374, -17.20718635581271272, 72.99409062911038859 ) ) ;
#37947=CARTESIAN_POINT ( 'NONE',  ( -15.26209398273251772, -21.93938324809698770, 68.68937616499954402 ) ) ;
#37951=CARTESIAN_POINT ( 'NONE',  ( -22.38400322090610217, -20.36826016184844335, 62.41934579407823236 ) ) ;
#37953=FACE_OUTER_BOUND ( 'NONE', #25622, .T. ) ;
#37957=CARTESIAN_POINT ( 'NONE',  ( -24.32886716615087153, -16.23426984194678724, 62.60800820172418923 ) ) ;
#37958=CARTESIAN_POINT ( 'NONE',  ( -11.82099749022622426, -9.899105802180386604, 64.21409645106085406 ) ) ;
#37959=B_SPLINE_CURVE_WITH_KNOTS ( 'NONE', 3,
 ( #13156, #35815, #6032, #13643, #2341, #28684, #1612, #24994, #43968, #47644 ),
 .UNSPECIFIED., .F., .F.,
 ( 4, 2, 2, 2, 4 ),
 ( 0.000000000000000000, 0.2500000000000000000, 0.5000000000000000000, 0.7500000000000000000, 1.000000000000000000 ),
 .UNSPECIFIED. ) ;
#37962=EDGE_LOOP ( 'NONE', ( #32193, #17794, #26702, #16265, #36908 ) ) ;
#37963=CARTESIAN_POINT ( 'NONE',  ( -20.16691211377460391, -21.73601867580754288, 72.58974061177721637 ) ) ;
#37964=ADVANCED_FACE ( 'NONE', ( #21254 ), #19822, .T. ) ;
#37965=ORIENTED_EDGE ( 'NONE', *, *, #31552, .F. ) ;
#37967=CARTESIAN_POINT ( 'NONE',  ( -21.62565899036455264, -11.23921691435401904, 53.88362224778187226 ) ) ;
#37969=CARTESIAN_POINT ( 'NONE',  ( -13.34909364474977522, -8.572319965759302107, 57.14684612213136461 ) ) ;
#37970=CARTESIAN_POINT ( 'NONE',  ( -16.91478550490786503, -21.84108428878278119, 72.18015306840750611 ) ) ;
#37971=VECTOR ( 'NONE', #10911, 1000.000000000000227 ) ;
#37972=VERTEX_POINT ( 'NONE', #26389 ) ;
#37973=CARTESIAN_POINT ( 'NONE',  ( -13.87299615820197296, -20.90301826156740717, 72.34096506744559463 ) ) ;
#37974=ORIENTED_EDGE ( 'NONE', *, *, #21210, .T. ) ;
#37975=CARTESIAN_POINT ( 'NONE',  ( -22.37828812292848824, -20.37331024823514980, 62.42713317377827309 ) ) ;
#37976=EDGE_CURVE ( 'NONE', #4804, #6954, #12871, .T. ) ;
#37977=CARTESIAN_POINT ( 'NONE',  ( -23.98474789688958353, -17.25007084823549874, 69.71339792561613535 ) ) ;
#37980=CARTESIAN_POINT ( 'NONE',  ( -24.87450840884172365, -14.73858704721042123, 59.35644987740099765 ) ) ;
#37981=CARTESIAN_POINT ( 'NONE',  ( -11.05753579597473113, -11.89914114276540680, 74.55840159191156147 ) ) ;
#37982=CARTESIAN_POINT ( 'NONE',  ( -18.75492427513048455, -7.882278092513721468, 73.93244671259982681 ) ) ;
#37983=EDGE_CURVE ( 'NONE', #19518, #43128, #3995, .T. ) ;
#37985=CARTESIAN_POINT ( 'NONE',  ( -10.93089496422971330, -11.15644115613137188, 64.32694814133255079 ) ) ;
#37986=CARTESIAN_POINT ( 'NONE',  ( -17.72612443559818018, -7.765381109175947927, 60.36588690973874094 ) ) ;
#37987=EDGE_CURVE ( 'NONE', #24972, #10986, #24846, .T. ) ;
#37988=CARTESIAN_POINT ( 'NONE',  ( -14.60079031338673516, -21.70357006634377584, 58.35892056026858654 ) ) ;
#37989=CARTESIAN_POINT ( 'NONE',  ( -24.08517543038346531, -12.49907855475201579, 73.52753481283211556 ) ) ;
#37990=VERTEX_POINT ( 'NONE', #37951 ) ;
#37991=CARTESIAN_POINT ( 'NONE',  ( -11.45751978572037011, -19.27057081285444085, 71.87181161472111057 ) ) ;
#37992=CARTESIAN_POINT ( 'NONE',  ( -24.38391081516821401, -14.06024225110868464, 73.12271507915593816 ) ) ;
#37993=CARTESIAN_POINT ( 'NONE',  ( -11.07877888056294147, -17.89008669626860737, 71.56718224920616933 ) ) ;
#37994=CARTESIAN_POINT ( 'NONE',  ( -23.56138519289638822, -11.33989039198723248, 69.89210750373884196 ) ) ;
#37997=ORIENTED_EDGE ( 'NONE', *, *, #46963, .F. ) ;
#38000=VERTEX_POINT ( 'NONE', #34249 ) ;
#38001=CARTESIAN_POINT ( 'NONE',  ( -11.30641337201207364, -19.06087391327494629, 68.31715392936506248 ) ) ;
#38002=CARTESIAN_POINT ( 'NONE',  ( -22.52510391186153171, -10.01533143912503832, 73.48161092902591918 ) ) ;
#38003=CARTESIAN_POINT ( 'NONE',  ( -14.67456088659309899, -21.24707878532894512, 58.45001277033151155 ) ) ;
#38004=EDGE_LOOP ( 'NONE', ( #32482, #27949, #24043, #6438, #19651 ) ) ;
#38005=FACE_OUTER_BOUND ( 'NONE', #8990, .T. ) ;
#38006=CARTESIAN_POINT ( 'NONE',  ( -16.66933960180709917, -7.791706125978248743, 74.11585391104840426 ) ) ;
#38007=CARTESIAN_POINT ( 'NONE',  ( -17.42409385541300892, -14.80920654474439679, 54.49999999999994316 ) ) ;
#38009=AXIS2_PLACEMENT_3D ( 'NONE', #27816, #44014, #31518 ) ;
#38011=CARTESIAN_POINT ( 'NONE',  ( -12.90354087724769272, -8.887350501024684490, 67.49447389996370816 ) ) ;
#38013=CARTESIAN_POINT ( 'NONE',  ( -14.04637585414641165, -8.168855721704870732, 70.83619327840688129 ) ) ;
#38014=CARTESIAN_POINT ( 'NONE',  ( -21.15569899156770717, -20.79502053738513112, 72.82446725055457648 ) ) ;
#38018=EDGE_CURVE ( 'NONE', #7220, #28, #28142, .T. ) ;
#38019=CARTESIAN_POINT ( 'NONE',  ( -13.87677485259778543, -8.712488334168142501, 74.40774694939290157 ) ) ;
#38023=B_SPLINE_CURVE_WITH_KNOTS ( 'NONE', 3,
 ( #4072, #34079, #18828, #11937, #8017, #34315, #33835, #11684, #23029, #15115 ),
 .UNSPECIFIED., .F., .F.,
 ( 4, 2, 2, 2, 4 ),
 ( 0.000000000000000000, 0.2500000000000000000, 0.5000000000000000000, 0.7500000000000000000, 1.000000000000000000 ),
 .UNSPECIFIED. ) ;
#38024=FACE_OUTER_BOUND ( 'NONE', #34913, .T. ) ;
#38026=CARTESIAN_POINT ( 'NONE',  ( -22.33376602745314798, -19.86903051493498040, 69.18890041286789483 ) ) ;
#38027=DIRECTION ( 'NONE',  ( 6.885933443815673122E-06, -1.077603661396111343E-05, 0.9999999999182304089 ) ) ;
#38030=EDGE_CURVE ( 'NONE', #7125, #6672, #26398, .T. ) ;
#38032=CARTESIAN_POINT ( 'NONE',  ( -22.24723880939002996, -9.656319818818069223, 59.86604062818025795 ) ) ;
#38033=CARTESIAN_POINT ( 'NONE',  ( -9.974130135034549482, -14.85786239279031840, 74.97591673537033330 ) ) ;
#38034=EDGE_CURVE ( 'NONE', #18836, #32319, #31725, .T. ) ;
#38035=CARTESIAN_POINT ( 'NONE',  ( -23.74619254753875808, -11.68933987248222550, 63.10218278636759237 ) ) ;
#38037=CARTESIAN_POINT ( 'NONE',  ( -12.06140467229625912, -20.05244645202335008, 54.27966884056654351 ) ) ;
#38038=EDGE_CURVE ( 'NONE', #33140, #4721, #29881, .T. ) ;
#38040=CARTESIAN_POINT ( 'NONE',  ( -17.91451304303208403, -22.24313331792350112, 61.99040607801043734 ) ) ;
#38043=CARTESIAN_POINT ( 'NONE',  ( -17.03575403388767384, -5.365376231199011414, 53.49999999999995026 ) ) ;
#38044=ORIENTED_EDGE ( 'NONE', *, *, #7217, .F. ) ;
#38045=DIRECTION ( 'NONE',  ( -0.8967515337576290602, 0.4425343904188011046, -9.546469663397771497E-09 ) ) ;
#38047=CARTESIAN_POINT ( 'NONE',  ( -16.26183769579148475, -7.855670737815882987, 60.50028478907629648 ) ) ;
#38048=CARTESIAN_POINT ( 'NONE',  ( -13.38462656077074442, -20.58719956993326861, 58.19650077713541947 ) ) ;
#38051=B_SPLINE_CURVE_WITH_KNOTS ( 'NONE', 1,
 ( #43699, #28902 ),
 .UNSPECIFIED., .F., .F.,
 ( 2, 2 ),
 ( 0.000000000000000000, 1.000000000000000000 ),
 .UNSPECIFIED. ) ;
#38056=FACE_OUTER_BOUND ( 'NONE', #3608, .T. ) ;
#38058=CARTESIAN_POINT ( 'NONE',  ( -12.70343478140934224, -9.045698024298063800, 70.94901720388561728 ) ) ;
#38059=CARTESIAN_POINT ( 'NONE',  ( -12.14425528403576848, -10.13739698163135117, 64.02914326607979945 ) ) ;
#38060=ORIENTED_EDGE ( 'NONE', *, *, #28932, .F. ) ;
#38061=( BOUNDED_SURFACE ( )  B_SPLINE_SURFACE ( 3, 1, ( 
 ( #9539, #36091 ),
 ( #21343, #17384 ),
 ( #31690, #39069 ),
 ( #36336, #24562 ),
 ( #13675, #9051 ),
 ( #5352, #2615 ),
 ( #43511, #43752 ) ),
 .UNSPECIFIED., .T., .F., .F. ) 
 B_SPLINE_SURFACE_WITH_KNOTS ( ( 4, 3, 4 ),
 ( 2, 2 ),
 ( 0.000000000000000000, 0.5000000000000000000, 1.000000000000000000 ),
 ( 0.000000000000000000, 1.000000000000000000 ),
 .UNSPECIFIED. ) 
 GEOMETRIC_REPRESENTATION_ITEM ( )  RATIONAL_B_SPLINE_SURFACE ( (
 ( 1.000000000000000000, 1.000000000000000000),
 ( 0.3333333333333335369, 0.3333333333333330373),
 ( 0.3333333333333335369, 0.3333333333333330373),
 ( 1.000000000000000000, 1.000000000000000000),
 ( 0.3333333333333333703, 0.3333333333333333703),
 ( 0.3333333333333333703, 0.3333333333333333703),
 ( 1.000000000000000000, 1.000000000000000000) ) ) 
 REPRESENTATION_ITEM ( '' )  SURFACE ( )  );
#38062=CARTESIAN_POINT ( 'NONE',  ( -10.96962953718779232, -17.51874670794821043, 68.39721950254519811 ) ) ;
#38067=B_SPLINE_CURVE_WITH_KNOTS ( 'NONE', 3,
 ( #15662, #662, #42027, #30717, #34624, #45743, #15907, #1625, #34866, #30952 ),
 .UNSPECIFIED., .F., .F.,
 ( 4, 2, 2, 2, 4 ),
 ( 0.6272669072783326749, 0.7522669073002039575, 0.8772669073220753511, 1.002266907343946745, 1.127266907365817916 ),
 .UNSPECIFIED. ) ;
#38068=CARTESIAN_POINT ( 'NONE',  ( -19.38354029837526937, -21.99704006310037130, 58.70224247979420085 ) ) ;
#38069=DIRECTION ( 'NONE',  ( -0.7670373483544790094, -0.6416024518573233415, 2.496223344567222537E-08 ) ) ;
#38070=CARTESIAN_POINT ( 'NONE',  ( -24.16171830865566861, -12.91022455891425125, 66.30246698681006023 ) ) ;
#38073=( BOUNDED_CURVE ( )  B_SPLINE_CURVE ( 3, ( #45639, #4992, #38206, #20003 ),
 .UNSPECIFIED., .F., .F. ) 
 B_SPLINE_CURVE_WITH_KNOTS ( ( 4, 4 ),
 ( 0.4074455897393702841, 0.5000000000000000000 ),
 .UNSPECIFIED. ) 
 CURVE ( )  GEOMETRIC_REPRESENTATION_ITEM ( )  RATIONAL_B_SPLINE_CURVE ( ( 0.6983129098261073864, 0.7760317562607140784, 0.8765941196520128376, 1.000000000000005773 ) ) 
 REPRESENTATION_ITEM ( '' )  );
#38077=B_SPLINE_CURVE_WITH_KNOTS ( 'NONE', 3,
 ( #5347, #31923, #23824, #34645, #1644, #42537, #27742, #16405, #4869, #16883 ),
 .UNSPECIFIED., .F., .F.,
 ( 4, 2, 2, 2, 4 ),
 ( 0.000000000000000000, 0.2500000000000000000, 0.5000000000000000000, 0.7500000000000000000, 1.000000000000000000 ),
 .UNSPECIFIED. ) ;
#38078=CARTESIAN_POINT ( 'NONE',  ( -17.79901357976508791, -7.766176623049141803, 63.96545652844361740 ) ) ;
#38080=EDGE_CURVE ( 'NONE', #6697, #24590, #15835, .T. ) ;
#38081=FACE_OUTER_BOUND ( 'NONE', #24946, .T. ) ;
#38083=CARTESIAN_POINT ( 'NONE',  ( -23.16275847746607752, -18.91806288495012112, 69.43805163930900903 ) ) ;
#38084=ORIENTED_EDGE ( 'NONE', *, *, #29266, .T. ) ;
#38086=ORIENTED_EDGE ( 'NONE', *, *, #31717, .F. ) ;
#38087=CARTESIAN_POINT ( 'NONE',  ( -17.06879511326789256, -7.767867012253359071, 73.97490359703523666 ) ) ;
#38088=CARTESIAN_POINT ( 'NONE',  ( -12.05727448861903639, -19.97649948735875114, 61.65324539733175868 ) ) ;
#38089=DIRECTION ( 'NONE',  ( -0.5652317888644006194, -0.8249321334856242194, 7.911723905267717726E-08 ) ) ;
#38090=ORIENTED_EDGE ( 'NONE', *, *, #1294, .F. ) ;
#38094=EDGE_CURVE ( 'NONE', #35350, #20172, #34897, .T. ) ;
#38095=CARTESIAN_POINT ( 'NONE',  ( -22.78151503426583702, -19.98625364524674097, 72.75905110386234753 ) ) ;
#38096=ORIENTED_EDGE ( 'NONE', *, *, #23137, .F. ) ;
#38098=CYLINDRICAL_SURFACE ( 'NONE', #28357, 0.1499999999999988287 ) ;
#38099=CARTESIAN_POINT ( 'NONE',  ( -20.16899036125798972, -7.883296231106626806, 73.82122343779342089 ) ) ;
#38100=ORIENTED_EDGE ( 'NONE', *, *, #40762, .T. ) ;
#38101=LINE ( 'NONE', #3911, #3155 ) ;
#38102=VERTEX_POINT ( 'NONE', #1498 ) ;
#38104=CARTESIAN_POINT ( 'NONE',  ( -10.18364478422453345, -13.05433800282328960, 71.46474530336836040 ) ) ;
#38105=EDGE_CURVE ( 'NONE', #31313, #19293, #6293, .T. ) ;
#38106=ADVANCED_FACE ( 'NONE', ( #20470 ), #35465, .T. ) ;
#38107=CARTESIAN_POINT ( 'NONE',  ( -24.35389707626741185, -16.10709931453381216, 62.87856533165624029 ) ) ;
#38108=ORIENTED_EDGE ( 'NONE', *, *, #25832, .F. ) ;
#38109=CARTESIAN_POINT ( 'NONE',  ( -24.26384900572966075, -13.06773595597165460, 69.91676003018049812 ) ) ;
#38112=DIRECTION ( 'NONE',  ( 0.5540494244615011832, -0.8324837747691418155, 2.496966302803637394E-17 ) ) ;
#38114=CARTESIAN_POINT ( 'NONE',  ( -22.13027617770598354, -9.033668753454486833, 63.35300274347135741 ) ) ;
#38117=CARTESIAN_POINT ( 'NONE',  ( -11.46207494020916862, -11.14107511578148113, 57.49437795721348010 ) ) ;
#38118=EDGE_LOOP ( 'NONE', ( #22976, #15934 ) ) ;
#38120=EDGE_CURVE ( 'NONE', #40496, #28056, #3852, .T. ) ;
#38122=ORIENTED_EDGE ( 'NONE', *, *, #17901, .F. ) ;
#38124=CARTESIAN_POINT ( 'NONE',  ( -10.64242474325409304, -12.85371797616438272, 71.35261706278205907 ) ) ;
#38125=B_SPLINE_CURVE_WITH_KNOTS ( 'NONE', 3,
 ( #14879, #21581, #21812, #26238, #3579, #33858, #6794, #13912, #44475, #3090 ),
 .UNSPECIFIED., .F., .F.,
 ( 4, 2, 2, 2, 4 ),
 ( 0.1272669073658506955, 0.2522669073463346678, 0.3772669073268186679, 0.5022669073073026125, 0.6272669072877865570 ),
 .UNSPECIFIED. ) ;
#38128=CARTESIAN_POINT ( 'NONE',  ( -12.43268922994311509, -19.71711825911901528, 61.69678636630293056 ) ) ;
#38129=CARTESIAN_POINT ( 'NONE',  ( -12.69763806180496601, -20.04058448603118592, 68.62185382311069759 ) ) ;
#38131=CARTESIAN_POINT ( 'NONE',  ( -12.14425506381237163, -10.13739722748950634, 64.32914326607961186 ) ) ;
#38133=DIRECTION ( 'NONE',  ( -9.593247862760507776E-06, -5.650837228699102996E-06, 0.9999999999380188020 ) ) ;
#38134=B_SPLINE_CURVE_WITH_KNOTS ( 'NONE', 3,
 ( #24515, #36517, #20802, #17333, #1845, #13633, #35802, #9241, #2079, #17080 ),
 .UNSPECIFIED., .F., .F.,
 ( 4, 2, 2, 2, 4 ),
 ( 0.000000000000000000, 0.2500000000000000000, 0.5000000000000000000, 0.7500000000000000000, 1.000000000000000000 ),
 .UNSPECIFIED. ) ;
#38135=CARTESIAN_POINT ( 'NONE',  ( -10.02898863523709316, -13.90543673706342886, 57.62541899832793035 ) ) ;
#38136=CARTESIAN_POINT ( 'NONE',  ( -21.90037927395905371, -9.427412627673714240, 59.73673662101968063 ) ) ;
#38137=ORIENTED_EDGE ( 'NONE', *, *, #27492, .F. ) ;
#38138=AXIS2_PLACEMENT_3D ( 'NONE', #25783, #26518, #3127 ) ;
#38139=ORIENTED_EDGE ( 'NONE', *, *, #17372, .F. ) ;
#38142=CARTESIAN_POINT ( 'NONE',  ( -24.86610161942810038, -14.46236550061385984, 66.29797407254456232 ) ) ;
#38143=CARTESIAN_POINT ( 'NONE',  ( -15.71124685674608124, -7.966721484443281653, 74.17165852965567296 ) ) ;
#38144=CARTESIAN_POINT ( 'NONE',  ( -22.04114742393716142, -9.481025248639417313, 59.73643293354757589 ) ) ;
#38145=EDGE_CURVE ( 'NONE', #383, #27062, #44037, .T. ) ;
#38148=CARTESIAN_POINT ( 'NONE',  ( -22.96481576609224717, -19.16891988936071556, 58.89882756593014790 ) ) ;
#38153=VERTEX_POINT ( 'NONE', #10104 ) ;
#38154=CARTESIAN_POINT ( 'NONE',  ( -12.55411140858086760, -19.90724249994213935, 65.15202838036978505 ) ) ;
#38155=ORIENTED_EDGE ( 'NONE', *, *, #28577, .T. ) ;
#38156=B_SPLINE_CURVE_WITH_KNOTS ( 'NONE', 3,
 ( #38992, #20288, #35293, #47371, #25433, #6242, #28881, #24482, #40444, #39970 ),
 .UNSPECIFIED., .F., .F.,
 ( 4, 2, 2, 2, 4 ),
 ( 0.000000000000000000, 0.2500000000000000000, 0.5000000000000000000, 0.7500000000000000000, 1.000000000000000000 ),
 .UNSPECIFIED. ) ;
#38159=VERTEX_POINT ( 'NONE', #14247 ) ;
#38160=CARTESIAN_POINT ( 'NONE',  ( -13.77528250856571645, -8.773395728905704516, 57.38456636527085664 ) ) ;
#38161=ADVANCED_FACE ( 'NONE', ( #3187 ), #15469, .T. ) ;
#38163=CARTESIAN_POINT ( 'NONE',  ( -17.72419709140651278, -21.80277058947482516, 58.70553378253836030 ) ) ;
#38164=EDGE_CURVE ( 'NONE', #18836, #32319, #4084, .T. ) ;
#38166=CARTESIAN_POINT ( 'NONE',  ( -22.23733827145997566, -19.96043728507621040, 65.70421731380814379 ) ) ;
#38167=EDGE_LOOP ( 'NONE', ( #776, #16319 ) ) ;
#38168=CARTESIAN_POINT ( 'NONE',  ( -14.98249323814573941, -9.880861343182303358, 53.49999999999995026 ) ) ;
#38172=CARTESIAN_POINT ( 'NONE',  ( -22.84361065395838608, -9.697247154002193170, 73.58886925941359891 ) ) ;
#38173=EDGE_LOOP ( 'NONE', ( #24181, #5111, #30317, #5777, #19455 ) ) ;
#38176=DIRECTION ( 'NONE',  ( -0.7111926860893348357, 0.6953514824629878355, 0.1033986416233889510 ) ) ;
#38178=CARTESIAN_POINT ( 'NONE',  ( -24.10561640116403481, -17.05872324192169032, 73.18336028593354570 ) ) ;
#38179=CARTESIAN_POINT ( 'NONE',  ( -15.80117947156642622, -7.538110422750471606, 67.24033040303804398 ) ) ;
#38181=CARTESIAN_POINT ( 'NONE',  ( -20.15615321779684521, -7.878236066423426109, 73.87096600761617538 ) ) ;
#38182=( BOUNDED_CURVE ( )  B_SPLINE_CURVE ( 3, ( #7207, #29595, #44625, #10883 ),
 .UNSPECIFIED., .F., .F. ) 
 B_SPLINE_CURVE_WITH_KNOTS ( ( 4, 4 ),
 ( 0.5000000000000000000, 0.9074455897393655102 ),
 .UNSPECIFIED. ) 
 CURVE ( )  GEOMETRIC_REPRESENTATION_ITEM ( )  RATIONAL_B_SPLINE_CURVE ( ( 0.9999999999999850120, 0.4567392136813225867, 0.3561768502900372058, 0.6983129098261126044 ) ) 
 REPRESENTATION_ITEM ( '' )  );
#38183=CARTESIAN_POINT ( 'NONE',  ( -12.05084272712144511, -19.96988037603709643, 61.51961716641547184 ) ) ;
#38186=ORIENTED_EDGE ( 'NONE', *, *, #18400, .F. ) ;
#38189=CARTESIAN_POINT ( 'NONE',  ( -19.80301260837064703, -21.44571507605098404, 69.23482476707422961 ) ) ;
#38191=CARTESIAN_POINT ( 'NONE',  ( -21.59804182614902146, -20.98026282434625500, 72.70941811628220819 ) ) ;
#38192=( BOUNDED_SURFACE ( )  B_SPLINE_SURFACE ( 3, 1, ( 
 ( #10570, #7374 ),
 ( #21649, #36405 ),
 ( #25580, #10083 ),
 ( #47992, #44547 ),
 ( #3415, #40587 ),
 ( #33193, #18420 ),
 ( #40843, #6872 ) ),
 .UNSPECIFIED., .T., .F., .F. ) 
 B_SPLINE_SURFACE_WITH_KNOTS ( ( 4, 3, 4 ),
 ( 2, 2 ),
 ( 0.000000000000000000, 0.5000000000000000000, 1.000000000000000000 ),
 ( 0.000000000000000000, 1.000000000000000000 ),
 .UNSPECIFIED. ) 
 GEOMETRIC_REPRESENTATION_ITEM ( )  RATIONAL_B_SPLINE_SURFACE ( (
 ( 1.000000000000000000, 1.000000000000000000),
 ( 0.3333333333333335369, 0.3333333333333330373),
 ( 0.3333333333333335369, 0.3333333333333330373),
 ( 1.000000000000000000, 1.000000000000000000),
 ( 0.3333333333333333703, 0.3333333333333333703),
 ( 0.3333333333333333703, 0.3333333333333333703),
 ( 1.000000000000000000, 1.000000000000000000) ) ) 
 REPRESENTATION_ITEM ( '' )  SURFACE ( )  );
#38194=EDGE_LOOP ( 'NONE', ( #41651, #18908, #1799, #44971, #1129 ) ) ;
#38196=EDGE_LOOP ( 'NONE', ( #11399, #20279, #4398, #2569, #36005 ) ) ;
#38197=CARTESIAN_POINT ( 'NONE',  ( -11.64547064851736202, -18.85300969848255193, 64.63218190802510321 ) ) ;
#38198=CARTESIAN_POINT ( 'NONE',  ( -18.85724798917316392, -7.906108138700305155, 67.18599644112759961 ) ) ;
#38201=CARTESIAN_POINT ( 'NONE',  ( -10.80691635537187878, -11.38640170085024828, 67.81853383790260636 ) ) ;
#38203=CARTESIAN_POINT ( 'NONE',  ( -13.62591164035943692, -20.69067956303819145, 65.05799250888908603 ) ) ;
#38204=CARTESIAN_POINT ( 'NONE',  ( -17.70613249112851761, -7.363797380145674865, 60.19405475747598899 ) ) ;
#38205=VERTEX_POINT ( 'NONE', #43366 ) ;
#38206=CARTESIAN_POINT ( 'NONE',  ( -18.07335586441531916, -21.82939548422117682, 65.35091948115599791 ) ) ;
#38207=B_SPLINE_CURVE_WITH_KNOTS ( 'NONE', 3,
 ( #21142, #1700, #2423, #13004, #17434, #47717, #32465, #9096, #47490, #24357 ),
 .UNSPECIFIED., .F., .F.,
 ( 4, 2, 2, 2, 4 ),
 ( 0.000000000000000000, 0.2500000000000000000, 0.5000000000000000000, 0.7500000000000000000, 1.000000000000000000 ),
 .UNSPECIFIED. ) ;
#38209=VERTEX_POINT ( 'NONE', #43607 ) ;
#38210=CARTESIAN_POINT ( 'NONE',  ( -19.74200936563730124, -21.46758226568296024, 68.94954551542706156 ) ) ;
#38213=FACE_OUTER_BOUND ( 'NONE', #21697, .T. ) ;
#38214=CARTESIAN_POINT ( 'NONE',  ( -12.86353962931362283, -9.432586330540292607, 74.33395128836551180 ) ) ;
#38215=CARTESIAN_POINT ( 'NONE',  ( -17.77594298899184366, -7.367433885636743618, 60.26556189360973548 ) ) ;
#38217=CARTESIAN_POINT ( 'NONE',  ( -11.49688049385020960, -18.62690763749001732, 64.76179218520603342 ) ) ;
#38218=EDGE_CURVE ( 'NONE', #21369, #15882, #29363, .T. ) ;
#38220=EDGE_CURVE ( 'NONE', #27631, #2446, #1717, .T. ) ;
#38221=CARTESIAN_POINT ( 'NONE',  ( -16.22585665461787841, -7.910893037574660447, 63.78084232168319545 ) ) ;
#38223=CARTESIAN_POINT ( 'NONE',  ( -12.18836193727821460, -19.53083876418623532, 57.94154444592973618 ) ) ;
#38228=CARTESIAN_POINT ( 'NONE',  ( -22.68646401470678953, -20.08284273627726435, 69.35913316877790180 ) ) ;
#38230=ORIENTED_EDGE ( 'NONE', *, *, #6756, .F. ) ;
#38233=CARTESIAN_POINT ( 'NONE',  ( -24.38441325179858410, -15.93105629309529370, 66.35765103335467074 ) ) ;
#38234=CARTESIAN_POINT ( 'NONE',  ( -23.22802958525249295, -10.13834356547682702, 63.27174767778126352 ) ) ;
#38236=ADVANCED_FACE ( 'NONE', ( #30045 ), #45716, .T. ) ;
#38238=EDGE_CURVE ( 'NONE', #31794, #31985, #4680, .T. ) ;
#38239=CARTESIAN_POINT ( 'NONE',  ( -23.62594491300536959, -11.45603751788689451, 66.70742424642772050 ) ) ;
#38240=AXIS2_PLACEMENT_3D ( 'NONE', #30792, #15240, #8139 ) ;
#38241=CARTESIAN_POINT ( 'NONE',  ( -10.05862335131466700, -15.92885902279982524, 64.69266873560974318 ) ) ;
#38243=CARTESIAN_POINT ( 'NONE',  ( -10.09423541311275763, -16.14245677117450839, 68.15484689107481131 ) ) ;
#38244=ORIENTED_EDGE ( 'NONE', *, *, #30060, .F. ) ;
#38246=CARTESIAN_POINT ( 'NONE',  ( -23.74454562765497556, -11.67923450027144305, 59.36747125042367657 ) ) ;
#38247=CARTESIAN_POINT ( 'NONE',  ( -24.54490520938829334, -12.61907488956320833, 69.97231776601158515 ) ) ;
#38248=CARTESIAN_POINT ( 'NONE',  ( -10.46153521202717229, -17.45973047739676076, 64.77739380354385901 ) ) ;
#38251=ORIENTED_EDGE ( 'NONE', *, *, #5460, .T. ) ;
#38254=DIRECTION ( 'NONE',  ( -0.8459089628457129306, -0.5333273165489313961, 7.771812504399799980E-08 ) ) ;
#38256=CARTESIAN_POINT ( 'NONE',  ( -20.94324281608204430, -8.242681057013424351, 60.09771182510558418 ) ) ;
#38257=CARTESIAN_POINT ( 'NONE',  ( -10.38360249164154325, -14.43747963625415487, 67.87272197508832505 ) ) ;
#38258=CARTESIAN_POINT ( 'NONE',  ( -24.41089624436030547, -15.77327213725850719, 65.94836039739031719 ) ) ;
#38260=CARTESIAN_POINT ( 'NONE',  ( -21.95523233784883033, -8.895446131873137929, 66.77654700642760588 ) ) ;
#38261=EDGE_CURVE ( 'NONE', #11018, #26541, #45551, .T. ) ;
#38265=CARTESIAN_POINT ( 'NONE',  ( -19.78614083979442029, -21.39864764726399216, 69.23482476778590922 ) ) ;
#38266=CARTESIAN_POINT ( 'NONE',  ( -20.21548144266859737, -8.389848675143694479, 66.88990156496440420 ) ) ;
#38267=DIRECTION ( 'NONE',  ( 6.865757730863489906E-07, 1.412849154798944614E-06, 0.9999999999987662092 ) ) ;
#38268=CARTESIAN_POINT ( 'NONE',  ( -10.40245588357037043, -14.17414831712846990, 61.20349182037644198 ) ) ;
#38269=ORIENTED_EDGE ( 'NONE', *, *, #45619, .T. ) ;
#38270=CARTESIAN_POINT ( 'NONE',  ( -10.37818569806566948, -17.22973468411262132, 61.27247807055057649 ) ) ;
#38271=( BOUNDED_CURVE ( )  B_SPLINE_CURVE ( 3, ( #11589, #37928, #26869, #45825 ),
 .UNSPECIFIED., .F., .F. ) 
 B_SPLINE_CURVE_WITH_KNOTS ( ( 4, 4 ),
 ( 0.5000000000000000000, 0.9074455897393649551 ),
 .UNSPECIFIED. ) 
 CURVE ( )  GEOMETRIC_REPRESENTATION_ITEM ( )  RATIONAL_B_SPLINE_CURVE ( ( 1.000000000000047296, 0.4567392136813318571, 0.3561768502899970157, 0.6983129098260942857 ) ) 
 REPRESENTATION_ITEM ( '' )  );
#38273=CARTESIAN_POINT ( 'NONE',  ( -20.13456941707305248, -8.355134980150365820, 70.55100345209505974 ) ) ;
#38274=CARTESIAN_POINT ( 'NONE',  ( -19.52026799707963178, -8.074260338512710078, 60.05273170036824126 ) ) ;
#38275=EDGE_LOOP ( 'NONE', ( #21892, #34058, #19834, #24600, #46027 ) ) ;
#38276=PLANE ( 'NONE',  #34651 ) ;
#38277=CARTESIAN_POINT ( 'NONE',  ( -20.86194851583517362, -21.41857929898468171, 58.74451539084461871 ) ) ;
#38278=CARTESIAN_POINT ( 'NONE',  ( -10.89280197141400919, -11.22507430941316642, 64.33377434530349603 ) ) ;
#38279=CARTESIAN_POINT ( 'NONE',  ( -21.12516169987187098, -20.80993955427394582, 69.06922321213187388 ) ) ;
#38280=SHAPE_DEFINITION_REPRESENTATION ( #40922, #22625 ) ;
#38281=B_SPLINE_CURVE_WITH_KNOTS ( 'NONE', 1,
 ( #40252, #2575 ),
 .UNSPECIFIED., .F., .F.,
 ( 2, 2 ),
 ( 0.000000000000000000, 1.000000000000000000 ),
 .UNSPECIFIED. ) ;
#38282=EDGE_CURVE ( 'NONE', #11545, #34062, #15760, .T. ) ;
#38283=CARTESIAN_POINT ( 'NONE',  ( -11.32469144785209103, -18.34471071427194744, 57.80714594245691984 ) ) ;
#38284=CARTESIAN_POINT ( 'NONE',  ( -10.56627932147773308, -16.21290872759732693, 71.74750383609593030 ) ) ;
#38285=CARTESIAN_POINT ( 'NONE',  ( -24.47371109942907808, -14.90716652360855576, 59.25772288469824645 ) ) ;
#38287=CARTESIAN_POINT ( 'NONE',  ( -17.59331746709300148, -7.761237804004919916, 63.70057029381062819 ) ) ;
#38289=CARTESIAN_POINT ( 'NONE',  ( -12.14070233592774706, -10.21533170167876392, 67.57067125136083519 ) ) ;
#38290=EDGE_CURVE ( 'NONE', #33105, #5915, #48240, .T. ) ;
#38291=ORIENTED_EDGE ( 'NONE', *, *, #14447, .F. ) ;
#38292=CARTESIAN_POINT ( 'NONE',  ( -11.88016137193916677, -19.16921147633432199, 71.57197012879584008 ) ) ;
#38293=CARTESIAN_POINT ( 'NONE',  ( -12.10369268100898132, -9.594121713099781346, 57.27430968559156810 ) ) ;
#38295=FACE_BOUND ( 'NONE', #17638, .T. ) ;
#38297=ORIENTED_EDGE ( 'NONE', *, *, #8995, .F. ) ;
#38300=CARTESIAN_POINT ( 'NONE',  ( -13.41559485503361948, -8.529420403834853559, 57.08472365561223683 ) ) ;
#38301=CARTESIAN_POINT ( 'NONE',  ( -12.18170072908086965, -10.17053062278287889, 64.32914326641392222 ) ) ;
#38302=CARTESIAN_POINT ( 'NONE',  ( -11.85162103594838001, -10.49015045520576983, 71.25420998615621215 ) ) ;
#38303=EDGE_CURVE ( 'NONE', #22272, #38392, #22115, .T. ) ;
#38304=CARTESIAN_POINT ( 'NONE',  ( -17.92193097897699872, -21.84160713959417421, 62.17535923543130139 ) ) ;
#38306=EDGE_CURVE ( 'NONE', #44794, #33937, #11555, .T. ) ;
#38308=AXIS2_PLACEMENT_3D ( 'NONE', #22987, #19269, #45873 ) ;
#38309=ORIENTED_EDGE ( 'NONE', *, *, #31301, .T. ) ;
#38310=EDGE_LOOP ( 'NONE', ( #42311, #36501, #29047, #15309, #6157 ) ) ;
#38312=EDGE_CURVE ( 'NONE', #29465, #40716, #5212, .T. ) ;
#38313=EDGE_CURVE ( 'NONE', #45950, #23554, #46283, .T. ) ;
#38314=CARTESIAN_POINT ( 'NONE',  ( -9.995623895585607599, -14.24219643007072023, 64.64449787557668969 ) ) ;
#38315=DIRECTION ( 'NONE',  ( -0.4749924142254751680, -0.8799898899579781109, -8.916637576350562172E-09 ) ) ;
#38317=CARTESIAN_POINT ( 'NONE',  ( -21.60699298862427398, -9.194826105172156261, 70.20302893975198799 ) ) ;
#38318=ORIENTED_EDGE ( 'NONE', *, *, #6611, .T. ) ;
#38321=CARTESIAN_POINT ( 'NONE',  ( -11.62344814847972252, -18.82242928093252843, 71.77866150141453261 ) ) ;
#38323=CARTESIAN_POINT ( 'NONE',  ( -24.46506320217640962, -17.24406362331221132, 72.99840605271779737 ) ) ;
#38324=( BOUNDED_CURVE ( )  B_SPLINE_CURVE ( 3, ( #20779, #42716, #32105, #12659 ),
 .UNSPECIFIED., .F., .F. ) 
 B_SPLINE_CURVE_WITH_KNOTS ( ( 4, 4 ),
 ( 0.9074455897393626236, 1.000000000000000000 ),
 .UNSPECIFIED. ) 
 CURVE ( )  GEOMETRIC_REPRESENTATION_ITEM ( )  RATIONAL_B_SPLINE_CURVE ( ( 0.6983129098261133816, 0.7760317562607157438, 0.8765941196520112833, 1.000000000000000000 ) ) 
 REPRESENTATION_ITEM ( '' )  );
#38332=CARTESIAN_POINT ( 'NONE',  ( -12.27604185553471616, -19.62628656662749549, 58.21210303282668264 ) ) ;
#38335=ORIENTED_EDGE ( 'NONE', *, *, #31932, .F. ) ;
#38336=( BOUNDED_SURFACE ( )  B_SPLINE_SURFACE ( 3, 1, ( 
 ( #4396, #14964 ),
 ( #27047, #26820 ),
 ( #8112, #19669 ),
 ( #23358, #30029 ),
 ( #45059, #23125 ),
 ( #19412, #4640 ),
 ( #15706, #30761 ) ),
 .UNSPECIFIED., .T., .F., .F. ) 
 B_SPLINE_SURFACE_WITH_KNOTS ( ( 4, 3, 4 ),
 ( 2, 2 ),
 ( 0.000000000000000000, 0.5000000000000000000, 1.000000000000000000 ),
 ( 0.000000000000000000, 1.000000000000000000 ),
 .UNSPECIFIED. ) 
 GEOMETRIC_REPRESENTATION_ITEM ( )  RATIONAL_B_SPLINE_SURFACE ( (
 ( 1.000000000000000000, 1.000000000000000000),
 ( 0.3333333333333335369, 0.3333333333333330373),
 ( 0.3333333333333335369, 0.3333333333333330373),
 ( 1.000000000000000000, 1.000000000000000000),
 ( 0.3333333333333333703, 0.3333333333333333703),
 ( 0.3333333333333333703, 0.3333333333333333703),
 ( 1.000000000000000000, 1.000000000000000000) ) ) 
 REPRESENTATION_ITEM ( '' )  SURFACE ( )  );
#38339=ORIENTED_EDGE ( 'NONE', *, *, #29114, .F. ) ;
#38341=CARTESIAN_POINT ( 'NONE',  ( -24.72725712452650981, -16.28144042551206638, 62.84974626185121593 ) ) ;
#38344=CARTESIAN_POINT ( 'NONE',  ( -10.43125871347677958, -13.91323993190135155, 57.59825034919892772 ) ) ;
#38345=CARTESIAN_POINT ( 'NONE',  ( -17.96757567997740423, -21.83837585814599080, 62.16976149166120535 ) ) ;
#38346=CARTESIAN_POINT ( 'NONE',  ( -14.28223569189418996, -8.054058993954978263, 67.36700916836338138 ) ) ;
#38347=ORIENTED_EDGE ( 'NONE', *, *, #9006, .T. ) ;
#38348=CARTESIAN_POINT ( 'NONE',  ( -15.39536932222403287, -19.92137602241599836, 54.07175714974879099 ) ) ;
#38351=CARTESIAN_POINT ( 'NONE',  ( -22.27817919856018136, -9.157513542003881568, 59.83675792137641736 ) ) ;
#38352=VERTEX_POINT ( 'NONE', #24343 ) ;
#38353=CARTESIAN_POINT ( 'NONE',  ( -11.46028008028683942, -18.56947564720590194, 61.56238700194530367 ) ) ;
#38355=CARTESIAN_POINT ( 'NONE',  ( -11.60247201135026884, -18.79965542285971836, 61.43277710409636683 ) ) ;
#38356=ORIENTED_EDGE ( 'NONE', *, *, #39480, .F. ) ;
#38358=B_SPLINE_CURVE_WITH_KNOTS ( 'NONE', 3,
 ( #8436, #27634, #19770, #34526, #23949, #46603, #34778, #5479, #4495, #8930 ),
 .UNSPECIFIED., .F., .F.,
 ( 4, 2, 2, 2, 4 ),
 ( 0.000000000000000000, 0.2500000000000000000, 0.5000000000000000000, 0.7500000000000000000, 1.000000000000000000 ),
 .UNSPECIFIED. ) ;
#38359=CARTESIAN_POINT ( 'NONE',  ( -22.85634334395279055, -10.39183557728184581, 66.65255357689962068 ) ) ;
#38360=LINE ( 'NONE', #23622, #23444 ) ;
#38364=CARTESIAN_POINT ( 'NONE',  ( -11.93195840498443516, -10.38844327383712773, 70.98365212470247343 ) ) ;
#38365=CARTESIAN_POINT ( 'NONE',  ( -23.26031998850344706, -18.67503058230525070, 69.57755490092647221 ) ) ;
#38366=CARTESIAN_POINT ( 'NONE',  ( -12.10131192688100299, -10.18592936015514816, 64.31442259820508411 ) ) ;
#38369=CARTESIAN_POINT ( 'NONE',  ( -22.44308142039503906, -9.846875392603276822, 70.16745681354213104 ) ) ;
#38371=EDGE_CURVE ( 'NONE', #6771, #8867, #37440, .T. ) ;
#38372=CARTESIAN_POINT ( 'NONE',  ( -14.54324430907851173, -21.67975036377454501, 58.42263788831355953 ) ) ;
#38374=CARTESIAN_POINT ( 'NONE',  ( -10.92506019527676209, -17.54181618899167105, 68.39162186085954431 ) ) ;
#38375=CARTESIAN_POINT ( 'NONE',  ( -12.47486999026313015, -19.83014042270297494, 64.87234644051179089 ) ) ;
#38378=VERTEX_POINT ( 'NONE', #27546 ) ;
#38379=AXIS2_PLACEMENT_3D ( 'NONE', #5848, #40531, #17400 ) ;
#38381=EDGE_CURVE ( 'NONE', #6140, #8644, #42183, .T. ) ;
#38382=ORIENTED_EDGE ( 'NONE', *, *, #12476, .T. ) ;
#38383=CARTESIAN_POINT ( 'NONE',  ( -24.47401588645412573, -14.84236399432835540, 59.39300237059229914 ) ) ;
#38385=CARTESIAN_POINT ( 'NONE',  ( -14.91602154273002689, -21.82451726398313241, 65.24563297375915738 ) ) ;
#38386=CARTESIAN_POINT ( 'NONE',  ( -11.40682184329331506, -18.48987001057684765, 65.04707367406611240 ) ) ;
#38388=VERTEX_POINT ( 'NONE', #35165 ) ;
#38390=CARTESIAN_POINT ( 'NONE',  ( -24.78816760170556677, -15.94238017617776215, 69.71962869939886787 ) ) ;
#38392=VERTEX_POINT ( 'NONE', #15961 ) ;
#38393=CARTESIAN_POINT ( 'NONE',  ( -12.83007325466668114, -20.09077588727113550, 72.10653676829758751 ) ) ;
#38395=ORIENTED_EDGE ( 'NONE', *, *, #3132, .T. ) ;
#38396=CARTESIAN_POINT ( 'NONE',  ( -12.41315173547891781, -9.850077678253004621, 57.38935532239157311 ) ) ;
#38397=ORIENTED_EDGE ( 'NONE', *, *, #12942, .T. ) ;
#38399=CARTESIAN_POINT ( 'NONE',  ( -10.61330293760801879, -12.98832031645814844, 67.88832347272310130 ) ) ;
#38401=CARTESIAN_POINT ( 'NONE',  ( -13.35550522631041837, -8.568183888810063209, 57.15463030501995689 ) ) ;
#38402=EDGE_CURVE ( 'NONE', #46585, #5353, #42824, .T. ) ;
#38403=CARTESIAN_POINT ( 'NONE',  ( -18.24929096724884658, -21.81104555038653103, 68.82986815895560540 ) ) ;
#38405=VECTOR ( 'NONE', #12320, 1000.000000000000227 ) ;
#38406=CARTESIAN_POINT ( 'NONE',  ( -16.50258162057404832, -20.23145840177225807, 53.49999999999995026 ) ) ;
#38408=CARTESIAN_POINT ( 'NONE',  ( -24.43375969181978036, -15.56263427672455713, 73.30303726254599894 ) ) ;
#38410=ORIENTED_EDGE ( 'NONE', *, *, #20048, .T. ) ;
#38411=CARTESIAN_POINT ( 'NONE',  ( -19.15013325158599855, -21.59352074159554746, 58.54124067949265253 ) ) ;
#38413=AXIS2_PLACEMENT_3D ( 'NONE', #20262, #35516, #31828 ) ;
#38414=CARTESIAN_POINT ( 'NONE',  ( -18.11396434131172128, -21.77512919714542150, 65.34532159443909904 ) ) ;
#38415=CARTESIAN_POINT ( 'NONE',  ( -19.98813035779708969, -21.37641423362171267, 72.55478737316022375 ) ) ;
#38416=B_SPLINE_CURVE_WITH_KNOTS ( 'NONE', 1,
 ( #37585, #26527 ),
 .UNSPECIFIED., .F., .F.,
 ( 2, 2 ),
 ( 0.000000000000000000, 1.000000000000000000 ),
 .UNSPECIFIED. ) ;
#38417=CARTESIAN_POINT ( 'NONE',  ( -18.38341875142146975, -21.74322078448643225, 69.10049320035381015 ) ) ;
#38418=CARTESIAN_POINT ( 'NONE',  ( -12.25434429315920859, -20.17366997322574562, 65.05170215947674706 ) ) ;
#38421=CARTESIAN_POINT ( 'NONE',  ( -18.46801905451614090, -7.836623195388690455, 74.12592262855558545 ) ) ;
#38423=ORIENTED_EDGE ( 'NONE', *, *, #2653, .F. ) ;
#38424=CARTESIAN_POINT ( 'NONE',  ( -10.37255316239921044, -15.11044245508572459, 57.71225695896244190 ) ) ;
#38425=CARTESIAN_POINT ( 'NONE',  ( -16.36834455927873222, -22.18410795223847387, 61.94063518049016182 ) ) ;
#38427=CARTESIAN_POINT ( 'NONE',  ( -20.75235147695052262, -8.143923935286606408, 63.41847357668724072 ) ) ;
#38428=FACE_OUTER_BOUND ( 'NONE', #20414, .T. ) ;
#38429=CARTESIAN_POINT ( 'NONE',  ( -14.22441598498101989, -8.081217260141077219, 67.44470407312981308 ) ) ;
#38430=CARTESIAN_POINT ( 'NONE',  ( -12.26157393735297596, -10.08170764524057894, 60.84452776435725951 ) ) ;
#38431=CARTESIAN_POINT ( 'NONE',  ( -13.98092790585787171, -8.714500222849059341, 74.27242791210171902 ) ) ;
#38434=EDGE_CURVE ( 'NONE', #25059, #27904, #18698, .T. ) ;
#38436=CARTESIAN_POINT ( 'NONE',  ( -15.50784783684063051, -8.076599273749138774, 74.07985659288991087 ) ) ;
#38437=CARTESIAN_POINT ( 'NONE',  ( -13.77834346862332637, -20.78674830809137575, 68.56698313520011823 ) ) ;
#38438=CARTESIAN_POINT ( 'NONE',  ( -17.46222794319647775, -7.759011850482251837, 67.03511641684839617 ) ) ;
#38440=ORIENTED_EDGE ( 'NONE', *, *, #16181, .F. ) ;
#38446=CARTESIAN_POINT ( 'NONE',  ( -17.56717618076180187, -7.360494862701306928, 63.73552352176282909 ) ) ;
#38447=EDGE_CURVE ( 'NONE', #24840, #6635, #12047, .T. ) ;
#38449=CARTESIAN_POINT ( 'NONE',  ( -24.10582418872880694, -12.72205642837049311, 69.77242970670894806 ) ) ;
#38450=EDGE_CURVE ( 'NONE', #10157, #7981, #28276, .T. ) ;
#38451=B_SPLINE_CURVE_WITH_KNOTS ( 'NONE', 1,
 ( #41514, #22823 ),
 .UNSPECIFIED., .F., .F.,
 ( 2, 2 ),
 ( 0.000000000000000000, 1.000000000000000000 ),
 .UNSPECIFIED. ) ;
#38457=EDGE_CURVE ( 'NONE', #35856, #19379, #22208, .T. ) ;
#38459=CARTESIAN_POINT ( 'NONE',  ( -13.89388974506275787, -21.36980381032900667, 72.11102993026078423 ) ) ;
#38461=CARTESIAN_POINT ( 'NONE',  ( -10.46492739217203471, -14.05366762209630949, 57.52113007005035428 ) ) ;
#38462=ORIENTED_EDGE ( 'NONE', *, *, #30311, .T. ) ;
#38463=LINE ( 'NONE', #38710, #46176 ) ;
#38464=FACE_OUTER_BOUND ( 'NONE', #1194, .T. ) ;
#38465=ORIENTED_EDGE ( 'NONE', *, *, #43150, .T. ) ;
#38466=CARTESIAN_POINT ( 'NONE',  ( -23.16117746674104438, -18.90708040007733359, 62.63934749780565880 ) ) ;
#38467=CARTESIAN_POINT ( 'NONE',  ( -22.53655473247544805, -20.22829521909097394, 65.88917159596024931 ) ) ;
#38468=CARTESIAN_POINT ( 'NONE',  ( -24.01409443880168126, -12.44853925549632301, 73.46898916292617798 ) ) ;
#38469=ORIENTED_EDGE ( 'NONE', *, *, #47945, .F. ) ;
#38470=CARTESIAN_POINT ( 'NONE',  ( -23.21283044961208830, -10.11939778159179859, 63.25681392212788268 ) ) ;
#38471=CARTESIAN_POINT ( 'NONE',  ( -17.85939470442713883, -21.79572004712530386, 58.63226791514592406 ) ) ;
#38472=( BOUNDED_CURVE ( )  B_SPLINE_CURVE ( 3, ( #40069, #20868, #29466, #21367 ),
 .UNSPECIFIED., .F., .F. ) 
 B_SPLINE_CURVE_WITH_KNOTS ( ( 4, 4 ),
 ( 0.000000000000000000, 0.4074455897393624570 ),
 .UNSPECIFIED. ) 
 CURVE ( )  GEOMETRIC_REPRESENTATION_ITEM ( )  RATIONAL_B_SPLINE_CURVE ( ( 1.000000000000000000, 0.4567392136813345216, 0.3561768502900312661, 0.6983129098260902889 ) ) 
 REPRESENTATION_ITEM ( '' )  );
#38473=CARTESIAN_POINT ( 'NONE',  ( -16.22585566360328357, -7.910893225427095388, 63.85938213801649255 ) ) ;
#38475=B_SPLINE_CURVE_WITH_KNOTS ( 'NONE', 1,
 ( #38623, #34924 ),
 .UNSPECIFIED., .F., .F.,
 ( 2, 2 ),
 ( 0.000000000000000000, 1.000000000000000000 ),
 .UNSPECIFIED. ) ;
#38476=CYLINDRICAL_SURFACE ( 'NONE', #2245, 7.500000000000001776 ) ;
#38477=CARTESIAN_POINT ( 'NONE',  ( -14.66630222544869078, -8.320656262913125545, 63.80450889863892172 ) ) ;
#38482=VERTEX_POINT ( 'NONE', #36599 ) ;
#38485=CARTESIAN_POINT ( 'NONE',  ( -10.46593773880539047, -17.47129530308245293, 64.72715759520706058 ) ) ;
#38488=CARTESIAN_POINT ( 'NONE',  ( -10.61606246679250631, -17.83465121431504841, 71.76729389568697570 ) ) ;
#38490=FACE_OUTER_BOUND ( 'NONE', #20481, .T. ) ;
#38491=EDGE_CURVE ( 'NONE', #48314, #24620, #11650, .T. ) ;
#38492=( BOUNDED_SURFACE ( )  B_SPLINE_SURFACE ( 3, 1, ( 
 ( #13130, #5541 ),
 ( #1586, #12668 ),
 ( #1833, #23771 ),
 ( #27693, #16595 ),
 ( #20061, #35065 ),
 ( #42723, #31636 ),
 ( #20563, #35556 ) ),
 .UNSPECIFIED., .T., .F., .F. ) 
 B_SPLINE_SURFACE_WITH_KNOTS ( ( 4, 3, 4 ),
 ( 2, 2 ),
 ( 0.000000000000000000, 0.5000000000000000000, 1.000000000000000000 ),
 ( 0.000000000000000000, 1.000000000000000000 ),
 .UNSPECIFIED. ) 
 GEOMETRIC_REPRESENTATION_ITEM ( )  RATIONAL_B_SPLINE_SURFACE ( (
 ( 1.000000000000000000, 1.000000000000000000),
 ( 0.3333333333333335369, 0.3333333333333330373),
 ( 0.3333333333333335369, 0.3333333333333330373),
 ( 1.000000000000000000, 1.000000000000000000),
 ( 0.3333333333333333703, 0.3333333333333333703),
 ( 0.3333333333333333703, 0.3333333333333333703),
 ( 1.000000000000000000, 1.000000000000000000) ) ) 
 REPRESENTATION_ITEM ( '' )  SURFACE ( )  );
#38495=PLANE ( 'NONE',  #346 ) ;
#38498=FACE_OUTER_BOUND ( 'NONE', #22184, .T. ) ;
#38499=CARTESIAN_POINT ( 'NONE',  ( -18.95312625172554633, -7.978243212125802231, 63.62192339619330994 ) ) ;
#38500=EDGE_CURVE ( 'NONE', #24292, #33660, #9812, .T. ) ;
#38504=CARTESIAN_POINT ( 'NONE',  ( -10.44216256679811217, -13.77595636612621988, 61.06254307272654813 ) ) ;
#38505=CARTESIAN_POINT ( 'NONE',  ( -21.72478623736860470, -8.725751437694626134, 70.30849399937490318 ) ) ;
#38506=CARTESIAN_POINT ( 'NONE',  ( -12.15399301493812878, -9.543295845094297292, 57.20440096431307353 ) ) ;
#38507=( BOUNDED_CURVE ( )  B_SPLINE_CURVE ( 3, ( #35449, #1734, #31767, #44548 ),
 .UNSPECIFIED., .F., .F. ) 
 B_SPLINE_CURVE_WITH_KNOTS ( ( 4, 4 ),
 ( 0.5000000000000000000, 0.9074455897393640669 ),
 .UNSPECIFIED. ) 
 CURVE ( )  GEOMETRIC_REPRESENTATION_ITEM ( )  RATIONAL_B_SPLINE_CURVE ( ( 0.9999999999999911182, 0.4567392136813318571, 0.3561768502900363731, 0.6983129098260949519 ) ) 
 REPRESENTATION_ITEM ( '' )  );
#38508=VERTEX_POINT ( 'NONE', #6351 ) ;
#38509=ORIENTED_EDGE ( 'NONE', *, *, #15889, .T. ) ;
#38511=CARTESIAN_POINT ( 'NONE',  ( -24.39763799706551950, -15.84669482609578317, 69.54779622430706354 ) ) ;
#38512=ADVANCED_FACE ( 'NONE', ( #20887 ), #10293, .T. ) ;
#38513=CARTESIAN_POINT ( 'NONE',  ( -10.45863924090583552, -14.11462608630872317, 61.21821294130609914 ) ) ;
#38514=ADVANCED_FACE ( 'NONE', ( #17164 ), #30609, .T. ) ;
#38515=EDGE_CURVE ( 'NONE', #15132, #6650, #33333, .T. ) ;
#38516=CARTESIAN_POINT ( 'NONE',  ( -17.79108452803360763, -21.84994637594637723, 58.69081321602850920 ) ) ;
#38518=AXIS2_PLACEMENT_3D ( 'NONE', #6858, #25094, #36875 ) ;
#38519=CARTESIAN_POINT ( 'NONE',  ( -20.25445156252866497, -7.916983464207429932, 73.90751836168473687 ) ) ;
#38521=DIRECTION ( 'NONE',  ( -0.3478314405900309603, -0.9375570856950864451, 9.567072274253696421E-17 ) ) ;
#38522=ADVANCED_FACE ( 'NONE', ( #29726 ), #37578, .T. ) ;
#38523=ORIENTED_EDGE ( 'NONE', *, *, #32601, .F. ) ;
#38524=CARTESIAN_POINT ( 'NONE',  ( -21.19335713336021243, -20.70964345786463312, 72.71373614481359482 ) ) ;
#38525=CARTESIAN_POINT ( 'NONE',  ( -24.16575376147897458, -12.74704232990201547, 69.77243002240838621 ) ) ;
#38526=ORIENTED_EDGE ( 'NONE', *, *, #18122, .F. ) ;
#38527=CYLINDRICAL_SURFACE ( 'NONE', #46530, 0.1500000000000080158 ) ;
#38528=CARTESIAN_POINT ( 'NONE',  ( -10.48067351556794158, -16.03044098841782628, 68.27767830705533925 ) ) ;
#38530=DIRECTION ( 'NONE',  ( -8.329294163758554984E-07, 2.487164605953353708E-06, -0.9999999999965601960 ) ) ;
#38531=CARTESIAN_POINT ( 'NONE',  ( -10.00830686992707896, -15.52368892135347878, 57.74509703396581983 ) ) ;
#38532=B_SPLINE_CURVE_WITH_KNOTS ( 'NONE', 3,
 ( #41876, #41135, #33979, #11580, #14747, #27088, #275, #22671, #3964, #15254 ),
 .UNSPECIFIED., .F., .F.,
 ( 4, 2, 2, 2, 4 ),
 ( 0.000000000000000000, 0.2500000000000000000, 0.5000000000000000000, 0.7500000000000000000, 1.000000000000000000 ),
 .UNSPECIFIED. ) ;
#38533=CARTESIAN_POINT ( 'NONE',  ( -13.35819042472069107, -21.05197888995676436, 61.70141705377209007 ) ) ;
#38536=CARTESIAN_POINT ( 'NONE',  ( -22.11925914797909343, -9.024813657292067859, 63.30658454184609241 ) ) ;
#38537=CARTESIAN_POINT ( 'NONE',  ( -20.82598581164736018, -21.43720942579135524, 58.75201007894592919 ) ) ;
#38539=FACE_BOUND ( 'NONE', #46645, .T. ) ;
#38544=ORIENTED_EDGE ( 'NONE', *, *, #39795, .F. ) ;
#38545=CARTESIAN_POINT ( 'NONE',  ( -24.47401588439613818, -14.84236418521736312, 59.54300237059217693 ) ) ;
#38546=VERTEX_POINT ( 'NONE', #11496 ) ;
#38548=CARTESIAN_POINT ( 'NONE',  ( -16.79748725893476546, -22.23297595151960238, 68.83414125832270258 ) ) ;
#38550=ORIENTED_EDGE ( 'NONE', *, *, #14225, .T. ) ;
#38551=CARTESIAN_POINT ( 'NONE',  ( -24.35389707626741185, -16.10709931453380861, 62.87856533165624029 ) ) ;
#38552=FACE_BOUND ( 'NONE', #30865, .T. ) ;
#38553=ORIENTED_EDGE ( 'NONE', *, *, #45348, .T. ) ;
#38556=VECTOR ( 'NONE', #37548, 1000.000000000000000 ) ;
#38557=CARTESIAN_POINT ( 'NONE',  ( -18.12717186014929283, -21.82707771419581633, 61.76047256604253732 ) ) ;
#38558=SURFACE_STYLE_USAGE ( .BOTH. , #17047 ) ;
#38559=LINE ( 'NONE', #23081, #27153 ) ;
#38560=CARTESIAN_POINT ( 'NONE',  ( -14.44809130310161471, -8.473323905341505480, 67.25975083863336579 ) ) ;
#38561=CARTESIAN_POINT ( 'NONE',  ( -10.29385316490627211, -12.64970523595484231, 64.38340807599202265 ) ) ;
#38564=ORIENTED_EDGE ( 'NONE', *, *, #23563, .T. ) ;
#38568=CARTESIAN_POINT ( 'NONE',  ( -10.38078070663892483, -14.50222156296672971, 67.85800126083267969 ) ) ;
#38570=CARTESIAN_POINT ( 'NONE',  ( -21.62013850256694525, -9.204234574478094899, 70.24205721712547756 ) ) ;
#38573=B_SPLINE_CURVE_WITH_KNOTS ( 'NONE', 3,
 ( #11610, #27357, #11864, #42390, #23192, #8659, #34008, #37700, #45123, #304 ),
 .UNSPECIFIED., .F., .F.,
 ( 4, 2, 2, 2, 4 ),
 ( 0.000000000000000000, 0.2500000000000000000, 0.5000000000000000000, 0.7500000000000000000, 1.000000000000000000 ),
 .UNSPECIFIED. ) ;
#38574=B_SPLINE_CURVE_WITH_KNOTS ( 'NONE', 3,
 ( #33365, #47934, #7062, #48409, #29221, #41033, #32434, #7315, #22315, #25047 ),
 .UNSPECIFIED., .F., .F.,
 ( 4, 2, 2, 2, 4 ),
 ( 0.000000000000000000, 0.2500000000000000000, 0.5000000000000000000, 0.7500000000000000000, 1.000000000000000000 ),
 .UNSPECIFIED. ) ;
#38576=ADVANCED_FACE ( 'NONE', ( #37333 ), #29006, .T. ) ;
#38577=CARTESIAN_POINT ( 'NONE',  ( -13.60238606012557483, -8.884930320952351579, 56.96967755506135234 ) ) ;
#38578=CARTESIAN_POINT ( 'NONE',  ( -10.99655737938916289, -18.57624151290433900, 57.99209991576458378 ) ) ;
#38580=CARTESIAN_POINT ( 'NONE',  ( -24.84793640206982701, -14.18443463346696909, 69.83770693398628282 ) ) ;
#38581=( BOUNDED_CURVE ( )  B_SPLINE_CURVE ( 3, ( #39526, #5569, #9743, #21056 ),
 .UNSPECIFIED., .F., .F. ) 
 B_SPLINE_CURVE_WITH_KNOTS ( ( 4, 4 ),
 ( 4.712388980384689674, 4.921828490624008623 ),
 .UNSPECIFIED. ) 
 CURVE ( )  GEOMETRIC_REPRESENTATION_ITEM ( )  RATIONAL_B_SPLINE_CURVE ( ( 1.000000000000000000, 0.9963479302455156006, 0.9963479302455156006, 1.000000000000000000 ) ) 
 REPRESENTATION_ITEM ( '' )  );
#38582=EDGE_CURVE ( 'NONE', #24972, #46199, #11014, .T. ) ;
#38583=VERTEX_POINT ( 'NONE', #26520 ) ;
#38587=CARTESIAN_POINT ( 'NONE',  ( -12.96596534320165972, -9.347742485070138940, 70.84925352874383009 ) ) ;
#38590=DIRECTION ( 'NONE',  ( 0.7248509490090241369, -0.6889057277456160922, 1.880377065355303572E-09 ) ) ;
#38591=ADVANCED_FACE ( 'NONE', ( #18137 ), #33152, .T. ) ;
#38592=CARTESIAN_POINT ( 'NONE',  ( -22.61657813405388495, -16.66287387207217563, 53.88362224778187226 ) ) ;
#38593=CARTESIAN_POINT ( 'NONE',  ( -11.38992724816770163, -18.36045063709194025, 61.46637994071404165 ) ) ;
#38594=ORIENTED_EDGE ( 'NONE', *, *, #44869, .F. ) ;
#38595=CARTESIAN_POINT ( 'NONE',  ( -15.96455646543153151, -7.503521033077919178, 63.86285157243441546 ) ) ;
#38596=VECTOR ( 'NONE', #39552, 1000.000000000000000 ) ;
#38599=CARTESIAN_POINT ( 'NONE',  ( -19.16507141099300782, -7.565355480308949332, 63.60806100508323624 ) ) ;
#38601=CARTESIAN_POINT ( 'NONE',  ( -24.74044779172452024, -16.21442189768792375, 62.63682720862403386 ) ) ;
#38602=VERTEX_POINT ( 'NONE', #29480 ) ;
#38605=CARTESIAN_POINT ( 'NONE',  ( -23.80139577239251736, -11.92276195191408839, 59.78235729430349465 ) ) ;
#38607=ORIENTED_EDGE ( 'NONE', *, *, #2829, .T. ) ;
#38608=DIRECTION ( 'NONE',  ( 0.5562740912439652075, 0.8309988781043535777, 7.851267780903552829E-08 ) ) ;
#38611=CARTESIAN_POINT ( 'NONE',  ( -15.17234920820390975, -21.91077519426012898, 68.77581698242099151 ) ) ;
#38613=CARTESIAN_POINT ( 'NONE',  ( -23.43037763135286156, -19.21690358092465800, 62.54745201246257835 ) ) ;
#38615=CARTESIAN_POINT ( 'NONE',  ( -10.61994057853096862, -11.77494598563924733, 74.66501929302266660 ) ) ;
#38618=ORIENTED_EDGE ( 'NONE', *, *, #6779, .F. ) ;
#38619=CARTESIAN_POINT ( 'NONE',  ( -10.47788155843228708, -15.67630068988790448, 61.33789014617833857 ) ) ;
#38621=CARTESIAN_POINT ( 'NONE',  ( -10.42558329592169386, -14.65956671939337319, 71.32782690272046011 ) ) ;
#38623=CARTESIAN_POINT ( 'NONE',  ( -23.80338573481879294, -11.80731802715296297, 59.76763678108634537 ) ) ;
#38624=CARTESIAN_POINT ( 'NONE',  ( -12.26902364965855519, -19.54473725125994221, 57.92682373989410394 ) ) ;
#38625=CARTESIAN_POINT ( 'NONE',  ( -19.78800712013224583, -21.87439760486632778, 65.62519571951479236 ) ) ;
#38628=VECTOR ( 'NONE', #34703, 1000.000000000000000 ) ;
#38629=CARTESIAN_POINT ( 'NONE',  ( -12.40538999107997498, -20.31523868419091272, 68.52152871938794476 ) ) ;
#38631=CARTESIAN_POINT ( 'NONE',  ( -11.64235247690698749, -18.84330696305777408, 68.51689631558762983 ) ) ;
#38632=CARTESIAN_POINT ( 'NONE',  ( -19.55442184481404766, -21.52995072282663358, 65.47958309245051112 ) ) ;
#38633=CARTESIAN_POINT ( 'NONE',  ( -17.79084047922378531, -7.768752242298102573, 60.23060768310389790 ) ) ;
#38634=( BOUNDED_SURFACE ( )  B_SPLINE_SURFACE ( 3, 1, ( 
 ( #1797, #35996 ),
 ( #10155, #39705 ),
 ( #28858, #21241 ),
 ( #39467, #32329 ),
 ( #47354, #14052 ),
 ( #28139, #47099 ),
 ( #25177, #2750 ) ),
 .UNSPECIFIED., .T., .F., .F. ) 
 B_SPLINE_SURFACE_WITH_KNOTS ( ( 4, 3, 4 ),
 ( 2, 2 ),
 ( 0.000000000000000000, 0.5000000000000000000, 1.000000000000000000 ),
 ( 0.000000000000000000, 1.000000000000000000 ),
 .UNSPECIFIED. ) 
 GEOMETRIC_REPRESENTATION_ITEM ( )  RATIONAL_B_SPLINE_SURFACE ( (
 ( 1.000000000000000000, 1.000000000000000000),
 ( 0.3333333333333335369, 0.3333333333333330373),
 ( 0.3333333333333335369, 0.3333333333333330373),
 ( 1.000000000000000000, 1.000000000000000000),
 ( 0.3333333333333333703, 0.3333333333333333703),
 ( 0.3333333333333333703, 0.3333333333333333703),
 ( 1.000000000000000000, 1.000000000000000000) ) ) 
 REPRESENTATION_ITEM ( '' )  SURFACE ( )  );
#38635=VECTOR ( 'NONE', #18463, 1000.000000000000000 ) ;
#38636=ORIENTED_EDGE ( 'NONE', *, *, #14617, .T. ) ;
#38640=CARTESIAN_POINT ( 'NONE',  ( -23.63568631841604883, -11.45792465866591137, 73.50626392806049125 ) ) ;
#38641=DIRECTION ( 'NONE',  ( 3.892913445306193086E-06, 4.639959643356220421E-06, 0.9999999999816580054 ) ) ;
#38642=CARTESIAN_POINT ( 'NONE',  ( -24.44253391677669285, -17.31023895159264470, 73.06991310009190954 ) ) ;
#38643=ORIENTED_EDGE ( 'NONE', *, *, #12314, .T. ) ;
#38644=( BOUNDED_CURVE ( )  B_SPLINE_CURVE ( 3, ( #43893, #21705, #48049, #21948 ),
 .UNSPECIFIED., .F., .F. ) 
 B_SPLINE_CURVE_WITH_KNOTS ( ( 4, 4 ),
 ( 1.570796326794896780, 1.780235837034217283 ),
 .UNSPECIFIED. ) 
 CURVE ( )  GEOMETRIC_REPRESENTATION_ITEM ( )  RATIONAL_B_SPLINE_CURVE ( ( 1.000000000000000000, 0.9963479302455154896, 0.9963479302455154896, 1.000000000000000000 ) ) 
 REPRESENTATION_ITEM ( '' )  );
#38645=CARTESIAN_POINT ( 'NONE',  ( -24.47853618617655158, -14.58602005854247174, 69.79708117814310242 ) ) ;
#38648=VERTEX_POINT ( 'NONE', #16636 ) ;
#38649=B_SPLINE_CURVE_WITH_KNOTS ( 'NONE', 3,
 ( #45450, #626, #12193, #45214, #27213, #42238, #8501, #11459, #23530, #35562 ),
 .UNSPECIFIED., .F., .F.,
 ( 4, 2, 2, 2, 4 ),
 ( 0.1272669073658180550, 0.2522669073463211786, 0.3772669073268243300, 0.5022669073073273704, 0.6272669072878305219 ),
 .UNSPECIFIED. ) ;
#38651=CARTESIAN_POINT ( 'NONE',  ( -22.17450840124994826, -19.95071447184853497, 65.70421734751553799 ) ) ;
#38653=CARTESIAN_POINT ( 'NONE',  ( -10.48085305489969521, -13.91959585118948617, 57.74825035244229809 ) ) ;
#38654=EDGE_CURVE ( 'NONE', #10403, #20439, #21076, .T. ) ;
#38655=ORIENTED_EDGE ( 'NONE', *, *, #18209, .F. ) ;
#38656=CARTESIAN_POINT ( 'NONE',  ( -19.46797834413568040, -22.79580085574647441, 53.49999999999995026 ) ) ;
#38658=CARTESIAN_POINT ( 'NONE',  ( -24.08907074505709645, -11.48026357735065872, 63.13713704106291402 ) ) ;
#38660=CARTESIAN_POINT ( 'NONE',  ( -12.69763806180496601, -20.04058448603118592, 68.62185382311069759 ) ) ;
#38661=EDGE_CURVE ( 'NONE', #18548, #4870, #38067, .T. ) ;
#38662=EDGE_CURVE ( 'NONE', #42753, #14825, #25843, .T. ) ;
#38666=CARTESIAN_POINT ( 'NONE',  ( -23.82448057917968143, -18.75384986479144800, 54.02312124697527906 ) ) ;
#38668=ORIENTED_EDGE ( 'NONE', *, *, #21062, .F. ) ;
#38669=CARTESIAN_POINT ( 'NONE',  ( -16.22922801436599727, -7.911814901714118164, 60.20028431044633521 ) ) ;
#38671=FACE_OUTER_BOUND ( 'NONE', #40596, .T. ) ;
#38672=CARTESIAN_POINT ( 'NONE',  ( -20.56585955126247001, -8.054015989788005925, 66.88829919087760345 ) ) ;
#38673=CARTESIAN_POINT ( 'NONE',  ( -12.55411140858086760, -19.90724249994213935, 65.15202838036978505 ) ) ;
#38676=CARTESIAN_POINT ( 'NONE',  ( -18.46801905451614090, -7.836623195388690455, 74.12592262855558545 ) ) ;
#38677=CARTESIAN_POINT ( 'NONE',  ( -22.09234465700630778, -20.09219189623108548, 62.23439162498055310 ) ) ;
#38678=EDGE_LOOP ( 'NONE', ( #32120, #15326 ) ) ;
#38679=CARTESIAN_POINT ( 'NONE',  ( -10.00761937521931522, -15.51608998476985946, 57.75288115419267854 ) ) ;
#38680=AXIS2_PLACEMENT_3D ( 'NONE', #45148, #31078, #81 ) ;
#38681=FACE_OUTER_BOUND ( 'NONE', #14067, .T. ) ;
#38683=PLANE ( 'NONE',  #43105 ) ;
#38684=CARTESIAN_POINT ( 'NONE',  ( -24.38391064099431915, -14.06024038319858960, 73.42271507915008044 ) ) ;
#38686=CARTESIAN_POINT ( 'NONE',  ( -23.66263630406368534, -11.51900531544784911, 70.30699535439772774 ) ) ;
#38687=VERTEX_POINT ( 'NONE', #42759 ) ;
#38689=EDGE_CURVE ( 'NONE', #34717, #47795, #18080, .T. ) ;
#38690=CARTESIAN_POINT ( 'NONE',  ( -19.19444523719849371, -21.63346107625851644, 58.53067200039218676 ) ) ;
#38691=CARTESIAN_POINT ( 'NONE',  ( -23.21283114448125673, -10.11939864774917908, 63.25681283445349123 ) ) ;
#38692=CARTESIAN_POINT ( 'NONE',  ( -19.36683724782897897, -21.58655468785150688, 62.00975759738177118 ) ) ;
#38695=ORIENTED_EDGE ( 'NONE', *, *, #27947, .F. ) ;
#38697=VERTEX_POINT ( 'NONE', #38304 ) ;
#38698=EDGE_CURVE ( 'NONE', #34217, #31055, #16342, .T. ) ;
#38699=CARTESIAN_POINT ( 'NONE',  ( -11.99234491386792634, -9.710313501827961602, 60.75929282996435887 ) ) ;
#38702=DIRECTION ( 'NONE',  ( -0.3739781583979218671, -0.9274375111247652459, -6.296758467538797382E-09 ) ) ;
#38704=DIRECTION ( 'NONE',  ( 0.6827297667453423591, 0.7306709694519485376, 5.176517822219623819E-09 ) ) ;
#38705=PLANE ( 'NONE',  #45368 ) ;
#38706=ORIENTED_EDGE ( 'NONE', *, *, #38018, .F. ) ;
#38707=FACE_OUTER_BOUND ( 'NONE', #43592, .T. ) ;
#38708=DIRECTION ( 'NONE',  ( 8.719004453613161891E-07, -8.513143893533137515E-07, 0.9999999999992574828 ) ) ;
#38709=ORIENTED_EDGE ( 'NONE', *, *, #16898, .F. ) ;
#38710=CARTESIAN_POINT ( 'NONE',  ( -11.98246295270348405, -15.60836430055780433, 53.49899999999994549 ) ) ;
#38711=CARTESIAN_POINT ( 'NONE',  ( -10.12038064680082172, -13.33925369334275324, 74.81671120912561435 ) ) ;
#38712=VERTEX_POINT ( 'NONE', #4597 ) ;
#38713=CARTESIAN_POINT ( 'NONE',  ( -23.50857174774670355, -19.10953103619692328, 62.46751498843644157 ) ) ;
#38714=FACE_OUTER_BOUND ( 'NONE', #38973, .T. ) ;
#38716=ORIENTED_EDGE ( 'NONE', *, *, #16016, .F. ) ;
#38717=CARTESIAN_POINT ( 'NONE',  ( -10.37599212182869124, -14.63324797960940593, 71.34254748307667171 ) ) ;
#38719=ADVANCED_FACE ( 'NONE', ( #38811 ), #17055, .T. ) ;
#38720=CARTESIAN_POINT ( 'NONE',  ( -22.17130319910813085, -20.55096425825585982, 58.87947600183965591 ) ) ;
#38721=CARTESIAN_POINT ( 'NONE',  ( -11.54683828446007254, -10.23068304809853935, 71.12926454345553395 ) ) ;
#38725=CARTESIAN_POINT ( 'NONE',  ( -17.59211730330735435, -7.811223398082945302, 63.85057029380297422 ) ) ;
#38727=EDGE_CURVE ( 'NONE', #12198, #26904, #6330, .T. ) ;
#38731=ORIENTED_EDGE ( 'NONE', *, *, #12231, .T. ) ;
#38734=CARTESIAN_POINT ( 'NONE',  ( -10.99586697244644640, -11.04334986774487781, 60.86381167495338929 ) ) ;
#38737=CARTESIAN_POINT ( 'NONE',  ( -14.47836531470152188, -7.966228403338186936, 64.04624744032878425 ) ) ;
#38738=CARTESIAN_POINT ( 'NONE',  ( -19.80301194551662647, -21.44571530912113744, 68.93482476707502826 ) ) ;
#38739=EDGE_CURVE ( 'NONE', #36187, #24622, #15119, .T. ) ;
#38741=CARTESIAN_POINT ( 'NONE',  ( -18.55957040452605611, -7.446158924837727788, 74.02559677774105751 ) ) ;
#38744=DIRECTION ( 'NONE',  ( 2.209513395486314832E-06, -7.769005149436063369E-07, -0.9999999999972571940 ) ) ;
#38745=B_SPLINE_CURVE_WITH_KNOTS ( 'NONE', 3,
 ( #24591, #39585, #5863, #28016, #1920, #20880, #35158, #43779, #46744, #46973 ),
 .UNSPECIFIED., .F., .F.,
 ( 4, 2, 2, 2, 4 ),
 ( 0.000000000000000000, 0.2500000000000000000, 0.5000000000000000000, 0.7500000000000000000, 1.000000000000000000 ),
 .UNSPECIFIED. ) ;
#38746=CARTESIAN_POINT ( 'NONE',  ( -10.09291391017891115, -16.13494330055838333, 68.16263215882007387 ) ) ;
#38747=EDGE_CURVE ( 'NONE', #39328, #18995, #43940, .T. ) ;
#38749=CARTESIAN_POINT ( 'NONE',  ( -13.27770768808250956, -9.107454094634595876, 63.90946529206384241 ) ) ;
#38750=DIRECTION ( 'NONE',  ( -0.8201047403141394909, 0.5722134347551369737, 7.883065731424289661E-08 ) ) ;
#38751=CARTESIAN_POINT ( 'NONE',  ( -24.56285135521319773, -12.67774455940246803, 69.93389527165277286 ) ) ;
#38754=ORIENTED_EDGE ( 'NONE', *, *, #16884, .T. ) ;
#38755=ORIENTED_EDGE ( 'NONE', *, *, #31363, .T. ) ;
#38757=CARTESIAN_POINT ( 'NONE',  ( -19.92736644894527842, -21.34646251977703102, 72.40478735915066011 ) ) ;
#38759=B_SPLINE_CURVE_WITH_KNOTS ( 'NONE', 3,
 ( #38780, #46426, #4817, #11714, #41999, #26742, #41761, #34840, #1340, #30685 ),
 .UNSPECIFIED., .F., .F.,
 ( 4, 2, 2, 2, 4 ),
 ( 0.6272669072877610219, 0.7522669073072782986, 0.8772669073267956863, 1.002266907346313074, 1.127266907365830351 ),
 .UNSPECIFIED. ) ;
#38760=CARTESIAN_POINT ( 'NONE',  ( -17.46222794319647775, -7.759011850482251837, 67.03511641684839617 ) ) ;
#38761=CARTESIAN_POINT ( 'NONE',  ( -17.52077441883401576, -21.86154573861348283, 58.82041992746825798 ) ) ;
#38762=CARTESIAN_POINT ( 'NONE',  ( -20.90753508896134960, -8.676468725517494818, 60.25614029449676678 ) ) ;
#38763=CARTESIAN_POINT ( 'NONE',  ( -14.13242279744181751, -8.574497162196566435, 74.21426705364891063 ) ) ;
#38764=CARTESIAN_POINT ( 'NONE',  ( -23.91467064781584995, -17.58181910956628613, 69.55772506159280510 ) ) ;
#38768=CARTESIAN_POINT ( 'NONE',  ( -21.63336539757928634, -9.153348366551478321, 66.94677872351418557 ) ) ;
#38769=CARTESIAN_POINT ( 'NONE',  ( -16.16828274592561243, -21.75012765010984239, 61.84748396296113526 ) ) ;
#38771=CARTESIAN_POINT ( 'NONE',  ( -13.35101845555447042, -21.04725863074550674, 61.62307991559396214 ) ) ;
#38772=CARTESIAN_POINT ( 'NONE',  ( -23.08487763607990928, -19.01185175973044039, 62.36879011380454330 ) ) ;
#38773=ORIENTED_EDGE ( 'NONE', *, *, #45555, .T. ) ;
#38776=CARTESIAN_POINT ( 'NONE',  ( -11.98712258119491203, -10.32100680013864569, 67.79337086303625881 ) ) ;
#38777=B_SPLINE_CURVE_WITH_KNOTS ( 'NONE', 3,
 ( #44614, #33251, #8169, #19235, #30339, #10870, #11122, #45347, #38172, #11601 ),
 .UNSPECIFIED., .F., .F.,
 ( 4, 2, 2, 2, 4 ),
 ( 0.6272669072783292332, 0.7522669073002161699, 0.8772669073221032177, 1.002266907343990265, 1.127266907365877202 ),
 .UNSPECIFIED. ) ;
#38778=( BOUNDED_CURVE ( )  B_SPLINE_CURVE ( 3, ( #16963, #28324, #5680, #36165 ),
 .UNSPECIFIED., .F., .F. ) 
 B_SPLINE_CURVE_WITH_KNOTS ( ( 4, 4 ),
 ( 0.000000000000000000, 0.4074455897393680637 ),
 .UNSPECIFIED. ) 
 CURVE ( )  GEOMETRIC_REPRESENTATION_ITEM ( )  RATIONAL_B_SPLINE_CURVE ( ( 1.000000000000000000, 0.4567392136813319126, 0.3561768502900302669, 0.6983129098260951739 ) ) 
 REPRESENTATION_ITEM ( '' )  );
#38780=CARTESIAN_POINT ( 'NONE',  ( -24.48810908846319734, -17.17637088580320537, 73.06831457992643664 ) ) ;
#38781=ORIENTED_EDGE ( 'NONE', *, *, #15368, .T. ) ;
#38782=FACE_OUTER_BOUND ( 'NONE', #34114, .T. ) ;
#38783=DIRECTION ( 'NONE',  ( 2.696738943264045022E-06, 1.002714486673431828E-05, 0.9999999999460920108 ) ) ;
#38784=( BOUNDED_CURVE ( )  B_SPLINE_CURVE ( 3, ( #23034, #38019, #34817, #42217 ),
 .UNSPECIFIED., .F., .F. ) 
 B_SPLINE_CURVE_WITH_KNOTS ( ( 4, 4 ),
 ( 0.000000000000000000, 0.4074455897393673975 ),
 .UNSPECIFIED. ) 
 CURVE ( )  GEOMETRIC_REPRESENTATION_ITEM ( )  RATIONAL_B_SPLINE_CURVE ( ( 1.000000000000000000, 0.4567392136813303027, 0.3561768502900297118, 0.6983129098260982826 ) ) 
 REPRESENTATION_ITEM ( '' )  );
#38785=CARTESIAN_POINT ( 'NONE',  ( -10.88594323032443967, -11.23743189042336788, 64.28735501138554298 ) ) ;
#38786=DIRECTION ( 'NONE',  ( -0.5729733056696844073, 0.8195740302071246042, 7.403245352187747277E-08 ) ) ;
#38788=CARTESIAN_POINT ( 'NONE',  ( -10.78031428196279329, -11.32923628920978310, 54.27966884056655061 ) ) ;
#38789=CARTESIAN_POINT ( 'NONE',  ( -17.36015951656348832, -7.359395083792595216, 67.20534920880687935 ) ) ;
#38791=EDGE_CURVE ( 'NONE', #31554, #29013, #27140, .T. ) ;
#38793=ORIENTED_EDGE ( 'NONE', *, *, #12337, .F. ) ;
#38795=EDGE_CURVE ( 'NONE', #44533, #5874, #31631, .T. ) ;
#38796=ORIENTED_EDGE ( 'NONE', *, *, #18486, .F. ) ;
#38797=CARTESIAN_POINT ( 'NONE',  ( -11.15030165360094117, -11.70430893863018262, 67.84537925602023734 ) ) ;
#38798=CARTESIAN_POINT ( 'NONE',  ( -13.21199625013959178, -9.217751934154737370, 67.66326273853178463 ) ) ;
#38799=VERTEX_POINT ( 'NONE', #39295 ) ;
#38800=LINE ( 'NONE', #5317, #13773 ) ;
#38801=( BOUNDED_CURVE ( )  B_SPLINE_CURVE ( 3, ( #26426, #42429, #34784, #45162 ),
 .UNSPECIFIED., .F., .F. ) 
 B_SPLINE_CURVE_WITH_KNOTS ( ( 4, 4 ),
 ( 0.9074455897393678416, 1.000000000000000000 ),
 .UNSPECIFIED. ) 
 CURVE ( )  GEOMETRIC_REPRESENTATION_ITEM ( )  RATIONAL_B_SPLINE_CURVE ( ( 0.6983129098261183776, 0.7760317562607200736, 0.8765941196520139478, 1.000000000000000000 ) ) 
 REPRESENTATION_ITEM ( '' )  );
#38802=FACE_BOUND ( 'NONE', #4900, .T. ) ;
#38803=ORIENTED_EDGE ( 'NONE', *, *, #21210, .F. ) ;
#38805=VERTEX_POINT ( 'NONE', #32158 ) ;
#38806=CARTESIAN_POINT ( 'NONE',  ( -17.98424483515344718, -22.23819686138322638, 61.91890007431585019 ) ) ;
#38808=CARTESIAN_POINT ( 'NONE',  ( -13.44265069500541898, -7.318461398084003200, 54.49999999999995026 ) ) ;
#38810=CARTESIAN_POINT ( 'NONE',  ( -14.48363557501458132, -8.456628546212041186, 67.55975083097567335 ) ) ;
#38811=FACE_OUTER_BOUND ( 'NONE', #37839, .T. ) ;
#38813=EDGE_LOOP ( 'NONE', ( #902, #36415, #36921, #12125, #6190 ) ) ;
#38814=ORIENTED_EDGE ( 'NONE', *, *, #38998, .F. ) ;
#38817=CARTESIAN_POINT ( 'NONE',  ( -17.70776835051902864, -22.25388969026799657, 58.52057945155585372 ) ) ;
#38818=DIRECTION ( 'NONE',  ( 4.116680954457742276E-07, 3.835121109574216710E-07, 0.9999999999998415712 ) ) ;
#38819=CARTESIAN_POINT ( 'NONE',  ( -21.53009296270428052, -9.139787401108153020, 70.43132584625033132 ) ) ;
#38823=LINE ( 'NONE', #39549, #6023 ) ;
#38824=CARTESIAN_POINT ( 'NONE',  ( -19.06702665442182365, -7.953160677532423506, 63.72529421800381044 ) ) ;
#38826=FACE_OUTER_BOUND ( 'NONE', #30702, .T. ) ;
#38827=ADVANCED_FACE ( 'NONE', ( #6957 ), #32176, .T. ) ;
#38829=CARTESIAN_POINT ( 'NONE',  ( -18.53556552080321751, -22.17591605216722428, 72.40015545304112266 ) ) ;
#38830=CARTESIAN_POINT ( 'NONE',  ( -21.52726260838264949, -9.076274878514674072, 70.13132538915753855 ) ) ;
#38831=CARTESIAN_POINT ( 'NONE',  ( -22.07021550121272568, -8.985394110722673133, 63.29815443424653409 ) ) ;
#38834=CARTESIAN_POINT ( 'NONE',  ( -16.19814381282456495, -21.75179583453235210, 58.58585572026735377 ) ) ;
#38835=CARTESIAN_POINT ( 'NONE',  ( -17.33262245845742910, -7.759502110702281463, 67.30567542699309058 ) ) ;
#38836=CARTESIAN_POINT ( 'NONE',  ( -20.11638923031699022, -7.862561834400525029, 73.84283875516227624 ) ) ;
#38837=ORIENTED_EDGE ( 'NONE', *, *, #29269, .F. ) ;
#38838=DIRECTION ( 'NONE',  ( -7.652304188939491606E-06, -2.165757507092278517E-06, -0.9999999999683759633 ) ) ;
#38840=CARTESIAN_POINT ( 'NONE',  ( -9.974591638057805909, -14.71890188683600087, 71.43444401210939532 ) ) ;
#38842=VERTEX_POINT ( 'NONE', #23438 ) ;
#38844=CARTESIAN_POINT ( 'NONE',  ( -24.64686309199095859, -12.98257247058134212, 62.97117624809372671 ) ) ;
#38849=CARTESIAN_POINT ( 'NONE',  ( -23.71561414012218094, -17.99693426085591952, 59.41867086777731544 ) ) ;
#38851=CARTESIAN_POINT ( 'NONE',  ( -20.75714322117456945, -21.47287265741918461, 58.83130466214971221 ) ) ;
#38853=CARTESIAN_POINT ( 'NONE',  ( -17.77921064978749044, -22.25082400685520057, 58.59048811498988840 ) ) ;
#38854=ORIENTED_EDGE ( 'NONE', *, *, #33815, .F. ) ;
#38855=B_SPLINE_CURVE_WITH_KNOTS ( 'NONE', 1,
 ( #1653, #46230 ),
 .UNSPECIFIED., .F., .F.,
 ( 2, 2 ),
 ( 0.000000000000000000, 1.000000000000000000 ),
 .UNSPECIFIED. ) ;
#38856=CARTESIAN_POINT ( 'NONE',  ( -15.82103535061131261, -7.533639916251397395, 67.39653228388428374 ) ) ;
#38858=B_SPLINE_CURVE_WITH_KNOTS ( 'NONE', 1,
 ( #35242, #5474 ),
 .UNSPECIFIED., .F., .F.,
 ( 2, 2 ),
 ( 0.000000000000000000, 1.000000000000000000 ),
 .UNSPECIFIED. ) ;
#38862=ORIENTED_EDGE ( 'NONE', *, *, #48243, .F. ) ;
#38864=CARTESIAN_POINT ( 'NONE',  ( -21.23484681875272528, -20.74088929683185611, 69.33978048267414351 ) ) ;
#38865=CARTESIAN_POINT ( 'NONE',  ( -10.99655682251556144, -18.57624055219563175, 57.99209882808910521 ) ) ;
#38868=CARTESIAN_POINT ( 'NONE',  ( -12.41953831520651264, -9.914705408137539422, 57.38935537466883119 ) ) ;
#38869=EDGE_CURVE ( 'NONE', #31039, #16383, #35702, .T. ) ;
#38871=CARTESIAN_POINT ( 'NONE',  ( -18.63018970549565978, -7.457396494496333794, 73.95569010969242640 ) ) ;
#38873=EDGE_LOOP ( 'NONE', ( #41375, #14319, #29474, #17826, #28590 ) ) ;
#38874=CARTESIAN_POINT ( 'NONE',  ( -12.35909018435058471, -20.27262818183478998, 68.52995730439641875 ) ) ;
#38875=CARTESIAN_POINT ( 'NONE',  ( -16.06904075904983031, -7.890656793283916670, 63.97011029956861705 ) ) ;
#38876=B_SPLINE_CURVE_WITH_KNOTS ( 'NONE', 3,
 ( #46574, #39412, #9633, #20941, #5694, #13529, #24649, #20703, #1978, #31540 ),
 .UNSPECIFIED., .F., .F.,
 ( 4, 2, 2, 2, 4 ),
 ( 0.000000000000000000, 0.2500000000000000000, 0.5000000000000000000, 0.7500000000000000000, 1.000000000000000000 ),
 .UNSPECIFIED. ) ;
#38878=( BOUNDED_SURFACE ( )  B_SPLINE_SURFACE ( 3, 1, ( 
 ( #8678, #42161 ),
 ( #552, #4483 ),
 ( #38197, #1039 ),
 ( #7961, #5218 ),
 ( #16033, #31074 ),
 ( #26907, #34998 ),
 ( #41917, #45864 ) ),
 .UNSPECIFIED., .T., .F., .F. ) 
 B_SPLINE_SURFACE_WITH_KNOTS ( ( 4, 3, 4 ),
 ( 2, 2 ),
 ( 0.000000000000000000, 0.5000000000000000000, 1.000000000000000000 ),
 ( 0.000000000000000000, 1.000000000000000000 ),
 .UNSPECIFIED. ) 
 GEOMETRIC_REPRESENTATION_ITEM ( )  RATIONAL_B_SPLINE_SURFACE ( (
 ( 1.000000000000000000, 1.000000000000000000),
 ( 0.3333333333333335369, 0.3333333333333330373),
 ( 0.3333333333333335369, 0.3333333333333330373),
 ( 1.000000000000000000, 1.000000000000000000),
 ( 0.3333333333333333703, 0.3333333333333333703),
 ( 0.3333333333333333703, 0.3333333333333333703),
 ( 1.000000000000000000, 1.000000000000000000) ) ) 
 REPRESENTATION_ITEM ( '' )  SURFACE ( )  );
#38879=CARTESIAN_POINT ( 'NONE',  ( -18.92901792560347829, -7.918630368440815026, 70.78556921992733919 ) ) ;
#38881=ORIENTED_EDGE ( 'NONE', *, *, #15687, .F. ) ;
#38882=CARTESIAN_POINT ( 'NONE',  ( -15.05422094890265683, -21.39590065587122325, 61.70888574689368511 ) ) ;
#38884=CARTESIAN_POINT ( 'NONE',  ( -22.17374636168253943, -9.068608547125135644, 63.37809084343794552 ) ) ;
#38886=EDGE_CURVE ( 'NONE', #32391, #20038, #13882, .T. ) ;
#38889=FACE_OUTER_BOUND ( 'NONE', #25152, .T. ) ;
#38890=VECTOR ( 'NONE', #16727, 1000.000000000000000 ) ;
#38891=VERTEX_POINT ( 'NONE', #42152 ) ;
#38892=CARTESIAN_POINT ( 'NONE',  ( -11.42587710518540334, -11.10406226247761019, 57.49431069621225276 ) ) ;
#38893=CARTESIAN_POINT ( 'NONE',  ( -16.16748626245079379, -22.20318634978239203, 54.27966884056655061 ) ) ;
#38895=EDGE_CURVE ( 'NONE', #17121, #10137, #4592, .T. ) ;
#38896=CARTESIAN_POINT ( 'NONE',  ( -13.14320010650797776, -9.203067583597343670, 71.14925540519338654 ) ) ;
#38897=EDGE_LOOP ( 'NONE', ( #17507, #8842, #1777, #27802, #4305 ) ) ;
#38898=DIRECTION ( 'NONE',  ( -0.4749924142254752235, -0.8799898899579782219, -8.916637576350563827E-09 ) ) ;
#38899=CARTESIAN_POINT ( 'NONE',  ( -18.57335281209669375, -21.76520412651811043, 72.57038810541313012 ) ) ;
#38901=CARTESIAN_POINT ( 'NONE',  ( -18.10946867608448940, -21.82882885753907942, 69.23003497527133732 ) ) ;
#38904=CARTESIAN_POINT ( 'NONE',  ( -24.42872760227104578, -14.00939437836273349, 73.41711714289721158 ) ) ;
#38905=CARTESIAN_POINT ( 'NONE',  ( -14.65746096889331263, -8.316078616448901784, 57.00567256703398300 ) ) ;
#38906=DIRECTION ( 'NONE',  ( -0.8604039311673230550, -0.5096126717731922495, 7.110477544621476444E-08 ) ) ;
#38907=VERTEX_POINT ( 'NONE', #45365 ) ;
#38909=CARTESIAN_POINT ( 'NONE',  ( -11.77169895589660342, -10.59578386207264700, 74.43885051664024388 ) ) ;
#38910=B_SPLINE_CURVE_WITH_KNOTS ( 'NONE', 1,
 ( #8767, #24026 ),
 .UNSPECIFIED., .F., .F.,
 ( 2, 2 ),
 ( 0.000000000000000000, 1.000000000000000000 ),
 .UNSPECIFIED. ) ;
#38911=EDGE_CURVE ( 'NONE', #7864, #31485, #30898, .T. ) ;
#38912=CARTESIAN_POINT ( 'NONE',  ( -24.61402911129809112, -12.85776555077031880, 66.40972601524751440 ) ) ;
#38913=CARTESIAN_POINT ( 'NONE',  ( -15.09544305450467938, -21.46351983957133669, 65.40596681500470311 ) ) ;
#38914=ORIENTED_EDGE ( 'NONE', *, *, #45976, .T. ) ;
#38915=ORIENTED_EDGE ( 'NONE', *, *, #13741, .T. ) ;
#38916=EDGE_CURVE ( 'NONE', #34444, #29137, #21596, .T. ) ;
#38917=CARTESIAN_POINT ( 'NONE',  ( -18.62860737289870983, -7.457144689169211027, 74.09710349057253609 ) ) ;
#38918=CARTESIAN_POINT ( 'NONE',  ( -14.60479746972646886, -7.913168098764732150, 60.50491608655884335 ) ) ;
#38920=CARTESIAN_POINT ( 'NONE',  ( -15.75439910800316845, -7.548642891367095764, 67.18361323375314953 ) ) ;
#38921=CARTESIAN_POINT ( 'NONE',  ( -10.68551981713787136, -12.73596763222149164, 64.28308208171728211 ) ) ;
#38923=CARTESIAN_POINT ( 'NONE',  ( -18.85724798917316392, -7.906108138700305155, 67.18599644112759961 ) ) ;
#38924=( BOUNDED_CURVE ( )  B_SPLINE_CURVE ( 3, ( #33015, #11363, #41157, #33495 ),
 .UNSPECIFIED., .F., .F. ) 
 B_SPLINE_CURVE_WITH_KNOTS ( ( 4, 4 ),
 ( 0.9074455897393701731, 1.000000000000000000 ),
 .UNSPECIFIED. ) 
 CURVE ( )  GEOMETRIC_REPRESENTATION_ITEM ( )  RATIONAL_B_SPLINE_CURVE ( ( 0.6983129098261113832, 0.7760317562607140784, 0.8765941196520102840, 1.000000000000000000 ) ) 
 REPRESENTATION_ITEM ( '' )  );
#38925=CARTESIAN_POINT ( 'NONE',  ( -10.95917937052863245, -17.62195967018737264, 71.58190244267143498 ) ) ;
#38929=CARTESIAN_POINT ( 'NONE',  ( -22.63674339536608926, -20.13198319316658313, 69.43063894133570102 ) ) ;
#38932=CARTESIAN_POINT ( 'NONE',  ( -22.71334156758821265, -10.13600392596141475, 63.22752948238618842 ) ) ;
#38933=CARTESIAN_POINT ( 'NONE',  ( -26.80819156775448420, -19.72453833035618942, 53.49999999999995026 ) ) ;
#38934=CARTESIAN_POINT ( 'NONE',  ( -21.46445858442271870, -9.092811667914396878, 70.43132491394226236 ) ) ;
#38935=EDGE_CURVE ( 'NONE', #39661, #18572, #14159, .T. ) ;
#38936=( BOUNDED_SURFACE ( )  B_SPLINE_SURFACE ( 3, 1, ( 
 ( #14866, #41244 ),
 ( #33847, #144 ),
 ( #43994, #10250 ),
 ( #25263, #40282 ),
 ( #6549, #4082 ),
 ( #861, #30669 ),
 ( #5042, #12182 ) ),
 .UNSPECIFIED., .T., .F., .F. ) 
 B_SPLINE_SURFACE_WITH_KNOTS ( ( 4, 3, 4 ),
 ( 2, 2 ),
 ( 0.000000000000000000, 0.5000000000000000000, 1.000000000000000000 ),
 ( 0.000000000000000000, 1.000000000000000000 ),
 .UNSPECIFIED. ) 
 GEOMETRIC_REPRESENTATION_ITEM ( )  RATIONAL_B_SPLINE_SURFACE ( (
 ( 1.000000000000000000, 1.000000000000000000),
 ( 0.3333333333333335369, 0.3333333333333330373),
 ( 0.3333333333333335369, 0.3333333333333330373),
 ( 1.000000000000000000, 1.000000000000000000),
 ( 0.3333333333333333703, 0.3333333333333333703),
 ( 0.3333333333333333703, 0.3333333333333333703),
 ( 1.000000000000000000, 1.000000000000000000) ) ) 
 REPRESENTATION_ITEM ( '' )  SURFACE ( )  );
#38938=ORIENTED_EDGE ( 'NONE', *, *, #24802, .T. ) ;
#38939=ORIENTED_EDGE ( 'NONE', *, *, #23618, .F. ) ;
#38940=VERTEX_POINT ( 'NONE', #12107 ) ;
#38941=EDGE_CURVE ( 'NONE', #14012, #6698, #1965, .T. ) ;
#38943=CARTESIAN_POINT ( 'NONE',  ( -11.00375763999895007, -18.58866327377100447, 57.96747934402117153 ) ) ;
#38945=CARTESIAN_POINT ( 'NONE',  ( -21.52107272639815960, -9.068161724387254097, 66.54661176836198422 ) ) ;
#38946=DIRECTION ( 'NONE',  ( -8.478320030308545538E-07, 8.009068449373887445E-06, -0.9999999999675679430 ) ) ;
#38947=VERTEX_POINT ( 'NONE', #5213 ) ;
#38948=CARTESIAN_POINT ( 'NONE',  ( -23.13707066727631556, -18.94018274121504319, 62.65406854393442160 ) ) ;
#38949=CARTESIAN_POINT ( 'NONE',  ( -19.03984369153074141, -21.67464089235836511, 58.93996235972087305 ) ) ;
#38950=EDGE_LOOP ( 'NONE', ( #8, #7610, #47067, #25501, #2868 ) ) ;
#38951=CARTESIAN_POINT ( 'NONE',  ( -16.78411497196904278, -21.83009869597352903, 68.69560651670111895 ) ) ;
#38952=DIRECTION ( 'NONE',  ( -0.003782665018460030538, -0.9999928456970870183, -9.532993539451315208E-09 ) ) ;
#38957=FACE_OUTER_BOUND ( 'NONE', #9827, .T. ) ;
#38958=VERTEX_POINT ( 'NONE', #35703 ) ;
#38959=CARTESIAN_POINT ( 'NONE',  ( -24.26156011361375420, -17.76763406014958591, 62.58022692647417529 ) ) ;
#38960=EDGE_CURVE ( 'NONE', #23831, #828, #37469, .T. ) ;
#38961=CARTESIAN_POINT ( 'NONE',  ( -14.64754011156049174, -7.895932636330921461, 60.52007478328511780 ) ) ;
#38962=CARTESIAN_POINT ( 'NONE',  ( -24.09941705946771862, -11.50122934708656608, 63.05194655968659845 ) ) ;
#38963=B_SPLINE_CURVE_WITH_KNOTS ( 'NONE', 3,
 ( #4058, #41458, #22507, #37019, #11191, #7506, #40726, #38001, #41217, #37257 ),
 .UNSPECIFIED., .F., .F.,
 ( 4, 2, 2, 2, 4 ),
 ( 0.6272669072877513630, 0.7522669073072626444, 0.8772669073267738149, 1.002266907346285096, 1.127266907365796378 ),
 .UNSPECIFIED. ) ;
#38964=CARTESIAN_POINT ( 'NONE',  ( -14.53471675559079834, -21.67622060161817643, 58.28900965065733430 ) ) ;
#38966=CARTESIAN_POINT ( 'NONE',  ( -19.24947176484442224, -8.051269630034916247, 59.96092964444785167 ) ) ;
#38967=EDGE_LOOP ( 'NONE', ( #39827, #34270, #43574, #47732, #21971 ) ) ;
#38968=CARTESIAN_POINT ( 'NONE',  ( -24.40947378145952129, -13.83047763063617630, 73.33091373203986052 ) ) ;
#38969=CARTESIAN_POINT ( 'NONE',  ( -22.78190067944302299, -10.22696095015725604, 66.84182243026252479 ) ) ;
#38970=CARTESIAN_POINT ( 'NONE',  ( -23.34288396506439867, -19.33377296368179543, 59.06906041190286771 ) ) ;
#38971=CARTESIAN_POINT ( 'NONE',  ( -14.20982565386415963, -21.02760505633974120, 72.03493667776581333 ) ) ;
#38973=EDGE_LOOP ( 'NONE', ( #11510, #14583, #37289, #4831, #36765 ) ) ;
#38975=CARTESIAN_POINT ( 'NONE',  ( -10.42822707016751416, -13.93690136499678900, 57.74825009391801700 ) ) ;
#38976=CARTESIAN_POINT ( 'NONE',  ( -10.81170448216924740, -12.36318809540519048, 57.34329390664808557 ) ) ;
#38977=ORIENTED_EDGE ( 'NONE', *, *, #45154, .F. ) ;
#38979=CARTESIAN_POINT ( 'NONE',  ( -12.18170095131842068, -10.17053037870675780, 64.02914326641410980 ) ) ;
#38980=CARTESIAN_POINT ( 'NONE',  ( -17.90041350441808632, -22.24413145357778987, 62.03682421940214908 ) ) ;
#38981=CARTESIAN_POINT ( 'NONE',  ( -24.46479344177693349, -14.44719919422189491, 66.18292729247950490 ) ) ;
#38983=ORIENTED_EDGE ( 'NONE', *, *, #31958, .F. ) ;
#38985=DIRECTION ( 'NONE',  ( -0.1648596854219665231, -0.9863170302304251624, 7.074492695208254125E-08 ) ) ;
#38986=CARTESIAN_POINT ( 'NONE',  ( -12.23301264461619553, -10.03852782535897958, 60.84446034103241630 ) ) ;
#38988=CARTESIAN_POINT ( 'NONE',  ( -18.54404894011023686, -22.17459442116309631, 72.47849261052394354 ) ) ;
#38989=B_SPLINE_CURVE_WITH_KNOTS ( 'NONE', 1,
 ( #41988, #22294 ),
 .UNSPECIFIED., .F., .F.,
 ( 2, 2 ),
 ( 0.000000000000000000, 1.000000000000000000 ),
 .UNSPECIFIED. ) ;
#38990=CARTESIAN_POINT ( 'NONE',  ( -10.42255780831017553, -12.26328212591781686, 57.52195625194215012 ) ) ;
#38992=CARTESIAN_POINT ( 'NONE',  ( -13.73970650151387751, -20.76112128469266693, 64.98628881673506896 ) ) ;
#38993=CARTESIAN_POINT ( 'NONE',  ( -10.75313395769540747, -12.68406982142872153, 64.49665988512677472 ) ) ;
#38994=ORIENTED_EDGE ( 'NONE', *, *, #43765, .T. ) ;
#38996=VECTOR ( 'NONE', #605, 1000.000000000000000 ) ;
#38998=EDGE_CURVE ( 'NONE', #27411, #39949, #17350, .T. ) ;
#38999=ADVANCED_FACE ( 'NONE', ( #5702 ), #37168, .T. ) ;
#39001=CARTESIAN_POINT ( 'NONE',  ( -20.06397218905901880, -8.325598534408126028, 73.73713175987984414 ) ) ;
#39002=EDGE_CURVE ( 'NONE', #35531, #9195, #5714, .T. ) ;
#39003=EDGE_CURVE ( 'NONE', #16707, #48003, #18944, .T. ) ;
#39004=B_SPLINE_CURVE_WITH_KNOTS ( 'NONE', 3,
 ( #10725, #25743, #22058, #23045, #38266, #4324, #30436, #4093, #5055, #12429 ),
 .UNSPECIFIED., .F., .F.,
 ( 4, 2, 2, 2, 4 ),
 ( 0.000000000000000000, 0.2500000000000000000, 0.5000000000000000000, 0.7500000000000000000, 1.000000000000000000 ),
 .UNSPECIFIED. ) ;
#39006=CARTESIAN_POINT ( 'NONE',  ( -12.12304913700627829, -10.15599584246782783, 60.76738117878467449 ) ) ;
#39009=CARTESIAN_POINT ( 'NONE',  ( -17.91414045948978639, -21.84516348726148394, 65.76020891215902964 ) ) ;
#39011=CARTESIAN_POINT ( 'NONE',  ( -21.84256997353123353, -8.809979007422205299, 66.77494628644626573 ) ) ;
#39012=CARTESIAN_POINT ( 'NONE',  ( -12.84719740098974583, -9.512790884556105553, 74.61923006383901225 ) ) ;
#39013=VERTEX_POINT ( 'NONE', #1503 ) ;
#39014=CARTESIAN_POINT ( 'NONE',  ( -18.57746183813887697, -21.71359645443963515, 72.57045538883467373 ) ) ;
#39015=ORIENTED_EDGE ( 'NONE', *, *, #11390, .T. ) ;
#39017=EDGE_CURVE ( 'NONE', #38546, #7285, #46582, .T. ) ;
#39019=CARTESIAN_POINT ( 'NONE',  ( -21.25455046938168735, -8.881090050001144931, 70.28699408244519020 ) ) ;
#39021=ORIENTED_EDGE ( 'NONE', *, *, #42783, .T. ) ;
#39022=CARTESIAN_POINT ( 'NONE',  ( -18.60622096112062707, -22.16490860957766529, 72.47006221837980888 ) ) ;
#39023=CARTESIAN_POINT ( 'NONE',  ( -10.98557813051190202, -17.68114236276378293, 71.56718193507127523 ) ) ;
#39025=AXIS2_PLACEMENT_3D ( 'NONE', #39628, #13257, #9359 ) ;
#39027=CARTESIAN_POINT ( 'NONE',  ( -19.16034511560328824, -20.04212228129345874, 53.69233794759168177 ) ) ;
#39028=CARTESIAN_POINT ( 'NONE',  ( -20.86738180659939701, -20.96527767495129879, 58.85295087929227265 ) ) ;
#39030=CARTESIAN_POINT ( 'NONE',  ( -16.27095827323975996, -7.851109476482911909, 64.08499918177189159 ) ) ;
#39032=CARTESIAN_POINT ( 'NONE',  ( -23.74619265052512418, -11.68934008440960426, 62.95218278636776432 ) ) ;
#39033=EDGE_LOOP ( 'NONE', ( #15845, #528, #27418, #25069, #38060 ) ) ;
#39034=CARTESIAN_POINT ( 'NONE',  ( -11.21157534608376061, -11.58358818987947814, 67.91864608155252370 ) ) ;
#39035=CARTESIAN_POINT ( 'NONE',  ( -22.93319430828029581, -10.48995392174254526, 63.08802662987923782 ) ) ;
#39037=FACE_BOUND ( 'NONE', #23230, .T. ) ;
#39039=VERTEX_POINT ( 'NONE', #42880 ) ;
#39042=CARTESIAN_POINT ( 'NONE',  ( -22.48430581236326731, -20.27711595259535571, 65.81926302645771898 ) ) ;
#39044=CARTESIAN_POINT ( 'NONE',  ( -23.44980453451081104, -18.46889374286061525, 73.06368236440982855 ) ) ;
#39045=ORIENTED_EDGE ( 'NONE', *, *, #42578, .F. ) ;
#39048=EDGE_CURVE ( 'NONE', #12811, #32800, #42248, .T. ) ;
#39051=CARTESIAN_POINT ( 'NONE',  ( -24.05059673655033947, -17.06518960458298650, 73.18336032079744768 ) ) ;
#39052=( BOUNDED_CURVE ( )  B_SPLINE_CURVE ( 3, ( #14953, #18658, #3405, #39326 ),
 .UNSPECIFIED., .F., .F. ) 
 B_SPLINE_CURVE_WITH_KNOTS ( ( 4, 4 ),
 ( 0.9074455897393621795, 1.000000000000000000 ),
 .UNSPECIFIED. ) 
 CURVE ( )  GEOMETRIC_REPRESENTATION_ITEM ( )  RATIONAL_B_SPLINE_CURVE ( ( 0.6983129098260896228, 0.7760317562606953157, 0.8765941196519987377, 1.000000000000000000 ) ) 
 REPRESENTATION_ITEM ( '' )  );
#39054=VECTOR ( 'NONE', #7402, 1000.000000000000114 ) ;
#39056=ORIENTED_EDGE ( 'NONE', *, *, #2858, .T. ) ;
#39057=CARTESIAN_POINT ( 'NONE',  ( -23.05109822670184272, -10.64471945476145898, 59.88586922199753104 ) ) ;
#39058=CARTESIAN_POINT ( 'NONE',  ( -26.59010385426081413, -19.80682416827059455, 54.49999999999995026 ) ) ;
#39059=ADVANCED_FACE ( 'NONE', ( #19660 ), #23993, .T. ) ;
#39062=EDGE_CURVE ( 'NONE', #39384, #21434, #36206, .T. ) ;
#39063=B_SPLINE_CURVE_WITH_KNOTS ( 'NONE', 1,
 ( #928, #15192 ),
 .UNSPECIFIED., .F., .F.,
 ( 2, 2 ),
 ( 0.000000000000000000, 1.000000000000000000 ),
 .UNSPECIFIED. ) ;
#39065=CARTESIAN_POINT ( 'NONE',  ( -10.37795889460693033, -14.56696403379599225, 68.14328054657653411 ) ) ;
#39066=( BOUNDED_CURVE ( )  B_SPLINE_CURVE ( 3, ( #30537, #972, #23377, #22648 ),
 .UNSPECIFIED., .F., .F. ) 
 B_SPLINE_CURVE_WITH_KNOTS ( ( 4, 4 ),
 ( 0.5000000000000000000, 0.9074455897393653991 ),
 .UNSPECIFIED. ) 
 CURVE ( )  GEOMETRIC_REPRESENTATION_ITEM ( )  RATIONAL_B_SPLINE_CURVE ( ( 1.000000000000007327, 0.4567392136813294146, 0.3561768502900241606, 0.6983129098260996148 ) ) 
 REPRESENTATION_ITEM ( '' )  );
#39068=CARTESIAN_POINT ( 'NONE',  ( -11.56806251476610115, -18.73522173559940995, 65.03234934376791898 ) ) ;
#39069=CARTESIAN_POINT ( 'NONE',  ( -18.97210877009940688, -7.521729958488855061, 66.94425830142937173 ) ) ;
#39070=B_SPLINE_CURVE_WITH_KNOTS ( 'NONE', 3,
 ( #25589, #40598, #40373, #2931, #48235, #36649, #6641, #29530, #32958, #37380 ),
 .UNSPECIFIED., .F., .F.,
 ( 4, 2, 2, 2, 4 ),
 ( 0.000000000000000000, 0.2500000000000000000, 0.5000000000000000000, 0.7500000000000000000, 1.000000000000000000 ),
 .UNSPECIFIED. ) ;
#39072=LINE ( 'NONE', #34653, #10793 ) ;
#39073=CARTESIAN_POINT ( 'NONE',  ( -22.29619887594318683, -17.36118473213641167, 53.49999999999995026 ) ) ;
#39075=ORIENTED_EDGE ( 'NONE', *, *, #33588, .T. ) ;
#39077=( BOUNDED_CURVE ( )  B_SPLINE_CURVE ( 3, ( #33125, #48402, #19102, #7056 ),
 .UNSPECIFIED., .F., .F. ) 
 B_SPLINE_CURVE_WITH_KNOTS ( ( 4, 4 ),
 ( 0.4074455897393615689, 0.5000000000000000000 ),
 .UNSPECIFIED. ) 
 CURVE ( )  GEOMETRIC_REPRESENTATION_ITEM ( )  RATIONAL_B_SPLINE_CURVE ( ( 0.6983129098260875134, 0.7760317562606922071, 0.8765941196519960732, 0.9999999999999981126 ) ) 
 REPRESENTATION_ITEM ( '' )  );
#39080=CARTESIAN_POINT ( 'NONE',  ( -10.37873872693602273, -15.23103030436339544, 74.95345861988057834 ) ) ;
#39081=VERTEX_POINT ( 'NONE', #15207 ) ;
#39082=CARTESIAN_POINT ( 'NONE',  ( -24.41553149706675896, -15.71832598455623398, 69.81835354388927328 ) ) ;
#39083=CARTESIAN_POINT ( 'NONE',  ( -10.90323534495222546, -12.10858216263579124, 57.47290069719868910 ) ) ;
#39084=CARTESIAN_POINT ( 'NONE',  ( -24.23115020962818278, -13.17656271950065161, 62.83264225666157188 ) ) ;
#39085=LINE ( 'NONE', #11593, #36093 ) ;
#39087=DIRECTION ( 'NONE',  ( -0.3478314405900308492, -0.9375570856950864451, 0.000000000000000000 ) ) ;
#39088=CARTESIAN_POINT ( 'NONE',  ( -20.88270717056239789, -21.40782548341276481, 58.82970473467946704 ) ) ;
#39089=CARTESIAN_POINT ( 'NONE',  ( -10.09263637371726041, -16.13336529236863015, 68.02121877882343881 ) ) ;
#39090=ORIENTED_EDGE ( 'NONE', *, *, #9006, .F. ) ;
#39091=CARTESIAN_POINT ( 'NONE',  ( -11.45027127459337279, -18.55327342931734691, 61.57151016578320935 ) ) ;
#39094=FACE_OUTER_BOUND ( 'NONE', #26972, .T. ) ;
#39095=B_SPLINE_CURVE_WITH_KNOTS ( 'NONE', 3,
 ( #21695, #33474, #7419, #26360, #45332, #22187, #37171, #44360, #40637, #14274 ),
 .UNSPECIFIED., .F., .F.,
 ( 4, 2, 2, 2, 4 ),
 ( 0.1272669073658244943, 0.2522669073463070233, 0.3772669073267895801, 0.5022669073072720813, 0.6272669072877545826 ),
 .UNSPECIFIED. ) ;
#39097=ORIENTED_EDGE ( 'NONE', *, *, #1828, .T. ) ;
#39103=CARTESIAN_POINT ( 'NONE',  ( -11.85162103594838001, -10.49015045520576983, 71.25420998615621215 ) ) ;
#39104=EDGE_CURVE ( 'NONE', #34125, #48039, #48499, .T. ) ;
#39106=CARTESIAN_POINT ( 'NONE',  ( -23.23016983938471824, -18.72167312165286646, 69.36542358921913376 ) ) ;
#39107=CARTESIAN_POINT ( 'NONE',  ( -13.89389072038462025, -21.36980434119256600, 72.11103101793651149 ) ) ;
#39110=CARTESIAN_POINT ( 'NONE',  ( -10.40277073914389661, -15.44443991871667166, 57.56792809063193062 ) ) ;
#39112=CARTESIAN_POINT ( 'NONE',  ( -22.42700276027757411, -19.70584140869366863, 72.66017131446398025 ) ) ;
#39113=DIRECTION ( 'NONE',  ( -1.081321489524789733E-05, -7.211308818607114576E-06, 0.9999999999155356756 ) ) ;
#39114=B_SPLINE_CURVE_WITH_KNOTS ( 'NONE', 1,
 ( #15176, #18894 ),
 .UNSPECIFIED., .F., .F.,
 ( 2, 2 ),
 ( 0.000000000000000000, 1.000000000000000000 ),
 .UNSPECIFIED. ) ;
#39115=ORIENTED_EDGE ( 'NONE', *, *, #27878, .F. ) ;
#39116=CARTESIAN_POINT ( 'NONE',  ( -20.17979545193272273, -21.30158238988698116, 72.28990119599492914 ) ) ;
#39117=CARTESIAN_POINT ( 'NONE',  ( -24.86601949095794239, -14.46076817688473071, 66.43938638393159124 ) ) ;
#39118=ADVANCED_FACE ( 'NONE', ( #7862 ), #22883, .T. ) ;
#39120=CARTESIAN_POINT ( 'NONE',  ( -22.79734351242366941, -10.24514170768878962, 66.69182257473532616 ) ) ;
#39123=ORIENTED_EDGE ( 'NONE', *, *, #25703, .F. ) ;
#39124=CARTESIAN_POINT ( 'NONE',  ( -24.41485940220508510, -14.44976662329334616, 66.18292729254385165 ) ) ;
#39125=AXIS2_PLACEMENT_3D ( 'NONE', #29502, #48214, #44534 ) ;
#39126=EDGE_CURVE ( 'NONE', #38697, #26255, #3549, .T. ) ;
#39128=CARTESIAN_POINT ( 'NONE',  ( -24.42331094741535580, -14.99212712107751955, 59.35373227113915107 ) ) ;
#39129=VECTOR ( 'NONE', #16429, 1000.000000000000114 ) ;
#39130=CARTESIAN_POINT ( 'NONE',  ( -14.31284414862750864, -10.25749249327297896, 53.88362224778187226 ) ) ;
#39131=EDGE_CURVE ( 'NONE', #39358, #20248, #10736, .T. ) ;
#39132=CARTESIAN_POINT ( 'NONE',  ( -18.90996479553717791, -7.968725069611966916, 66.90071784165556323 ) ) ;
#39134=CARTESIAN_POINT ( 'NONE',  ( -10.49786192289579922, -13.78684457455405088, 57.51995378590393670 ) ) ;
#39135=ORIENTED_EDGE ( 'NONE', *, *, #4349, .T. ) ;
#39136=CARTESIAN_POINT ( 'NONE',  ( -10.00806915883838855, -14.09796239111615890, 61.11095435805616205 ) ) ;
#39139=CARTESIAN_POINT ( 'NONE',  ( -24.42549660922115251, -13.91739599595199728, 69.80842429065324950 ) ) ;
#39140=CARTESIAN_POINT ( 'NONE',  ( -18.39951258112534305, -22.19516185762106275, 69.00009993223443416 ) ) ;
#39142=ORIENTED_EDGE ( 'NONE', *, *, #3461, .F. ) ;
#39143=CARTESIAN_POINT ( 'NONE',  ( -11.93102524044397938, -10.47028995287008257, 71.26893105764186487 ) ) ;
#39144=CARTESIAN_POINT ( 'NONE',  ( -14.77897477670383353, -8.270997283837589364, 56.73511376018900876 ) ) ;
#39145=B_SPLINE_CURVE_WITH_KNOTS ( 'NONE', 1,
 ( #4269, #11403 ),
 .UNSPECIFIED., .F., .F.,
 ( 2, 2 ),
 ( 0.000000000000000000, 1.000000000000000000 ),
 .UNSPECIFIED. ) ;
#39146=CARTESIAN_POINT ( 'NONE',  ( -10.89682964601354698, -17.33834430218308498, 64.62739378818586999 ) ) ;
#39150=CARTESIAN_POINT ( 'NONE',  ( -10.93232766038821424, -17.55941949638709687, 68.38249893951126523 ) ) ;
#39151=DIRECTION ( 'NONE',  ( -0.7107718805962432995, -0.7034225854731134264, -7.722840056494082694E-09 ) ) ;
#39152=DIRECTION ( 'NONE',  ( 0.8603613874411328855, -0.3191920208248662516, -0.3973597071195153485 ) ) ;
#39154=ORIENTED_EDGE ( 'NONE', *, *, #32752, .T. ) ;
#39155=CARTESIAN_POINT ( 'NONE',  ( -11.68335768792166185, -18.81469630946190819, 68.51689631952916670 ) ) ;
#39156=CARTESIAN_POINT ( 'NONE',  ( -13.27770768808250956, -9.107454094634595876, 63.90946529206384241 ) ) ;
#39157=ORIENTED_EDGE ( 'NONE', *, *, #46345, .T. ) ;
#39158=VECTOR ( 'NONE', #36219, 1000.000000000000227 ) ;
#39159=CARTESIAN_POINT ( 'NONE',  ( -15.82103535061131261, -7.533639916251397395, 67.39653228388428374 ) ) ;
#39162=CARTESIAN_POINT ( 'NONE',  ( -13.06442264889613192, -8.767972821088468649, 64.10284853510081859 ) ) ;
#39163=EDGE_CURVE ( 'NONE', #18099, #27374, #12027, .T. ) ;
#39165=CARTESIAN_POINT ( 'NONE',  ( -15.69736356130078647, -8.025520047610617880, 70.90989840317035942 ) ) ;
#39168=CARTESIAN_POINT ( 'NONE',  ( -13.00210270896756803, -8.813292789292800578, 64.04799975586527694 ) ) ;
#39169=DIRECTION ( 'NONE',  ( -0.1738928961406289164, 0.9847645711904029486, 7.871847295470929299E-08 ) ) ;
#39171=DIRECTION ( 'NONE',  ( -1.411223638961666279E-06, -4.279116281890322592E-06, -0.9999999999898487868 ) ) ;
#39172=CARTESIAN_POINT ( 'NONE',  ( -14.09638704727594138, -8.593948190025162859, 74.19954651715224259 ) ) ;
#39173=EDGE_CURVE ( 'NONE', #19371, #25718, #30751, .T. ) ;
#39174=ORIENTED_EDGE ( 'NONE', *, *, #14822, .F. ) ;
#39177=CARTESIAN_POINT ( 'NONE',  ( -24.87123163304818974, -14.59964195235338735, 62.89791815715346956 ) ) ;
#39179=EDGE_CURVE ( 'NONE', #21955, #6964, #29773, .T. ) ;
#39180=CARTESIAN_POINT ( 'NONE',  ( -14.78754730678460660, -8.270772302057270764, 60.46996282000571199 ) ) ;
#39181=VERTEX_POINT ( 'NONE', #24081 ) ;
#39183=ADVANCED_FACE ( 'NONE', ( #31458 ), #24277, .T. ) ;
#39184=CARTESIAN_POINT ( 'NONE',  ( -22.53429313110963150, -9.952421254863264011, 73.78161091678163075 ) ) ;
#39185=VERTEX_POINT ( 'NONE', #9553 ) ;
#39186=CARTESIAN_POINT ( 'NONE',  ( -10.99575410903449679, -18.57485570963264010, 57.85068653066719691 ) ) ;
#39187=AXIS2_PLACEMENT_3D ( 'NONE', #399, #22554, #29215 ) ;
#39188=EDGE_CURVE ( 'NONE', #47654, #28368, #34030, .T. ) ;
#39189=CARTESIAN_POINT ( 'NONE',  ( -17.59211729576255934, -7.811223397794364587, 63.55057029380298417 ) ) ;
#39190=ORIENTED_EDGE ( 'NONE', *, *, #14610, .F. ) ;
#39191=CARTESIAN_POINT ( 'NONE',  ( -10.78771056441093101, -12.58245623652513068, 57.43743428873830936 ) ) ;
#39193=CARTESIAN_POINT ( 'NONE',  ( -10.12501222943673085, -13.31701186804058601, 74.78479332379183120 ) ) ;
#39194=AXIS2_PLACEMENT_3D ( 'NONE', #14287, #44610, #48285 ) ;
#39196=EDGE_LOOP ( 'NONE', ( #7891, #1745 ) ) ;
#39197=CARTESIAN_POINT ( 'NONE',  ( -14.22938784291135406, -8.524548850093141894, 71.02957622767809198 ) ) ;
#39198=CARTESIAN_POINT ( 'NONE',  ( -12.52524223387102253, -19.88411517873010226, 61.60498656843740406 ) ) ;
#39199=CARTESIAN_POINT ( 'NONE',  ( -24.05845721068777010, -12.57644527891515551, 73.54225570276561541 ) ) ;
#39200=ORIENTED_EDGE ( 'NONE', *, *, #43310, .F. ) ;
#39202=CARTESIAN_POINT ( 'NONE',  ( -14.68443175557002434, -7.881056518746638595, 60.45962889931271178 ) ) ;
#39203=CARTESIAN_POINT ( 'NONE',  ( -24.11734051643545484, -11.53754943384703147, 63.05944116141331790 ) ) ;
#39204=VECTOR ( 'NONE', #12141, 1000.000000000000000 ) ;
#39205=( BOUNDED_CURVE ( )  B_SPLINE_CURVE ( 3, ( #20741, #39207, #9672, #5492 ),
 .UNSPECIFIED., .F., .F. ) 
 B_SPLINE_CURVE_WITH_KNOTS ( ( 4, 4 ),
 ( 0.4074455897279358751, 0.5000000000000000000 ),
 .UNSPECIFIED. ) 
 CURVE ( )  GEOMETRIC_REPRESENTATION_ITEM ( )  RATIONAL_B_SPLINE_CURVE ( ( 0.6983129097972999855, 0.7760317562358755028, 0.8765941196367799115, 1.000000000000023315 ) ) 
 REPRESENTATION_ITEM ( '' )  );
#39207=CARTESIAN_POINT ( 'NONE',  ( -11.17819277842271930, -11.53937649752676720, 67.61864623736559565 ) ) ;
#39208=CARTESIAN_POINT ( 'NONE',  ( -10.45720024584091945, -15.50224739959347175, 61.26618945053532173 ) ) ;
#39209=CARTESIAN_POINT ( 'NONE',  ( -10.38541819892233597, -17.25046345042985507, 61.25768869185118604 ) ) ;
#39210=ORIENTED_EDGE ( 'NONE', *, *, #43070, .F. ) ;
#39211=CARTESIAN_POINT ( 'NONE',  ( -10.41569439578338496, -15.57669382292980131, 61.05261153187079515 ) ) ;
#39213=CARTESIAN_POINT ( 'NONE',  ( -17.72634075389897035, -21.85272461700124680, 58.55553378267870812 ) ) ;
#39214=CARTESIAN_POINT ( 'NONE',  ( -24.86566085326441211, -14.45379301838039865, 66.37631023280182774 ) ) ;
#39216=CARTESIAN_POINT ( 'NONE',  ( -14.07761835836965858, -20.95746660330474143, 72.22607703844037985 ) ) ;
#39217=EDGE_CURVE ( 'NONE', #5635, #4167, #12972, .T. ) ;
#39220=CARTESIAN_POINT ( 'NONE',  ( -24.47371109942907808, -14.90716652360855576, 59.25772288469824645 ) ) ;
#39221=DIRECTION ( 'NONE',  ( -8.226841962295982234E-06, 2.386003339349608660E-06, 0.9999999999633130132 ) ) ;
#39222=EDGE_LOOP ( 'NONE', ( #21384, #2440, #42464, #12489, #40244 ) ) ;
#39224=CARTESIAN_POINT ( 'NONE',  ( -23.99312320239454976, -11.29471777418100231, 66.60709819448160829 ) ) ;
#39225=CARTESIAN_POINT ( 'NONE',  ( -17.90018989731357735, -22.24414728290300047, 62.01502546368934077 ) ) ;
#39226=CARTESIAN_POINT ( 'NONE',  ( -12.74057395449646712, -20.01165780218009971, 68.62192124028820217 ) ) ;
#39227=CARTESIAN_POINT ( 'NONE',  ( -15.03764954898300488, -21.45148416623199594, 58.32185190926050211 ) ) ;
#39228=EDGE_LOOP ( 'NONE', ( #8692, #42992, #7076, #15275 ) ) ;
#39229=CARTESIAN_POINT ( 'NONE',  ( -22.35906936724365579, -19.84913318925590175, 72.94400511917729091 ) ) ;
#39230=( BOUNDED_SURFACE ( )  B_SPLINE_SURFACE ( 3, 1, ( 
 ( #727, #30533 ),
 ( #45553, #23142 ),
 ( #4408, #19426 ),
 ( #1436, #16451 ),
 ( #20156, #32456 ),
 ( #43307, #16927 ),
 ( #31484, #1927 ) ),
 .UNSPECIFIED., .T., .F., .F. ) 
 B_SPLINE_SURFACE_WITH_KNOTS ( ( 4, 3, 4 ),
 ( 2, 2 ),
 ( 0.000000000000000000, 0.5000000000000000000, 1.000000000000000000 ),
 ( 0.000000000000000000, 1.000000000000000000 ),
 .UNSPECIFIED. ) 
 GEOMETRIC_REPRESENTATION_ITEM ( )  RATIONAL_B_SPLINE_SURFACE ( (
 ( 1.000000000000000000, 1.000000000000000000),
 ( 0.3333333333333335369, 0.3333333333333330373),
 ( 0.3333333333333335369, 0.3333333333333330373),
 ( 1.000000000000000000, 1.000000000000000000),
 ( 0.3333333333333333703, 0.3333333333333333703),
 ( 0.3333333333333333703, 0.3333333333333333703),
 ( 1.000000000000000000, 1.000000000000000000) ) ) 
 REPRESENTATION_ITEM ( '' )  SURFACE ( )  );
#39231=CARTESIAN_POINT ( 'NONE',  ( -11.50273385864769438, -11.07591097799543256, 57.50903212538073461 ) ) ;
#39232=LINE ( 'NONE', #12399, #17299 ) ;
#39234=CARTESIAN_POINT ( 'NONE',  ( -17.40545348791034286, -7.756229321676927135, 70.90524440011041918 ) ) ;
#39235=B_SPLINE_CURVE_WITH_KNOTS ( 'NONE', 3,
 ( #36553, #36081, #43996, #20842, #10251, #36796, #2365, #24786, #21335, #17377 ),
 .UNSPECIFIED., .F., .F.,
 ( 4, 2, 2, 2, 4 ),
 ( 0.6272669072877758989, 0.7522669073072892898, 0.8772669073268026807, 1.002266907346315961, 1.127266907365829463 ),
 .UNSPECIFIED. ) ;
#39237=CARTESIAN_POINT ( 'NONE',  ( -13.37043603341178688, -9.101843825305518720, 64.19330030611368443 ) ) ;
#39239=CARTESIAN_POINT ( 'NONE',  ( -24.54003134496739946, -12.60314121952208311, 69.96517145308561680 ) ) ;
#39241=CARTESIAN_POINT ( 'NONE',  ( -10.75313422144682463, -12.68406895456895889, 64.34006388750040628 ) ) ;
#39242=VECTOR ( 'NONE', #18760, 1000.000000000000114 ) ;
#39245=VERTEX_POINT ( 'NONE', #27522 ) ;
#39247=DIRECTION ( 'NONE',  ( -0.5088156898428700670, -0.8608754809899751281, -5.922709712363688559E-08 ) ) ;
#39248=CARTESIAN_POINT ( 'NONE',  ( -14.81535805098777736, -7.777528402031247623, 53.89198173725363716 ) ) ;
#39250=CARTESIAN_POINT ( 'NONE',  ( -11.60006141122767609, -10.16330251221877390, 71.08397807149754044 ) ) ;
#39252=CARTESIAN_POINT ( 'NONE',  ( -22.92107871295896970, -10.47515356817426202, 59.82876682489222020 ) ) ;
#39255=CARTESIAN_POINT ( 'NONE',  ( -10.39538363539702104, -14.16717768424945412, 68.00232930279112509 ) ) ;
#39256=CARTESIAN_POINT ( 'NONE',  ( -24.46146587544552276, -14.38248120490118609, 66.46820668217904426 ) ) ;
#39258=FACE_OUTER_BOUND ( 'NONE', #41159, .T. ) ;
#39260=VERTEX_POINT ( 'NONE', #6079 ) ;
#39261=B_SPLINE_CURVE_WITH_KNOTS ( 'NONE', 3,
 ( #33902, #4598, #19617, #41292, #12227, #30475, #34625, #30953, #7827, #45964 ),
 .UNSPECIFIED., .F., .F.,
 ( 4, 2, 2, 2, 4 ),
 ( 0.000000000000000000, 0.2500000000000000000, 0.5000000000000000000, 0.7500000000000000000, 1.000000000000000000 ),
 .UNSPECIFIED. ) ;
#39262=CARTESIAN_POINT ( 'NONE',  ( -13.33866014084052409, -21.03912497029407902, 61.61622683954244195 ) ) ;
#39264=EDGE_LOOP ( 'NONE', ( #9527, #14331, #7933, #30920, #28209 ) ) ;
#39265=CARTESIAN_POINT ( 'NONE',  ( -17.39128687056474121, -21.86710222072322907, 58.54986106076864161 ) ) ;
#39266=B_SPLINE_CURVE_WITH_KNOTS ( 'NONE', 3,
 ( #19080, #42470, #23517, #15862, #34326, #8489, #31133, #19321, #4543, #613 ),
 .UNSPECIFIED., .F., .F.,
 ( 4, 2, 2, 2, 4 ),
 ( 0.000000000000000000, 0.2500000000000000000, 0.5000000000000000000, 0.7500000000000000000, 1.000000000000000000 ),
 .UNSPECIFIED. ) ;
#39268=VECTOR ( 'NONE', #45002, 1000.000000000000114 ) ;
#39269=CARTESIAN_POINT ( 'NONE',  ( -19.11145711862998553, -7.964113067175272676, 63.58089235102941217 ) ) ;
#39271=ORIENTED_EDGE ( 'NONE', *, *, #41183, .F. ) ;
#39272=CYLINDRICAL_SURFACE ( 'NONE', #18911, 0.1499999999999979128 ) ;
#39273=DIRECTION ( 'NONE',  ( 0.9862050927915949616, 0.1655279884246635413, 7.765682856207886445E-08 ) ) ;
#39275=VECTOR ( 'NONE', #32265, 1000.000000000000000 ) ;
#39276=EDGE_CURVE ( 'NONE', #3179, #8795, #34459, .T. ) ;
#39277=CARTESIAN_POINT ( 'NONE',  ( -12.27604185553471616, -19.62628656662749549, 58.21210303282668264 ) ) ;
#39279=EDGE_CURVE ( 'NONE', #47942, #4057, #24473, .T. ) ;
#39282=LINE ( 'NONE', #4828, #27436 ) ;
#39283=VERTEX_POINT ( 'NONE', #21594 ) ;
#39285=CARTESIAN_POINT ( 'NONE',  ( -11.17650184932293733, -11.65192102369769422, 67.90399238740950238 ) ) ;
#39287=ORIENTED_EDGE ( 'NONE', *, *, #2167, .T. ) ;
#39288=CARTESIAN_POINT ( 'NONE',  ( -19.99669925590731268, -21.37628624441394010, 68.81993804536961079 ) ) ;
#39289=ORIENTED_EDGE ( 'NONE', *, *, #23553, .F. ) ;
#39293=CARTESIAN_POINT ( 'NONE',  ( -23.17271923358804031, -18.80355860159679082, 66.12389479708080842 ) ) ;
#39294=CARTESIAN_POINT ( 'NONE',  ( -17.42308114789593532, -7.359157070716391580, 67.21377881820035327 ) ) ;
#39295=CARTESIAN_POINT ( 'NONE',  ( -18.11889358109259973, -21.82488563948435711, 65.64532159284070190 ) ) ;
#39298=ORIENTED_EDGE ( 'NONE', *, *, #29300, .F. ) ;
#39300=EDGE_CURVE ( 'NONE', #23723, #36238, #33131, .T. ) ;
#39301=CARTESIAN_POINT ( 'NONE',  ( -13.86064791321372880, -8.266642500320580567, 74.39228826228381308 ) ) ;
#39303=CARTESIAN_POINT ( 'NONE',  ( -21.12749503816145591, -21.27438112535048376, 62.22816062766979428 ) ) ;
#39304=( BOUNDED_SURFACE ( )  B_SPLINE_SURFACE ( 3, 1, ( 
 ( #15716, #30773 ),
 ( #22391, #26577 ),
 ( #41343, #7880 ),
 ( #7391, #45548 ),
 ( #18941, #37384 ),
 ( #19185, #41848 ),
 ( #3676, #22641 ) ),
 .UNSPECIFIED., .T., .F., .F. ) 
 B_SPLINE_SURFACE_WITH_KNOTS ( ( 4, 3, 4 ),
 ( 2, 2 ),
 ( 0.000000000000000000, 0.5000000000000000000, 1.000000000000000000 ),
 ( 0.000000000000000000, 1.000000000000000000 ),
 .UNSPECIFIED. ) 
 GEOMETRIC_REPRESENTATION_ITEM ( )  RATIONAL_B_SPLINE_SURFACE ( (
 ( 1.000000000000000000, 1.000000000000000000),
 ( 0.3333333333333335369, 0.3333333333333330373),
 ( 0.3333333333333335369, 0.3333333333333330373),
 ( 1.000000000000000000, 1.000000000000000000),
 ( 0.3333333333333333703, 0.3333333333333333703),
 ( 0.3333333333333333703, 0.3333333333333333703),
 ( 1.000000000000000000, 1.000000000000000000) ) ) 
 REPRESENTATION_ITEM ( '' )  SURFACE ( )  );
#39305=CARTESIAN_POINT ( 'NONE',  ( -20.84119837601463487, -20.97572066283330727, 62.26471400470415318 ) ) ;
#39308=B_SPLINE_CURVE_WITH_KNOTS ( 'NONE', 3,
 ( #29249, #21619, #48195, #10770, #13953, #13718, #43795, #14425, #32919, #40093 ),
 .UNSPECIFIED., .F., .F.,
 ( 4, 2, 2, 2, 4 ),
 ( 0.000000000000000000, 0.2500000000000000000, 0.5000000000000000000, 0.7500000000000000000, 1.000000000000000000 ),
 .UNSPECIFIED. ) ;
#39309=ORIENTED_EDGE ( 'NONE', *, *, #30922, .T. ) ;
#39310=CARTESIAN_POINT ( 'NONE',  ( -14.72034176431206198, -21.75144939791099929, 61.77567047156098567 ) ) ;
#39311=PLANE ( 'NONE',  #33944 ) ;
#39312=DIRECTION ( 'NONE',  ( -3.597453700672850830E-07, -4.264980243973025121E-06, 0.9999999999908403270 ) ) ;
#39313=AXIS2_PLACEMENT_3D ( 'NONE', #47265, #40575, #28781 ) ;
#39314=ORIENTED_EDGE ( 'NONE', *, *, #48438, .F. ) ;
#39315=CARTESIAN_POINT ( 'NONE',  ( -24.31482301288783532, -13.31912224170856618, 59.66267924674057355 ) ) ;
#39316=CARTESIAN_POINT ( 'NONE',  ( -22.84886394736722792, -9.702774549906752810, 73.59665770010028041 ) ) ;
#39317=CARTESIAN_POINT ( 'NONE',  ( -11.01020281012788971, -12.00512747626467025, 74.84374947347477303 ) ) ;
#39319=ORIENTED_EDGE ( 'NONE', *, *, #31082, .F. ) ;
#39320=DIRECTION ( 'NONE',  ( 0.2664710960620865765, -0.9638429098994649724, 4.833213314675752896E-08 ) ) ;
#39321=CARTESIAN_POINT ( 'NONE',  ( -24.82995637329867122, -15.61904065536996278, 73.20292520421178040 ) ) ;
#39322=CARTESIAN_POINT ( 'NONE',  ( -17.96469556627129194, -21.78991212287910884, 65.53459228959106042 ) ) ;
#39323=VERTEX_POINT ( 'NONE', #29702 ) ;
#39324=CARTESIAN_POINT ( 'NONE',  ( -19.42896739221782809, -21.56812523091047851, 62.29503644570711174 ) ) ;
#39326=CARTESIAN_POINT ( 'NONE',  ( -24.47432067347917695, -14.77756146504815327, 59.52828185648635184 ) ) ;
#39327=DIRECTION ( 'NONE',  ( 0.1571515419521612722, -0.9875744999047174622, 7.433889655140131751E-08 ) ) ;
#39328=VERTEX_POINT ( 'NONE', #32891 ) ;
#39329=EDGE_CURVE ( 'NONE', #22802, #28574, #29460, .T. ) ;
#39335=CARTESIAN_POINT ( 'NONE',  ( -24.18037252889021005, -17.94870914462638822, 59.18873732074431615 ) ) ;
#39339=ORIENTED_EDGE ( 'NONE', *, *, #27492, .T. ) ;
#39340=CARTESIAN_POINT ( 'NONE',  ( -11.21783165637758550, -18.93062460193366192, 64.93202459354702683 ) ) ;
#39342=EDGE_CURVE ( 'NONE', #44748, #35674, #26015, .T. ) ;
#39343=ADVANCED_FACE ( 'NONE', ( #44742 ), #13692, .F. ) ;
#39346=ORIENTED_EDGE ( 'NONE', *, *, #23060, .F. ) ;
#39347=EDGE_CURVE ( 'NONE', #3920, #6656, #40942, .T. ) ;
#39348=CARTESIAN_POINT ( 'NONE',  ( -24.05813527555462628, -11.41757595432783745, 63.06562998582658253 ) ) ;
#39350=PLANE ( 'NONE',  #12307 ) ;
#39353=EDGE_CURVE ( 'NONE', #37344, #21796, #38574, .T. ) ;
#39354=( BOUNDED_CURVE ( )  B_SPLINE_CURVE ( 3, ( #35268, #38969, #34791, #42188 ),
 .UNSPECIFIED., .F., .F. ) 
 B_SPLINE_CURVE_WITH_KNOTS ( ( 4, 4 ),
 ( 0.9074455897393628456, 1.000000000000000000 ),
 .UNSPECIFIED. ) 
 CURVE ( )  GEOMETRIC_REPRESENTATION_ITEM ( )  RATIONAL_B_SPLINE_CURVE ( ( 0.6983129098260694168, 0.7760317562606778852, 0.8765941196519880796, 1.000000000000000000 ) ) 
 REPRESENTATION_ITEM ( '' )  );
#39358=VERTEX_POINT ( 'NONE', #40062 ) ;
#39359=ORIENTED_EDGE ( 'NONE', *, *, #13750, .F. ) ;
#39360=CARTESIAN_POINT ( 'NONE',  ( -11.39127492490111315, -11.16067319722467666, 60.69357916181100876 ) ) ;
#39361=ADVANCED_FACE ( 'NONE', ( #10994 ), #47686, .T. ) ;
#39363=CARTESIAN_POINT ( 'NONE',  ( -23.61204160381034711, -11.53669949605622769, 66.42214514747726639 ) ) ;
#39365=CARTESIAN_POINT ( 'NONE',  ( -13.42948644998191732, -8.996466925491649391, 56.85478874482843992 ) ) ;
#39366=FACE_OUTER_BOUND ( 'NONE', #17591, .T. ) ;
#39367=( BOUNDED_SURFACE ( )  B_SPLINE_SURFACE ( 3, 1, ( 
 ( #28346, #43611 ),
 ( #39424, #20711 ),
 ( #9643, #16985 ),
 ( #47051, #5930 ),
 ( #20951, #36659 ),
 ( #44569, #14482 ),
 ( #13775, #25371 ) ),
 .UNSPECIFIED., .T., .F., .F. ) 
 B_SPLINE_SURFACE_WITH_KNOTS ( ( 4, 3, 4 ),
 ( 2, 2 ),
 ( 0.000000000000000000, 0.5000000000000000000, 1.000000000000000000 ),
 ( 0.000000000000000000, 1.000000000000000000 ),
 .UNSPECIFIED. ) 
 GEOMETRIC_REPRESENTATION_ITEM ( )  RATIONAL_B_SPLINE_SURFACE ( (
 ( 1.000000000000000000, 1.000000000000000000),
 ( 0.3333333333333335369, 0.3333333333333330373),
 ( 0.3333333333333335369, 0.3333333333333330373),
 ( 1.000000000000000000, 1.000000000000000000),
 ( 0.3333333333333333703, 0.3333333333333333703),
 ( 0.3333333333333333703, 0.3333333333333333703),
 ( 1.000000000000000000, 1.000000000000000000) ) ) 
 REPRESENTATION_ITEM ( '' )  SURFACE ( )  );
#39369=FACE_OUTER_BOUND ( 'NONE', #31071, .T. ) ;
#39371=CARTESIAN_POINT ( 'NONE',  ( -20.66696806162329025, -21.06910005082376358, 58.79475164909958096 ) ) ;
#39373=ORIENTED_EDGE ( 'NONE', *, *, #15261, .F. ) ;
#39375=CARTESIAN_POINT ( 'NONE',  ( -11.25622321624083355, -18.98904307544693282, 64.86051675911045322 ) ) ;
#39376=( BOUNDED_SURFACE ( )  B_SPLINE_SURFACE ( 3, 1, ( 
 ( #22598, #26292 ),
 ( #41071, #15681 ),
 ( #34390, #22352 ),
 ( #11514, #18399 ),
 ( #45760, #19145 ),
 ( #37595, #48445 ),
 ( #3899, #26536 ) ),
 .UNSPECIFIED., .T., .F., .F. ) 
 B_SPLINE_SURFACE_WITH_KNOTS ( ( 4, 3, 4 ),
 ( 2, 2 ),
 ( 0.000000000000000000, 0.5000000000000000000, 1.000000000000000000 ),
 ( 0.000000000000000000, 1.000000000000000000 ),
 .UNSPECIFIED. ) 
 GEOMETRIC_REPRESENTATION_ITEM ( )  RATIONAL_B_SPLINE_SURFACE ( (
 ( 1.000000000000000000, 1.000000000000000000),
 ( 0.3333333333333335369, 0.3333333333333330373),
 ( 0.3333333333333335369, 0.3333333333333330373),
 ( 1.000000000000000000, 1.000000000000000000),
 ( 0.3333333333333333703, 0.3333333333333333703),
 ( 0.3333333333333333703, 0.3333333333333333703),
 ( 1.000000000000000000, 1.000000000000000000) ) ) 
 REPRESENTATION_ITEM ( '' )  SURFACE ( )  );
#39377=CARTESIAN_POINT ( 'NONE',  ( -21.49816216734858898, -9.116934002111024782, 70.13132539266752019 ) ) ;
#39380=AXIS2_PLACEMENT_3D ( 'NONE', #7091, #33644, #22109 ) ;
#39381=CARTESIAN_POINT ( 'NONE',  ( -22.64171105389675276, -20.12707350008254892, 69.36756280019827159 ) ) ;
#39382=CARTESIAN_POINT ( 'NONE',  ( -18.98647511214439731, -7.985344313229808755, 67.18455284397973060 ) ) ;
#39383=ADVANCED_FACE ( 'NONE', ( #43767 ), #20818, .T. ) ;
#39384=VERTEX_POINT ( 'NONE', #36822 ) ;
#39385=CARTESIAN_POINT ( 'NONE',  ( -23.65719169145585710, -18.88999977852593659, 69.41655123612174805 ) ) ;
#39386=ORIENTED_EDGE ( 'NONE', *, *, #13969, .F. ) ;
#39387=CARTESIAN_POINT ( 'NONE',  ( -17.85728874018076340, -21.84618329174708151, 61.89007996730683203 ) ) ;
#39388=CARTESIAN_POINT ( 'NONE',  ( -21.31115985637654120, -8.927249709250721921, 73.88656608925673197 ) ) ;
#39389=ORIENTED_EDGE ( 'NONE', *, *, #22985, .F. ) ;
#39390=EDGE_CURVE ( 'NONE', #28, #7220, #43305, .T. ) ;
#39393=CARTESIAN_POINT ( 'NONE',  ( -11.42117823542190358, -10.39672530145416829, 74.57738459077027926 ) ) ;
#39394=B_SPLINE_CURVE_WITH_KNOTS ( 'NONE', 1,
 ( #31662, #42509 ),
 .UNSPECIFIED., .F., .F.,
 ( 2, 2 ),
 ( 0.000000000000000000, 1.000000000000000000 ),
 .UNSPECIFIED. ) ;
#39395=ORIENTED_EDGE ( 'NONE', *, *, #21616, .T. ) ;
#39396=CARTESIAN_POINT ( 'NONE',  ( -15.19396558280303822, -21.91766586989539434, 68.61946996636811491 ) ) ;
#39397=CARTESIAN_POINT ( 'NONE',  ( -10.64225270876709217, -11.72539899671273211, 74.75178466342971717 ) ) ;
#39398=CARTESIAN_POINT ( 'NONE',  ( -10.93128702722934698, -17.42536716698162280, 64.70027491337052084 ) ) ;
#39399=ORIENTED_EDGE ( 'NONE', *, *, #14546, .F. ) ;
#39401=CARTESIAN_POINT ( 'NONE',  ( -10.85841931818429629, -17.37798394237199062, 64.91267318220633342 ) ) ;
#39403=VECTOR ( 'NONE', #6112, 1000.000000000000000 ) ;
#39409=CARTESIAN_POINT ( 'NONE',  ( -11.77030184709744454, -18.93651027082609417, 68.32575532107205163 ) ) ;
#39410=ORIENTED_EDGE ( 'NONE', *, *, #5470, .T. ) ;
#39411=CARTESIAN_POINT ( 'NONE',  ( -15.67484944857656082, -7.976566202440097619, 67.02518389757648265 ) ) ;
#39412=CARTESIAN_POINT ( 'NONE',  ( -19.37709741767962157, -21.53135792448401986, 61.99503678469526591 ) ) ;
#39414=ADVANCED_FACE ( 'NONE', ( #10885 ), #43916, .T. ) ;
#39415=CARTESIAN_POINT ( 'NONE',  ( -12.48160889263952811, -19.84176915467957869, 68.63657425450733740 ) ) ;
#39416=CARTESIAN_POINT ( 'NONE',  ( -10.57723003925373106, -17.74759380694297306, 71.75373442408677249 ) ) ;
#39419=ADVANCED_FACE ( 'NONE', ( #40207 ), #21724, .T. ) ;
#39420=CARTESIAN_POINT ( 'NONE',  ( -22.42594789675818845, -19.77792426076253918, 69.45945937764655298 ) ) ;
#39421=CARTESIAN_POINT ( 'NONE',  ( -20.83485745854687821, -8.694536277584232309, 60.03052354408486480 ) ) ;
#39424=CARTESIAN_POINT ( 'NONE',  ( -24.47559319016939483, -14.50700548578266513, 59.39867536442299212 ) ) ;
#39426=EDGE_CURVE ( 'NONE', #27258, #6094, #40921, .T. ) ;
#39427=EDGE_LOOP ( 'NONE', ( #20382, #46572, #44571, #24308, #27805 ) ) ;
#39428=ORIENTED_EDGE ( 'NONE', *, *, #48257, .F. ) ;
#39429=ORIENTED_EDGE ( 'NONE', *, *, #36469, .F. ) ;
#39432=CARTESIAN_POINT ( 'NONE',  ( -12.55198883488284878, -12.25722835735234639, 54.07175714974878389 ) ) ;
#39434=ORIENTED_EDGE ( 'NONE', *, *, #4037, .F. ) ;
#39436=VECTOR ( 'NONE', #38254, 1000.000000000000114 ) ;
#39437=CARTESIAN_POINT ( 'NONE',  ( -22.57893663749957369, -9.999394138389961384, 73.49633153340955971 ) ) ;
#39438=ORIENTED_EDGE ( 'NONE', *, *, #612, .F. ) ;
#39440=CARTESIAN_POINT ( 'NONE',  ( -11.22150886908280931, -18.16670198096008093, 58.22203402163793839 ) ) ;
#39441=DIRECTION ( 'NONE',  ( -0.06306825763707681054, 0.9980092158285026605, 2.415158932891090200E-08 ) ) ;
#39442=VERTEX_POINT ( 'NONE', #25189 ) ;
#39443=CARTESIAN_POINT ( 'NONE',  ( -19.80301227694363675, -21.44571519258606074, 69.08482476707463604 ) ) ;
#39444=EDGE_CURVE ( 'NONE', #3865, #20439, #44167, .T. ) ;
#39445=ORIENTED_EDGE ( 'NONE', *, *, #26722, .T. ) ;
#39447=ORIENTED_EDGE ( 'NONE', *, *, #13871, .T. ) ;
#39448=FACE_OUTER_BOUND ( 'NONE', #42790, .T. ) ;
#39452=CARTESIAN_POINT ( 'NONE',  ( -14.67819097860952482, -7.883573037801185457, 60.44279363819690332 ) ) ;
#39454=CARTESIAN_POINT ( 'NONE',  ( -15.43182990062313564, -8.046249867383863830, 74.36513541778452918 ) ) ;
#39455=CARTESIAN_POINT ( 'NONE',  ( -17.65810221059773610, -7.762793303104816189, 63.56529088875731759 ) ) ;
#39457=ORIENTED_EDGE ( 'NONE', *, *, #14859, .F. ) ;
#39458=CARTESIAN_POINT ( 'NONE',  ( -17.55068613527580723, -7.810228624652221896, 63.85057029484593727 ) ) ;
#39459=CARTESIAN_POINT ( 'NONE',  ( -24.66123687018043498, -13.04105289088702158, 63.03275384083246990 ) ) ;
#39464=AXIS2_PLACEMENT_3D ( 'NONE', #25883, #7427, #30083 ) ;
#39465=EDGE_LOOP ( 'NONE', ( #12682, #34945, #25739, #35341, #28725 ) ) ;
#39466=ADVANCED_FACE ( 'NONE', ( #6951 ), #10168, .T. ) ;
#39467=CARTESIAN_POINT ( 'NONE',  ( -20.95545100651803594, -20.91135505560678709, 65.59926067308570907 ) ) ;
#39470=CARTESIAN_POINT ( 'NONE',  ( -16.71957921250844592, -21.82421608262117729, 68.71032757591046902 ) ) ;
#39471=CARTESIAN_POINT ( 'NONE',  ( -10.66160605790631344, -13.00123564105898666, 68.03832347539896830 ) ) ;
#39472=CARTESIAN_POINT ( 'NONE',  ( -14.55661340756572741, -8.423408737790397893, 64.07513534474681194 ) ) ;
#39473=CARTESIAN_POINT ( 'NONE',  ( -19.44376822123183146, -7.638105259791415413, 60.07597700946195829 ) ) ;
#39475=CARTESIAN_POINT ( 'NONE',  ( -10.90323534495222546, -12.10858216263579124, 57.47290069719868910 ) ) ;
#39476=VERTEX_POINT ( 'NONE', #2762 ) ;
#39477=B_SPLINE_CURVE_WITH_KNOTS ( 'NONE', 3,
 ( #40574, #10787, #44787, #6854, #25809, #22358, #40826, #7111, #30975, #8565 ),
 .UNSPECIFIED., .F., .F.,
 ( 4, 2, 2, 2, 4 ),
 ( 0.000000000000000000, 0.2500000000000000000, 0.5000000000000000000, 0.7500000000000000000, 1.000000000000000000 ),
 .UNSPECIFIED. ) ;
#39479=DIRECTION ( 'NONE',  ( 9.593247862241308766E-06, 5.650837229295286289E-06, -0.9999999999380186910 ) ) ;
#39480=EDGE_CURVE ( 'NONE', #12385, #17470, #35893, .T. ) ;
#39481=CARTESIAN_POINT ( 'NONE',  ( -22.11801487708262215, -20.07437006378957989, 58.76442739134373028 ) ) ;
#39482=VERTEX_POINT ( 'NONE', #41167 ) ;
#39484=ADVANCED_FACE ( 'NONE', ( #32566 ), #33027, .T. ) ;
#39485=CARTESIAN_POINT ( 'NONE',  ( -10.41686238704247103, -12.27912473904753021, 57.52868529117814234 ) ) ;
#39486=CARTESIAN_POINT ( 'NONE',  ( -24.30998853687411554, -13.26019858907717897, 66.44679832887018733 ) ) ;
#39487=CARTESIAN_POINT ( 'NONE',  ( -10.93244803288776090, -12.03909807633519513, 71.24428013274216198 ) ) ;
#39490=ORIENTED_EDGE ( 'NONE', *, *, #14910, .F. ) ;
#39493=CARTESIAN_POINT ( 'NONE',  ( -14.10937626179043924, -8.137098231162246620, 70.85240724826557823 ) ) ;
#39494=EDGE_CURVE ( 'NONE', #4523, #4476, #14462, .T. ) ;
#39496=DIRECTION ( 'NONE',  ( -0.9410372374137779827, -0.3383029970317210644, -1.029646047569396398E-09 ) ) ;
#39498=CARTESIAN_POINT ( 'NONE',  ( -12.05806040642128707, -10.23620046216302448, 67.51368956197082127 ) ) ;
#39500=DIRECTION ( 'NONE',  ( 3.840743001415272461E-07, -4.934726759164745929E-06, 0.9999999999877503543 ) ) ;
#39501=CARTESIAN_POINT ( 'NONE',  ( -18.19389323530821301, -22.21941482433020809, 65.53027461949925225 ) ) ;
#39502=VERTEX_POINT ( 'NONE', #57 ) ;
#39503=( BOUNDED_CURVE ( )  B_SPLINE_CURVE ( 3, ( #7795, #7542, #34105, #6799 ),
 .UNSPECIFIED., .F., .F. ) 
 B_SPLINE_CURVE_WITH_KNOTS ( ( 4, 4 ),
 ( 0.4074455897393655657, 0.5000000000000000000 ),
 .UNSPECIFIED. ) 
 CURVE ( )  GEOMETRIC_REPRESENTATION_ITEM ( )  RATIONAL_B_SPLINE_CURVE ( ( 0.6983129098260920653, 0.7760317562606952047, 0.8765941196519972944, 0.9999999999999966693 ) ) 
 REPRESENTATION_ITEM ( '' )  );
#39504=CARTESIAN_POINT ( 'NONE',  ( -24.41687585340592648, -14.48898466279928954, 66.48292730085977098 ) ) ;
#39505=CARTESIAN_POINT ( 'NONE',  ( -12.94846201263913521, -9.425283042519069454, 74.39093336797685652 ) ) ;
#39506=VERTEX_POINT ( 'NONE', #18754 ) ;
#39507=CARTESIAN_POINT ( 'NONE',  ( -20.54979434103954361, -8.489990112051950533, 63.61121512946457557 ) ) ;
#39508=CARTESIAN_POINT ( 'NONE',  ( -18.57780522812731050, -21.71353757645834648, 72.30013330437641628 ) ) ;
#39509=ORIENTED_EDGE ( 'NONE', *, *, #12475, .F. ) ;
#39511=CARTESIAN_POINT ( 'NONE',  ( -22.68646480449111635, -20.08284195570847430, 69.35913425646373298 ) ) ;
#39513=CARTESIAN_POINT ( 'NONE',  ( -10.89280197141400919, -11.22507430941316642, 64.33377434530349603 ) ) ;
#39516=FACE_OUTER_BOUND ( 'NONE', #2287, .T. ) ;
#39517=CARTESIAN_POINT ( 'NONE',  ( -24.53780083649505173, -12.59584922708229904, 69.95738295622972203 ) ) ;
#39518=( BOUNDED_CURVE ( )  B_SPLINE_CURVE ( 3, ( #30755, #22624, #41835, #234 ),
 .UNSPECIFIED., .F., .F. ) 
 B_SPLINE_CURVE_WITH_KNOTS ( ( 4, 4 ),
 ( 0.4074455897393584602, 0.5000000000000000000 ),
 .UNSPECIFIED. ) 
 CURVE ( )  GEOMETRIC_REPRESENTATION_ITEM ( )  RATIONAL_B_SPLINE_CURVE ( ( 0.6983129098260868473, 0.7760317562606771080, 0.8765941196519766443, 0.9999999999999747979 ) ) 
 REPRESENTATION_ITEM ( '' )  );
#39519=CARTESIAN_POINT ( 'NONE',  ( -11.96181355942711910, -19.87549434724351727, 58.11177690156993947 ) ) ;
#39520=FACE_OUTER_BOUND ( 'NONE', #4143, .T. ) ;
#39521=CARTESIAN_POINT ( 'NONE',  ( -11.47771180081793574, -11.11285131991801478, 60.78958965739695230 ) ) ;
#39522=CARTESIAN_POINT ( 'NONE',  ( -16.45013838383832550, -21.79965580723203189, 68.83993634381745608 ) ) ;
#39523=ORIENTED_EDGE ( 'NONE', *, *, #39017, .F. ) ;
#39524=CARTESIAN_POINT ( 'NONE',  ( -10.45863951484398946, -14.11462368554138536, 60.91821294131582931 ) ) ;
#39525=CARTESIAN_POINT ( 'NONE',  ( -14.30213453930070244, -8.044712385003874644, 67.39941695810342992 ) ) ;
#39526=CARTESIAN_POINT ( 'NONE',  ( -21.35673258969864818, -10.96416394607318878, 53.49999999999995026 ) ) ;
#39530=VERTEX_POINT ( 'NONE', #19248 ) ;
#39533=EDGE_CURVE ( 'NONE', #15132, #6650, #4474, .T. ) ;
#39534=CARTESIAN_POINT ( 'NONE',  ( -15.46331485788676297, -8.033501021233417916, 70.60989570331041421 ) ) ;
#39535=CARTESIAN_POINT ( 'NONE',  ( -23.11919465953077690, -18.88152036183635119, 65.89559798510001087 ) ) ;
#39536=CARTESIAN_POINT ( 'NONE',  ( -17.43865353846181421, -7.359098165012483150, 67.19852322307089310 ) ) ;
#39537=CARTESIAN_POINT ( 'NONE',  ( -17.05968203966123298, -22.25103879409192231, 72.27887915399999486 ) ) ;
#39538=CARTESIAN_POINT ( 'NONE',  ( -22.91296630721855720, -15.15889098507616950, 54.07175714974879099 ) ) ;
#39540=VERTEX_POINT ( 'NONE', #45127 ) ;
#39542=CARTESIAN_POINT ( 'NONE',  ( -12.26902364965855519, -19.54473725125994221, 57.92682373989410394 ) ) ;
#39543=CARTESIAN_POINT ( 'NONE',  ( -16.58751095051766100, -21.80939428823196025, 65.22564390318967753 ) ) ;
#39547=EDGE_CURVE ( 'NONE', #21025, #45248, #20542, .T. ) ;
#39549=CARTESIAN_POINT ( 'NONE',  ( -24.06787342886325121, -18.28917680027896608, 47.99999999999994316 ) ) ;
#39551=PLANE ( 'NONE',  #4865 ) ;
#39552=DIRECTION ( 'NONE',  ( 3.549360974554993999E-17, -6.371834667797928663E-18, -1.000000000000000000 ) ) ;
#39553=EDGE_LOOP ( 'NONE', ( #27371, #19988, #30562, #5268, #37872 ) ) ;
#39554=DIRECTION ( 'NONE',  ( -0.7300417127692488961, -0.6834025882427879894, -6.612978995310452690E-09 ) ) ;
#39555=B_SPLINE_CURVE_WITH_KNOTS ( 'NONE', 1,
 ( #34524, #26418 ),
 .UNSPECIFIED., .F., .F.,
 ( 2, 2 ),
 ( 0.000000000000000000, 1.000000000000000000 ),
 .UNSPECIFIED. ) ;
#39556=B_SPLINE_CURVE_WITH_KNOTS ( 'NONE', 3,
 ( #37723, #19263, #34266, #554, #45631, #26909, #23213, #19501, #35716, #8680 ),
 .UNSPECIFIED., .F., .F.,
 ( 4, 2, 2, 2, 4 ),
 ( 0.000000000000000000, 0.2500000000000000000, 0.5000000000000000000, 0.7500000000000000000, 1.000000000000000000 ),
 .UNSPECIFIED. ) ;
#39561=ORIENTED_EDGE ( 'NONE', *, *, #25495, .F. ) ;
#39562=CYLINDRICAL_SURFACE ( 'NONE', #21071, 0.1499999999999956923 ) ;
#39563=CARTESIAN_POINT ( 'NONE',  ( -22.85826336087821176, -10.39655209224729226, 63.37185958068533864 ) ) ;
#39565=ORIENTED_EDGE ( 'NONE', *, *, #19567, .T. ) ;
#39566=CARTESIAN_POINT ( 'NONE',  ( -24.43113031232903865, -15.58634216689856622, 73.30303748141028564 ) ) ;
#39567=ORIENTED_EDGE ( 'NONE', *, *, #37330, .F. ) ;
#39568=CARTESIAN_POINT ( 'NONE',  ( -14.77890319739905145, -21.35274797201484276, 65.25029445929627059 ) ) ;
#39569=DIRECTION ( 'NONE',  ( 1.206829990107966821E-05, 1.995688255855010801E-06, 0.9999999999251867333 ) ) ;
#39570=ORIENTED_EDGE ( 'NONE', *, *, #4077, .T. ) ;
#39571=CARTESIAN_POINT ( 'NONE',  ( -18.68070144837527735, -7.415226739706411330, 54.27966884056654351 ) ) ;
#39573=EDGE_CURVE ( 'NONE', #34284, #11137, #34497, .T. ) ;
#39574=CARTESIAN_POINT ( 'NONE',  ( -16.79871736827016449, -7.783984993247369921, 73.84529564069914898 ) ) ;
#39575=DIRECTION ( 'NONE',  ( 3.549360974554993999E-17, -6.371834667797928663E-18, -1.000000000000000000 ) ) ;
#39577=CARTESIAN_POINT ( 'NONE',  ( -10.46253608402116519, -14.07554757472905571, 60.91821325758270689 ) ) ;
#39580=ORIENTED_EDGE ( 'NONE', *, *, #32645, .F. ) ;
#39582=DIRECTION ( 'NONE',  ( 5.517078692044801135E-07, 1.257343604232908019E-06, 0.9999999999990574207 ) ) ;
#39584=ORIENTED_EDGE ( 'NONE', *, *, #30149, .T. ) ;
#39585=CARTESIAN_POINT ( 'NONE',  ( -14.78518025053764440, -21.29286684132125984, 58.16617891046453082 ) ) ;
#39586=CARTESIAN_POINT ( 'NONE',  ( -23.22909885928854834, -6.086929677699679075, 53.49999999999995026 ) ) ;
#39588=CARTESIAN_POINT ( 'NONE',  ( -13.55325570056783491, -20.70509005021970594, 57.93161203092463296 ) ) ;
#39590=CARTESIAN_POINT ( 'NONE',  ( -24.45201643071094111, -14.25170847814747077, 69.65275273439885950 ) ) ;
#39591=B_SPLINE_CURVE_WITH_KNOTS ( 'NONE', 3,
 ( #27455, #19335, #34344, #23535, #31147, #45711, #31646, #24022, #16361, #23287 ),
 .UNSPECIFIED., .F., .F.,
 ( 4, 2, 2, 2, 4 ),
 ( 0.6272669072977269389, 0.7522669073147544294, 0.8772669073317820310, 1.002266907348809521, 1.127266907365837012 ),
 .UNSPECIFIED. ) ;
#39592=CARTESIAN_POINT ( 'NONE',  ( -19.55776627226465791, -21.47609803464143852, 62.10389610901621182 ) ) ;
#39593=DIRECTION ( 'NONE',  ( 0.3111098983483954195, 0.8385765505603234304, -0.4472135954999584273 ) ) ;
#39598=CARTESIAN_POINT ( 'NONE',  ( -10.91133513969588087, -12.10202850713728218, 74.44351760842475585 ) ) ;
#39600=AXIS2_PLACEMENT_3D ( 'NONE', #44363, #40640, #43638 ) ;
#39602=CARTESIAN_POINT ( 'NONE',  ( -11.40217217410143391, -18.47541073860962513, 61.28270649782702151 ) ) ;
#39607=EDGE_CURVE ( 'NONE', #14112, #10001, #22394, .T. ) ;
#39611=CARTESIAN_POINT ( 'NONE',  ( -14.97837282748989729, -8.193824179639600302, 60.73484884663594130 ) ) ;
#39612=CARTESIAN_POINT ( 'NONE',  ( -11.17472172325445356, -18.86502640884145876, 64.92519864151283571 ) ) ;
#39613=VERTEX_POINT ( 'NONE', #4720 ) ;
#39614=CARTESIAN_POINT ( 'NONE',  ( -11.34829033918305718, -18.40080557649748272, 64.89140246238697785 ) ) ;
#39615=ADVANCED_FACE ( 'NONE', ( #4466 ), #19742, .T. ) ;
#39616=EDGE_CURVE ( 'NONE', #23182, #1656, #44434, .T. ) ;
#39617=CARTESIAN_POINT ( 'NONE',  ( -13.65828898514496537, -20.76952646431350757, 65.00101022825411690 ) ) ;
#39618=CARTESIAN_POINT ( 'NONE',  ( -22.53429319464570924, -9.952421322533329118, 73.48161091678163359 ) ) ;
#39619=CARTESIAN_POINT ( 'NONE',  ( -18.52416312356643147, -7.896186446804856374, 73.84064402154488960 ) ) ;
#39620=DIRECTION ( 'NONE',  ( -0.4780674886490096087, 0.8783231047267435754, 5.292596395488305015E-08 ) ) ;
#39621=CARTESIAN_POINT ( 'NONE',  ( -14.84568658978198563, -7.819606672530345470, 56.95025746631047525 ) ) ;
#39622=DIRECTION ( 'NONE',  ( -1.077913161506870186E-05, 7.121115479698836302E-06, 0.9999999999165498643 ) ) ;
#39624=CARTESIAN_POINT ( 'NONE',  ( -15.49415903819706486, -8.028509590827587417, 74.22985659018391402 ) ) ;
#39625=VERTEX_POINT ( 'NONE', #47478 ) ;
#39627=CARTESIAN_POINT ( 'NONE',  ( -21.71080454141873517, -9.207639020309585476, 70.22312793020654453 ) ) ;
#39628=CARTESIAN_POINT ( 'NONE',  ( -17.81164871297510643, -7.369293837194203611, 60.23060767647208280 ) ) ;
#39629=ORIENTED_EDGE ( 'NONE', *, *, #26456, .F. ) ;
#39630=CARTESIAN_POINT ( 'NONE',  ( -13.65769536888696223, -21.23707814910688541, 68.56350999071767660 ) ) ;
#39631=EDGE_CURVE ( 'NONE', #21822, #12832, #34317, .T. ) ;
#39633=EDGE_LOOP ( 'NONE', ( #18046, #10037, #11253, #46920, #16431 ) ) ;
#39634=CARTESIAN_POINT ( 'NONE',  ( -15.12888584993918428, -21.89692032561032775, 68.83238837976321634 ) ) ;
#39635=( BOUNDED_CURVE ( )  B_SPLINE_CURVE ( 3, ( #45355, #22451, #23188, #15035 ),
 .UNSPECIFIED., .F., .F. ) 
 B_SPLINE_CURVE_WITH_KNOTS ( ( 4, 4 ),
 ( 0.5000000000000000000, 0.9074455897393626236 ),
 .UNSPECIFIED. ) 
 CURVE ( )  GEOMETRIC_REPRESENTATION_ITEM ( )  RATIONAL_B_SPLINE_CURVE ( ( 1.000000000000005107, 0.4567392136813230308, 0.3561768502900233835, 0.6983129098261116052 ) ) 
 REPRESENTATION_ITEM ( '' )  );
#39636=CARTESIAN_POINT ( 'NONE',  ( -17.65810221059773610, -7.762793303104816189, 63.56529088875731759 ) ) ;
#39638=VERTEX_POINT ( 'NONE', #32214 ) ;
#39641=CARTESIAN_POINT ( 'NONE',  ( -23.91010245674826251, -17.57297063409389537, 62.75888927877479517 ) ) ;
#39642=CARTESIAN_POINT ( 'NONE',  ( -12.99758137947571157, -9.386477775907486887, 71.14925353122600882 ) ) ;
#39644=EDGE_LOOP ( 'NONE', ( #11708, #25174, #30710, #41139, #30747 ) ) ;
#39646=CARTESIAN_POINT ( 'NONE',  ( -24.30680323434813062, -16.08559572138876703, 62.87863259089944279 ) ) ;
#39647=EDGE_LOOP ( 'NONE', ( #7967, #37721 ) ) ;
#39648=CARTESIAN_POINT ( 'NONE',  ( -15.75283698213507755, -7.548994588147243334, 67.32502552484606895 ) ) ;
#39651=DIRECTION ( 'NONE',  ( 0.1539336739619741601, 0.9880811829098680166, 6.607022902453645889E-08 ) ) ;
#39653=CARTESIAN_POINT ( 'NONE',  ( -15.68875476689939852, -7.563362019294005201, 70.79645224690898431 ) ) ;
#39654=B_SPLINE_CURVE_WITH_KNOTS ( 'NONE', 3,
 ( #34202, #33966, #30302, #495, #4419, #46281, #45565, #23150, #22915, #11820, #19196, #23382 ),
 .UNSPECIFIED., .F., .F.,
 ( 4, 2, 2, 2, 2, 4 ),
 ( 0.1735808155647264317, 0.3368604174146633268, 0.5001400192646002774, 0.6634196211145371169, 0.7450594220395003742, 0.8266992229644638535 ),
 .UNSPECIFIED. ) ;
#39655=( BOUNDED_SURFACE ( )  B_SPLINE_SURFACE ( 3, 1, ( 
 ( #44211, #32613 ),
 ( #40256, #47875 ),
 ( #29403, #10460 ),
 ( #32838, #18059 ),
 ( #25467, #39758 ),
 ( #44680, #6520 ),
 ( #21771, #40720 ) ),
 .UNSPECIFIED., .T., .F., .F. ) 
 B_SPLINE_SURFACE_WITH_KNOTS ( ( 4, 3, 4 ),
 ( 2, 2 ),
 ( 0.000000000000000000, 0.5000000000000000000, 1.000000000000000000 ),
 ( 0.000000000000000000, 1.000000000000000000 ),
 .UNSPECIFIED. ) 
 GEOMETRIC_REPRESENTATION_ITEM ( )  RATIONAL_B_SPLINE_SURFACE ( (
 ( 1.000000000000000000, 1.000000000000000000),
 ( 0.3333333333333335369, 0.3333333333333330373),
 ( 0.3333333333333335369, 0.3333333333333330373),
 ( 1.000000000000000000, 1.000000000000000000),
 ( 0.3333333333333333703, 0.3333333333333333703),
 ( 0.3333333333333333703, 0.3333333333333333703),
 ( 1.000000000000000000, 1.000000000000000000) ) ) 
 REPRESENTATION_ITEM ( '' )  SURFACE ( )  );
#39656=ORIENTED_EDGE ( 'NONE', *, *, #20054, .T. ) ;
#39657=CARTESIAN_POINT ( 'NONE',  ( -22.83929682888979329, -10.29453308790037980, 66.55654356380499337 ) ) ;
#39658=CARTESIAN_POINT ( 'NONE',  ( -19.24035349434955577, -7.583912967164861740, 63.68735177183580021 ) ) ;
#39659=CARTESIAN_POINT ( 'NONE',  ( -12.52591726580351228, -9.195683270288645517, 74.50418291613799227 ) ) ;
#39660=CARTESIAN_POINT ( 'NONE',  ( -11.16720114480400383, -11.56054632708127627, 67.61864607954859707 ) ) ;
#39661=VERTEX_POINT ( 'NONE', #20885 ) ;
#39662=( BOUNDED_CURVE ( )  B_SPLINE_CURVE ( 3, ( #28363, #32299, #2005, #12842 ),
 .UNSPECIFIED., .F., .F. ) 
 B_SPLINE_CURVE_WITH_KNOTS ( ( 4, 4 ),
 ( 1.570796326794896780, 1.780235837034217727 ),
 .UNSPECIFIED. ) 
 CURVE ( )  GEOMETRIC_REPRESENTATION_ITEM ( )  RATIONAL_B_SPLINE_CURVE ( ( 1.000000000000000000, 0.9963479302455154896, 0.9963479302455154896, 1.000000000000000000 ) ) 
 REPRESENTATION_ITEM ( '' )  );
#39664=ORIENTED_EDGE ( 'NONE', *, *, #46911, .F. ) ;
#39665=EDGE_CURVE ( 'NONE', #45314, #32695, #33220, .T. ) ;
#39666=CARTESIAN_POINT ( 'NONE',  ( -10.88210962122359504, -12.31514282983516750, 57.55687129713847128 ) ) ;
#39671=EDGE_CURVE ( 'NONE', #13315, #10765, #9170, .T. ) ;
#39672=FACE_OUTER_BOUND ( 'NONE', #27637, .T. ) ;
#39673=ORIENTED_EDGE ( 'NONE', *, *, #48669, .T. ) ;
#39674=ADVANCED_FACE ( 'NONE', ( #16254 ), #25551, .T. ) ;
#39675=CARTESIAN_POINT ( 'NONE',  ( -10.96069698787312596, -18.51437578577013809, 57.92219301334858272 ) ) ;
#39676=CARTESIAN_POINT ( 'NONE',  ( -17.76877443916874810, -21.80232427043311816, 62.06462945740774018 ) ) ;
#39677=ADVANCED_FACE ( 'NONE', ( #21611 ), #9577, .T. ) ;
#39680=ORIENTED_EDGE ( 'NONE', *, *, #32517, .F. ) ;
#39681=CARTESIAN_POINT ( 'NONE',  ( -13.51337628678458636, -21.15025853544303303, 65.08605242239845268 ) ) ;
#39682=ORIENTED_EDGE ( 'NONE', *, *, #36604, .T. ) ;
#39683=CARTESIAN_POINT ( 'NONE',  ( -11.94538260508191385, -19.85760771564406113, 58.12671156609361134 ) ) ;
#39685=CARTESIAN_POINT ( 'NONE',  ( -19.37616744185158879, -21.99900390342548206, 58.71002665166666645 ) ) ;
#39686=B_SPLINE_CURVE_WITH_KNOTS ( 'NONE', 1,
 ( #30356, #45366 ),
 .UNSPECIFIED., .F., .F.,
 ( 2, 2 ),
 ( 0.000000000000000000, 1.000000000000000000 ),
 .UNSPECIFIED. ) ;
#39687=ORIENTED_EDGE ( 'NONE', *, *, #30238, .T. ) ;
#39690=B_SPLINE_CURVE_WITH_KNOTS ( 'NONE', 1,
 ( #46799, #20462 ),
 .UNSPECIFIED., .F., .F.,
 ( 2, 2 ),
 ( 0.000000000000000000, 1.000000000000000000 ),
 .UNSPECIFIED. ) ;
#39694=CARTESIAN_POINT ( 'NONE',  ( -19.14405459605125515, -8.023800501541026975, 60.15196141296932808 ) ) ;
#39698=DIRECTION ( 'NONE',  ( -0.2466764125338440639, -0.9690979039805150963, 7.162324212089591066E-08 ) ) ;
#39700=CARTESIAN_POINT ( 'NONE',  ( -13.24006525392636391, -20.97423447465198976, 61.70301720779925603 ) ) ;
#39704=ORIENTED_EDGE ( 'NONE', *, *, #46856, .F. ) ;
#39705=CARTESIAN_POINT ( 'NONE',  ( -21.30572535954460633, -21.16897061578360351, 65.69798576082847319 ) ) ;
#39706=CARTESIAN_POINT ( 'NONE',  ( -24.40844971322602319, -15.79084262311724629, 73.41792560911460441 ) ) ;
#39707=ORIENTED_EDGE ( 'NONE', *, *, #3689, .T. ) ;
#39708=CARTESIAN_POINT ( 'NONE',  ( -9.974481508125691676, -14.72588544478808181, 71.37136786695171509 ) ) ;
#39710=CARTESIAN_POINT ( 'NONE',  ( -14.49033176393974109, -8.453654632373657662, 63.89864959097710084 ) ) ;
#39711=CARTESIAN_POINT ( 'NONE',  ( -13.65828898514496359, -20.76952646431350757, 65.00101022825411690 ) ) ;
#39712=CARTESIAN_POINT ( 'NONE',  ( -10.40127108354264429, -12.32249413655887871, 57.51352655450988749 ) ) ;
#39713=VERTEX_POINT ( 'NONE', #36596 ) ;
#39714=B_SPLINE_CURVE_WITH_KNOTS ( 'NONE', 3,
 ( #41655, #22709, #15040, #7694, #4966, #7941, #15523, #26387, #23430, #19003 ),
 .UNSPECIFIED., .F., .F.,
 ( 4, 2, 2, 2, 4 ),
 ( 0.000000000000000000, 0.2500000000000000000, 0.5000000000000000000, 0.7500000000000000000, 1.000000000000000000 ),
 .UNSPECIFIED. ) ;
#39715=B_SPLINE_CURVE_WITH_KNOTS ( 'NONE', 3,
 ( #41052, #7336, #26036, #21845, #3878, #15169, #7082, #33386, #22840, #22095 ),
 .UNSPECIFIED., .F., .F.,
 ( 4, 2, 2, 2, 4 ),
 ( 0.1272669073658152239, 0.2522669073463065237, 0.3772669073267979067, 0.5022669073072891788, 0.6272669072877805618 ),
 .UNSPECIFIED. ) ;
#39717=CARTESIAN_POINT ( 'NONE',  ( -17.20949509180255887, -7.759470163990226155, 74.37506982372057962 ) ) ;
#39720=LINE ( 'NONE', #48075, #30610 ) ;
#39722=DIRECTION ( 'NONE',  ( -0.7364384864160969935, 0.6765045127160409510, 1.031360481960658298E-08 ) ) ;
#39723=CARTESIAN_POINT ( 'NONE',  ( -22.54890198535468571, -19.65079054415343052, 72.93840789290602800 ) ) ;
#39724=EDGE_CURVE ( 'NONE', #13505, #34212, #29157, .T. ) ;
#39725=CARTESIAN_POINT ( 'NONE',  ( -11.05034076241727625, -11.79557573020262318, 71.37388789199357575 ) ) ;
#39726=CYLINDRICAL_SURFACE ( 'NONE', #1596, 0.1500000000000017153 ) ;
#39728=ORIENTED_EDGE ( 'NONE', *, *, #30189, .T. ) ;
#39730=CARTESIAN_POINT ( 'NONE',  ( -14.91112529534803066, -8.221969756899694559, 57.13527940342243028 ) ) ;
#39731=CARTESIAN_POINT ( 'NONE',  ( -15.35027142736847239, -7.653576728715946409, 74.26480947788739684 ) ) ;
#39732=B_SPLINE_CURVE_WITH_KNOTS ( 'NONE', 1,
 ( #39919, #20731 ),
 .UNSPECIFIED., .F., .F.,
 ( 2, 2 ),
 ( 0.000000000000000000, 1.000000000000000000 ),
 .UNSPECIFIED. ) ;
#39733=B_SPLINE_CURVE_WITH_KNOTS ( 'NONE', 3,
 ( #22588, #34380, #29733, #33394, #44768, #11019, #37843, #33906, #22340, #26281 ),
 .UNSPECIFIED., .F., .F.,
 ( 4, 2, 2, 2, 4 ),
 ( 0.000000000000000000, 0.2500000000000000000, 0.5000000000000000000, 0.7500000000000000000, 1.000000000000000000 ),
 .UNSPECIFIED. ) ;
#39734=CARTESIAN_POINT ( 'NONE',  ( -14.15287076785618403, -8.620510619550140419, 70.95631002325610837 ) ) ;
#39735=DIRECTION ( 'NONE',  ( -0.8037372918934696520, 0.5949843406508664723, 7.322964617522835370E-08 ) ) ;
#39736=ORIENTED_EDGE ( 'NONE', *, *, #2044, .T. ) ;
#39737=EDGE_CURVE ( 'NONE', #38388, #12632, #42874, .T. ) ;
#39738=CARTESIAN_POINT ( 'NONE',  ( -19.29969712032438522, -22.01937259328346741, 58.64790515966043216 ) ) ;
#39739=DIRECTION ( 'NONE',  ( -0.7800143876985551339, 0.6257615799833393666, -5.505484598862901566E-08 ) ) ;
#39740=ADVANCED_FACE ( 'NONE', ( #37835 ), #4129, .T. ) ;
#39742=CARTESIAN_POINT ( 'NONE',  ( -11.32469277870022850, -18.34471304272907588, 58.10714594244493725 ) ) ;
#39743=CARTESIAN_POINT ( 'NONE',  ( -12.87691244601553819, -9.487112660658324259, 74.31923044616551977 ) ) ;
#39744=ORIENTED_EDGE ( 'NONE', *, *, #17217, .T. ) ;
#39745=EDGE_CURVE ( 'NONE', #15007, #2827, #39715, .T. ) ;
#39747=CARTESIAN_POINT ( 'NONE',  ( -12.17848440243300523, -19.44617680680578786, 57.99852596820085182 ) ) ;
#39749=CARTESIAN_POINT ( 'NONE',  ( -23.91467064781584995, -17.58181910956628613, 69.55772506159280510 ) ) ;
#39750=ADVANCED_FACE ( 'NONE', ( #22579 ), #47280, .T. ) ;
#39752=CARTESIAN_POINT ( 'NONE',  ( -22.58346115289088729, -19.54005522229931202, 72.75286664271261827 ) ) ;
#39754=CARTESIAN_POINT ( 'NONE',  ( -22.06352460594304787, -8.980016202103444201, 63.37649054182217867 ) ) ;
#39755=ADVANCED_FACE ( 'NONE', ( #3371 ), #11012, .T. ) ;
#39756=CARTESIAN_POINT ( 'NONE',  ( -11.91452160938943550, -19.82401263394628543, 58.18328287794685139 ) ) ;
#39757=CARTESIAN_POINT ( 'NONE',  ( -23.77562434277295367, -17.86939608417919345, 59.01850491586762359 ) ) ;
#39758=CARTESIAN_POINT ( 'NONE',  ( -11.51414000101334345, -10.27201461766008350, 74.62540520127058130 ) ) ;
#39759=CARTESIAN_POINT ( 'NONE',  ( -16.23115966991289127, -7.455249367085269974, 60.31533194998537084 ) ) ;
#39765=EDGE_LOOP ( 'NONE', ( #8590, #16163, #24069, #44229 ) ) ;
#39766=DIRECTION ( 'NONE',  ( -0.8960627639203775363, 0.4439273849576907960, 5.674307174482189006E-17 ) ) ;
#39767=VECTOR ( 'NONE', #44396, 1000.000000000000114 ) ;
#39769=EDGE_LOOP ( 'NONE', ( #27280, #12949, #42920, #39157, #43430 ) ) ;
#39772=CARTESIAN_POINT ( 'NONE',  ( -18.78856086716502816, -7.485212962163699579, 70.47044390587494433 ) ) ;
#39773=CARTESIAN_POINT ( 'NONE',  ( -23.15062744802226291, -18.83573658997407207, 65.84006125137906906 ) ) ;
#39774=ADVANCED_FACE ( 'NONE', ( #36840 ), #33634, .T. ) ;
#39777=CARTESIAN_POINT ( 'NONE',  ( -10.72958719098378744, -16.85608497040940534, 57.97144002984030209 ) ) ;
#39778=EDGE_LOOP ( 'NONE', ( #18901, #7686, #27422, #41521, #21447 ) ) ;
#39779=ORIENTED_EDGE ( 'NONE', *, *, #47253, .T. ) ;
#39781=CARTESIAN_POINT ( 'NONE',  ( -20.78451513435706133, -21.00713107796517320, 62.12943504870421663 ) ) ;
#39782=CARTESIAN_POINT ( 'NONE',  ( -23.37999588001404661, -18.58199455739222827, 69.57899840282863124 ) ) ;
#39783=( BOUNDED_SURFACE ( )  B_SPLINE_SURFACE ( 3, 1, ( 
 ( #9122, #8884 ),
 ( #38905, #5185 ),
 ( #39144, #31524 ),
 ( #24388, #20924 ),
 ( #46560, #20449 ),
 ( #35448, #16724 ),
 ( #31766, #13033 ) ),
 .UNSPECIFIED., .T., .F., .F. ) 
 B_SPLINE_SURFACE_WITH_KNOTS ( ( 4, 3, 4 ),
 ( 2, 2 ),
 ( 0.000000000000000000, 0.5000000000000000000, 1.000000000000000000 ),
 ( 0.000000000000000000, 1.000000000000000000 ),
 .UNSPECIFIED. ) 
 GEOMETRIC_REPRESENTATION_ITEM ( )  RATIONAL_B_SPLINE_SURFACE ( (
 ( 1.000000000000000000, 1.000000000000000000),
 ( 0.3333333333333335369, 0.3333333333333330373),
 ( 0.3333333333333335369, 0.3333333333333330373),
 ( 1.000000000000000000, 1.000000000000000000),
 ( 0.3333333333333333703, 0.3333333333333333703),
 ( 0.3333333333333333703, 0.3333333333333333703),
 ( 1.000000000000000000, 1.000000000000000000) ) ) 
 REPRESENTATION_ITEM ( '' )  SURFACE ( )  );
#39785=EDGE_CURVE ( 'NONE', #10750, #46952, #24000, .T. ) ;
#39787=CARTESIAN_POINT ( 'NONE',  ( -24.37447228737878291, -15.64171875516282384, 69.60595450079478042 ) ) ;
#39788=CARTESIAN_POINT ( 'NONE',  ( -22.12663539644009703, -20.06189125452669586, 62.52879380229166628 ) ) ;
#39789=ORIENTED_EDGE ( 'NONE', *, *, #29500, .T. ) ;
#39790=CARTESIAN_POINT ( 'NONE',  ( -23.08260857892799578, -18.93003297495478776, 62.35406880915004280 ) ) ;
#39791=B_SPLINE_CURVE_WITH_KNOTS ( 'NONE', 3,
 ( #43896, #2516, #37186, #3471, #21707, #40187, #10867, #17520, #36946, #32548 ),
 .UNSPECIFIED., .F., .F.,
 ( 4, 2, 2, 2, 4 ),
 ( 0.6272669072878258589, 0.7522669073073262602, 0.8772669073268266615, 1.002266907346327063, 1.127266907365827464 ),
 .UNSPECIFIED. ) ;
#39792=( BOUNDED_CURVE ( )  B_SPLINE_CURVE ( 3, ( #19033, #18785, #42175, #26671 ),
 .UNSPECIFIED., .F., .F. ) 
 B_SPLINE_CURVE_WITH_KNOTS ( ( 4, 4 ),
 ( 0.4074455897393750581, 0.5000000000000000000 ),
 .UNSPECIFIED. ) 
 CURVE ( )  GEOMETRIC_REPRESENTATION_ITEM ( )  RATIONAL_B_SPLINE_CURVE ( ( 0.6983129098261062762, 0.7760317562607026431, 0.8765941196519984047, 0.9999999999999887867 ) ) 
 REPRESENTATION_ITEM ( '' )  );
#39795=EDGE_CURVE ( 'NONE', #1251, #47122, #25663, .T. ) ;
#39797=B_SPLINE_CURVE_WITH_KNOTS ( 'NONE', 3,
 ( #12672, #42726, #1103, #24255, #16100, #38771, #39262, #31141, #42235, #8991 ),
 .UNSPECIFIED., .F., .F.,
 ( 4, 2, 2, 2, 4 ),
 ( 0.6272669072877719021, 0.7522669073072933976, 0.8772669073268148932, 1.002266907346336389, 1.127266907365857884 ),
 .UNSPECIFIED. ) ;
#39798=CARTESIAN_POINT ( 'NONE',  ( -10.27345454978659944, -12.71824136398891980, 64.45331520391344782 ) ) ;
#39799=CARTESIAN_POINT ( 'NONE',  ( -24.47371109942907808, -14.90716652360855576, 59.25772288469824645 ) ) ;
#39800=ADVANCED_FACE ( 'NONE', ( #44761 ), #35608, .T. ) ;
#39801=ORIENTED_EDGE ( 'NONE', *, *, #7016, .T. ) ;
#39803=EDGE_CURVE ( 'NONE', #22946, #15624, #28022, .T. ) ;
#39804=CARTESIAN_POINT ( 'NONE',  ( -24.47401588851211685, -14.84236380343934769, 59.24300237059242136 ) ) ;
#39805=PLANE ( 'NONE',  #26853 ) ;
#39806=VERTEX_POINT ( 'NONE', #38301 ) ;
#39808=ORIENTED_EDGE ( 'NONE', *, *, #33178, .T. ) ;
#39809=CYLINDRICAL_SURFACE ( 'NONE', #22651, 0.1500000000000063782 ) ;
#39813=CARTESIAN_POINT ( 'NONE',  ( -21.88020232903564732, -20.20778407762765738, 59.06442927265397458 ) ) ;
#39814=CARTESIAN_POINT ( 'NONE',  ( -13.38575581802539993, -9.030060914960570173, 60.72478133471773987 ) ) ;
#39816=VERTEX_POINT ( 'NONE', #12459 ) ;
#39817=CARTESIAN_POINT ( 'NONE',  ( -10.46640841813360900, -14.03671436131648242, 61.20204760743435202 ) ) ;
#39818=CARTESIAN_POINT ( 'NONE',  ( -14.82998572905333390, -8.253659511465704313, 60.32556042082950398 ) ) ;
#39819=CARTESIAN_POINT ( 'NONE',  ( -24.35389707626741185, -16.10709931453380861, 62.87856533165624029 ) ) ;
#39820=ADVANCED_FACE ( 'NONE', ( #27725 ), #8072, .F. ) ;
#39821=ORIENTED_EDGE ( 'NONE', *, *, #1565, .T. ) ;
#39823=EDGE_CURVE ( 'NONE', #3385, #38805, #38559, .T. ) ;
#39824=CARTESIAN_POINT ( 'NONE',  ( -19.57252240754909067, -21.52402959972952701, 65.47046003899923505 ) ) ;
#39826=EDGE_CURVE ( 'NONE', #17630, #12655, #29297, .T. ) ;
#39827=ORIENTED_EDGE ( 'NONE', *, *, #19200, .F. ) ;
#39829=CARTESIAN_POINT ( 'NONE',  ( -24.43827367352892210, -15.52193379869737200, 73.28831629023289906 ) ) ;
#39832=CARTESIAN_POINT ( 'NONE',  ( -10.12358845859998624, -13.32384912816304556, 74.72171712345732431 ) ) ;
#39833=CARTESIAN_POINT ( 'NONE',  ( -23.52949419687348964, -11.28347464189849703, 70.17738639980606763 ) ) ;
#39834=CARTESIAN_POINT ( 'NONE',  ( -23.08260857892799578, -18.93003297495478776, 62.35406880915004280 ) ) ;
#39835=CARTESIAN_POINT ( 'NONE',  ( -13.11718577119540718, -9.290850031293775402, 67.37942741453835538 ) ) ;
#39836=CARTESIAN_POINT ( 'NONE',  ( -13.90059129645203662, -21.37345143546091819, 72.10324577624415099 ) ) ;
#39839=ORIENTED_EDGE ( 'NONE', *, *, #21021, .F. ) ;
#39841=CARTESIAN_POINT ( 'NONE',  ( -10.44997270537017897, -15.86517854522099391, 61.24608883751315602 ) ) ;
#39842=CARTESIAN_POINT ( 'NONE',  ( -23.61204096558246235, -11.53669824655086451, 66.72214514747398084 ) ) ;
#39843=CARTESIAN_POINT ( 'NONE',  ( -15.96294676038700899, -7.962953527514619267, 67.15623976804144490 ) ) ;
#39844=CARTESIAN_POINT ( 'NONE',  ( -21.31115985637654120, -8.927249709250720144, 73.88656608925673197 ) ) ;
#39846=CARTESIAN_POINT ( 'NONE',  ( -17.92193097897700227, -21.84160713959417066, 62.17535923543130849 ) ) ;
#39848=ORIENTED_EDGE ( 'NONE', *, *, #36939, .F. ) ;
#39850=CARTESIAN_POINT ( 'NONE',  ( -10.66703313327717417, -12.79807994555918960, 64.56836111017611302 ) ) ;
#39852=DIRECTION ( 'NONE',  ( -0.4251432040024066272, -0.9051260995521939190, -1.185120001106687566E-09 ) ) ;
#39854=VERTEX_POINT ( 'NONE', #8297 ) ;
#39856=CARTESIAN_POINT ( 'NONE',  ( -10.56627859465609376, -16.21290490039525167, 71.44750383612122846 ) ) ;
#39857=CARTESIAN_POINT ( 'NONE',  ( -17.58536440216138885, -7.758048768718602162, 59.96572088198239214 ) ) ;
#39861=ORIENTED_EDGE ( 'NONE', *, *, #16565, .T. ) ;
#39862=FACE_OUTER_BOUND ( 'NONE', #27046, .T. ) ;
#39864=AXIS2_PLACEMENT_3D ( 'NONE', #24476, #46635, #39479 ) ;
#39867=CARTESIAN_POINT ( 'NONE',  ( -10.22954393756624114, -12.87502507475396918, 67.93843551393385383 ) ) ;
#39868=EDGE_LOOP ( 'NONE', ( #22724, #6370, #17414, #25247, #29919 ) ) ;
#39869=CARTESIAN_POINT ( 'NONE',  ( -13.72515530044423393, -21.27626469894021355, 68.59478590258110842 ) ) ;
#39870=FACE_OUTER_BOUND ( 'NONE', #23130, .T. ) ;
#39871=ORIENTED_EDGE ( 'NONE', *, *, #42471, .F. ) ;
#39872=CARTESIAN_POINT ( 'NONE',  ( -24.47217469005613211, -14.64471752244937441, 62.71296487297676947 ) ) ;
#39875=CARTESIAN_POINT ( 'NONE',  ( -14.71758685070772366, -21.32224385381664788, 62.05089037315948275 ) ) ;
#39876=ORIENTED_EDGE ( 'NONE', *, *, #5398, .T. ) ;
#39877=CARTESIAN_POINT ( 'NONE',  ( -18.68070144837527735, -7.415226739706411330, 53.49999999999994316 ) ) ;
#39878=EDGE_CURVE ( 'NONE', #37416, #31355, #8533, .T. ) ;
#39879=CARTESIAN_POINT ( 'NONE',  ( -10.96069643151774109, -18.51437482595545347, 57.92219192461608657 ) ) ;
#39882=EDGE_CURVE ( 'NONE', #27105, #36936, #5724, .T. ) ;
#39885=ORIENTED_EDGE ( 'NONE', *, *, #9691, .T. ) ;
#39886=B_SPLINE_CURVE_WITH_KNOTS ( 'NONE', 3,
 ( #40646, #26621, #26368, #11353, #18986, #763, #4950, #41383, #4447, #22944 ),
 .UNSPECIFIED., .F., .F.,
 ( 4, 2, 2, 2, 4 ),
 ( 0.1272669073658213301, 0.2522669073463013611, 0.3772669073267813644, 0.5022669073072614232, 0.6272669072877414820 ),
 .UNSPECIFIED. ) ;
#39887=FACE_OUTER_BOUND ( 'NONE', #9503, .T. ) ;
#39888=CARTESIAN_POINT ( 'NONE',  ( -24.31965416599553720, -16.01388414632039314, 62.70214577705259273 ) ) ;
#39889=ORIENTED_EDGE ( 'NONE', *, *, #44678, .F. ) ;
#39890=CARTESIAN_POINT ( 'NONE',  ( -20.76545062400256825, -8.150403215067090201, 63.48934267039048507 ) ) ;
#39893=CARTESIAN_POINT ( 'NONE',  ( -11.85162103594838001, -10.49015045520576983, 71.25420998615621215 ) ) ;
#39894=CARTESIAN_POINT ( 'NONE',  ( -20.57971641534515328, -8.060397143422079580, 66.90387173718066549 ) ) ;
#39897=ADVANCED_FACE ( 'NONE', ( #23808 ), #31420, .T. ) ;
#39898=CARTESIAN_POINT ( 'NONE',  ( -24.22092332596094977, -12.93687947476191269, 66.45246741375130739 ) ) ;
#39899=CARTESIAN_POINT ( 'NONE',  ( -20.70232273485035890, -8.624288160964143302, 60.14125250309182036 ) ) ;
#39900=CARTESIAN_POINT ( 'NONE',  ( -12.65882755920527458, -9.609488432089360543, 74.20434181795738482 ) ) ;
#39903=ORIENTED_EDGE ( 'NONE', *, *, #16268, .F. ) ;
#39904=VECTOR ( 'NONE', #455, 1000.000000000000114 ) ;
#39905=VERTEX_POINT ( 'NONE', #16865 ) ;
#39907=CARTESIAN_POINT ( 'NONE',  ( -24.87123163304818974, -14.59964195235338735, 62.89791815715346956 ) ) ;
#39908=CARTESIAN_POINT ( 'NONE',  ( -23.70135507383723805, -11.71146680393053607, 62.95218278684509983 ) ) ;
#39909=B_SPLINE_CURVE_WITH_KNOTS ( 'NONE', 3,
 ( #46387, #31845, #46634, #20761, #27419, #35761, #42452, #27905, #23749, #23983 ),
 .UNSPECIFIED., .F., .F.,
 ( 4, 2, 2, 2, 4 ),
 ( 0.6272669072878050978, 0.7522669073073239288, 0.8772669073268426487, 1.002266907346361480, 1.127266907365880311 ),
 .UNSPECIFIED. ) ;
#39910=CARTESIAN_POINT ( 'NONE',  ( -11.42962470904260464, -10.38539412368214521, 74.62380407152070916 ) ) ;
#39911=AXIS2_PLACEMENT_3D ( 'NONE', #30752, #1172, #38112 ) ;
#39912=ORIENTED_EDGE ( 'NONE', *, *, #40980, .T. ) ;
#39913=LINE ( 'NONE', #21685, #40774 ) ;
#39914=CARTESIAN_POINT ( 'NONE',  ( -12.97018521796328017, -9.340428432532196013, 74.73411830381819243 ) ) ;
#39916=CARTESIAN_POINT ( 'NONE',  ( -10.61357140615669792, -13.19155887971477448, 71.50828586566468914 ) ) ;
#39917=CARTESIAN_POINT ( 'NONE',  ( -12.93804115531433396, -9.435551541445537538, 70.86427763179355566 ) ) ;
#39918=( BOUNDED_CURVE ( )  B_SPLINE_CURVE ( 3, ( #41161, #38178, #11607, #15279 ),
 .UNSPECIFIED., .F., .F. ) 
 B_SPLINE_CURVE_WITH_KNOTS ( ( 4, 4 ),
 ( 0.9074455897393652881, 1.000000000000000000 ),
 .UNSPECIFIED. ) 
 CURVE ( )  GEOMETRIC_REPRESENTATION_ITEM ( )  RATIONAL_B_SPLINE_CURVE ( ( 0.6983129098261124934, 0.7760317562607149666, 0.8765941196520108392, 1.000000000000000000 ) ) 
 REPRESENTATION_ITEM ( '' )  );
#39919=CARTESIAN_POINT ( 'NONE',  ( -12.05806040642128707, -10.23620046216302448, 67.51368956197082127 ) ) ;
#39920=ORIENTED_EDGE ( 'NONE', *, *, #12145, .T. ) ;
#39921=LINE ( 'NONE', #45584, #8667 ) ;
#39922=VERTEX_POINT ( 'NONE', #13888 ) ;
#39923=CARTESIAN_POINT ( 'NONE',  ( -14.20982686782564386, -8.534409222511607496, 71.02397852537180256 ) ) ;
#39924=DIRECTION ( 'NONE',  ( -0.9466432954593471116, -0.3222832157619556770, -8.771047023603929338E-09 ) ) ;
#39925=CARTESIAN_POINT ( 'NONE',  ( -18.16442973052015830, -21.82037594034854422, 65.63972370452951566 ) ) ;
#39928=CARTESIAN_POINT ( 'NONE',  ( -20.17342227129689292, -21.73347691371985846, 72.52666002253516808 ) ) ;
#39929=FACE_OUTER_BOUND ( 'NONE', #46375, .T. ) ;
#39930=VECTOR ( 'NONE', #23775, 1000.000000000000114 ) ;
#39931=CARTESIAN_POINT ( 'NONE',  ( -13.62948724496060215, -8.926948417807865965, 57.26967755883410405 ) ) ;
#39932=CARTESIAN_POINT ( 'NONE',  ( -10.47299162366406478, -15.63514707757639854, 61.33789045486464886 ) ) ;
#39935=( BOUNDED_CURVE ( )  B_SPLINE_CURVE ( 3, ( #46945, #43270, #9288, #39799 ),
 .UNSPECIFIED., .F., .F. ) 
 B_SPLINE_CURVE_WITH_KNOTS ( ( 4, 4 ),
 ( 0.4074455897393629566, 0.5000000000000000000 ),
 .UNSPECIFIED. ) 
 CURVE ( )  GEOMETRIC_REPRESENTATION_ITEM ( )  RATIONAL_B_SPLINE_CURVE ( ( 0.6983129098260936196, 0.7760317562607117470, 0.8765941196520176115, 1.000000000000020650 ) ) 
 REPRESENTATION_ITEM ( '' )  );
#39937=AXIS2_PLACEMENT_3D ( 'NONE', #11293, #18412, #14693 ) ;
#39938=VECTOR ( 'NONE', #4099, 999.9999999999998863 ) ;
#39939=CARTESIAN_POINT ( 'NONE',  ( -17.00889379717436611, -21.85058792022787699, 68.90380497144548144 ) ) ;
#39942=CYLINDRICAL_SURFACE ( 'NONE', #17213, 0.1500000000000017708 ) ;
#39946=ORIENTED_EDGE ( 'NONE', *, *, #43703, .F. ) ;
#39947=DIRECTION ( 'NONE',  ( -0.9974380310868017352, -0.07153582418399355436, 3.008056591778321396E-08 ) ) ;
#39948=FACE_OUTER_BOUND ( 'NONE', #33777, .T. ) ;
#39949=VERTEX_POINT ( 'NONE', #13651 ) ;
#39951=CARTESIAN_POINT ( 'NONE',  ( -10.45004451964941872, -15.89438299218807771, 71.59183561948579211 ) ) ;
#39953=CARTESIAN_POINT ( 'NONE',  ( -11.61616642816477807, -18.80577669094758164, 68.22249455738848667 ) ) ;
#39955=CARTESIAN_POINT ( 'NONE',  ( -16.24320552860936928, -21.75975297682954945, 58.58025747933638172 ) ) ;
#39956=VERTEX_POINT ( 'NONE', #31907 ) ;
#39957=FACE_BOUND ( 'NONE', #16345, .T. ) ;
#39958=AXIS2_PLACEMENT_3D ( 'NONE', #19537, #27656, #831 ) ;
#39960=CYLINDRICAL_SURFACE ( 'NONE', #9994, 0.1500000000000019651 ) ;
#39961=EDGE_CURVE ( 'NONE', #29649, #43613, #46924, .T. ) ;
#39962=EDGE_CURVE ( 'NONE', #39384, #21434, #7988, .T. ) ;
#39963=CARTESIAN_POINT ( 'NONE',  ( -20.69509252757554307, -8.115601716887088202, 63.49616818922779515 ) ) ;
#39965=CARTESIAN_POINT ( 'NONE',  ( -11.64902330566212463, -10.02396254413167576, 53.49999999999994316 ) ) ;
#39966=( NAMED_UNIT ( * ) SI_UNIT ( $, .STERADIAN. ) SOLID_ANGLE_UNIT ( ) );
#39968=EDGE_CURVE ( 'NONE', #7647, #12505, #20871, .T. ) ;
#39969=CARTESIAN_POINT ( 'NONE',  ( -13.25446207031254886, -8.635133168339066856, 60.57916952436288227 ) ) ;
#39970=CARTESIAN_POINT ( 'NONE',  ( -13.73970969606274473, -20.76112332560825990, 65.28628881671112083 ) ) ;
#39971=CARTESIAN_POINT ( 'NONE',  ( -11.52367759983210149, -11.04269222737732470, 57.50903262756441592 ) ) ;
#39972=ORIENTED_EDGE ( 'NONE', *, *, #18486, .T. ) ;
#39973=VERTEX_POINT ( 'NONE', #36537 ) ;
#39975=EDGE_CURVE ( 'NONE', #46413, #28927, #31668, .T. ) ;
#39976=CARTESIAN_POINT ( 'NONE',  ( -10.85841931818429629, -17.37798394237198707, 64.91267318220633342 ) ) ;
#39978=CYLINDRICAL_SURFACE ( 'NONE', #23730, 0.1500000000000006051 ) ;
#39981=AXIS2_PLACEMENT_3D ( 'NONE', #3594, #26749, #11239 ) ;
#39982=CARTESIAN_POINT ( 'NONE',  ( -15.43264099835366565, -7.630132484668774140, 74.24132189675523819 ) ) ;
#39984=CARTESIAN_POINT ( 'NONE',  ( -10.98866448286933029, -11.05551018869101298, 60.81739231005553847 ) ) ;
#39985=VECTOR ( 'NONE', #47395, 1000.000000000000227 ) ;
#39986=CARTESIAN_POINT ( 'NONE',  ( -22.05805477923917124, -20.12249178580863784, 62.23998944766726282 ) ) ;
#39987=ORIENTED_EDGE ( 'NONE', *, *, #45361, .F. ) ;
#39989=B_SPLINE_CURVE_WITH_KNOTS ( 'NONE', 3,
 ( #32311, #47335, #13565, #28611, #39928, #6201, #7672, #7423, #26364, #22677 ),
 .UNSPECIFIED., .F., .F.,
 ( 4, 2, 2, 2, 4 ),
 ( 0.6272669072974624838, 0.7522669073145729079, 0.8772669073316834432, 1.002266907348793978, 1.127266907365904292 ),
 .UNSPECIFIED. ) ;
#39990=CARTESIAN_POINT ( 'NONE',  ( -14.69606858684902306, -21.31402952851196986, 61.93600410282152779 ) ) ;
#39993=CARTESIAN_POINT ( 'NONE',  ( -18.54257441268414297, -21.71939603377284911, 72.58510895925300588 ) ) ;
#39995=CARTESIAN_POINT ( 'NONE',  ( -17.93190708896392493, -21.84390349538901077, 58.29064763788917958 ) ) ;
#39996=CARTESIAN_POINT ( 'NONE',  ( -23.40706900507760224, -18.44293855997280929, 73.06368236814604700 ) ) ;
#39997=EDGE_CURVE ( 'NONE', #47492, #24829, #10321, .T. ) ;
#39998=CARTESIAN_POINT ( 'NONE',  ( -15.27707121964805381, -8.090297697211889627, 74.28805465071215508 ) ) ;
#39999=CARTESIAN_POINT ( 'NONE',  ( -22.48114071483173149, -19.64927648862363796, 72.94400547034429394 ) ) ;
#40000=ORIENTED_EDGE ( 'NONE', *, *, #45972, .T. ) ;
#40001=CARTESIAN_POINT ( 'NONE',  ( -10.38243336603528277, -15.21964919048783393, 57.65972899058709800 ) ) ;
#40002=CARTESIAN_POINT ( 'NONE',  ( -24.14679772577363437, -12.68507108172156883, 70.05770892828130059 ) ) ;
#40005=CARTESIAN_POINT ( 'NONE',  ( -20.06975372951847447, -8.274133229585533655, 73.73568642813194174 ) ) ;
#40007=ADVANCED_FACE ( 'NONE', ( #5814 ), #2104, .T. ) ;
#40010=DIRECTION ( 'NONE',  ( -3.892913453477729145E-06, -4.639959647628106577E-06, -0.9999999999816580054 ) ) ;
#40011=ORIENTED_EDGE ( 'NONE', *, *, #14859, .T. ) ;
#40012=CARTESIAN_POINT ( 'NONE',  ( -10.69339011031838105, -12.88606202777132914, 64.55370748154987837 ) ) ;
#40014=CARTESIAN_POINT ( 'NONE',  ( -14.28136839270488423, -8.054466369743188636, 67.45313376895239799 ) ) ;
#40015=CARTESIAN_POINT ( 'NONE',  ( -10.00048885941320087, -15.43727575513289629, 57.69075912652810700 ) ) ;
#40016=ORIENTED_EDGE ( 'NONE', *, *, #20237, .F. ) ;
#40018=VECTOR ( 'NONE', #32779, 1000.000000000000000 ) ;
#40020=B_SPLINE_CURVE_WITH_KNOTS ( 'NONE', 3,
 ( #2648, #21130, #10761, #6828, #10530, #17886, #44510, #13476, #29479, #6102 ),
 .UNSPECIFIED., .F., .F.,
 ( 4, 2, 2, 2, 4 ),
 ( 0.000000000000000000, 0.2500000000000000000, 0.5000000000000000000, 0.7500000000000000000, 1.000000000000000000 ),
 .UNSPECIFIED. ) ;
#40022=ORIENTED_EDGE ( 'NONE', *, *, #7906, .T. ) ;
#40025=CARTESIAN_POINT ( 'NONE',  ( -15.62222905942471840, -7.993050613273783966, 70.89517703929612935 ) ) ;
#40027=EDGE_CURVE ( 'NONE', #8571, #25, #13602, .T. ) ;
#40028=CARTESIAN_POINT ( 'NONE',  ( -12.90958250904497362, -8.882692446305687994, 67.50225915842231927 ) ) ;
#40029=CARTESIAN_POINT ( 'NONE',  ( -22.79734351242366941, -10.24514170768878962, 66.69182257473532616 ) ) ;
#40030=CARTESIAN_POINT ( 'NONE',  ( -13.12535629923256941, -9.217633289312832545, 71.26414145609075490 ) ) ;
#40031=ORIENTED_EDGE ( 'NONE', *, *, #38220, .T. ) ;
#40039=ORIENTED_EDGE ( 'NONE', *, *, #21275, .F. ) ;
#40042=CARTESIAN_POINT ( 'NONE',  ( -24.78816760170556677, -15.94238017617776215, 69.71962869939886787 ) ) ;
#40044=CARTESIAN_POINT ( 'NONE',  ( -11.28069604468732479, -11.45046212628238358, 67.80791698215925578 ) ) ;
#40045=ORIENTED_EDGE ( 'NONE', *, *, #43989, .F. ) ;
#40048=CARTESIAN_POINT ( 'NONE',  ( -14.42215129996211154, -7.990733167546266280, 63.89640551974409988 ) ) ;
#40049=ORIENTED_EDGE ( 'NONE', *, *, #14465, .T. ) ;
#40050=VECTOR ( 'NONE', #23973, 1000.000000000000000 ) ;
#40051=CARTESIAN_POINT ( 'NONE',  ( -19.51114651407244338, -7.656733154341000436, 60.14748342315007790 ) ) ;
#40052=EDGE_CURVE ( 'NONE', #748, #21369, #12065, .T. ) ;
#40053=CARTESIAN_POINT ( 'NONE',  ( -11.29134393598116937, -11.33126488396075260, 64.16354160640879911 ) ) ;
#40054=CARTESIAN_POINT ( 'NONE',  ( -18.07488717577700754, -21.77899923650016589, 65.64532180046710153 ) ) ;
#40055=ORIENTED_EDGE ( 'NONE', *, *, #30786, .F. ) ;
#40056=CARTESIAN_POINT ( 'NONE',  ( -20.77611426707521858, -20.95444529357722629, 58.75361203847226932 ) ) ;
#40059=CARTESIAN_POINT ( 'NONE',  ( -14.60479643987598841, -7.913168514039711887, 60.50491717424539218 ) ) ;
#40062=CARTESIAN_POINT ( 'NONE',  ( -11.02242957576233451, -11.85532881267382166, 74.57312195644870201 ) ) ;
#40063=CARTESIAN_POINT ( 'NONE',  ( -22.71059208588729561, -10.14448404190931186, 70.02650598627910483 ) ) ;
#40064=LINE ( 'NONE', #43284, #35304 ) ;
#40065=ORIENTED_EDGE ( 'NONE', *, *, #10169, .T. ) ;
#40067=UNCERTAINTY_MEASURE_WITH_UNIT (LENGTH_MEASURE( 1.000000000000000082E-05 ), #47112, 'distance_accuracy_value', 'NONE');
#40068=( BOUNDED_CURVE ( )  B_SPLINE_CURVE ( 3, ( #27902, #4775, #20032, #34802 ),
 .UNSPECIFIED., .F., .F. ) 
 B_SPLINE_CURVE_WITH_KNOTS ( ( 4, 4 ),
 ( 0.000000000000000000, 0.4074455897393594039 ),
 .UNSPECIFIED. ) 
 CURVE ( )  GEOMETRIC_REPRESENTATION_ITEM ( )  RATIONAL_B_SPLINE_CURVE ( ( 1.000000000000000000, 0.4567392136813357428, 0.3561768502900316546, 0.6983129098260878465 ) ) 
 REPRESENTATION_ITEM ( '' )  );
#40069=CARTESIAN_POINT ( 'NONE',  ( -16.65185932245351452, -21.81708442718849383, 65.51092266128213737 ) ) ;
#40070=CARTESIAN_POINT ( 'NONE',  ( -16.52316554273587101, -21.80170452179945073, 65.24036514508233608 ) ) ;
#40073=CARTESIAN_POINT ( 'NONE',  ( -24.77957839681537777, -15.99319750247286542, 66.20178371291459030 ) ) ;
#40076=CARTESIAN_POINT ( 'NONE',  ( -24.06787342886325121, -18.28917680027896608, 54.27966884056654351 ) ) ;
#40078=AXIS2_PLACEMENT_3D ( 'NONE', #25215, #40237, #40953 ) ;
#40079=CARTESIAN_POINT ( 'NONE',  ( -11.42587710518540334, -11.10406226247761019, 57.49431069621225276 ) ) ;
#40080=CARTESIAN_POINT ( 'NONE',  ( -21.89269609535176997, -8.848005330197558749, 66.78337213843711595 ) ) ;
#40081=DIRECTION ( 'NONE',  ( -0.3478314405900341799, -0.9375570856950852239, 0.000000000000000000 ) ) ;
#40082=( BOUNDED_CURVE ( )  B_SPLINE_CURVE ( 3, ( #44844, #3707, #18971, #33468 ),
 .UNSPECIFIED., .F., .F. ) 
 B_SPLINE_CURVE_WITH_KNOTS ( ( 4, 4 ),
 ( 0.9074455897393706172, 1.000000000000000000 ),
 .UNSPECIFIED. ) 
 CURVE ( )  GEOMETRIC_REPRESENTATION_ITEM ( )  RATIONAL_B_SPLINE_CURVE ( ( 0.6983129098261035006, 0.7760317562607071951, 0.8765941196520060652, 1.000000000000000000 ) ) 
 REPRESENTATION_ITEM ( '' )  );
#40084=CARTESIAN_POINT ( 'NONE',  ( -11.22844613476422282, -11.44458948612160221, 64.43409918096024569 ) ) ;
#40085=( BOUNDED_CURVE ( )  B_SPLINE_CURVE ( 3, ( #39976, #13120, #47376, #47611 ),
 .UNSPECIFIED., .F., .F. ) 
 B_SPLINE_CURVE_WITH_KNOTS ( ( 4, 4 ),
 ( 0.000000000000000000, 0.4074455897393624570 ),
 .UNSPECIFIED. ) 
 CURVE ( )  GEOMETRIC_REPRESENTATION_ITEM ( )  RATIONAL_B_SPLINE_CURVE ( ( 1.000000000000000000, 0.4567392136813325787, 0.3561768502900305444, 0.6983129098260937306 ) ) 
 REPRESENTATION_ITEM ( '' )  );
#40086=CARTESIAN_POINT ( 'NONE',  ( -20.50928888383101167, -8.027964920953767347, 66.82458168832727097 ) ) ;
#40088=ORIENTED_EDGE ( 'NONE', *, *, #17901, .T. ) ;
#40089=ORIENTED_EDGE ( 'NONE', *, *, #30963, .F. ) ;
#40090=B_SPLINE_CURVE_WITH_KNOTS ( 'NONE', 3,
 ( #34519, #22735, #7476, #12123, #33784, #7714, #16039, #15548, #41424, #30124 ),
 .UNSPECIFIED., .F., .F.,
 ( 4, 2, 2, 2, 4 ),
 ( 0.000000000000000000, 0.2500000000000000000, 0.5000000000000000000, 0.7500000000000000000, 1.000000000000000000 ),
 .UNSPECIFIED. ) ;
#40091=EDGE_CURVE ( 'NONE', #34163, #48033, #2635, .T. ) ;
#40092=CARTESIAN_POINT ( 'NONE',  ( -22.88264614489240856, -10.34704276773305764, 63.35713876973677827 ) ) ;
#40093=CARTESIAN_POINT ( 'NONE',  ( -19.99112977906324318, -8.296885409642934306, 74.02096600045412345 ) ) ;
#40094=CARTESIAN_POINT ( 'NONE',  ( -14.92764478915313653, -21.34891159457319532, 61.63600440564275829 ) ) ;
#40095=CIRCLE ( 'NONE', #799, 0.4000000000000006883 ) ;
#40096=CARTESIAN_POINT ( 'NONE',  ( -11.01524394860871858, -17.62490983191025862, 71.86718188073483304 ) ) ;
#40097=ADVANCED_FACE ( 'NONE', ( #21783 ), #18636, .T. ) ;
#40098=CARTESIAN_POINT ( 'NONE',  ( -14.07063681424402724, -8.156626161945256470, 70.87957628055752934 ) ) ;
#40100=( BOUNDED_CURVE ( )  B_SPLINE_CURVE ( 3, ( #44859, #25403, #21946, #21703 ),
 .UNSPECIFIED., .F., .F. ) 
 B_SPLINE_CURVE_WITH_KNOTS ( ( 4, 4 ),
 ( 0.5000000000000000000, 0.9074455897393651771 ),
 .UNSPECIFIED. ) 
 CURVE ( )  GEOMETRIC_REPRESENTATION_ITEM ( )  RATIONAL_B_SPLINE_CURVE ( ( 1.000000000000009548, 0.4567392136813376302, 0.3561768502900256594, 0.6983129098260838497 ) ) 
 REPRESENTATION_ITEM ( '' )  );
#40102=CARTESIAN_POINT ( 'NONE',  ( -21.94683289283972982, -20.15404817794292214, 62.34512228983284388 ) ) ;
#40103=CARTESIAN_POINT ( 'NONE',  ( -13.12613380977788147, -20.89454282643029259, 58.16154686733092660 ) ) ;
#40106=EDGE_CURVE ( 'NONE', #34964, #16737, #3556, .T. ) ;
#40107=ORIENTED_EDGE ( 'NONE', *, *, #35239, .T. ) ;
#40108=EDGE_CURVE ( 'NONE', #43339, #17712, #47904, .T. ) ;
#40109=CARTESIAN_POINT ( 'NONE',  ( -13.88833677318074500, -20.91193151007171736, 64.87139997340349851 ) ) ;
#40110=EDGE_CURVE ( 'NONE', #42299, #6219, #25973, .T. ) ;
#40113=PLANE ( 'NONE',  #5330 ) ;
#40115=CARTESIAN_POINT ( 'NONE',  ( -10.88286923018596575, -17.43962093083235843, 68.11193994895104709 ) ) ;
#40116=ORIENTED_EDGE ( 'NONE', *, *, #42284, .T. ) ;
#40117=FACE_OUTER_BOUND ( 'NONE', #25025, .T. ) ;
#40119=EDGE_LOOP ( 'NONE', ( #15034, #48221 ) ) ;
#40121=CARTESIAN_POINT ( 'NONE',  ( -19.21722672681719146, -7.578212081832392144, 63.63100440621975906 ) ) ;
#40122=ORIENTED_EDGE ( 'NONE', *, *, #21678, .T. ) ;
#40125=VERTEX_POINT ( 'NONE', #18562 ) ;
#40126=DIRECTION ( 'NONE',  ( 1.078708504465006897E-05, 7.367657514171588156E-06, 0.9999999999146782503 ) ) ;
#40127=AXIS2_PLACEMENT_3D ( 'NONE', #6243, #36261, #36975 ) ;
#40129=CARTESIAN_POINT ( 'NONE',  ( -23.92719381113450083, -11.17417296164256157, 70.00715453762190066 ) ) ;
#40130=ORIENTED_EDGE ( 'NONE', *, *, #32043, .F. ) ;
#40131=LINE ( 'NONE', #6393, #21573 ) ;
#40132=CARTESIAN_POINT ( 'NONE',  ( -16.86460949297358525, -7.773444642497263857, 70.64603134899243742 ) ) ;
#40133=CARTESIAN_POINT ( 'NONE',  ( -24.09973193186370111, -12.53120327594186634, 69.98062835556456207 ) ) ;
#40134=CARTESIAN_POINT ( 'NONE',  ( -23.16791676868475491, -10.71612278230448823, 60.01692287334890352 ) ) ;
#40136=ORIENTED_EDGE ( 'NONE', *, *, #33890, .T. ) ;
#40137=VERTEX_POINT ( 'NONE', #14852 ) ;
#40139=CARTESIAN_POINT ( 'NONE',  ( -21.42336286209559759, -21.09487474236010485, 69.23945462178221533 ) ) ;
#40140=EDGE_LOOP ( 'NONE', ( #42775, #32203, #43745, #1087, #47609 ) ) ;
#40141=CARTESIAN_POINT ( 'NONE',  ( -10.43972881942000086, -15.77115500203794873, 64.52243715390834211 ) ) ;
#40143=CARTESIAN_POINT ( 'NONE',  ( -11.07857809310684338, -11.73724795245126273, 71.38860870961248395 ) ) ;
#40144=CARTESIAN_POINT ( 'NONE',  ( -16.93852767260800007, -21.79234520888179460, 68.88663808031736835 ) ) ;
#40145=CARTESIAN_POINT ( 'NONE',  ( -12.31380134045779506, -10.02538898168817916, 60.55918086676557976 ) ) ;
#40146=EDGE_LOOP ( 'NONE', ( #38469, #17259, #18566, #39298, #28609 ) ) ;
#40147=EDGE_CURVE ( 'NONE', #12505, #7647, #17371, .T. ) ;
#40148=CARTESIAN_POINT ( 'NONE',  ( -10.55579457777002439, -13.45742151464481751, 74.96352273250263920 ) ) ;
#40149=CARTESIAN_POINT ( 'NONE',  ( -14.55015457993596328, -8.362855509585410019, 70.87390454733632339 ) ) ;
#40151=CARTESIAN_POINT ( 'NONE',  ( -19.70639647806698136, -21.90109437720271757, 65.57990800639531415 ) ) ;
#40154=ORIENTED_EDGE ( 'NONE', *, *, #2796, .T. ) ;
#40156=CARTESIAN_POINT ( 'NONE',  ( -24.87126894608573124, -14.60124070896847392, 62.75650584303257062 ) ) ;
#40157=CARTESIAN_POINT ( 'NONE',  ( -23.34288396506439867, -19.33377296368179543, 59.06906041190286771 ) ) ;
#40158=VECTOR ( 'NONE', #17548, 1000.000000000000000 ) ;
#40161=CARTESIAN_POINT ( 'NONE',  ( -24.47010849973345614, -14.47977947063238879, 69.95275342396321605 ) ) ;
#40163=EDGE_CURVE ( 'NONE', #20660, #9213, #4785, .T. ) ;
#40168=CARTESIAN_POINT ( 'NONE',  ( -10.61465111059293598, -17.83148713366484017, 71.66743938577346285 ) ) ;
#40170=CARTESIAN_POINT ( 'NONE',  ( -24.47066272824306665, -14.57993217219608795, 62.99824437345093031 ) ) ;
#40171=CARTESIAN_POINT ( 'NONE',  ( -23.33631914962121456, -10.27599873017480903, 59.77920290994538988 ) ) ;
#40172=ORIENTED_EDGE ( 'NONE', *, *, #25442, .F. ) ;
#40174=CARTESIAN_POINT ( 'NONE',  ( -10.11824970337647223, -16.26811690260224452, 71.56254994910038647 ) ) ;
#40176=LINE ( 'NONE', #25394, #11635 ) ;
#40178=CARTESIAN_POINT ( 'NONE',  ( -21.42981983006149349, -21.09080987443381261, 69.23167044377096602 ) ) ;
#40179=DIRECTION ( 'NONE',  ( -0.5263399769092093061, 0.8502742079512979334, 7.678741024442198749E-08 ) ) ;
#40183=CARTESIAN_POINT ( 'NONE',  ( -16.65185932245351452, -21.81708442718849383, 65.51092266128213737 ) ) ;
#40184=EDGE_LOOP ( 'NONE', ( #14453, #7098, #2856, #22566, #46379 ) ) ;
#40185=CARTESIAN_POINT ( 'NONE',  ( -11.95967870817407430, -14.07562448187690940, 53.88362224778186516 ) ) ;
#40186=CARTESIAN_POINT ( 'NONE',  ( -11.82257370584654943, -19.00738327630861946, 71.68685835237670290 ) ) ;
#40187=CARTESIAN_POINT ( 'NONE',  ( -22.94659349086428435, -9.808683002949324603, 70.11840218492315557 ) ) ;
#40189=CARTESIAN_POINT ( 'NONE',  ( -16.09337608010665477, -22.13948405174236811, 58.40090292489767876 ) ) ;
#40190=CARTESIAN_POINT ( 'NONE',  ( -11.86342561440307186, -10.47520584478210814, 71.26333307341455736 ) ) ;
#40192=ORIENTED_EDGE ( 'NONE', *, *, #44259, .F. ) ;
#40193=EDGE_LOOP ( 'NONE', ( #30543, #32870 ) ) ;
#40194=DIRECTION ( 'NONE',  ( 3.549360974554993999E-17, -6.371834667797928663E-18, -1.000000000000000000 ) ) ;
#40196=CARTESIAN_POINT ( 'NONE',  ( -23.46260529264823447, -11.17067950781535579, 73.36193301757424479 ) ) ;
#40200=DIRECTION ( 'NONE',  ( -0.3478314405900341799, -0.9375570856950852239, 0.000000000000000000 ) ) ;
#40201=CARTESIAN_POINT ( 'NONE',  ( -19.24025795797341942, -7.996846695050864540, 60.24620885950562865 ) ) ;
#40203=B_SPLINE_CURVE_WITH_KNOTS ( 'NONE', 1,
 ( #4819, #19842 ),
 .UNSPECIFIED., .F., .F.,
 ( 2, 2 ),
 ( 0.000000000000000000, 1.000000000000000000 ),
 .UNSPECIFIED. ) ;
#40205=CARTESIAN_POINT ( 'NONE',  ( -24.72694788909437236, -16.28301151488813403, 62.70833397083087846 ) ) ;
#40207=FACE_OUTER_BOUND ( 'NONE', #3795, .T. ) ;
#40208=CARTESIAN_POINT ( 'NONE',  ( -20.60788153932096023, -8.518722016582884748, 63.32593600985608617 ) ) ;
#40209=ADVANCED_FACE ( 'NONE', ( #20041 ), #47846, .T. ) ;
#40210=ORIENTED_EDGE ( 'NONE', *, *, #47895, .T. ) ;
#40215=DIRECTION ( 'NONE',  ( 0.07061531369766044230, 0.9975036227860933913, 1.268851335910971019E-08 ) ) ;
#40216=FACE_OUTER_BOUND ( 'NONE', #38873, .T. ) ;
#40217=CARTESIAN_POINT ( 'NONE',  ( -10.67250920137991521, -11.65805311173287961, 71.20205571017048385 ) ) ;
#40220=ORIENTED_EDGE ( 'NONE', *, *, #9086, .F. ) ;
#40224=CARTESIAN_POINT ( 'NONE',  ( -12.23165125622869631, -10.02867215863997608, 67.64329750964374455 ) ) ;
#40225=( BOUNDED_CURVE ( )  B_SPLINE_CURVE ( 3, ( #8734, #35294, #47118, #35542 ),
 .UNSPECIFIED., .F., .F. ) 
 B_SPLINE_CURVE_WITH_KNOTS ( ( 4, 4 ),
 ( 0.4074455897393624015, 0.5000000000000000000 ),
 .UNSPECIFIED. ) 
 CURVE ( )  GEOMETRIC_REPRESENTATION_ITEM ( )  RATIONAL_B_SPLINE_CURVE ( ( 0.6983129098260898449, 0.7760317562606841024, 0.8765941196519841938, 0.9999999999999820144 ) ) 
 REPRESENTATION_ITEM ( '' )  );
#40229=CARTESIAN_POINT ( 'NONE',  ( -10.45256735519816615, -15.43993469624229853, 57.56792809193251514 ) ) ;
#40230=ORIENTED_EDGE ( 'NONE', *, *, #28705, .F. ) ;
#40231=CARTESIAN_POINT ( 'NONE',  ( -10.39215594834096024, -14.30487625923878880, 64.53803863383089379 ) ) ;
#40233=CARTESIAN_POINT ( 'NONE',  ( -20.54786284059405688, -21.13826946137156781, 62.25904375309657723 ) ) ;
#40234=VERTEX_POINT ( 'NONE', #45677 ) ;
#40236=( BOUNDED_CURVE ( )  B_SPLINE_CURVE ( 3, ( #43743, #28947, #32413, #1642 ),
 .UNSPECIFIED., .F., .F. ) 
 B_SPLINE_CURVE_WITH_KNOTS ( ( 4, 4 ),
 ( 0.5000000000000000000, 0.9074455897393596260 ),
 .UNSPECIFIED. ) 
 CURVE ( )  GEOMETRIC_REPRESENTATION_ITEM ( )  RATIONAL_B_SPLINE_CURVE ( ( 1.000000000000023981, 0.4567392136813375192, 0.3561768502900155564, 0.6983129098260840717 ) ) 
 REPRESENTATION_ITEM ( '' )  );
#40237=DIRECTION ( 'NONE',  ( -0.2771212459065067191, 0.9608349572466770017, 4.100231986695772107E-08 ) ) ;
#40238=EDGE_LOOP ( 'NONE', ( #33330, #17585 ) ) ;
#40241=CARTESIAN_POINT ( 'NONE',  ( -17.78451647839747807, -7.367880489560593382, 60.18722466726725884 ) ) ;
#40243=CARTESIAN_POINT ( 'NONE',  ( -9.980621257831284510, -14.49716697860085546, 67.95776503052229600 ) ) ;
#40244=ORIENTED_EDGE ( 'NONE', *, *, #35920, .F. ) ;
#40245=CARTESIAN_POINT ( 'NONE',  ( -11.92829163603010301, -19.83900259450906489, 58.02708122498009402 ) ) ;
#40247=EDGE_CURVE ( 'NONE', #14322, #31196, #29675, .T. ) ;
#40249=CARTESIAN_POINT ( 'NONE',  ( -16.72801347667246574, -21.77457299860571283, 65.45237662829435976 ) ) ;
#40250=CARTESIAN_POINT ( 'NONE',  ( -17.19811928533322387, -9.313850733363548073, 54.07175714974879099 ) ) ;
#40251=EDGE_LOOP ( 'NONE', ( #17117, #33013, #38230, #24384, #9518 ) ) ;
#40252=CARTESIAN_POINT ( 'NONE',  ( -15.40811923343077083, -21.56513327689926030, 72.06047564147742435 ) ) ;
#40253=CARTESIAN_POINT ( 'NONE',  ( -10.76011810543446323, -12.66604461453143493, 60.79853557587211554 ) ) ;
#40254=CARTESIAN_POINT ( 'NONE',  ( -24.92071865458970947, -14.23843710221147774, 54.02312124697527906 ) ) ;
#40256=CARTESIAN_POINT ( 'NONE',  ( -11.57126885336172073, -10.86466612894600381, 74.59451641100736197 ) ) ;
#40257=EDGE_CURVE ( 'NONE', #45412, #8644, #11444, .T. ) ;
#40258=CARTESIAN_POINT ( 'NONE',  ( -16.78181722113097152, -22.23154757984593388, 68.73914717078854153 ) ) ;
#40259=PLANE ( 'NONE',  #22990 ) ;
#40260=ORIENTED_EDGE ( 'NONE', *, *, #33405, .F. ) ;
#40261=CARTESIAN_POINT ( 'NONE',  ( -18.52416312356643147, -7.896186446804856374, 73.84064402154488960 ) ) ;
#40262=CARTESIAN_POINT ( 'NONE',  ( -21.52725980274252393, -9.076272844571150245, 70.43132538913752683 ) ) ;
#40263=CARTESIAN_POINT ( 'NONE',  ( -18.55957040452605611, -7.446158924837727788, 74.02559677774105751 ) ) ;
#40264=ORIENTED_EDGE ( 'NONE', *, *, #47916, .T. ) ;
#40266=ORIENTED_EDGE ( 'NONE', *, *, #30081, .T. ) ;
#40268=ORIENTED_EDGE ( 'NONE', *, *, #4498, .T. ) ;
#40270=CARTESIAN_POINT ( 'NONE',  ( -12.84690951644825851, -8.931012861620404308, 67.56438176077992352 ) ) ;
#40271=CYLINDRICAL_SURFACE ( 'NONE', #25188, 0.1499999999999991063 ) ;
#40273=ORIENTED_EDGE ( 'NONE', *, *, #39573, .F. ) ;
#40274=ORIENTED_EDGE ( 'NONE', *, *, #4581, .T. ) ;
#40277=CARTESIAN_POINT ( 'NONE',  ( -10.82849021881276386, -17.15435654512475594, 61.15743105340639119 ) ) ;
#40278=EDGE_CURVE ( 'NONE', #43505, #10981, #35771, .T. ) ;
#40281=EDGE_CURVE ( 'NONE', #33252, #20890, #5008, .T. ) ;
#40282=CARTESIAN_POINT ( 'NONE',  ( -15.32518410995109193, -21.95751795911967008, 72.16080160551160816 ) ) ;
#40283=CARTESIAN_POINT ( 'NONE',  ( -20.00946539473887142, -8.250368680643830999, 73.87096600125035195 ) ) ;
#40284=ORIENTED_EDGE ( 'NONE', *, *, #15183, .F. ) ;
#40285=LINE ( 'NONE', #24790, #28062 ) ;
#40289=CARTESIAN_POINT ( 'NONE',  ( -16.34036753895378524, -21.72486956401631630, 58.51258804093296106 ) ) ;
#40290=CARTESIAN_POINT ( 'NONE',  ( -11.35825037048775066, -11.21643016533577075, 60.67885780704620657 ) ) ;
#40291=EDGE_CURVE ( 'NONE', #35967, #11672, #14998, .T. ) ;
#40292=ORIENTED_EDGE ( 'NONE', *, *, #32943, .T. ) ;
#40293=CARTESIAN_POINT ( 'NONE',  ( -19.50103315386265024, -8.068942516160735323, 60.37581784757137626 ) ) ;
#40294=EDGE_CURVE ( 'NONE', #700, #44129, #43815, .T. ) ;
#40295=CARTESIAN_POINT ( 'NONE',  ( -22.83929682888979329, -10.29453308790038157, 66.55654356380499337 ) ) ;
#40296=CARTESIAN_POINT ( 'NONE',  ( -21.68499490698325971, -9.192515188766618550, 66.81149992326716358 ) ) ;
#40297=VERTEX_POINT ( 'NONE', #35290 ) ;
#40298=CARTESIAN_POINT ( 'NONE',  ( -10.42302287260171312, -13.97751933429587012, 57.73352905910142852 ) ) ;
#40299=CARTESIAN_POINT ( 'NONE',  ( -10.42431094601142050, -14.74024948089186537, 71.32782695460157640 ) ) ;
#40300=DIRECTION ( 'NONE',  ( -0.3478314405900309603, -0.9375570856950864451, 0.000000000000000000 ) ) ;
#40303=ORIENTED_EDGE ( 'NONE', *, *, #31433, .T. ) ;
#40304=FACE_OUTER_BOUND ( 'NONE', #28093, .T. ) ;
#40305=CARTESIAN_POINT ( 'NONE',  ( -13.70502021987594077, -20.80197949353049580, 68.87113990053892110 ) ) ;
#40306=CARTESIAN_POINT ( 'NONE',  ( -11.36794959886231915, -18.31963617796164812, 57.80714594517343841 ) ) ;
#40308=ORIENTED_EDGE ( 'NONE', *, *, #22655, .T. ) ;
#40309=CYLINDRICAL_SURFACE ( 'NONE', #6366, 0.1500000000000080158 ) ;
#40310=EDGE_CURVE ( 'NONE', #14550, #1220, #45987, .T. ) ;
#40311=CARTESIAN_POINT ( 'NONE',  ( -19.04787736696107103, -7.538188104413229063, 67.02354920417977269 ) ) ;
#40312=CARTESIAN_POINT ( 'NONE',  ( -15.69205246790211561, -7.972184624072811587, 74.49474465824219749 ) ) ;
#40313=ORIENTED_EDGE ( 'NONE', *, *, #46255, .T. ) ;
#40314=CARTESIAN_POINT ( 'NONE',  ( -11.22166882806820176, -18.93646342201198607, 64.86894282563231684 ) ) ;
#40315=CARTESIAN_POINT ( 'NONE',  ( -24.28579947082789303, -13.18942387424446494, 62.84736316175410309 ) ) ;
#40316=ORIENTED_EDGE ( 'NONE', *, *, #12933, .F. ) ;
#40317=EDGE_LOOP ( 'NONE', ( #35140, #47245, #32923, #40511, #6815 ) ) ;
#40321=CARTESIAN_POINT ( 'NONE',  ( -23.39635208968330105, -11.04794396834914494, 70.04777744521437910 ) ) ;
#40322=CARTESIAN_POINT ( 'NONE',  ( -14.87886258693389507, -8.287862487286286495, 60.33612870302592057 ) ) ;
#40323=CARTESIAN_POINT ( 'NONE',  ( -12.35395094432871410, -20.26789845123980527, 68.59303345011528563 ) ) ;
#40324=CARTESIAN_POINT ( 'NONE',  ( -22.22370946352282672, -9.111183370010303761, 59.90666632495347699 ) ) ;
#40325=ORIENTED_EDGE ( 'NONE', *, *, #23442, .T. ) ;
#40326=ORIENTED_EDGE ( 'NONE', *, *, #16423, .F. ) ;
#40328=CARTESIAN_POINT ( 'NONE',  ( -21.80947398209100285, -9.353160252369512762, 63.49153755919518005 ) ) ;
#40329=CARTESIAN_POINT ( 'NONE',  ( -11.01524411412108151, -17.62491020911333450, 71.56718188073510589 ) ) ;
#40330=CARTESIAN_POINT ( 'NONE',  ( -18.54539007733004397, -7.443902428285554151, 74.00097724639977059 ) ) ;
#40331=VERTEX_POINT ( 'NONE', #2545 ) ;
#40332=EDGE_CURVE ( 'NONE', #13421, #27240, #21014, .T. ) ;
#40334=ORIENTED_EDGE ( 'NONE', *, *, #45438, .F. ) ;
#40335=CARTESIAN_POINT ( 'NONE',  ( -14.59650283654637271, -21.27602155829186259, 61.78033139454115030 ) ) ;
#40336=CARTESIAN_POINT ( 'NONE',  ( -23.98955618046187865, -11.28797293959267023, 66.59931407123043812 ) ) ;
#40339=FACE_OUTER_BOUND ( 'NONE', #8431, .T. ) ;
#40340=VERTEX_POINT ( 'NONE', #25660 ) ;
#40341=B_SPLINE_CURVE_WITH_KNOTS ( 'NONE', 3,
 ( #23199, #537, #4468, #30837, #30352, #7700, #45853, #4000, #37450, #34752 ),
 .UNSPECIFIED., .F., .F.,
 ( 4, 2, 2, 2, 4 ),
 ( 0.000000000000000000, 0.2500000000000000000, 0.5000000000000000000, 0.7500000000000000000, 1.000000000000000000 ),
 .UNSPECIFIED. ) ;
#40343=CARTESIAN_POINT ( 'NONE',  ( -12.78931795874336430, -9.563283354468385511, 74.60457613011958244 ) ) ;
#40344=ADVANCED_FACE ( 'NONE', ( #36971 ), #14790, .T. ) ;
#40345=DIRECTION ( 'NONE',  ( 0.9372362738803845517, 0.3486949482324239735, -5.386914174890155429E-09 ) ) ;
#40347=( BOUNDED_CURVE ( )  B_SPLINE_CURVE ( 3, ( #3926, #4174, #34419, #11307 ),
 .UNSPECIFIED., .F., .F. ) 
 B_SPLINE_CURVE_WITH_KNOTS ( ( 4, 4 ),
 ( 0.4074455897393696180, 0.5000000000000000000 ),
 .UNSPECIFIED. ) 
 CURVE ( )  GEOMETRIC_REPRESENTATION_ITEM ( )  RATIONAL_B_SPLINE_CURVE ( ( 0.6983129098261106060, 0.7760317562606908748, 0.8765941196519806411, 0.9999999999999641398 ) ) 
 REPRESENTATION_ITEM ( '' )  );
#40349=EDGE_LOOP ( 'NONE', ( #39090, #7556, #6540, #10549, #47497 ) ) ;
#40350=CARTESIAN_POINT ( 'NONE',  ( -20.95199379672471096, -20.85531803099279458, 65.88453983062113650 ) ) ;
#40351=ORIENTED_EDGE ( 'NONE', *, *, #14353, .T. ) ;
#40354=VERTEX_POINT ( 'NONE', #6958 ) ;
#40358=CARTESIAN_POINT ( 'NONE',  ( -18.71757194967216975, -7.929750632967406787, 70.37068030597254165 ) ) ;
#40359=EDGE_CURVE ( 'NONE', #39039, #30917, #2251, .T. ) ;
#40361=( BOUNDED_CURVE ( )  B_SPLINE_CURVE ( 3, ( #20844, #24309, #35607, #35370 ),
 .UNSPECIFIED., .F., .F. ) 
 B_SPLINE_CURVE_WITH_KNOTS ( ( 4, 4 ),
 ( 0.4074455897393707837, 0.5000000000000000000 ),
 .UNSPECIFIED. ) 
 CURVE ( )  GEOMETRIC_REPRESENTATION_ITEM ( )  RATIONAL_B_SPLINE_CURVE ( ( 0.6983129098261093848, 0.7760317562607007558, 0.8765941196519941858, 0.9999999999999816813 ) ) 
 REPRESENTATION_ITEM ( '' )  );
#40362=CARTESIAN_POINT ( 'NONE',  ( -20.12289019246589206, -7.865124395032225380, 73.90592041591946781 ) ) ;
#40364=( BOUNDED_CURVE ( )  B_SPLINE_CURVE ( 3, ( #4492, #15553, #45153, #41685 ),
 .UNSPECIFIED., .F., .F. ) 
 B_SPLINE_CURVE_WITH_KNOTS ( ( 4, 4 ),
 ( 0.4074455897393695625, 0.5000000000000000000 ),
 .UNSPECIFIED. ) 
 CURVE ( )  GEOMETRIC_REPRESENTATION_ITEM ( )  RATIONAL_B_SPLINE_CURVE ( ( 0.6983129098261096068, 0.7760317562606910968, 0.8765941196519815293, 0.9999999999999659162 ) ) 
 REPRESENTATION_ITEM ( '' )  );
#40365=CARTESIAN_POINT ( 'NONE',  ( -19.97164353606484255, -21.81018995992316079, 69.11977899231902711 ) ) ;
#40367=CARTESIAN_POINT ( 'NONE',  ( -11.95960950777170062, -10.43434529725880466, 67.69000071772322258 ) ) ;
#40369=VECTOR ( 'NONE', #32658, 1000.000000000000114 ) ;
#40371=ORIENTED_EDGE ( 'NONE', *, *, #20068, .F. ) ;
#40372=CARTESIAN_POINT ( 'NONE',  ( -23.34092575347512266, -10.28207967581048088, 59.78698817202694471 ) ) ;
#40373=CARTESIAN_POINT ( 'NONE',  ( -11.88348671940001999, -10.53106331603155077, 70.98395522823196302 ) ) ;
#40374=EDGE_LOOP ( 'NONE', ( #45288, #45900, #10094, #18189, #40326 ) ) ;
#40375=CARTESIAN_POINT ( 'NONE',  ( -11.42587710518540334, -11.10406226247761019, 57.49431069621225276 ) ) ;
#40377=DIRECTION ( 'NONE',  ( -5.731567514496413899E-31, -1.020425574103664789E-16, -1.000000000000000000 ) ) ;
#40379=( BOUNDED_SURFACE ( )  B_SPLINE_SURFACE ( 3, 1, ( 
 ( #6915, #18714 ),
 ( #17978, #33728 ),
 ( #15010, #30073 ),
 ( #18975, #18225 ),
 ( #48273, #7176 ),
 ( #11345, #14749 ),
 ( #29821, #44850 ) ),
 .UNSPECIFIED., .T., .F., .F. ) 
 B_SPLINE_SURFACE_WITH_KNOTS ( ( 4, 3, 4 ),
 ( 2, 2 ),
 ( 0.000000000000000000, 0.5000000000000000000, 1.000000000000000000 ),
 ( 0.000000000000000000, 1.000000000000000000 ),
 .UNSPECIFIED. ) 
 GEOMETRIC_REPRESENTATION_ITEM ( )  RATIONAL_B_SPLINE_SURFACE ( (
 ( 1.000000000000000000, 1.000000000000000000),
 ( 0.3333333333333335369, 0.3333333333333330373),
 ( 0.3333333333333335369, 0.3333333333333330373),
 ( 1.000000000000000000, 1.000000000000000000),
 ( 0.3333333333333333703, 0.3333333333333333703),
 ( 0.3333333333333333703, 0.3333333333333333703),
 ( 1.000000000000000000, 1.000000000000000000) ) ) 
 REPRESENTATION_ITEM ( '' )  SURFACE ( )  );
#40380=VERTEX_POINT ( 'NONE', #6715 ) ;
#40381=CARTESIAN_POINT ( 'NONE',  ( -20.78299823145727387, -8.610459808214880439, 59.85597358678664648 ) ) ;
#40382=CARTESIAN_POINT ( 'NONE',  ( -17.19980194945414809, -7.762775306501539241, 70.64035839668011363 ) ) ;
#40383=CARTESIAN_POINT ( 'NONE',  ( -16.56702387822477363, -22.20979222136662656, 65.33226067334068432 ) ) ;
#40387=CARTESIAN_POINT ( 'NONE',  ( -17.68062394802985793, -21.85468638579756373, 58.41113140978044527 ) ) ;
#40388=LINE ( 'NONE', #47775, #37054 ) ;
#40389=CARTESIAN_POINT ( 'NONE',  ( -23.89200480383413350, -11.11192299349349533, 70.07706151945906470 ) ) ;
#40390=CARTESIAN_POINT ( 'NONE',  ( -11.37338168604670408, -19.15691247995520996, 71.87341272242258583 ) ) ;
#40391=ORIENTED_EDGE ( 'NONE', *, *, #45324, .T. ) ;
#40392=EDGE_CURVE ( 'NONE', #42072, #36064, #14314, .T. ) ;
#40393=CARTESIAN_POINT ( 'NONE',  ( -24.45201636468675943, -14.25170757634699825, 69.95275273439749242 ) ) ;
#40394=CARTESIAN_POINT ( 'NONE',  ( -12.47302444406249933, -9.241390648102244754, 74.43267637782378188 ) ) ;
#40397=CARTESIAN_POINT ( 'NONE',  ( -13.64450405064090788, -21.22941549479649126, 68.57908268650601258 ) ) ;
#40398=CARTESIAN_POINT ( 'NONE',  ( -12.99758330771203951, -9.386476247090117297, 70.84925353123610137 ) ) ;
#40399=CYLINDRICAL_SURFACE ( 'NONE', #28877, 0.1500000000000063227 ) ;
#40400=EDGE_LOOP ( 'NONE', ( #29792, #31493, #38244, #2820, #26233 ) ) ;
#40401=CARTESIAN_POINT ( 'NONE',  ( -14.65765131015531253, -21.78034674156931061, 53.49999999999994316 ) ) ;
#40402=VERTEX_POINT ( 'NONE', #10423 ) ;
#40403=FACE_OUTER_BOUND ( 'NONE', #18243, .T. ) ;
#40405=EDGE_CURVE ( 'NONE', #8735, #26020, #32639, .T. ) ;
#40406=PLANE ( 'NONE',  #5354 ) ;
#40407=ORIENTED_EDGE ( 'NONE', *, *, #41868, .F. ) ;
#40409=CARTESIAN_POINT ( 'NONE',  ( -24.02655296236175175, -11.35792967378293916, 66.53719098615387395 ) ) ;
#40410=DIRECTION ( 'NONE',  ( 0.4007314504464623006, -0.1985303619678229492, 0.8944271909999157444 ) ) ;
#40411=EDGE_CURVE ( 'NONE', #3011, #38799, #27430, .T. ) ;
#40412=CARTESIAN_POINT ( 'NONE',  ( -10.05141141991806641, -15.87983426743701543, 64.60797347950868641 ) ) ;
#40414=DIRECTION ( 'NONE',  ( 0.6408936281290997794, 0.7676297007174212039, 4.260501105223829885E-08 ) ) ;
#40415=ORIENTED_EDGE ( 'NONE', *, *, #43427, .F. ) ;
#40416=CARTESIAN_POINT ( 'NONE',  ( -12.12786991918758339, -13.32596279628197600, 53.49999999999995026 ) ) ;
#40417=CARTESIAN_POINT ( 'NONE',  ( -16.09337498760136853, -22.13948385882417824, 58.40090183616962349 ) ) ;
#40418=CARTESIAN_POINT ( 'NONE',  ( -23.98474799315784978, -17.25007060033011896, 69.41339792561625188 ) ) ;
#40419=CARTESIAN_POINT ( 'NONE',  ( -13.17770392829461912, -20.93059606819637608, 58.15311748147730952 ) ) ;
#40420=DIRECTION ( 'NONE',  ( 0.9163203205182083311, 0.4004460890125009498, -2.380681616944615543E-09 ) ) ;
#40422=ORIENTED_EDGE ( 'NONE', *, *, #32814, .F. ) ;
#40424=CARTESIAN_POINT ( 'NONE',  ( -23.68653687815194786, -11.57061008776567945, 66.43686604568146947 ) ) ;
#40425=CARTESIAN_POINT ( 'NONE',  ( -21.73662441638723308, -9.231682010981758779, 66.67622112302015580 ) ) ;
#40427=FACE_OUTER_BOUND ( 'NONE', #35188, .T. ) ;
#40428=CARTESIAN_POINT ( 'NONE',  ( -11.71830028707309523, -18.86652491371886242, 71.91515846292473668 ) ) ;
#40429=CARTESIAN_POINT ( 'NONE',  ( -15.34465393633500518, -21.54586957516256263, 68.86120835375241711 ) ) ;
#40430=CARTESIAN_POINT ( 'NONE',  ( -10.40888613812686359, -14.10966362093629378, 61.06821293886368807 ) ) ;
#40431=DIRECTION ( 'NONE',  ( -5.731567514496413899E-31, -1.020425574103664789E-16, -1.000000000000000000 ) ) ;
#40433=CARTESIAN_POINT ( 'NONE',  ( -24.35389707626741185, -16.10709931453381216, 62.87856533165624029 ) ) ;
#40434=ADVANCED_FACE ( 'NONE', ( #48558 ), #7463, .T. ) ;
#40437=CARTESIAN_POINT ( 'NONE',  ( -23.75797251732913296, -17.78947179557082592, 59.00378417803962350 ) ) ;
#40439=ADVANCED_FACE ( 'NONE', ( #1028 ), #541, .T. ) ;
#40441=CARTESIAN_POINT ( 'NONE',  ( -10.39679176622870038, -14.24023819782134481, 64.40275955115841100 ) ) ;
#40443=CARTESIAN_POINT ( 'NONE',  ( -21.02642643314752036, -20.81301377900324212, 69.24377353718439565 ) ) ;
#40444=CARTESIAN_POINT ( 'NONE',  ( -13.77494768682002935, -20.78293651617081750, 65.28628829308328818 ) ) ;
#40445=CARTESIAN_POINT ( 'NONE',  ( -11.58273428586415221, -10.94902261066962978, 57.31976413542670201 ) ) ;
#40446=ORIENTED_EDGE ( 'NONE', *, *, #33947, .F. ) ;
#40449=ORIENTED_EDGE ( 'NONE', *, *, #32593, .T. ) ;
#40451=CARTESIAN_POINT ( 'NONE',  ( -19.03885666732217885, -7.536228653801991584, 67.15717731432056326 ) ) ;
#40452=( BOUNDED_CURVE ( )  B_SPLINE_CURVE ( 3, ( #26991, #19856, #24037, #414 ),
 .UNSPECIFIED., .F., .F. ) 
 B_SPLINE_CURVE_WITH_KNOTS ( ( 4, 4 ),
 ( 0.5000000000000000000, 0.9074455897393708392 ),
 .UNSPECIFIED. ) 
 CURVE ( )  GEOMETRIC_REPRESENTATION_ITEM ( )  RATIONAL_B_SPLINE_CURVE ( ( 1.000000000000017986, 0.4567392136813231973, 0.3561768502900144462, 0.6983129098261110501 ) ) 
 REPRESENTATION_ITEM ( '' )  );
#40455=CARTESIAN_POINT ( 'NONE',  ( -15.55171133418867235, -7.598245370416885969, 70.79485226425863686 ) ) ;
#40457=CARTESIAN_POINT ( 'NONE',  ( -13.47381639519378105, -21.12577003491056260, 65.24274829841968426 ) ) ;
#40458=CARTESIAN_POINT ( 'NONE',  ( -23.23520415037899411, -10.14728669485665691, 63.22185993134614534 ) ) ;
#40460=CARTESIAN_POINT ( 'NONE',  ( -15.28291115335697192, -21.52618774670101232, 68.72592918174676413 ) ) ;
#40462=EDGE_LOOP ( 'NONE', ( #41047, #11170, #14651, #4515, #27837 ) ) ;
#40463=B_SPLINE_CURVE_WITH_KNOTS ( 'NONE', 3,
 ( #22992, #328, #15312, #30376, #22484, #45876, #26185, #27150, #7483, #37977 ),
 .UNSPECIFIED., .F., .F.,
 ( 4, 2, 2, 2, 4 ),
 ( 0.000000000000000000, 0.2500000000000000000, 0.5000000000000000000, 0.7500000000000000000, 1.000000000000000000 ),
 .UNSPECIFIED. ) ;
#40464=FACE_OUTER_BOUND ( 'NONE', #22021, .T. ) ;
#40465=CARTESIAN_POINT ( 'NONE',  ( -10.33531692083374587, -17.10115316349580894, 57.87255846826901262 ) ) ;
#40468=DIRECTION ( 'NONE',  ( -5.731567514496413899E-31, -1.020425574103664789E-16, -1.000000000000000000 ) ) ;
#40470=CARTESIAN_POINT ( 'NONE',  ( -24.05420634179087358, -17.20676946999824608, 69.69867738674849988 ) ) ;
#40471=CARTESIAN_POINT ( 'NONE',  ( -15.11195830621016256, -21.41632612911037370, 65.40596681519618016 ) ) ;
#40472=CARTESIAN_POINT ( 'NONE',  ( -23.92992157843938728, -17.39298733450930001, 66.24357246489365991 ) ) ;
#40473=EDGE_LOOP ( 'NONE', ( #39045, #25165, #17661, #34379, #31814 ) ) ;
#40475=CARTESIAN_POINT ( 'NONE',  ( -10.72789316105772528, -12.76937900761250155, 60.90739623444811457 ) ) ;
#40476=CARTESIAN_POINT ( 'NONE',  ( -23.30963478160716562, -18.69084381296369912, 69.30844128244088154 ) ) ;
#40478=CARTESIAN_POINT ( 'NONE',  ( -10.12326195556307695, -13.32541703369907893, 74.86313051124790263 ) ) ;
#40479=PLANE ( 'NONE',  #28913 ) ;
#40480=VERTEX_POINT ( 'NONE', #23440 ) ;
#40481=CARTESIAN_POINT ( 'NONE',  ( -24.33626633208317713, -17.58850949613905001, 66.04333621789641029 ) ) ;
#40486=ORIENTED_EDGE ( 'NONE', *, *, #9959, .T. ) ;
#40487=EDGE_CURVE ( 'NONE', #43456, #15655, #16730, .T. ) ;
#40491=B_SPLINE_CURVE_WITH_KNOTS ( 'NONE', 3,
 ( #32378, #6515, #21296, #36042, #28674, #6017, #21536, #16607, #47149, #13144 ),
 .UNSPECIFIED., .F., .F.,
 ( 4, 2, 2, 2, 4 ),
 ( 0.6272669072877486984, 0.7522669073072625334, 0.8772669073267762574, 1.002266907346290203, 1.127266907365803927 ),
 .UNSPECIFIED. ) ;
#40492=CARTESIAN_POINT ( 'NONE',  ( -14.34311226469532841, -8.523215522210126238, 70.74574244503894249 ) ) ;
#40493=( BOUNDED_SURFACE ( )  B_SPLINE_SURFACE ( 3, 1, ( 
 ( #38421, #46321 ),
 ( #19472, #7935 ),
 ( #35215, #4710 ),
 ( #23424, #16009 ),
 ( #37943, #4457 ),
 ( #19238, #38917 ),
 ( #38676, #23679 ) ),
 .UNSPECIFIED., .T., .F., .F. ) 
 B_SPLINE_SURFACE_WITH_KNOTS ( ( 4, 3, 4 ),
 ( 2, 2 ),
 ( 0.000000000000000000, 0.5000000000000000000, 1.000000000000000000 ),
 ( 0.000000000000000000, 1.000000000000000000 ),
 .UNSPECIFIED. ) 
 GEOMETRIC_REPRESENTATION_ITEM ( )  RATIONAL_B_SPLINE_SURFACE ( (
 ( 1.000000000000000000, 1.000000000000000000),
 ( 0.3333333333333335369, 0.3333333333333330373),
 ( 0.3333333333333335369, 0.3333333333333330373),
 ( 1.000000000000000000, 1.000000000000000000),
 ( 0.3333333333333333703, 0.3333333333333333703),
 ( 0.3333333333333333703, 0.3333333333333333703),
 ( 1.000000000000000000, 1.000000000000000000) ) ) 
 REPRESENTATION_ITEM ( '' )  SURFACE ( )  );
#40495=CARTESIAN_POINT ( 'NONE',  ( -13.16256456194319391, -9.182988408105495992, 60.59517097614691039 ) ) ;
#40496=VERTEX_POINT ( 'NONE', #38692 ) ;
#40497=ORIENTED_EDGE ( 'NONE', *, *, #24071, .F. ) ;
#40498=AXIS2_PLACEMENT_3D ( 'NONE', #25906, #22215, #10647 ) ;
#40499=EDGE_CURVE ( 'NONE', #4075, #25448, #22696, .T. ) ;
#40500=EDGE_CURVE ( 'NONE', #33937, #47544, #47888, .T. ) ;
#40502=CARTESIAN_POINT ( 'NONE',  ( -10.81230840161673967, -17.25685697075765646, 64.64211442681141762 ) ) ;
#40503=LINE ( 'NONE', #36318, #41806 ) ;
#40505=( BOUNDED_CURVE ( )  B_SPLINE_CURVE ( 3, ( #5797, #17084, #35572, #43469 ),
 .UNSPECIFIED., .F., .F. ) 
 B_SPLINE_CURVE_WITH_KNOTS ( ( 4, 4 ),
 ( 0.9074455897393701731, 1.000000000000000000 ),
 .UNSPECIFIED. ) 
 CURVE ( )  GEOMETRIC_REPRESENTATION_ITEM ( )  RATIONAL_B_SPLINE_CURVE ( ( 0.6983129098261056100, 0.7760317562607090824, 0.8765941196520071754, 1.000000000000000000 ) ) 
 REPRESENTATION_ITEM ( '' )  );
#40506=EDGE_LOOP ( 'NONE', ( #3200, #35403, #48498, #18670, #3159 ) ) ;
#40508=CARTESIAN_POINT ( 'NONE',  ( -10.40277084706750621, -15.44444119821074501, 57.86792809062919218 ) ) ;
#40510=CARTESIAN_POINT ( 'NONE',  ( -10.13784000599894597, -13.25541019000276499, 74.79322239981686948 ) ) ;
#40511=ORIENTED_EDGE ( 'NONE', *, *, #29378, .T. ) ;
#40512=CARTESIAN_POINT ( 'NONE',  ( -11.22967194918012268, -11.54873428709711902, 67.61864634137779717 ) ) ;
#40514=CARTESIAN_POINT ( 'NONE',  ( -22.46951418628932728, -9.956841189560520888, 73.48161090405926643 ) ) ;
#40515=CARTESIAN_POINT ( 'NONE',  ( -24.83596929353047145, -14.05522739703532054, 73.24554619393663302 ) ) ;
#40516=CARTESIAN_POINT ( 'NONE',  ( -18.72680718162379421, -7.880610904852766829, 70.67068030199192208 ) ) ;
#40518=VERTEX_POINT ( 'NONE', #4471 ) ;
#40519=CARTESIAN_POINT ( 'NONE',  ( -12.99758330771203951, -9.386476247090117297, 70.84925353123610137 ) ) ;
#40522=CARTESIAN_POINT ( 'NONE',  ( -24.32752796592761158, -15.96791130369872391, 66.06324927019940674 ) ) ;
#40526=CARTESIAN_POINT ( 'NONE',  ( -10.71355325306214645, -11.57327142899409189, 71.28849651251223918 ) ) ;
#40529=CARTESIAN_POINT ( 'NONE',  ( -11.72362823715024227, -10.74660985594761797, 74.54770848788524518 ) ) ;
#40530=ORIENTED_EDGE ( 'NONE', *, *, #40554, .F. ) ;
#40531=DIRECTION ( 'NONE',  ( -5.731567514496413899E-31, -1.020425574103664789E-16, -1.000000000000000000 ) ) ;
#40532=CARTESIAN_POINT ( 'NONE',  ( -13.18904211892902367, -11.30002761096173280, 54.07175714974879099 ) ) ;
#40533=DIRECTION ( 'NONE',  ( -0.3566357048164924826, 0.9342435303763381160, -8.054691247152028744E-09 ) ) ;
#40534=CARTESIAN_POINT ( 'NONE',  ( -23.43742028209110373, -18.48928452435560743, 72.76368265771812105 ) ) ;
#40535=ORIENTED_EDGE ( 'NONE', *, *, #29551, .T. ) ;
#40536=CARTESIAN_POINT ( 'NONE',  ( -10.45863924090583552, -14.11462608630872317, 61.21821294130609914 ) ) ;
#40537=CARTESIAN_POINT ( 'NONE',  ( -24.17899325218984785, -11.66673737571591296, 59.66731058339561855 ) ) ;
#40538=CARTESIAN_POINT ( 'NONE',  ( -23.32531047696446080, -18.57448983302084855, 69.29371930760996179 ) ) ;
#40540=DIRECTION ( 'NONE',  ( -0.4749924142254751680, -0.8799898899579781109, -8.916637576350562172E-09 ) ) ;
#40543=ORIENTED_EDGE ( 'NONE', *, *, #797, .T. ) ;
#40544=ORIENTED_EDGE ( 'NONE', *, *, #40837, .T. ) ;
#40545=CARTESIAN_POINT ( 'NONE',  ( -24.16575343130564590, -12.74704122656904914, 69.92243002240397232 ) ) ;
#40548=CARTESIAN_POINT ( 'NONE',  ( -20.69509252757554307, -8.115601716887088202, 63.49616818922779515 ) ) ;
#40550=CARTESIAN_POINT ( 'NONE',  ( -25.31403878743076774, -21.34684298153750603, 53.49999999999995026 ) ) ;
#40552=ORIENTED_EDGE ( 'NONE', *, *, #12885, .T. ) ;
#40553=ORIENTED_EDGE ( 'NONE', *, *, #21755, .F. ) ;
#40554=EDGE_CURVE ( 'NONE', #31720, #24011, #7309, .T. ) ;
#40555=DIRECTION ( 'NONE',  ( 0.2843796944294933460, 0.9587117342539337450, 5.205739956168971478E-08 ) ) ;
#40558=CARTESIAN_POINT ( 'NONE',  ( -21.91378931226059024, -9.437005245162470857, 63.41983640775033848 ) ) ;
#40559=CARTESIAN_POINT ( 'NONE',  ( -19.04042241193164386, -7.536568769452434147, 67.01576393362593365 ) ) ;
#40560=CARTESIAN_POINT ( 'NONE',  ( -18.62265789082445622, -7.456197966475932581, 73.94790266681903290 ) ) ;
#40561=EDGE_CURVE ( 'NONE', #44055, #32492, #39686, .T. ) ;
#40562=ORIENTED_EDGE ( 'NONE', *, *, #14735, .T. ) ;
#40566=CARTESIAN_POINT ( 'NONE',  ( -12.69763806180496601, -20.04058448603118592, 68.62185382311069759 ) ) ;
#40568=CARTESIAN_POINT ( 'NONE',  ( -12.00532783130394776, -19.33158900886926546, 58.07115174146640157 ) ) ;
#40572=CARTESIAN_POINT ( 'NONE',  ( -21.62177555926896133, -9.207315420440883358, 66.66149954055094895 ) ) ;
#40573=ORIENTED_EDGE ( 'NONE', *, *, #2901, .T. ) ;
#40574=CARTESIAN_POINT ( 'NONE',  ( -15.11195812866605692, -21.41632606413040918, 65.10596681519622564 ) ) ;
#40575=DIRECTION ( 'NONE',  ( 0.8037372918934696520, -0.5949843406508663612, -7.322964617522714932E-08 ) ) ;
#40577=CARTESIAN_POINT ( 'NONE',  ( -20.87058525438150625, -20.90343409458096602, 65.81283875100656644 ) ) ;
#40578=ORIENTED_EDGE ( 'NONE', *, *, #39724, .T. ) ;
#40579=CARTESIAN_POINT ( 'NONE',  ( -23.85820194903862657, -17.69173191509663567, 62.48833042115954584 ) ) ;
#40580=CARTESIAN_POINT ( 'NONE',  ( -11.50075376218807754, -18.54175998082050825, 64.81877447156344374 ) ) ;
#40581=ORIENTED_EDGE ( 'NONE', *, *, #40832, .F. ) ;
#40582=CARTESIAN_POINT ( 'NONE',  ( -13.71293426195967413, -21.26916566922604801, 68.64120525947689089 ) ) ;
#40583=FACE_OUTER_BOUND ( 'NONE', #43191, .T. ) ;
#40584=ORIENTED_EDGE ( 'NONE', *, *, #31976, .T. ) ;
#40586=EDGE_CURVE ( 'NONE', #166, #35459, #27918, .T. ) ;
#40587=CARTESIAN_POINT ( 'NONE',  ( -19.63995608841934626, -21.92282860479379991, 65.65141533869274326 ) ) ;
#40588=CARTESIAN_POINT ( 'NONE',  ( -24.86203810447890561, -14.38333402024011143, 66.36009642219894999 ) ) ;
#40589=ORIENTED_EDGE ( 'NONE', *, *, #5408, .F. ) ;
#40590=CARTESIAN_POINT ( 'NONE',  ( -13.38462506958126141, -20.58719851387657940, 58.04650077714654088 ) ) ;
#40591=VECTOR ( 'NONE', #31019, 1000.000000000000000 ) ;
#40592=AXIS2_PLACEMENT_3D ( 'NONE', #28227, #5593, #42535 ) ;
#40593=DIRECTION ( 'NONE',  ( -2.331190579393116502E-06, 8.511884082828543324E-06, -0.9999999999610567070 ) ) ;
#40596=EDGE_LOOP ( 'NONE', ( #24759, #32659, #39707, #17481, #25876 ) ) ;
#40597=CARTESIAN_POINT ( 'NONE',  ( -23.37892143032667391, -10.33223586073257572, 59.79541750854375692 ) ) ;
#40598=CARTESIAN_POINT ( 'NONE',  ( -11.90535080888287212, -10.50279376357651095, 70.96893075550114816 ) ) ;
#40599=DIRECTION ( 'NONE',  ( -0.4156784896208465252, -0.1649587623211697662, 0.8944271909999157444 ) ) ;
#40600=B_SPLINE_CURVE_WITH_KNOTS ( 'NONE', 1,
 ( #35575, #24756 ),
 .UNSPECIFIED., .F., .F.,
 ( 2, 2 ),
 ( 0.000000000000000000, 1.000000000000000000 ),
 .UNSPECIFIED. ) ;
#40602=CARTESIAN_POINT ( 'NONE',  ( -17.42409385541300892, -14.80920654474439502, 75.49999999999994316 ) ) ;
#40603=CARTESIAN_POINT ( 'NONE',  ( -13.06813783877040969, -9.265530354883374287, 67.66470656304637998 ) ) ;
#40604=CARTESIAN_POINT ( 'NONE',  ( -15.62222905942472018, -7.993050613273783966, 70.89517703929612935 ) ) ;
#40607=FACE_OUTER_BOUND ( 'NONE', #46936, .T. ) ;
#40609=EDGE_CURVE ( 'NONE', #43726, #2066, #46152, .T. ) ;
#40611=CARTESIAN_POINT ( 'NONE',  ( -13.46747890590686403, -9.034676489092227314, 60.43950277890026967 ) ) ;
#40612=EDGE_CURVE ( 'NONE', #14770, #2068, #46813, .T. ) ;
#40614=EDGE_CURVE ( 'NONE', #33854, #24550, #7435, .T. ) ;
#40615=ORIENTED_EDGE ( 'NONE', *, *, #8824, .F. ) ;
#40616=CARTESIAN_POINT ( 'NONE',  ( -20.70232273485035890, -8.624288160964143302, 60.14125250309182036 ) ) ;
#40617=DIRECTION ( 'NONE',  ( -8.339041841313433703E-07, -7.401745998521586792E-06, 0.9999999999722594124 ) ) ;
#40618=CARTESIAN_POINT ( 'NONE',  ( -15.93879930885702656, -7.917138641544857691, 67.15479422225767792 ) ) ;
#40619=CARTESIAN_POINT ( 'NONE',  ( -11.41592704872699748, -19.21438508446953364, 71.94331831479362904 ) ) ;
#40620=ADVANCED_FACE ( 'NONE', ( #20477 ), #42540, .T. ) ;
#40621=( BOUNDED_CURVE ( )  B_SPLINE_CURVE ( 3, ( #6651, #21443, #6170, #10588 ),
 .UNSPECIFIED., .F., .F. ) 
 B_SPLINE_CURVE_WITH_KNOTS ( ( 4, 4 ),
 ( 0.000000000000000000, 0.4074455897393706727 ),
 .UNSPECIFIED. ) 
 CURVE ( )  GEOMETRIC_REPRESENTATION_ITEM ( )  RATIONAL_B_SPLINE_CURVE ( ( 1.000000000000000000, 0.4567392136813168690, 0.3561768502900247158, 0.6983129098261233736 ) ) 
 REPRESENTATION_ITEM ( '' )  );
#40623=CARTESIAN_POINT ( 'NONE',  ( -24.06787342886325121, -18.28917680027896608, 53.49999999999994316 ) ) ;
#40624=AXIS2_PLACEMENT_3D ( 'NONE', #36900, #18193, #33201 ) ;
#40625=AXIS2_PLACEMENT_3D ( 'NONE', #43449, #47137, #1830 ) ;
#40626=LINE ( 'NONE', #10121, #17040 ) ;
#40627=ORIENTED_EDGE ( 'NONE', *, *, #8780, .F. ) ;
#40628=CARTESIAN_POINT ( 'NONE',  ( -13.70633956305045409, -21.26533489984594283, 68.64899269501005108 ) ) ;
#40629=AXIS2_PLACEMENT_3D ( 'NONE', #22536, #149, #41492 ) ;
#40630=CARTESIAN_POINT ( 'NONE',  ( -12.55524250210389425, -20.44813591936859609, 71.91315377446979085 ) ) ;
#40631=CARTESIAN_POINT ( 'NONE',  ( -14.91112529534803066, -8.221969756899694559, 57.13527940342243028 ) ) ;
#40632=( BOUNDED_CURVE ( )  B_SPLINE_CURVE ( 3, ( #32186, #47678, #13445, #36341 ),
 .UNSPECIFIED., .F., .F. ) 
 B_SPLINE_CURVE_WITH_KNOTS ( ( 4, 4 ),
 ( 0.9074455897393706172, 1.000000000000000000 ),
 .UNSPECIFIED. ) 
 CURVE ( )  GEOMETRIC_REPRESENTATION_ITEM ( )  RATIONAL_B_SPLINE_CURVE ( ( 0.6983129098261082746, 0.7760317562607114139, 0.8765941196520086187, 1.000000000000000000 ) ) 
 REPRESENTATION_ITEM ( '' )  );
#40633=ORIENTED_EDGE ( 'NONE', *, *, #24197, .F. ) ;
#40634=( BOUNDED_CURVE ( )  B_SPLINE_CURVE ( 3, ( #490, #8360, #38374, #15968 ),
 .UNSPECIFIED., .F., .F. ) 
 B_SPLINE_CURVE_WITH_KNOTS ( ( 4, 4 ),
 ( 0.9074455897393635118, 1.000000000000000000 ),
 .UNSPECIFIED. ) 
 CURVE ( )  GEOMETRIC_REPRESENTATION_ITEM ( )  RATIONAL_B_SPLINE_CURVE ( ( 0.6983129098260831835, 0.7760317562606896535, 0.8765941196519952960, 1.000000000000000000 ) ) 
 REPRESENTATION_ITEM ( '' )  );
#40635=CARTESIAN_POINT ( 'NONE',  ( -12.01648241349452917, -10.28590705807702932, 67.49896869922172016 ) ) ;
#40636=ORIENTED_EDGE ( 'NONE', *, *, #28908, .T. ) ;
#40637=CARTESIAN_POINT ( 'NONE',  ( -10.47154223249567728, -17.48601752977970492, 64.82013545767874518 ) ) ;
#40638=CARTESIAN_POINT ( 'NONE',  ( -23.65624121974494898, -11.51332442490695307, 66.42214514605623776 ) ) ;
#40639=ORIENTED_EDGE ( 'NONE', *, *, #45578, .F. ) ;
#40640=DIRECTION ( 'NONE',  ( 0.9410372374137780938, 0.3383029970317210089, 1.029646055599927174E-09 ) ) ;
#40641=CARTESIAN_POINT ( 'NONE',  ( -20.06975372951847447, -8.274133229585533655, 73.73568642813194174 ) ) ;
#40643=DIRECTION ( 'NONE',  ( 4.116680954457742276E-07, 3.835121109574216710E-07, 0.9999999999998415712 ) ) ;
#40646=CARTESIAN_POINT ( 'NONE',  ( -10.52422430310768320, -17.61911375464911700, 68.21226508126260057 ) ) ;
#40647=CARTESIAN_POINT ( 'NONE',  ( -12.27604185553471616, -19.62628656662749549, 58.21210303282668264 ) ) ;
#40649=CARTESIAN_POINT ( 'NONE',  ( -24.87177708793343811, -14.62301390258337896, 62.81272869172535422 ) ) ;
#40650=( BOUNDED_SURFACE ( )  B_SPLINE_SURFACE ( 3, 1, ( 
 ( #25858, #22175 ),
 ( #3444, #36435 ),
 ( #31627, #42944 ),
 ( #24244, #39250 ),
 ( #9467, #5532 ),
 ( #20551, #1824 ),
 ( #31862, #13122 ) ),
 .UNSPECIFIED., .T., .F., .F. ) 
 B_SPLINE_SURFACE_WITH_KNOTS ( ( 4, 3, 4 ),
 ( 2, 2 ),
 ( 0.000000000000000000, 0.5000000000000000000, 1.000000000000000000 ),
 ( 0.000000000000000000, 1.000000000000000000 ),
 .UNSPECIFIED. ) 
 GEOMETRIC_REPRESENTATION_ITEM ( )  RATIONAL_B_SPLINE_SURFACE ( (
 ( 1.000000000000000000, 1.000000000000000000),
 ( 0.3333333333333335369, 0.3333333333333330373),
 ( 0.3333333333333335369, 0.3333333333333330373),
 ( 1.000000000000000000, 1.000000000000000000),
 ( 0.3333333333333333703, 0.3333333333333333703),
 ( 0.3333333333333333703, 0.3333333333333333703),
 ( 1.000000000000000000, 1.000000000000000000) ) ) 
 REPRESENTATION_ITEM ( '' )  SURFACE ( )  );
#40651=CARTESIAN_POINT ( 'NONE',  ( -10.43125892716163960, -13.91323834088958122, 57.44825034920751960 ) ) ;
#40652=CARTESIAN_POINT ( 'NONE',  ( -22.69189081882976566, -20.07747925453471183, 69.35134909049985197 ) ) ;
#40653=CYLINDRICAL_SURFACE ( 'NONE', #43119, 0.1500000000000043521 ) ;
#40654=CARTESIAN_POINT ( 'NONE',  ( -13.49409790474204840, -20.66256726344224504, 61.53118467422925164 ) ) ;
#40655=CARTESIAN_POINT ( 'NONE',  ( -24.29232374648589854, -16.16102685949518403, 62.89328677060923667 ) ) ;
#40657=ORIENTED_EDGE ( 'NONE', *, *, #37704, .T. ) ;
#40658=CARTESIAN_POINT ( 'NONE',  ( -24.50093619861336336, -12.48040563361249333, 73.38192204494465898 ) ) ;
#40660=ORIENTED_EDGE ( 'NONE', *, *, #12755, .T. ) ;
#40662=CARTESIAN_POINT ( 'NONE',  ( -20.52631159502315938, -8.474406804437011331, 60.04945086230327433 ) ) ;
#40663=CARTESIAN_POINT ( 'NONE',  ( -21.23484681875272528, -20.74088929683185611, 69.33978048267414351 ) ) ;
#40664=CARTESIAN_POINT ( 'NONE',  ( -21.80513198786261597, -9.285521334292361928, 63.48593961849922351 ) ) ;
#40665=CARTESIAN_POINT ( 'NONE',  ( -12.51133688094842888, -19.86980477907010822, 61.28190024782882972 ) ) ;
#40666=FACE_BOUND ( 'NONE', #23163, .T. ) ;
#40667=EDGE_CURVE ( 'NONE', #21578, #24254, #6174, .T. ) ;
#40668=CARTESIAN_POINT ( 'NONE',  ( -23.89968641036289299, -17.46782332651663339, 66.24357233134217893 ) ) ;
#40671=AXIS2_PLACEMENT_3D ( 'NONE', #42171, #4993, #46825 ) ;
#40673=ORIENTED_EDGE ( 'NONE', *, *, #39353, .F. ) ;
#40674=CARTESIAN_POINT ( 'NONE',  ( -24.12706943888446887, -11.55726411819128785, 63.09184898997396829 ) ) ;
#40676=EDGE_CURVE ( 'NONE', #18426, #44255, #36189, .T. ) ;
#40677=CARTESIAN_POINT ( 'NONE',  ( -24.71152906796918458, -13.26113485863129071, 59.55606250353000775 ) ) ;
#40678=VECTOR ( 'NONE', #28662, 1000.000000000000114 ) ;
#40680=FACE_OUTER_BOUND ( 'NONE', #37671, .T. ) ;
#40681=CARTESIAN_POINT ( 'NONE',  ( -11.84468983566281608, -9.872329927957173012, 64.17914326340513753 ) ) ;
#40682=CARTESIAN_POINT ( 'NONE',  ( -16.51570212919159530, -21.75045681730355795, 65.50947872143868267 ) ) ;
#40684=VERTEX_POINT ( 'NONE', #42881 ) ;
#40686=ADVANCED_FACE ( 'NONE', ( #9147 ), #13539, .T. ) ;
#40687=ORIENTED_EDGE ( 'NONE', *, *, #34330, .T. ) ;
#40690=ADVANCED_FACE ( 'NONE', ( #1992 ), #39367, .T. ) ;
#40691=CARTESIAN_POINT ( 'NONE',  ( -24.61377439452271076, -12.85684087295677891, 66.49585060569550876 ) ) ;
#40692=CARTESIAN_POINT ( 'NONE',  ( -16.16379340615718618, -22.15191857530921382, 58.47080845268740035 ) ) ;
#40696=CARTESIAN_POINT ( 'NONE',  ( -22.09234465700630423, -20.09219189623108548, 62.23439162498055310 ) ) ;
#40697=ORIENTED_EDGE ( 'NONE', *, *, #28705, .T. ) ;
#40698=B_SPLINE_CURVE_WITH_KNOTS ( 'NONE', 3,
 ( #19902, #34908, #46007, #1906, #24328, #34670, #28005, #1175, #31221, #12262 ),
 .UNSPECIFIED., .F., .F.,
 ( 4, 2, 2, 2, 4 ),
 ( 0.1272669073658189987, 0.2522669073463225109, 0.3772669073268261064, 0.5022669073073295909, 0.6272669072878331864 ),
 .UNSPECIFIED. ) ;
#40703=AXIS2_PLACEMENT_3D ( 'NONE', #13914, #39320, #21095 ) ;
#40706=CARTESIAN_POINT ( 'NONE',  ( -17.82542875633258106, -7.370011655844420417, 60.18086518042608901 ) ) ;
#40707=CARTESIAN_POINT ( 'NONE',  ( -11.07356217608303695, -11.86355251018914991, 74.84223526849542907 ) ) ;
#40708=CARTESIAN_POINT ( 'NONE',  ( -23.38313847423633263, -10.33780256150599541, 59.85849373767491954 ) ) ;
#40709=EDGE_CURVE ( 'NONE', #8636, #46413, #44410, .T. ) ;
#40710=ORIENTED_EDGE ( 'NONE', *, *, #35921, .T. ) ;
#40711=CARTESIAN_POINT ( 'NONE',  ( -11.10681587527927938, -11.67891925637714223, 71.10332952723315714 ) ) ;
#40712=CARTESIAN_POINT ( 'NONE',  ( -24.41841346439724347, -17.37497344050957437, 69.45693887357894880 ) ) ;
#40713=AXIS2_PLACEMENT_3D ( 'NONE', #24259, #45935, #12195 ) ;
#40714=CARTESIAN_POINT ( 'NONE',  ( -10.68602809008750576, -16.88409676349039046, 57.70232650191087487 ) ) ;
#40716=VERTEX_POINT ( 'NONE', #40151 ) ;
#40720=CARTESIAN_POINT ( 'NONE',  ( -11.42962537269896117, -10.38539323336976494, 74.62380298385740218 ) ) ;
#40721=B_SPLINE_CURVE_WITH_KNOTS ( 'NONE', 3,
 ( #35639, #20149, #35159, #20402, #12987, #13219, #31957, #35405, #12765, #27779 ),
 .UNSPECIFIED., .F., .F.,
 ( 4, 2, 2, 2, 4 ),
 ( 0.000000000000000000, 0.2500000000000000000, 0.5000000000000000000, 0.7500000000000000000, 1.000000000000000000 ),
 .UNSPECIFIED. ) ;
#40724=CARTESIAN_POINT ( 'NONE',  ( -14.41428275390769365, -7.994163218335415877, 63.97474169571218283 ) ) ;
#40725=EDGE_LOOP ( 'NONE', ( #38716, #18070, #14271, #9956 ) ) ;
#40726=CARTESIAN_POINT ( 'NONE',  ( -11.32138995524401182, -19.08233857334280970, 68.31665992013745381 ) ) ;
#40729=ORIENTED_EDGE ( 'NONE', *, *, #41275, .T. ) ;
#40730=DIRECTION ( 'NONE',  ( -5.731567514496413899E-31, -1.020425574103664789E-16, -1.000000000000000000 ) ) ;
#40731=EDGE_LOOP ( 'NONE', ( #32587, #4852, #43309, #48476, #2562 ) ) ;
#40733=ORIENTED_EDGE ( 'NONE', *, *, #35384, .T. ) ;
#40735=CARTESIAN_POINT ( 'NONE',  ( -14.40713916828295460, -8.490940588968131308, 70.91884656573979839 ) ) ;
#40737=CARTESIAN_POINT ( 'NONE',  ( -10.90759852523040507, -17.49952041063523822, 68.09721944423129969 ) ) ;
#40738=CARTESIAN_POINT ( 'NONE',  ( -21.94242186726961208, -9.397052521110282441, 60.00699132926281010 ) ) ;
#40739=CARTESIAN_POINT ( 'NONE',  ( -12.79487214375358839, -8.971058656907512585, 71.03580700614087107 ) ) ;
#40742=EDGE_LOOP ( 'NONE', ( #19908, #3754, #23763, #26316, #45196 ) ) ;
#40747=AXIS2_PLACEMENT_3D ( 'NONE', #38415, #34480, #1235 ) ;
#40748=CARTESIAN_POINT ( 'NONE',  ( -23.45031237530261947, -11.14340064005916098, 70.10030580274290912 ) ) ;
#40750=ORIENTED_EDGE ( 'NONE', *, *, #47455, .T. ) ;
#40751=CARTESIAN_POINT ( 'NONE',  ( -10.72530867274958410, -17.00760959713300835, 57.97288447305809456 ) ) ;
#40755=CARTESIAN_POINT ( 'NONE',  ( -11.27324709396361335, -11.46480877714557778, 67.69034896821969483 ) ) ;
#40756=ADVANCED_FACE ( 'NONE', ( #10361 ), #3684, .T. ) ;
#40758=CARTESIAN_POINT ( 'NONE',  ( -7.334870405450504727, -11.98365049024292972, 53.49999999999995026 ) ) ;
#40760=ADVANCED_FACE ( 'NONE', ( #21444 ), #14253, .T. ) ;
#40761=CARTESIAN_POINT ( 'NONE',  ( -10.12326218194131044, -13.32541594658350448, 74.86312942357149325 ) ) ;
#40762=EDGE_CURVE ( 'NONE', #25517, #43113, #36427, .T. ) ;
#40764=VERTEX_POINT ( 'NONE', #17954 ) ;
#40765=CARTESIAN_POINT ( 'NONE',  ( -11.12943539273130611, -10.82423919798514689, 57.30928973319082331 ) ) ;
#40766=VECTOR ( 'NONE', #46561, 1000.000000000000000 ) ;
#40767=CARTESIAN_POINT ( 'NONE',  ( -24.42401512115494455, -14.72416081258524834, 62.72913071971822063 ) ) ;
#40769=CARTESIAN_POINT ( 'NONE',  ( -19.44376929052122449, -7.638105555415076076, 60.07597592072836790 ) ) ;
#40771=ORIENTED_EDGE ( 'NONE', *, *, #30139, .F. ) ;
#40773=VECTOR ( 'NONE', #895, 1000.000000000000227 ) ;
#40774=VECTOR ( 'NONE', #2489, 1000.000000000000114 ) ;
#40775=CARTESIAN_POINT ( 'NONE',  ( -12.65090885562174350, -19.92943164506675657, 64.97561006052195864 ) ) ;
#40777=FACE_BOUND ( 'NONE', #7332, .T. ) ;
#40780=CARTESIAN_POINT ( 'NONE',  ( -13.43447785487663637, -11.00382355316531147, 53.88362224778187226 ) ) ;
#40782=CARTESIAN_POINT ( 'NONE',  ( -21.56016804333223646, -8.612711131324969571, 73.64482796973915413 ) ) ;
#40784=CARTESIAN_POINT ( 'NONE',  ( -10.53028993777715883, -16.28642212234895226, 71.73278239416407587 ) ) ;
#40787=( BOUNDED_CURVE ( )  B_SPLINE_CURVE ( 3, ( #40115, #13972, #43573, #9836 ),
 .UNSPECIFIED., .F., .F. ) 
 B_SPLINE_CURVE_WITH_KNOTS ( ( 4, 4 ),
 ( 0.5000000000000000000, 0.9074455897393635118 ),
 .UNSPECIFIED. ) 
 CURVE ( )  GEOMETRIC_REPRESENTATION_ITEM ( )  RATIONAL_B_SPLINE_CURVE ( ( 1.000000000000000888, 0.4567392136813381853, 0.3561768502900318212, 0.6983129098260827394 ) ) 
 REPRESENTATION_ITEM ( '' )  );
#40788=PLANE ( 'NONE',  #43214 ) ;
#40789=ORIENTED_EDGE ( 'NONE', *, *, #12268, .F. ) ;
#40790=CARTESIAN_POINT ( 'NONE',  ( -16.16379449968008331, -22.15191876840708929, 58.47080954035841671 ) ) ;
#40791=CARTESIAN_POINT ( 'NONE',  ( -13.44724237933888134, -20.56996776775315183, 58.34650027598461719 ) ) ;
#40792=EDGE_CURVE ( 'NONE', #27869, #34125, #8887, .T. ) ;
#40795=FACE_OUTER_BOUND ( 'NONE', #14161, .T. ) ;
#40796=CARTESIAN_POINT ( 'NONE',  ( -20.67761229128902656, -8.545853924536821467, 66.92536870251414882 ) ) ;
#40797=CARTESIAN_POINT ( 'NONE',  ( -20.82184643845504723, -8.178298495136663959, 63.49776821231386492 ) ) ;
#40798=CARTESIAN_POINT ( 'NONE',  ( -21.25156111013253835, -21.20098409628925396, 65.70641164036103987 ) ) ;
#40799=CARTESIAN_POINT ( 'NONE',  ( -14.16498672988215191, -8.109065889264286398, 70.91612917212019340 ) ) ;
#40800=CARTESIAN_POINT ( 'NONE',  ( -14.73375560093340120, -21.75656996136207866, 61.75105004614717785 ) ) ;
#40801=( BOUNDED_SURFACE ( )  B_SPLINE_SURFACE ( 3, 1, ( 
 ( #9456, #6241 ),
 ( #17776, #21732 ),
 ( #28646, #35772 ),
 ( #24481, #25432 ),
 ( #39486, #28879 ),
 ( #47115, #18016 ),
 ( #36259, #17301 ) ),
 .UNSPECIFIED., .T., .F., .F. ) 
 B_SPLINE_SURFACE_WITH_KNOTS ( ( 4, 3, 4 ),
 ( 2, 2 ),
 ( 0.000000000000000000, 0.5000000000000000000, 1.000000000000000000 ),
 ( 0.000000000000000000, 1.000000000000000000 ),
 .UNSPECIFIED. ) 
 GEOMETRIC_REPRESENTATION_ITEM ( )  RATIONAL_B_SPLINE_SURFACE ( (
 ( 1.000000000000000000, 1.000000000000000000),
 ( 0.3333333333333335369, 0.3333333333333330373),
 ( 0.3333333333333335369, 0.3333333333333330373),
 ( 1.000000000000000000, 1.000000000000000000),
 ( 0.3333333333333333703, 0.3333333333333333703),
 ( 0.3333333333333333703, 0.3333333333333333703),
 ( 1.000000000000000000, 1.000000000000000000) ) ) 
 REPRESENTATION_ITEM ( '' )  SURFACE ( )  );
#40802=ORIENTED_EDGE ( 'NONE', *, *, #24628, .T. ) ;
#40803=VERTEX_POINT ( 'NONE', #33451 ) ;
#40807=PLANE ( 'NONE',  #37791 ) ;
#40810=AXIS2_PLACEMENT_3D ( 'NONE', #36910, #48244, #48488 ) ;
#40814=CIRCLE ( 'NONE', #14846, 6.899999999999997691 ) ;
#40816=CARTESIAN_POINT ( 'NONE',  ( -22.00056318799662591, -20.10656996550254050, 62.25055788910309218 ) ) ;
#40817=CARTESIAN_POINT ( 'NONE',  ( -12.27604185553471616, -19.62628656662749549, 58.21210303282668264 ) ) ;
#40820=B_SPLINE_CURVE_WITH_KNOTS ( 'NONE', 3,
 ( #31353, #23746, #16563, #11924, #20277, #41958, #15838, #39226, #8463, #1303 ),
 .UNSPECIFIED., .F., .F.,
 ( 4, 2, 2, 2, 4 ),
 ( 0.000000000000000000, 0.2500000000000000000, 0.5000000000000000000, 0.7500000000000000000, 1.000000000000000000 ),
 .UNSPECIFIED. ) ;
#40823=CARTESIAN_POINT ( 'NONE',  ( -21.54616816135207813, -9.151524939380248469, 66.88823273622162446 ) ) ;
#40826=CARTESIAN_POINT ( 'NONE',  ( -15.24014793263337531, -21.45986350121160058, 65.33270079998744961 ) ) ;
#40830=VERTEX_POINT ( 'NONE', #44827 ) ;
#40832=EDGE_CURVE ( 'NONE', #4358, #35167, #11080, .T. ) ;
#40833=EDGE_CURVE ( 'NONE', #18877, #31039, #42048, .T. ) ;
#40835=ORIENTED_EDGE ( 'NONE', *, *, #6694, .T. ) ;
#40836=CARTESIAN_POINT ( 'NONE',  ( -12.84691039585993444, -8.931012183600500975, 67.56438067310742213 ) ) ;
#40837=EDGE_CURVE ( 'NONE', #2827, #15007, #14985, .T. ) ;
#40838=CARTESIAN_POINT ( 'NONE',  ( -16.50454536406711981, -22.20232556258728351, 65.34068991928313608 ) ) ;
#40839=VECTOR ( 'NONE', #26817, 1000.000000000000227 ) ;
#40841=CARTESIAN_POINT ( 'NONE',  ( -13.71339110807025641, -20.80363600241853561, 65.13628881288371986 ) ) ;
#40842=EDGE_CURVE ( 'NONE', #26529, #35577, #47559, .T. ) ;
#40843=CARTESIAN_POINT ( 'NONE',  ( -19.67760665824181388, -21.48965406232008490, 65.75014118398131302 ) ) ;
#40845=ORIENTED_EDGE ( 'NONE', *, *, #36924, .T. ) ;
#40848=VECTOR ( 'NONE', #28400, 1000.000000000000000 ) ;
#40849=CARTESIAN_POINT ( 'NONE',  ( -11.38016085489450901, -11.27755116225183230, 60.67885732596114678 ) ) ;
#40850=EDGE_CURVE ( 'NONE', #33575, #45950, #13845, .T. ) ;
#40851=ORIENTED_EDGE ( 'NONE', *, *, #11581, .F. ) ;
#40853=CARTESIAN_POINT ( 'NONE',  ( -12.96596534320165794, -9.347742485070138940, 70.84925352874383009 ) ) ;
#40854=CARTESIAN_POINT ( 'NONE',  ( -24.66733291767277692, -16.55538881886969804, 59.30987817879385915 ) ) ;
#40858=CARTESIAN_POINT ( 'NONE',  ( -23.25757715627672795, -10.17517474196413474, 63.18690702823881367 ) ) ;
#40859=CARTESIAN_POINT ( 'NONE',  ( -16.78865592400587659, -21.78030535593112305, 68.99560651886281448 ) ) ;
#40860=CARTESIAN_POINT ( 'NONE',  ( -23.93648101794248362, -17.51022725521227841, 65.95829288617392194 ) ) ;
#40862=ORIENTED_EDGE ( 'NONE', *, *, #23553, .T. ) ;
#40863=CARTESIAN_POINT ( 'NONE',  ( -24.31482381427648676, -13.31912605980313735, 59.36267924676594987 ) ) ;
#40865=DIRECTION ( 'NONE',  ( -1.148482744091818979E-06, 2.957121237693701878E-08, 0.9999999999993399724 ) ) ;
#40867=VERTEX_POINT ( 'NONE', #30052 ) ;
#40870=CARTESIAN_POINT ( 'NONE',  ( -24.85884029783971982, -14.32113974155904046, 66.29637463883811677 ) ) ;
#40871=AXIS2_PLACEMENT_3D ( 'NONE', #1049, #565, #4028 ) ;
#40872=CARTESIAN_POINT ( 'NONE',  ( -15.37142651463144460, -21.97085505939421779, 72.14551830437926583 ) ) ;
#40873=CARTESIAN_POINT ( 'NONE',  ( -11.65600162890749303, -18.86286912916044400, 68.51689600618566089 ) ) ;
#40875=VERTEX_POINT ( 'NONE', #256 ) ;
#40877=CARTESIAN_POINT ( 'NONE',  ( -23.54032652647746104, -11.40454826030700808, 66.61317707917329756 ) ) ;
#40878=CARTESIAN_POINT ( 'NONE',  ( -10.39215594834096024, -14.30487625923878880, 64.53803863383089379 ) ) ;
#40879=EDGE_CURVE ( 'NONE', #46319, #34661, #43803, .T. ) ;
#40880=ORIENTED_EDGE ( 'NONE', *, *, #5131, .F. ) ;
#40882=VECTOR ( 'NONE', #24093, 1000.000000000000227 ) ;
#40884=CARTESIAN_POINT ( 'NONE',  ( -24.38756562526642213, -15.91227465074932290, 66.34852784166324113 ) ) ;
#40886=CARTESIAN_POINT ( 'NONE',  ( -13.51659408464697698, -24.65568926594394128, 53.49999999999995026 ) ) ;
#40887=ORIENTED_EDGE ( 'NONE', *, *, #13012, .T. ) ;
#40888=CARTESIAN_POINT ( 'NONE',  ( -24.38143503755601316, -15.58083059521001168, 73.30303748419844112 ) ) ;
#40889=CARTESIAN_POINT ( 'NONE',  ( -15.38020936669038008, -6.822612233742264110, 53.49999999999995026 ) ) ;
#40891=CARTESIAN_POINT ( 'NONE',  ( -21.43532435649834866, -21.08734459619973123, 69.19303634238183065 ) ) ;
#40892=CARTESIAN_POINT ( 'NONE',  ( -10.64854695470030599, -12.86019059820356958, 64.55364013863997741 ) ) ;
#40893=EDGE_CURVE ( 'NONE', #33146, #14550, #39066, .T. ) ;
#40896=EDGE_CURVE ( 'NONE', #9377, #6262, #40634, .T. ) ;
#40899=DIRECTION ( 'NONE',  ( 0.3124635249310678264, 0.8422251632096483531, 0.4393441931380604459 ) ) ;
#40900=ORIENTED_EDGE ( 'NONE', *, *, #7163, .T. ) ;
#40905=ORIENTED_EDGE ( 'NONE', *, *, #17608, .F. ) ;
#40906=EDGE_LOOP ( 'NONE', ( #42508, #39395 ) ) ;
#40908=CARTESIAN_POINT ( 'NONE',  ( -11.14144638094932382, -18.81445342923831987, 61.39055447797494480 ) ) ;
#40909=CARTESIAN_POINT ( 'NONE',  ( -10.52215087187021325, -13.37195826583270986, 74.67817647370830514 ) ) ;
#40911=CARTESIAN_POINT ( 'NONE',  ( -24.02655244371635845, -11.35792869308308717, 66.53719207489109522 ) ) ;
#40916=CARTESIAN_POINT ( 'NONE',  ( -14.78766009005058812, -21.34800739930362568, 58.45145834864037937 ) ) ;
#40918=CARTESIAN_POINT ( 'NONE',  ( -24.72725712452650981, -16.28144042551206638, 62.84974626185121593 ) ) ;
#40921=LINE ( 'NONE', #3488, #33408 ) ;
#40922=PRODUCT_DEFINITION_SHAPE ( 'NONE', 'NONE',  #18332 ) ;
#40923=CARTESIAN_POINT ( 'NONE',  ( -16.42344266294433908, -21.79157980633116054, 58.28585275688816836 ) ) ;
#40924=ORIENTED_EDGE ( 'NONE', *, *, #28908, .F. ) ;
#40925=CARTESIAN_POINT ( 'NONE',  ( -14.04638888798549701, -8.616795679365674587, 70.72957572181515218 ) ) ;
#40926=CARTESIAN_POINT ( 'NONE',  ( -10.23569597183452728, -12.85201410577908732, 67.99478283741052564 ) ) ;
#40928=CARTESIAN_POINT ( 'NONE',  ( -24.71334378318632830, -13.26952680650525274, 59.47772536435775947 ) ) ;
#40929=CARTESIAN_POINT ( 'NONE',  ( -24.27425269666204244, -13.36807298356958817, 59.66267976136047935 ) ) ;
#40931=( BOUNDED_CURVE ( )  B_SPLINE_CURVE ( 3, ( #24856, #39627, #44308, #32252 ),
 .UNSPECIFIED., .F., .F. ) 
 B_SPLINE_CURVE_WITH_KNOTS ( ( 4, 4 ),
 ( 0.5000000000000000000, 0.9074455897393751691 ),
 .UNSPECIFIED. ) 
 CURVE ( )  GEOMETRIC_REPRESENTATION_ITEM ( )  RATIONAL_B_SPLINE_CURVE ( ( 0.9999999999999952260, 0.4567392136813065440, 0.3561768502900240496, 0.6983129098261426915 ) ) 
 REPRESENTATION_ITEM ( '' )  );
#40932=CARTESIAN_POINT ( 'NONE',  ( -11.51143670280680986, -18.65567654335754355, 68.51689928321519574 ) ) ;
#40933=CARTESIAN_POINT ( 'NONE',  ( -23.82366728017863622, -10.99486018697619372, 73.47698013610775547 ) ) ;
#40934=ORIENTED_EDGE ( 'NONE', *, *, #16565, .F. ) ;
#40935=EDGE_LOOP ( 'NONE', ( #42565, #30995, #24005, #8154 ) ) ;
#40938=CYLINDRICAL_SURFACE ( 'NONE', #13841, 0.1500000000000045186 ) ;
#40940=CARTESIAN_POINT ( 'NONE',  ( -18.90223155190902915, -7.506551502853892721, 67.01416387246997886 ) ) ;
#40942=( BOUNDED_CURVE ( )  B_SPLINE_CURVE ( 3, ( #14165, #10742, #40780, #40532 ),
 .UNSPECIFIED., .F., .F. ) 
 B_SPLINE_CURVE_WITH_KNOTS ( ( 4, 4 ),
 ( 4.712388980384689674, 4.921828490624010399 ),
 .UNSPECIFIED. ) 
 CURVE ( )  GEOMETRIC_REPRESENTATION_ITEM ( )  RATIONAL_B_SPLINE_CURVE ( ( 1.000000000000000000, 0.9963479302455154896, 0.9963479302455154896, 1.000000000000000000 ) ) 
 REPRESENTATION_ITEM ( '' )  );
#40944=CARTESIAN_POINT ( 'NONE',  ( -24.60930328113607501, -12.84061010741178066, 66.50257946727398917 ) ) ;
#40945=CARTESIAN_POINT ( 'NONE',  ( -15.62101046192594289, -7.580605815997546237, 70.72494447658496597 ) ) ;
#40947=VECTOR ( 'NONE', #13515, 999.9999999999998863 ) ;
#40950=EDGE_LOOP ( 'NONE', ( #41865, #45313, #46658, #40924, #32248 ) ) ;
#40951=CARTESIAN_POINT ( 'NONE',  ( -10.37462440636232053, -14.89569459299594634, 75.09778901493891112 ) ) ;
#40952=AXIS2_PLACEMENT_3D ( 'NONE', #16156, #30968, #46474 ) ;
#40953=DIRECTION ( 'NONE',  ( -6.471065199890530885E-06, -1.909039593073236381E-06, 0.9999999999772404280 ) ) ;
#40954=( BOUNDED_CURVE ( )  B_SPLINE_CURVE ( 3, ( #23725, #39198, #12135, #27639 ),
 .UNSPECIFIED., .F., .F. ) 
 B_SPLINE_CURVE_WITH_KNOTS ( ( 4, 4 ),
 ( 0.000000000000000000, 0.4074455897393634562 ),
 .UNSPECIFIED. ) 
 CURVE ( )  GEOMETRIC_REPRESENTATION_ITEM ( )  RATIONAL_B_SPLINE_CURVE ( ( 1.000000000000000000, 0.4567392136813290815, 0.3561768502900292122, 0.6983129098261003920 ) ) 
 REPRESENTATION_ITEM ( '' )  );
#40955=EDGE_LOOP ( 'NONE', ( #37035, #38983, #22197, #22128, #34140 ) ) ;
#40957=CARTESIAN_POINT ( 'NONE',  ( -14.98927377128267047, -8.246306944878837086, 57.14999999999994884 ) ) ;
#40959=ORIENTED_EDGE ( 'NONE', *, *, #47650, .T. ) ;
#40960=CARTESIAN_POINT ( 'NONE',  ( -11.97137584462052828, -19.88590378904827460, 58.06535876572594645 ) ) ;
#40961=EDGE_CURVE ( 'NONE', #31485, #10695, #44127, .T. ) ;
#40962=CARTESIAN_POINT ( 'NONE',  ( -15.65237751681051570, -7.981625683898254664, 67.14006984041519388 ) ) ;
#40966=CARTESIAN_POINT ( 'NONE',  ( -10.55090139406780558, -17.68373120125836806, 68.14076041135473361 ) ) ;
#40967=EDGE_LOOP ( 'NONE', ( #25216, #33905, #47758, #9794, #2432 ) ) ;
#40968=CARTESIAN_POINT ( 'NONE',  ( -10.58771178721467798, -11.84651422905517926, 74.67185031923813199 ) ) ;
#40970=CARTESIAN_POINT ( 'NONE',  ( -19.49109506855409180, -21.54969648977046148, 62.28031529404344013 ) ) ;
#40972=ADVANCED_FACE ( 'NONE', ( #23635 ), #18689, .T. ) ;
#40975=ORIENTED_EDGE ( 'NONE', *, *, #27377, .F. ) ;
#40976=CARTESIAN_POINT ( 'NONE',  ( -17.72612443559818018, -7.765381109175947927, 60.36588690973874094 ) ) ;
#40979=CARTESIAN_POINT ( 'NONE',  ( -18.52415950777489684, -7.896185818571675341, 74.14064402152244782 ) ) ;
#40980=EDGE_CURVE ( 'NONE', #22485, #44170, #23827, .T. ) ;
#40981=CARTESIAN_POINT ( 'NONE',  ( -22.60138646627221348, -10.09559420857893741, 73.67088087145607744 ) ) ;
#40982=CARTESIAN_POINT ( 'NONE',  ( -11.72709874728437107, -10.00842693884592549, 67.69235173591077626 ) ) ;
#40984=CYLINDRICAL_SURFACE ( 'NONE', #37280, 0.1500000000000029088 ) ;
#40986=CARTESIAN_POINT ( 'NONE',  ( -14.61429364226973782, -21.70915942589378744, 58.28805155203381361 ) ) ;
#40987=ORIENTED_EDGE ( 'NONE', *, *, #30655, .T. ) ;
#40988=VERTEX_POINT ( 'NONE', #35172 ) ;
#40994=ADVANCED_FACE ( 'NONE', ( #13234 ), #20163, .T. ) ;
#40998=ORIENTED_EDGE ( 'NONE', *, *, #24031, .T. ) ;
#40999=ORIENTED_EDGE ( 'NONE', *, *, #15531, .T. ) ;
#41001=CARTESIAN_POINT ( 'NONE',  ( -11.48094281790512738, -10.31654952874404962, 74.57851759402076652 ) ) ;
#41003=CARTESIAN_POINT ( 'NONE',  ( -16.06050865347321732, -9.480920197610746669, 54.07175714974878389 ) ) ;
#41006=ORIENTED_EDGE ( 'NONE', *, *, #38145, .T. ) ;
#41008=AXIS2_PLACEMENT_3D ( 'NONE', #15141, #33122, #22307 ) ;
#41009=CARTESIAN_POINT ( 'NONE',  ( -10.48067351556794158, -16.03044098841782628, 68.27767830705533925 ) ) ;
#41010=FACE_OUTER_BOUND ( 'NONE', #35985, .T. ) ;
#41011=ORIENTED_EDGE ( 'NONE', *, *, #26194, .T. ) ;
#41012=CARTESIAN_POINT ( 'NONE',  ( -9.939267784769082681, -14.33236412611010913, 53.49999999999994316 ) ) ;
#41014=CARTESIAN_POINT ( 'NONE',  ( -12.95699726224880699, -8.846094125884357950, 64.02291131566488502 ) ) ;
#41015=CARTESIAN_POINT ( 'NONE',  ( -19.52605192831022407, -21.48662393483848376, 65.74869660756507983 ) ) ;
#41017=CARTESIAN_POINT ( 'NONE',  ( -9.990077291455589759, -14.31953385297554071, 64.56520754649302773 ) ) ;
#41019=VERTEX_POINT ( 'NONE', #24835 ) ;
#41020=CARTESIAN_POINT ( 'NONE',  ( -17.91610874870965020, -22.24302035646641684, 62.13181838639658139 ) ) ;
#41022=PLANE ( 'NONE',  #16388 ) ;
#41023=DIRECTION ( 'NONE',  ( 0.9862050927915949616, 0.1655279884246635413, 7.765682856207886445E-08 ) ) ;
#41025=CARTESIAN_POINT ( 'NONE',  ( -22.99015471925471843, -19.14192088663603997, 62.44587121756105574 ) ) ;
#41026=CARTESIAN_POINT ( 'NONE',  ( -24.69822963474414479, -13.19963333263893190, 59.54763306486673713 ) ) ;
#41027=LINE ( 'NONE', #7310, #43555 ) ;
#41030=EDGE_CURVE ( 'NONE', #2787, #15048, #48487, .T. ) ;
#41031=ORIENTED_EDGE ( 'NONE', *, *, #31433, .F. ) ;
#41032=CYLINDRICAL_SURFACE ( 'NONE', #46279, 0.1499999999999987454 ) ;
#41033=CARTESIAN_POINT ( 'NONE',  ( -13.70219457171530841, -20.73773636609404036, 61.70749392003438061 ) ) ;
#41034=CARTESIAN_POINT ( 'NONE',  ( -24.41779626044834828, -14.51093891981887651, 62.78584623703071799 ) ) ;
#41035=EDGE_CURVE ( 'NONE', #18330, #38687, #19107, .T. ) ;
#41037=ORIENTED_EDGE ( 'NONE', *, *, #35816, .T. ) ;
#41038=CARTESIAN_POINT ( 'NONE',  ( -10.13226805943771858, -16.33660356775173739, 71.49104427242312454 ) ) ;
#41039=VECTOR ( 'NONE', #10194, 1000.000000000000227 ) ;
#41040=ORIENTED_EDGE ( 'NONE', *, *, #47434, .T. ) ;
#41041=FACE_OUTER_BOUND ( 'NONE', #33836, .T. ) ;
#41043=CARTESIAN_POINT ( 'NONE',  ( -24.34138250757122535, -16.17068267630804002, 62.89328676667767581 ) ) ;
#41045=CARTESIAN_POINT ( 'NONE',  ( -21.53861886228549949, -21.02004079589906027, 72.63951149839988375 ) ) ;
#41046=CARTESIAN_POINT ( 'NONE',  ( -23.05807922735651161, -10.57113180461529822, 59.60203456339924344 ) ) ;
#41047=ORIENTED_EDGE ( 'NONE', *, *, #25562, .T. ) ;
#41049=DIRECTION ( 'NONE',  ( 0.9562635972186041000, -0.2925062950340273638, 4.666065131241568958E-08 ) ) ;
#41050=CARTESIAN_POINT ( 'NONE',  ( -22.28902059852239503, -19.84295448483234736, 69.45801383501738258 ) ) ;
#41051=CARTESIAN_POINT ( 'NONE',  ( -19.38982564003701725, -21.99536589193390412, 58.66360838363829799 ) ) ;
#41052=CARTESIAN_POINT ( 'NONE',  ( -10.03904597514415009, -13.82694077737217242, 57.56329639008353638 ) ) ;
#41054=CARTESIAN_POINT ( 'NONE',  ( -14.13370316840849483, -8.630624890407778693, 74.19954649408759906 ) ) ;
#41055=EDGE_CURVE ( 'NONE', #14468, #20890, #7964, .T. ) ;
#41056=VERTEX_POINT ( 'NONE', #5396 ) ;
#41058=CARTESIAN_POINT ( 'NONE',  ( -17.38762135442090795, -7.756298984960698917, 63.43568405917763897 ) ) ;
#41061=EDGE_CURVE ( 'NONE', #28368, #26240, #46528, .T. ) ;
#41062=AXIS2_PLACEMENT_3D ( 'NONE', #11935, #34077, #7019 ) ;
#41064=CARTESIAN_POINT ( 'NONE',  ( -11.57789998141014820, -10.19135890511387110, 71.11893103769725144 ) ) ;
#41066=ORIENTED_EDGE ( 'NONE', *, *, #20153, .F. ) ;
#41068=ORIENTED_EDGE ( 'NONE', *, *, #2858, .F. ) ;
#41070=LINE ( 'NONE', #11278, #35534 ) ;
#41071=CARTESIAN_POINT ( 'NONE',  ( -10.38863864971416184, -14.24588297309210816, 57.60391932725825370 ) ) ;
#41072=EDGE_LOOP ( 'NONE', ( #20498, #31007, #26941, #27871, #33539 ) ) ;
#41074=CARTESIAN_POINT ( 'NONE',  ( -10.53028993777715883, -16.28642212234895226, 71.73278239416407587 ) ) ;
#41075=CARTESIAN_POINT ( 'NONE',  ( -21.53594150109643834, -20.54048459808615235, 72.52446133926662242 ) ) ;
#41076=ADVANCED_FACE ( 'NONE', ( #12530 ), #400, .T. ) ;
#41077=ORIENTED_EDGE ( 'NONE', *, *, #16820, .F. ) ;
#41078=DIRECTION ( 'NONE',  ( -0.9999247414263408018, 0.01226831216845469807, 5.367905339378915168E-08 ) ) ;
#41079=( BOUNDED_CURVE ( )  B_SPLINE_CURVE ( 3, ( #19526, #31336, #34534, #15324 ),
 .UNSPECIFIED., .F., .F. ) 
 B_SPLINE_CURVE_WITH_KNOTS ( ( 4, 4 ),
 ( 0.9074455897393685078, 1.000000000000000000 ),
 .UNSPECIFIED. ) 
 CURVE ( )  GEOMETRIC_REPRESENTATION_ITEM ( )  RATIONAL_B_SPLINE_CURVE ( ( 0.6983129098261100509, 0.7760317562607128572, 0.8765941196520095069, 1.000000000000000000 ) ) 
 REPRESENTATION_ITEM ( '' )  );
#41082=CARTESIAN_POINT ( 'NONE',  ( -10.51956558245075080, -15.96174594004655312, 64.73444859219196701 ) ) ;
#41084=PLANE ( 'NONE',  #610 ) ;
#41085=CARTESIAN_POINT ( 'NONE',  ( -24.31057894323393143, -16.31947677049899781, 59.41772612388854924 ) ) ;
#41086=VERTEX_POINT ( 'NONE', #46274 ) ;
#41087=FACE_OUTER_BOUND ( 'NONE', #5149, .T. ) ;
#41088=CARTESIAN_POINT ( 'NONE',  ( -18.97054302448013985, -7.521389842619064403, 67.08567168106696954 ) ) ;
#41089=ORIENTED_EDGE ( 'NONE', *, *, #47053, .T. ) ;
#41091=DIRECTION ( 'NONE',  ( 0.09855345062332551698, 0.9951317587989213509, 3.188559572831062401E-08 ) ) ;
#41092=CARTESIAN_POINT ( 'NONE',  ( -21.62985240417965827, -8.659687547922406026, 73.76275303717041254 ) ) ;
#41093=ORIENTED_EDGE ( 'NONE', *, *, #19086, .F. ) ;
#41095=( BOUNDED_CURVE ( )  B_SPLINE_CURVE ( 3, ( #38131, #15229, #45797, #38366 ),
 .UNSPECIFIED., .F., .F. ) 
 B_SPLINE_CURVE_WITH_KNOTS ( ( 4, 4 ),
 ( 0.9074455897393632897, 1.000000000000000000 ),
 .UNSPECIFIED. ) 
 CURVE ( )  GEOMETRIC_REPRESENTATION_ITEM ( )  RATIONAL_B_SPLINE_CURVE ( ( 0.6983129098260925094, 0.7760317562606977582, 0.8765941196520002920, 1.000000000000000000 ) ) 
 REPRESENTATION_ITEM ( '' )  );
#41096=CARTESIAN_POINT ( 'NONE',  ( -10.44202778021669609, -14.30845378979165794, 64.68803863533310050 ) ) ;
#41097=CARTESIAN_POINT ( 'NONE',  ( -10.08672033063305840, -16.09972936581058889, 68.12767827759553541 ) ) ;
#41098=VERTEX_POINT ( 'NONE', #32691 ) ;
#41102=B_SPLINE_CURVE_WITH_KNOTS ( 'NONE', 3,
 ( #39908, #9651, #29065, #24422, #6427, #20718, #6659, #44113, #10117, #25379 ),
 .UNSPECIFIED., .F., .F.,
 ( 4, 2, 2, 2, 4 ),
 ( 0.000000000000000000, 0.2500000000000000000, 0.5000000000000000000, 0.7500000000000000000, 1.000000000000000000 ),
 .UNSPECIFIED. ) ;
#41104=ORIENTED_EDGE ( 'NONE', *, *, #37328, .F. ) ;
#41106=CARTESIAN_POINT ( 'NONE',  ( -24.42668993457695592, -13.99045928592870958, 73.40799407547365263 ) ) ;
#41108=CARTESIAN_POINT ( 'NONE',  ( -24.31883679440356261, -17.63164986302842152, 66.20003142906764992 ) ) ;
#41109=CARTESIAN_POINT ( 'NONE',  ( -17.17596094306194487, -7.763534178167762256, 70.79035842408370627 ) ) ;
#41111=CARTESIAN_POINT ( 'NONE',  ( -14.65765131015531253, -21.78034674156931061, 54.27966884056655061 ) ) ;
#41114=B_SPLINE_CURVE_WITH_KNOTS ( 'NONE', 3,
 ( #29398, #22494, #2802, #30143, #29155, #37008, #3529, #48342, #40472, #37491 ),
 .UNSPECIFIED., .F., .F.,
 ( 4, 2, 2, 2, 4 ),
 ( 0.000000000000000000, 0.2500000000000000000, 0.5000000000000000000, 0.7500000000000000000, 1.000000000000000000 ),
 .UNSPECIFIED. ) ;
#41115=CARTESIAN_POINT ( 'NONE',  ( -14.60689809042302834, -8.346551666329650843, 64.08978840692947188 ) ) ;
#41116=CARTESIAN_POINT ( 'NONE',  ( -13.49987391503245426, -9.012479888650673843, 60.43950329012445621 ) ) ;
#41117=B_SPLINE_CURVE_WITH_KNOTS ( 'NONE', 1,
 ( #4692, #19716 ),
 .UNSPECIFIED., .F., .F.,
 ( 2, 2 ),
 ( 0.000000000000000000, 1.000000000000000000 ),
 .UNSPECIFIED. ) ;
#41119=EDGE_CURVE ( 'NONE', #6698, #32393, #6359, .T. ) ;
#41120=EDGE_CURVE ( 'NONE', #22754, #16663, #37306, .T. ) ;
#41121=ORIENTED_EDGE ( 'NONE', *, *, #19302, .T. ) ;
#41122=CARTESIAN_POINT ( 'NONE',  ( -12.36794914932409561, -19.72224030764921565, 61.39678633597973345 ) ) ;
#41123=CARTESIAN_POINT ( 'NONE',  ( -10.64449958474462932, -13.06134669730016995, 71.43658536801360981 ) ) ;
#41124=CARTESIAN_POINT ( 'NONE',  ( -11.68224399338930297, -10.06205091296609488, 67.62084114930100043 ) ) ;
#41125=CYLINDRICAL_SURFACE ( 'NONE', #38240, 0.1500000000000035194 ) ;
#41126=EDGE_LOOP ( 'NONE', ( #40562, #13413, #40862, #9001, #19119 ) ) ;
#41127=CARTESIAN_POINT ( 'NONE',  ( -23.61204160381034711, -11.53669949605622769, 66.42214514747726639 ) ) ;
#41128=CARTESIAN_POINT ( 'NONE',  ( -14.28769015366465567, -8.051497000463099241, 67.51620991724109899 ) ) ;
#41129=EDGE_CURVE ( 'NONE', #10747, #32823, #685, .T. ) ;
#41130=VERTEX_POINT ( 'NONE', #39844 ) ;
#41131=CARTESIAN_POINT ( 'NONE',  ( -22.24652905638778577, -19.95594847178128362, 62.11950460074248781 ) ) ;
#41132=CARTESIAN_POINT ( 'NONE',  ( -11.25989433568915032, -11.38792842781904469, 64.44882039367774951 ) ) ;
#41133=CARTESIAN_POINT ( 'NONE',  ( -24.78881009142557090, -15.93819564886128148, 66.17669525438618905 ) ) ;
#41135=CARTESIAN_POINT ( 'NONE',  ( -17.43688372600657743, -7.809108077429288919, 67.02039585984587688 ) ) ;
#41136=EDGE_LOOP ( 'NONE', ( #39912, #16225 ) ) ;
#41137=CARTESIAN_POINT ( 'NONE',  ( -22.78262153964987036, -19.98509753430224833, 72.90046450679021461 ) ) ;
#41138=CARTESIAN_POINT ( 'NONE',  ( -19.47283698296378418, -21.55511232968401814, 62.28943840551588806 ) ) ;
#41139=ORIENTED_EDGE ( 'NONE', *, *, #27239, .F. ) ;
#41140=CARTESIAN_POINT ( 'NONE',  ( -16.58751391467172098, -21.80939466075598077, 65.52564390317479592 ) ) ;
#41141=CARTESIAN_POINT ( 'NONE',  ( -9.908656216309283948, -19.57032361137281384, 53.49999999999995026 ) ) ;
#41144=CARTESIAN_POINT ( 'NONE',  ( -21.35639191854221508, -21.13703508191276015, 69.17733319344661425 ) ) ;
#41147=PLANE ( 'NONE',  #47876 ) ;
#41148=ORIENTED_EDGE ( 'NONE', *, *, #2044, .F. ) ;
#41149=CARTESIAN_POINT ( 'NONE',  ( -12.18719842096713357, -10.08886484896570934, 64.04386393395434141 ) ) ;
#41150=CARTESIAN_POINT ( 'NONE',  ( -11.39127492490111315, -11.16067319722467843, 60.69357916181100876 ) ) ;
#41153=LINE ( 'NONE', #7683, #21176 ) ;
#41154=LINE ( 'NONE', #48532, #42100 ) ;
#41156=ORIENTED_EDGE ( 'NONE', *, *, #31692, .T. ) ;
#41157=CARTESIAN_POINT ( 'NONE',  ( -11.14611441067771658, -11.60115924236117024, 67.91304812855648265 ) ) ;
#41158=CARTESIAN_POINT ( 'NONE',  ( -20.19053640067075506, -7.838066347919499854, 54.27966884056654351 ) ) ;
#41159=EDGE_LOOP ( 'NONE', ( #47887, #4176, #28791, #46469, #33945 ) ) ;
#41160=CARTESIAN_POINT ( 'NONE',  ( -15.33667684601822856, -7.657446057057493150, 74.21839124043556524 ) ) ;
#41161=CARTESIAN_POINT ( 'NONE',  ( -24.09792889798371007, -17.08130376423426000, 73.18336032035891492 ) ) ;
#41162=CARTESIAN_POINT ( 'NONE',  ( -13.43921408130402995, -8.993432070331126127, 60.73950277491898930 ) ) ;
#41163=CARTESIAN_POINT ( 'NONE',  ( -11.61693612796584141, -18.71788356627799388, 64.76209452048259152 ) ) ;
#41164=CARTESIAN_POINT ( 'NONE',  ( -24.74352993119518374, -16.19876237476239922, 62.75361995816021476 ) ) ;
#41165=FACE_BOUND ( 'NONE', #12609, .T. ) ;
#41166=CARTESIAN_POINT ( 'NONE',  ( -19.59076105604923868, -21.93735943072320538, 62.15536986693265931 ) ) ;
#41167=CARTESIAN_POINT ( 'NONE',  ( -13.62948724496060215, -8.926948417807865965, 57.26967755883410405 ) ) ;
#41168=CARTESIAN_POINT ( 'NONE',  ( -16.65537282897929927, -21.76815620359785797, 68.76730947549657458 ) ) ;
#41169=LINE ( 'NONE', #5813, #30477 ) ;
#41171=ORIENTED_EDGE ( 'NONE', *, *, #9221, .T. ) ;
#41172=CARTESIAN_POINT ( 'NONE',  ( -24.12071557656922494, -11.54438865435207795, 63.06722852297808402 ) ) ;
#41173=CARTESIAN_POINT ( 'NONE',  ( -9.990623027812100432, -14.31192454061599229, 64.57299275950818185 ) ) ;
#41174=CARTESIAN_POINT ( 'NONE',  ( -12.10000935918735010, -20.02047918228639034, 61.50340342271149296 ) ) ;
#41178=CARTESIAN_POINT ( 'NONE',  ( -11.81178692268928643, -10.62566621335946770, 74.43885052268630886 ) ) ;
#41181=ORIENTED_EDGE ( 'NONE', *, *, #39002, .F. ) ;
#41183=EDGE_CURVE ( 'NONE', #47012, #25059, #33730, .T. ) ;
#41185=DIRECTION ( 'NONE',  ( -6.258914682829359833E-07, 5.777405174637831559E-07, 0.9999999999996371791 ) ) ;
#41186=AXIS2_PLACEMENT_3D ( 'NONE', #8384, #19713, #7422 ) ;
#41188=CARTESIAN_POINT ( 'NONE',  ( -18.97054410961560578, -7.521390078327941708, 67.08567059339527816 ) ) ;
#41189=EDGE_CURVE ( 'NONE', #5480, #9880, #3221, .T. ) ;
#41191=CARTESIAN_POINT ( 'NONE',  ( -10.37541943412130863, -14.96049300415475436, 75.08306784598362071 ) ) ;
#41196=CARTESIAN_POINT ( 'NONE',  ( -13.86230672564574284, -20.89334503125211029, 68.45625163552200831 ) ) ;
#41198=CARTESIAN_POINT ( 'NONE',  ( -23.92719435707370224, -11.17417392741853988, 70.00715344888816105 ) ) ;
#41199=CARTESIAN_POINT ( 'NONE',  ( -11.10300331676175567, -11.79817459733614093, 74.74767048167663575 ) ) ;
#41200=CARTESIAN_POINT ( 'NONE',  ( -22.80623672001925328, -19.96042370788389064, 72.79400547454775960 ) ) ;
#41203=PLANE ( 'NONE',  #34413 ) ;
#41204=CARTESIAN_POINT ( 'NONE',  ( -24.30112618867181240, -13.25578303422174997, 59.64795780745660636 ) ) ;
#41205=DIRECTION ( 'NONE',  ( 0.6973657521612035559, -0.7167154300785206766, 1.015100524683467946E-08 ) ) ;
#41206=EDGE_LOOP ( 'NONE', ( #13760, #22445, #35688, #11488, #41329 ) ) ;
#41209=CARTESIAN_POINT ( 'NONE',  ( -10.77303329795002895, -12.62668660113453178, 60.79853568451941470 ) ) ;
#41210=CARTESIAN_POINT ( 'NONE',  ( -17.95971906749393554, -21.78880692639934225, 61.87535914958314009 ) ) ;
#41214=CARTESIAN_POINT ( 'NONE',  ( -17.77159098340391097, -22.25115097675990583, 58.59827546209168503 ) ) ;
#41215=CARTESIAN_POINT ( 'NONE',  ( -24.27133562072960871, -13.11802050994479707, 59.24779033130878503 ) ) ;
#41217=CARTESIAN_POINT ( 'NONE',  ( -11.29821430689275630, -19.04912289309577744, 68.32415498359496553 ) ) ;
#41218=CARTESIAN_POINT ( 'NONE',  ( -15.37833354036149380, -8.114753493370539417, 74.15273655567226285 ) ) ;
#41219=PLANE ( 'NONE',  #18726 ) ;
#41220=( BOUNDED_SURFACE ( )  B_SPLINE_SURFACE ( 3, 1, ( 
 ( #22577, #29476 ),
 ( #37090, #26767 ),
 ( #26515, #18883 ),
 ( #3876, #3616 ),
 ( #40796, #34369 ),
 ( #45250, #30226 ),
 ( #8070, #7334 ) ),
 .UNSPECIFIED., .T., .F., .F. ) 
 B_SPLINE_SURFACE_WITH_KNOTS ( ( 4, 3, 4 ),
 ( 2, 2 ),
 ( 0.000000000000000000, 0.5000000000000000000, 1.000000000000000000 ),
 ( 0.000000000000000000, 1.000000000000000000 ),
 .UNSPECIFIED. ) 
 GEOMETRIC_REPRESENTATION_ITEM ( )  RATIONAL_B_SPLINE_SURFACE ( (
 ( 1.000000000000000000, 1.000000000000000000),
 ( 0.3333333333333335369, 0.3333333333333330373),
 ( 0.3333333333333335369, 0.3333333333333330373),
 ( 1.000000000000000000, 1.000000000000000000),
 ( 0.3333333333333333703, 0.3333333333333333703),
 ( 0.3333333333333333703, 0.3333333333333333703),
 ( 1.000000000000000000, 1.000000000000000000) ) ) 
 REPRESENTATION_ITEM ( '' )  SURFACE ( )  );
#41221=ADVANCED_FACE ( 'NONE', ( #10302 ), #14195, .T. ) ;
#41222=ORIENTED_EDGE ( 'NONE', *, *, #30174, .T. ) ;
#41223=CARTESIAN_POINT ( 'NONE',  ( -17.06879511326789256, -7.767867012253359071, 73.97490359703523666 ) ) ;
#41224=CARTESIAN_POINT ( 'NONE',  ( -10.07990710174555460, -16.41795825442990520, 53.76227901944321985 ) ) ;
#41228=CARTESIAN_POINT ( 'NONE',  ( -24.79685378108793259, -15.88006503112767476, 69.71120271104469168 ) ) ;
#41230=CARTESIAN_POINT ( 'NONE',  ( -10.84199182719153320, -17.34482810118634433, 61.36563051411450687 ) ) ;
#41231=( BOUNDED_CURVE ( )  B_SPLINE_CURVE ( 3, ( #38587, #27268, #42545, #15430 ),
 .UNSPECIFIED., .F., .F. ) 
 B_SPLINE_CURVE_WITH_KNOTS ( ( 4, 4 ),
 ( 0.4074455897393674531, 0.5000000000000000000 ),
 .UNSPECIFIED. ) 
 CURVE ( )  GEOMETRIC_REPRESENTATION_ITEM ( )  RATIONAL_B_SPLINE_CURVE ( ( 0.6983129098261020573, 0.7760317562606975361, 0.8765941196519944079, 0.9999999999999865663 ) ) 
 REPRESENTATION_ITEM ( '' )  );
#41233=ORIENTED_EDGE ( 'NONE', *, *, #44073, .F. ) ;
#41235=ADVANCED_FACE ( 'NONE', ( #36138 ), #47962, .T. ) ;
#41236=CARTESIAN_POINT ( 'NONE',  ( -10.45452701611611168, -14.15586467111139690, 61.21821260753697658 ) ) ;
#41237=CARTESIAN_POINT ( 'NONE',  ( -11.35719102664687874, -18.40077844947705188, 58.09242476654641507 ) ) ;
#41240=( BOUNDED_SURFACE ( )  B_SPLINE_SURFACE ( 3, 1, ( 
 ( #23828, #42543 ),
 ( #5107, #12956 ),
 ( #31443, #46479 ),
 ( #20120, #22926 ),
 ( #12732, #45323 ),
 ( #28239, #30313 ),
 ( #11575, #16887 ) ),
 .UNSPECIFIED., .T., .F., .F. ) 
 B_SPLINE_SURFACE_WITH_KNOTS ( ( 4, 3, 4 ),
 ( 2, 2 ),
 ( 0.000000000000000000, 0.5000000000000000000, 1.000000000000000000 ),
 ( 0.000000000000000000, 1.000000000000000000 ),
 .UNSPECIFIED. ) 
 GEOMETRIC_REPRESENTATION_ITEM ( )  RATIONAL_B_SPLINE_SURFACE ( (
 ( 1.000000000000000000, 1.000000000000000000),
 ( 0.3333333333333335369, 0.3333333333333330373),
 ( 0.3333333333333335369, 0.3333333333333330373),
 ( 1.000000000000000000, 1.000000000000000000),
 ( 0.3333333333333333703, 0.3333333333333333703),
 ( 0.3333333333333333703, 0.3333333333333333703),
 ( 1.000000000000000000, 1.000000000000000000) ) ) 
 REPRESENTATION_ITEM ( '' )  SURFACE ( )  );
#41243=EDGE_CURVE ( 'NONE', #33165, #36602, #5434, .T. ) ;
#41244=CARTESIAN_POINT ( 'NONE',  ( -15.39388989008627995, -21.97733388496078177, 72.23070757706680922 ) ) ;
#41246=CARTESIAN_POINT ( 'NONE',  ( -24.77723877343947478, -16.00713684962007122, 66.24820200538215431 ) ) ;
#41247=EDGE_CURVE ( 'NONE', #11764, #31313, #7007, .T. ) ;
#41249=CARTESIAN_POINT ( 'NONE',  ( -15.87557675045462169, -7.931373007531637320, 67.29007279016111909 ) ) ;
#41251=CARTESIAN_POINT ( 'NONE',  ( -24.85757945293173776, -20.98010847878158813, 54.49999999999995026 ) ) ;
#41252=LINE ( 'NONE', #625, #28406 ) ;
#41253=CARTESIAN_POINT ( 'NONE',  ( -11.32469144785208925, -18.34471071427194389, 57.80714594245691984 ) ) ;
#41255=CARTESIAN_POINT ( 'NONE',  ( -20.00946575929301474, -8.250368826910309039, 74.02096600124984604 ) ) ;
#41256=CARTESIAN_POINT ( 'NONE',  ( -15.31160308370628442, -21.95360096069865108, 72.20721981275677592 ) ) ;
#41259=ORIENTED_EDGE ( 'NONE', *, *, #27664, .F. ) ;
#41260=B_SPLINE_CURVE_WITH_KNOTS ( 'NONE', 3,
 ( #19505, #30857, #19025, #38203, #45868, #41680, #34031, #4255, #7965, #19766 ),
 .UNSPECIFIED., .F., .F.,
 ( 4, 2, 2, 2, 4 ),
 ( 0.000000000000000000, 0.2500000000000000000, 0.5000000000000000000, 0.7500000000000000000, 1.000000000000000000 ),
 .UNSPECIFIED. ) ;
#41261=CARTESIAN_POINT ( 'NONE',  ( -12.77796340496265870, -17.75258416873320400, 53.49999999999995026 ) ) ;
#41262=CARTESIAN_POINT ( 'NONE',  ( -10.74038475888173672, -11.51784756383862351, 71.22827500095982600 ) ) ;
#41263=FACE_BOUND ( 'NONE', #31319, .T. ) ;
#41264=B_SPLINE_CURVE_WITH_KNOTS ( 'NONE', 3,
 ( #28840, #10136, #25155, #21696, #6449, #2730, #17738, #45822, #15991, #4211 ),
 .UNSPECIFIED., .F., .F.,
 ( 4, 2, 2, 2, 4 ),
 ( 0.000000000000000000, 0.2500000000000000000, 0.5000000000000000000, 0.7500000000000000000, 1.000000000000000000 ),
 .UNSPECIFIED. ) ;
#41265=ORIENTED_EDGE ( 'NONE', *, *, #7171, .T. ) ;
#41267=CARTESIAN_POINT ( 'NONE',  ( -14.97188219925329378, -8.199429090594037461, 57.14999999999994174 ) ) ;
#41269=CARTESIAN_POINT ( 'NONE',  ( -23.93648101794248362, -17.51022725521227841, 65.95829288617392194 ) ) ;
#41271=CARTESIAN_POINT ( 'NONE',  ( -10.47603521207407518, -16.02136065384195973, 71.86239274348770323 ) ) ;
#41273=CARTESIAN_POINT ( 'NONE',  ( -12.72371041375474299, -9.029147237807901405, 70.94951108828513497 ) ) ;
#41274=CARTESIAN_POINT ( 'NONE',  ( -16.97112922959608383, -7.770054067326150005, 70.49035865952242830 ) ) ;
#41275=EDGE_CURVE ( 'NONE', #36030, #26171, #38784, .T. ) ;
#41277=EDGE_LOOP ( 'NONE', ( #15550, #29718, #16890, #7917, #16816 ) ) ;
#41278=CARTESIAN_POINT ( 'NONE',  ( -16.17771238455266314, -22.15437642958356435, 58.42439015775072875 ) ) ;
#41280=CARTESIAN_POINT ( 'NONE',  ( -18.37541875070384734, -22.19822623024843011, 69.01503475768117823 ) ) ;
#41282=AXIS2_PLACEMENT_3D ( 'NONE', #45946, #45722, #15387 ) ;
#41284=VERTEX_POINT ( 'NONE', #45917 ) ;
#41287=CARTESIAN_POINT ( 'NONE',  ( -21.26726687448728015, -20.65992264386038713, 69.28123431651795272 ) ) ;
#41288=CARTESIAN_POINT ( 'NONE',  ( -16.64495962069230117, -22.21910613783234822, 65.33909019606271329 ) ) ;
#41289=CARTESIAN_POINT ( 'NONE',  ( -24.23813412381375088, -12.99935709875259526, 66.31718868320673721 ) ) ;
#41291=EDGE_CURVE ( 'NONE', #11910, #1437, #42467, .T. ) ;
#41292=CARTESIAN_POINT ( 'NONE',  ( -19.41839133894716340, -8.097970443116885519, 60.03263303940221363 ) ) ;
#41293=ORIENTED_EDGE ( 'NONE', *, *, #12542, .F. ) ;
#41294=EDGE_LOOP ( 'NONE', ( #4936, #8563, #35437, #19350, #26824 ) ) ;
#41295=CARTESIAN_POINT ( 'NONE',  ( -16.22958052549516950, -7.455513305798441515, 60.45674424308347739 ) ) ;
#41296=CARTESIAN_POINT ( 'NONE',  ( -9.990623107247818879, -14.31192343302863179, 64.57299167182827659 ) ) ;
#41297=CARTESIAN_POINT ( 'NONE',  ( -10.40860991809309155, -15.50898095412354571, 57.85320721669017985 ) ) ;
#41302=EDGE_CURVE ( 'NONE', #26240, #44533, #33110, .T. ) ;
#41303=CARTESIAN_POINT ( 'NONE',  ( -16.05912136036848636, -21.67647323057698827, 58.39658775893972376 ) ) ;
#41305=EDGE_CURVE ( 'NONE', #41870, #37220, #20232, .T. ) ;
#41307=EDGE_CURVE ( 'NONE', #3548, #2848, #1320, .T. ) ;
#41309=FACE_OUTER_BOUND ( 'NONE', #48678, .T. ) ;
#41311=DIRECTION ( 'NONE',  ( -0.5263399769092093061, 0.8502742079512978224, 7.678741024442198749E-08 ) ) ;
#41313=VERTEX_POINT ( 'NONE', #46401 ) ;
#41316=CARTESIAN_POINT ( 'NONE',  ( -22.09139187696106887, -9.002414929697756918, 63.34153754183413554 ) ) ;
#41318=CARTESIAN_POINT ( 'NONE',  ( -10.50465667362414912, -15.86897300143100331, 64.50771547874023781 ) ) ;
#41319=EDGE_CURVE ( 'NONE', #1220, #31794, #32013, .T. ) ;
#41322=DIRECTION ( 'NONE',  ( 4.664556981411351282E-06, -8.285185778185610086E-06, 0.9999999999547987128 ) ) ;
#41323=ORIENTED_EDGE ( 'NONE', *, *, #19487, .T. ) ;
#41324=EDGE_CURVE ( 'NONE', #18740, #23020, #17252, .T. ) ;
#41325=EDGE_CURVE ( 'NONE', #14412, #27215, #33830, .T. ) ;
#41326=CARTESIAN_POINT ( 'NONE',  ( -21.35358943365839579, -4.907296734360127033, 54.60745305979834541 ) ) ;
#41327=CARTESIAN_POINT ( 'NONE',  ( -24.47217469005601131, -14.64471752244405067, 62.71296487297676947 ) ) ;
#41328=LINE ( 'NONE', #44797, #23396 ) ;
#41329=ORIENTED_EDGE ( 'NONE', *, *, #9712, .F. ) ;
#41331=CARTESIAN_POINT ( 'NONE',  ( -22.31145688432076568, -19.82056192467315370, 65.81307812901205523 ) ) ;
#41333=EDGE_LOOP ( 'NONE', ( #38938, #37128 ) ) ;
#41334=CARTESIAN_POINT ( 'NONE',  ( -19.61601503992405071, -21.50980213996393786, 65.76486213821364402 ) ) ;
#41336=LINE ( 'NONE', #7628, #27924 ) ;
#41338=VERTEX_POINT ( 'NONE', #23997 ) ;
#41339=CARTESIAN_POINT ( 'NONE',  ( -22.89702288877819214, -9.753446293288515534, 73.66816357947271854 ) ) ;
#41341=CARTESIAN_POINT ( 'NONE',  ( -10.39386236808646480, -14.28108337702217945, 64.38803875189576331 ) ) ;
#41343=CARTESIAN_POINT ( 'NONE',  ( -20.00308622248979162, -8.244632374337111713, 70.13611736960565679 ) ) ;
#41344=CARTESIAN_POINT ( 'NONE',  ( -11.12358220677134035, -11.75903396576748605, 71.08860871065073184 ) ) ;
#41345=CARTESIAN_POINT ( 'NONE',  ( -20.51476236319894753, -8.030485483676169878, 66.97378244640404432 ) ) ;
#41347=AXIS2_PLACEMENT_3D ( 'NONE', #13291, #28585, #39171 ) ;
#41349=CARTESIAN_POINT ( 'NONE',  ( -11.53247046633659245, -18.68106308600668441, 64.74707076449911369 ) ) ;
#41350=EDGE_CURVE ( 'NONE', #43006, #37616, #7350, .T. ) ;
#41358=CARTESIAN_POINT ( 'NONE',  ( -22.00903739223959477, -8.936221312270376416, 63.30498424023031845 ) ) ;
#41360=( BOUNDED_CURVE ( )  B_SPLINE_CURVE ( 3, ( #22010, #29154, #33544, #45167 ),
 .UNSPECIFIED., .F., .F. ) 
 B_SPLINE_CURVE_WITH_KNOTS ( ( 4, 4 ),
 ( 0.4074455897393693959, 0.5000000000000000000 ),
 .UNSPECIFIED. ) 
 CURVE ( )  GEOMETRIC_REPRESENTATION_ITEM ( )  RATIONAL_B_SPLINE_CURVE ( ( 0.6983129098261122714, 0.7760317562607196296, 0.8765941196520169454, 1.000000000000007550 ) ) 
 REPRESENTATION_ITEM ( '' )  );
#41361=ORIENTED_EDGE ( 'NONE', *, *, #46117, .T. ) ;
#41362=CARTESIAN_POINT ( 'NONE',  ( -15.09544296547830022, -21.46351980780830715, 65.25596681500472585 ) ) ;
#41363=CARTESIAN_POINT ( 'NONE',  ( -24.16575343130564590, -12.74704122656904914, 69.92243002240397232 ) ) ;
#41365=CARTESIAN_POINT ( 'NONE',  ( -22.04378365035703879, -20.13510231884741231, 62.24911246861644543 ) ) ;
#41367=ORIENTED_EDGE ( 'NONE', *, *, #27051, .T. ) ;
#41368=CARTESIAN_POINT ( 'NONE',  ( -19.96689475682054038, -8.233588121658772963, 74.01536847284175735 ) ) ;
#41369=( BOUNDED_CURVE ( )  B_SPLINE_CURVE ( 3, ( #28312, #42845, #38896, #9113 ),
 .UNSPECIFIED., .F., .F. ) 
 B_SPLINE_CURVE_WITH_KNOTS ( ( 4, 4 ),
 ( 0.5000000000000000000, 0.9074455897393642889 ),
 .UNSPECIFIED. ) 
 CURVE ( )  GEOMETRIC_REPRESENTATION_ITEM ( )  RATIONAL_B_SPLINE_CURVE ( ( 1.000000000000013323, 0.4567392136813366310, 0.3561768502900224953, 0.6983129098260856260 ) ) 
 REPRESENTATION_ITEM ( '' )  );
#41372=VERTEX_POINT ( 'NONE', #5278 ) ;
#41373=DIRECTION ( 'NONE',  ( 0.7364384864160969935, -0.6765045127160409510, -1.031360483216681931E-08 ) ) ;
#41374=CARTESIAN_POINT ( 'NONE',  ( -20.52762743779272014, -8.534807845156915818, 63.31121513079826713 ) ) ;
#41375=ORIENTED_EDGE ( 'NONE', *, *, #35383, .F. ) ;
#41377=EDGE_CURVE ( 'NONE', #47695, #48717, #23511, .T. ) ;
#41378=EDGE_CURVE ( 'NONE', #25345, #31288, #17059, .T. ) ;
#41381=DIRECTION ( 'NONE',  ( 2.662580029140978055E-06, -1.091441817711415488E-05, 0.9999999999368930359 ) ) ;
#41382=CARTESIAN_POINT ( 'NONE',  ( -10.79572390357762046, -11.40795830647630282, 67.80360014157953685 ) ) ;
#41383=CARTESIAN_POINT ( 'NONE',  ( -10.54224321960240651, -17.66275930416250262, 68.29710731422549941 ) ) ;
#41384=CARTESIAN_POINT ( 'NONE',  ( -13.36191307535780659, -8.564050219684345322, 57.16241883859221673 ) ) ;
#41385=ORIENTED_EDGE ( 'NONE', *, *, #36823, .T. ) ;
#41386=B_SPLINE_CURVE_WITH_KNOTS ( 'NONE', 1,
 ( #41555, #30730 ),
 .UNSPECIFIED., .F., .F.,
 ( 2, 2 ),
 ( 0.000000000000000000, 1.000000000000000000 ),
 .UNSPECIFIED. ) ;
#41387=CARTESIAN_POINT ( 'NONE',  ( -15.23931321672068329, -21.51228997375478968, 68.58152699338896241 ) ) ;
#41388=CARTESIAN_POINT ( 'NONE',  ( -10.37743716876973643, -14.51010320183636715, 64.27315137562472103 ) ) ;
#41389=CARTESIAN_POINT ( 'NONE',  ( -24.27033198218900978, -13.12649362337911718, 62.83264177274070050 ) ) ;
#41390=EDGE_CURVE ( 'NONE', #6207, #45223, #40085, .T. ) ;
#41392=LINE ( 'NONE', #11121, #8601 ) ;
#41394=VERTEX_POINT ( 'NONE', #35778 ) ;
#41395=EDGE_LOOP ( 'NONE', ( #33923, #30359, #15743, #1316, #28795 ) ) ;
#41396=CARTESIAN_POINT ( 'NONE',  ( -16.84904595140906025, -21.78683020288652372, 72.23713474854929473 ) ) ;
#41398=EDGE_LOOP ( 'NONE', ( #30815, #9277 ) ) ;
#41400=CARTESIAN_POINT ( 'NONE',  ( -23.96075645138428456, -17.45014240273063066, 65.94357239682317129 ) ) ;
#41401=CARTESIAN_POINT ( 'NONE',  ( -11.91470689456726717, -9.793200236000155101, 64.21569601040394559 ) ) ;
#41402=DIRECTION ( 'NONE',  ( 0.3224496555704357559, 0.8691421305882567339, 0.3749909018349820711 ) ) ;
#41403=CARTESIAN_POINT ( 'NONE',  ( -21.59090693955708318, -20.98503893958440258, 72.63108097743202052 ) ) ;
#41404=CARTESIAN_POINT ( 'NONE',  ( -10.82793724842355765, -11.34591556451386651, 67.87510537416113721 ) ) ;
#41406=CARTESIAN_POINT ( 'NONE',  ( -10.90759836534377492, -17.49952001658422063, 68.39721944423101263 ) ) ;
#41408=ADVANCED_FACE ( 'NONE', ( #6494 ), #6249, .T. ) ;
#41409=DIRECTION ( 'NONE',  ( -4.436160455182634911E-06, -7.761523761658527715E-06, 0.9999999999600395206 ) ) ;
#41410=CARTESIAN_POINT ( 'NONE',  ( -14.98927377128279304, -8.246306944878790901, 47.99999999999994316 ) ) ;
#41411=CARTESIAN_POINT ( 'NONE',  ( -15.54561509764458371, -8.065849839147006151, 74.37985694181431029 ) ) ;
#41414=DIRECTION ( 'NONE',  ( 0.7489133456531319455, 0.6626679415081376812, -6.686399186099785819E-09 ) ) ;
#41415=CARTESIAN_POINT ( 'NONE',  ( -17.78516316699992217, -21.85793681952389989, 65.48965078530844153 ) ) ;
#41418=VERTEX_POINT ( 'NONE', #9218 ) ;
#41420=ORIENTED_EDGE ( 'NONE', *, *, #11660, .T. ) ;
#41424=CARTESIAN_POINT ( 'NONE',  ( -11.28350022557402177, -11.44842874720234427, 64.44882000253240051 ) ) ;
#41425=CARTESIAN_POINT ( 'NONE',  ( -17.04413539470109740, -21.84925844046378174, 72.45071136019464575 ) ) ;
#41426=ORIENTED_EDGE ( 'NONE', *, *, #11192, .T. ) ;
#41429=ORIENTED_EDGE ( 'NONE', *, *, #46729, .T. ) ;
#41431=CARTESIAN_POINT ( 'NONE',  ( -19.17437844398820701, -7.979623566120205957, 63.44561363416070776 ) ) ;
#41432=VERTEX_POINT ( 'NONE', #32103 ) ;
#41433=CARTESIAN_POINT ( 'NONE',  ( -10.37795889460693033, -14.56696403379599225, 68.14328054657653411 ) ) ;
#41434=FACE_OUTER_BOUND ( 'NONE', #5862, .T. ) ;
#41435=CARTESIAN_POINT ( 'NONE',  ( -17.23716279620991187, -7.361383508276583498, 70.63002447061150235 ) ) ;
#41437=CARTESIAN_POINT ( 'NONE',  ( -19.78614083979442029, -21.39864764726399216, 69.23482476778590922 ) ) ;
#41439=DIRECTION ( 'NONE',  ( -2.575747231244379256E-06, 1.267954838346457742E-05, 0.9999999999162972886 ) ) ;
#41440=CARTESIAN_POINT ( 'NONE',  ( -24.72811879990099726, -13.33785195616451169, 59.54923321989076612 ) ) ;
#41442=ORIENTED_EDGE ( 'NONE', *, *, #34226, .T. ) ;
#41445=CARTESIAN_POINT ( 'NONE',  ( -10.74942749874026759, -12.69977847772782376, 61.08388229708562989 ) ) ;
#41446=AXIS2_PLACEMENT_3D ( 'NONE', #27181, #42203, #12397 ) ;
#41447=CARTESIAN_POINT ( 'NONE',  ( -23.70015231925135168, -18.82353928378165975, 69.47867257277708575 ) ) ;
#41448=CARTESIAN_POINT ( 'NONE',  ( -23.90395749478602383, -11.13306750868542316, 70.09199524523918967 ) ) ;
#41449=EDGE_CURVE ( 'NONE', #34559, #26512, #41966, .T. ) ;
#41450=EDGE_CURVE ( 'NONE', #26955, #35971, #28444, .T. ) ;
#41451=CARTESIAN_POINT ( 'NONE',  ( -11.09851747596991700, -11.69606064988821714, 71.09420651392984780 ) ) ;
#41454=ADVANCED_FACE ( 'NONE', ( #10190 ), #47126, .F. ) ;
#41455=CARTESIAN_POINT ( 'NONE',  ( -24.65023673758593148, -12.99629830290576038, 63.01759453279318279 ) ) ;
#41456=CARTESIAN_POINT ( 'NONE',  ( -14.54749350918765671, -8.372447261038937327, 64.07506791522041567 ) ) ;
#41457=ORIENTED_EDGE ( 'NONE', *, *, #45976, .F. ) ;
#41458=CARTESIAN_POINT ( 'NONE',  ( -11.33913397532896461, -19.10776957548626953, 68.39406486076410374 ) ) ;
#41460=AXIS2_PLACEMENT_3D ( 'NONE', #11461, #45452, #11710 ) ;
#41461=EDGE_CURVE ( 'NONE', #47803, #7640, #16114, .T. ) ;
#41462=CARTESIAN_POINT ( 'NONE',  ( -15.43407032490635267, -8.097972375076935236, 74.36520272443641488 ) ) ;
#41463=CARTESIAN_POINT ( 'NONE',  ( -13.65828898514496359, -20.76952646431350757, 65.00101022825411690 ) ) ;
#41465=CARTESIAN_POINT ( 'NONE',  ( -18.39951258112534305, -22.19516185762106275, 69.00009993223443416 ) ) ;
#41466=CARTESIAN_POINT ( 'NONE',  ( -10.06879755192725412, -15.99802040037407203, 64.62116216602396435 ) ) ;
#41471=CARTESIAN_POINT ( 'NONE',  ( -20.57278697373333998, -8.057206101692887756, 66.89608655064280640 ) ) ;
#41473=CARTESIAN_POINT ( 'NONE',  ( -24.85158094034050436, -14.23037817089475787, 69.85286472968408589 ) ) ;
#41476=ORIENTED_EDGE ( 'NONE', *, *, #829, .F. ) ;
#41477=B_SPLINE_CURVE_WITH_KNOTS ( 'NONE', 1,
 ( #31914, #27732 ),
 .UNSPECIFIED., .F., .F.,
 ( 2, 2 ),
 ( 0.000000000000000000, 1.000000000000000000 ),
 .UNSPECIFIED. ) ;
#41479=CARTESIAN_POINT ( 'NONE',  ( -20.25191534917341230, -8.350868906188830820, 70.26572394742477456 ) ) ;
#41480=CARTESIAN_POINT ( 'NONE',  ( -19.36518065869528726, -8.031383756764064685, 59.97565108339750850 ) ) ;
#41482=VECTOR ( 'NONE', #8126, 999.9999999999998863 ) ;
#41484=B_SPLINE_CURVE_WITH_KNOTS ( 'NONE', 3,
 ( #2932, #2216, #47530, #17226, #28575, #32273, #25590, #47293, #9861, #44559 ),
 .UNSPECIFIED., .F., .F.,
 ( 4, 2, 2, 2, 4 ),
 ( 0.000000000000000000, 0.2500000000000000000, 0.5000000000000000000, 0.7500000000000000000, 1.000000000000000000 ),
 .UNSPECIFIED. ) ;
#41485=CARTESIAN_POINT ( 'NONE',  ( -16.29356323290813435, -7.846682106953448255, 63.97011323776958847 ) ) ;
#41486=CARTESIAN_POINT ( 'NONE',  ( -10.21805405031902225, -12.91800167290361578, 67.78186406512817541 ) ) ;
#41491=ORIENTED_EDGE ( 'NONE', *, *, #29731, .T. ) ;
#41492=DIRECTION ( 'NONE',  ( -5.731567514496413899E-31, -1.020425574103664789E-16, -1.000000000000000000 ) ) ;
#41495=CARTESIAN_POINT ( 'NONE',  ( -13.12790236870489302, -8.721809449924828428, 64.09601920791236296 ) ) ;
#41496=CARTESIAN_POINT ( 'NONE',  ( -21.12516169987187098, -20.80993955427394582, 69.06922321213187388 ) ) ;
#41497=DIRECTION ( 'NONE',  ( 0.9375570856950865561, -0.3478314405900308492, 0.000000000000000000 ) ) ;
#41498=CARTESIAN_POINT ( 'NONE',  ( -17.72634068467203505, -21.85272461955047874, 58.70553378267869249 ) ) ;
#41499=EDGE_CURVE ( 'NONE', #36571, #27722, #9881, .T. ) ;
#41500=ORIENTED_EDGE ( 'NONE', *, *, #16489, .T. ) ;
#41501=FACE_OUTER_BOUND ( 'NONE', #32354, .T. ) ;
#41502=CARTESIAN_POINT ( 'NONE',  ( -24.42218830102925509, -14.64588410380239480, 62.71296487252168816 ) ) ;
#41503=( BOUNDED_CURVE ( )  B_SPLINE_CURVE ( 3, ( #28222, #9038, #16875, #47428 ),
 .UNSPECIFIED., .F., .F. ) 
 B_SPLINE_CURVE_WITH_KNOTS ( ( 4, 4 ),
 ( 0.9074455897393589598, 1.000000000000000000 ),
 .UNSPECIFIED. ) 
 CURVE ( )  GEOMETRIC_REPRESENTATION_ITEM ( )  RATIONAL_B_SPLINE_CURVE ( ( 0.6983129098260747458, 0.7760317562606824371, 0.8765941196519908551, 1.000000000000000000 ) ) 
 REPRESENTATION_ITEM ( '' )  );
#41504=CARTESIAN_POINT ( 'NONE',  ( -20.04802834295863789, -8.319537469032344035, 70.32388470383602908 ) ) ;
#41505=CARTESIAN_POINT ( 'NONE',  ( -10.07920524814866958, -16.05700196042000272, 68.10050966415293772 ) ) ;
#41506=ORIENTED_EDGE ( 'NONE', *, *, #25160, .T. ) ;
#41507=LINE ( 'NONE', #44731, #38556 ) ;
#41508=CARTESIAN_POINT ( 'NONE',  ( -15.62037199135231980, -25.42245057690201193, 54.61912878955446615 ) ) ;
#41509=CARTESIAN_POINT ( 'NONE',  ( -18.83585931754296183, -7.494105970839488151, 70.48572750873847781 ) ) ;
#41510=FACE_BOUND ( 'NONE', #4350, .T. ) ;
#41511=ORIENTED_EDGE ( 'NONE', *, *, #5297, .T. ) ;
#41512=CYLINDRICAL_SURFACE ( 'NONE', #39981, 0.1500000000000022704 ) ;
#41513=CARTESIAN_POINT ( 'NONE',  ( -10.48067290732983281, -16.03043740265091444, 67.97767830707738312 ) ) ;
#41514=CARTESIAN_POINT ( 'NONE',  ( -10.93232766038821424, -17.55941949638709687, 68.38249893951126523 ) ) ;
#41515=EDGE_CURVE ( 'NONE', #35967, #11672, #886, .T. ) ;
#41518=ORIENTED_EDGE ( 'NONE', *, *, #33554, .F. ) ;
#41520=EDGE_CURVE ( 'NONE', #4699, #46319, #41962, .T. ) ;
#41521=ORIENTED_EDGE ( 'NONE', *, *, #39975, .F. ) ;
#41522=CARTESIAN_POINT ( 'NONE',  ( -10.34288728022239923, -21.73268535153714254, 53.49999999999995026 ) ) ;
#41523=CARTESIAN_POINT ( 'NONE',  ( -10.99655737938916289, -18.57624151290433900, 57.99209991576458378 ) ) ;
#41524=CARTESIAN_POINT ( 'NONE',  ( -21.59992848427141965, -8.639514894543184553, 73.70154514716914207 ) ) ;
#41526=( BOUNDED_CURVE ( )  B_SPLINE_CURVE ( 3, ( #30210, #23062, #33613, #44992 ),
 .UNSPECIFIED., .F., .F. ) 
 B_SPLINE_CURVE_WITH_KNOTS ( ( 4, 4 ),
 ( 0.4074455897393624570, 0.5000000000000000000 ),
 .UNSPECIFIED. ) 
 CURVE ( )  GEOMETRIC_REPRESENTATION_ITEM ( )  RATIONAL_B_SPLINE_CURVE ( ( 0.6983129098260937306, 0.7760317562606965369, 0.8765941196519979606, 0.9999999999999963363 ) ) 
 REPRESENTATION_ITEM ( '' )  );
#41533=ORIENTED_EDGE ( 'NONE', *, *, #26318, .F. ) ;
#41534=LINE ( 'NONE', #424, #2890 ) ;
#41537=CARTESIAN_POINT ( 'NONE',  ( -19.37616851487812752, -21.99900361761337919, 58.71002773933979313 ) ) ;
#41538=CARTESIAN_POINT ( 'NONE',  ( -10.57910610510154470, -13.34370840258270441, 74.97817676091081296 ) ) ;
#41539=EDGE_CURVE ( 'NONE', #9250, #5475, #43550, .T. ) ;
#41541=CARTESIAN_POINT ( 'NONE',  ( -14.21691873732594402, -8.585707597842299421, 74.27124835653124535 ) ) ;
#41542=DIRECTION ( 'NONE',  ( 1.424565731581784133E-06, -1.060674514654238452E-05, 0.9999999999427338082 ) ) ;
#41545=ORIENTED_EDGE ( 'NONE', *, *, #6056, .F. ) ;
#41546=EDGE_LOOP ( 'NONE', ( #11781, #35821, #23341, #6874, #3458 ) ) ;
#41547=CARTESIAN_POINT ( 'NONE',  ( -17.56717618076180187, -7.360494862701306928, 63.73552352176282909 ) ) ;
#41548=CARTESIAN_POINT ( 'NONE',  ( -11.86838291625971742, -9.845553222893467904, 64.14418898700822069 ) ) ;
#41549=DIRECTION ( 'NONE',  ( 0.9893521221787096032, -0.1455416721783832079, -6.188545272020241572E-08 ) ) ;
#41550=PLANE ( 'NONE',  #46478 ) ;
#41551=ORIENTED_EDGE ( 'NONE', *, *, #29829, .T. ) ;
#41553=B_SPLINE_CURVE_WITH_KNOTS ( 'NONE', 3,
 ( #38414, #520, #34733, #45111, #33746, #22436, #11357, #37430, #3979, #3725 ),
 .UNSPECIFIED., .F., .F.,
 ( 4, 2, 2, 2, 4 ),
 ( 0.000000000000000000, 0.2500000000000000000, 0.5000000000000000000, 0.7500000000000000000, 1.000000000000000000 ),
 .UNSPECIFIED. ) ;
#41554=ORIENTED_EDGE ( 'NONE', *, *, #46908, .F. ) ;
#41555=CARTESIAN_POINT ( 'NONE',  ( -10.41531639268335496, -14.04517892474411589, 60.93293405735092705 ) ) ;
#41558=STYLED_ITEM ( 'NONE', ( #27243 ), #48318 ) ;
#41559=ADVANCED_FACE ( 'NONE', ( #74 ), #48089, .T. ) ;
#41561=CARTESIAN_POINT ( 'NONE',  ( -16.39887994223181167, -21.73372354711506560, 61.75568132718285597 ) ) ;
#41562=VECTOR ( 'NONE', #46502, 1000.000000000000227 ) ;
#41564=CARTESIAN_POINT ( 'NONE',  ( -10.47368616940683772, -17.49164935309025282, 64.67093470525151133 ) ) ;
#41565=CARTESIAN_POINT ( 'NONE',  ( -24.18257650347943866, -11.67453741916809662, 59.58897441446281817 ) ) ;
#41566=ORIENTED_EDGE ( 'NONE', *, *, #46092, .T. ) ;
#41569=CARTESIAN_POINT ( 'NONE',  ( -10.06879755192725412, -15.99802040037407203, 64.62116216602396435 ) ) ;
#41572=CARTESIAN_POINT ( 'NONE',  ( -16.04133765461606842, -7.488482771185046794, 63.80977704063102607 ) ) ;
#41573=ORIENTED_EDGE ( 'NONE', *, *, #30490, .T. ) ;
#41575=CARTESIAN_POINT ( 'NONE',  ( -24.27661814142333796, -16.49973396376381984, 62.73761853866894711 ) ) ;
#41579=CARTESIAN_POINT ( 'NONE',  ( -20.29576920503309623, -8.423958534466374104, 70.47930128339966416 ) ) ;
#41581=ORIENTED_EDGE ( 'NONE', *, *, #6660, .T. ) ;
#41582=DIRECTION ( 'NONE',  ( 0.7800143876985550229, -0.6257615799833393666, 5.505484597913564244E-08 ) ) ;
#41584=FACE_OUTER_BOUND ( 'NONE', #103, .T. ) ;
#41585=EDGE_LOOP ( 'NONE', ( #35494, #40657, #44990, #14335, #38423 ) ) ;
#41586=CARTESIAN_POINT ( 'NONE',  ( -11.10470791607724550, -18.75498134223953883, 61.46206221440264983 ) ) ;
#41587=EDGE_CURVE ( 'NONE', #6672, #7125, #37221, .T. ) ;
#41588=CARTESIAN_POINT ( 'NONE',  ( -21.25455046938168735, -8.881090050001144931, 70.28699408244519020 ) ) ;
#41589=ORIENTED_EDGE ( 'NONE', *, *, #29043, .F. ) ;
#41591=CARTESIAN_POINT ( 'NONE',  ( -10.47299162366406478, -15.63514707757639854, 61.33789045486464886 ) ) ;
#41592=DIRECTION ( 'NONE',  ( -5.731567514496413899E-31, -1.020425574103664789E-16, -1.000000000000000000 ) ) ;
#41594=PLANE ( 'NONE',  #5261 ) ;
#41600=CARTESIAN_POINT ( 'NONE',  ( -10.70566866894272984, -16.94585410378973123, 57.98760548748136046 ) ) ;
#41602=AXIS2_PLACEMENT_3D ( 'NONE', #16277, #1042, #8429 ) ;
#41603=CARTESIAN_POINT ( 'NONE',  ( -9.974215857974789046, -14.86484893678357544, 74.91283499353951925 ) ) ;
#41605=CARTESIAN_POINT ( 'NONE',  ( -20.37299750454370439, -8.405577324698718655, 66.78104082189589974 ) ) ;
#41606=CARTESIAN_POINT ( 'NONE',  ( -19.39856565954547207, -21.58093498248654996, 65.76486340091366856 ) ) ;
#41607=CARTESIAN_POINT ( 'NONE',  ( -21.84382042562961246, -9.380945574151434485, 59.91274429023591352 ) ) ;
#41608=EDGE_CURVE ( 'NONE', #12328, #24536, #14359, .T. ) ;
#41610=EDGE_CURVE ( 'NONE', #18022, #4434, #30805, .T. ) ;
#41611=ORIENTED_EDGE ( 'NONE', *, *, #44912, .T. ) ;
#41612=ADVANCED_FACE ( 'NONE', ( #44645 ), #40938, .T. ) ;
#41613=CARTESIAN_POINT ( 'NONE',  ( -23.40706704545067041, -18.44294168544361057, 72.76368236816873036 ) ) ;
#41614=DIRECTION ( 'NONE',  ( -0.2771212459065067191, 0.9608349572466771127, 4.100231986695772107E-08 ) ) ;
#41615=CARTESIAN_POINT ( 'NONE',  ( -13.29845767883066543, -21.01266560759323809, 61.63150935275904629 ) ) ;
#41617=ORIENTED_EDGE ( 'NONE', *, *, #813, .F. ) ;
#41618=CARTESIAN_POINT ( 'NONE',  ( -10.61330328728660533, -12.98831903967553636, 67.73832347272893628 ) ) ;
#41619=FACE_OUTER_BOUND ( 'NONE', #41294, .T. ) ;
#41621=CARTESIAN_POINT ( 'NONE',  ( -14.80056147340629380, -21.78207226143426922, 61.82095877133116346 ) ) ;
#41625=LINE ( 'NONE', #18465, #24948 ) ;
#41627=CARTESIAN_POINT ( 'NONE',  ( -12.30444741248500051, -20.22242042389802918, 64.98019641849691652 ) ) ;
#41630=ORIENTED_EDGE ( 'NONE', *, *, #37603, .F. ) ;
#41633=ORIENTED_EDGE ( 'NONE', *, *, #35045, .T. ) ;
#41636=CARTESIAN_POINT ( 'NONE',  ( -17.68496342731873483, -21.80445415968011247, 58.40553376440286115 ) ) ;
#41637=DIRECTION ( 'NONE',  ( -0.4501286257827956661, -0.8929637284072021730, 1.500157795982635103E-08 ) ) ;
#41638=CARTESIAN_POINT ( 'NONE',  ( -22.20320197231171733, -19.92390356480266433, 66.00421731406686376 ) ) ;
#41640=ORIENTED_EDGE ( 'NONE', *, *, #42600, .T. ) ;
#41642=CARTESIAN_POINT ( 'NONE',  ( -12.52476177601987040, -19.87868524014693605, 65.16674890854918090 ) ) ;
#41643=ADVANCED_FACE ( 'NONE', ( #317 ), #45630, .T. ) ;
#41645=CARTESIAN_POINT ( 'NONE',  ( -17.20139249542113191, -7.812750000685961815, 70.49035839633111777 ) ) ;
#41646=ORIENTED_EDGE ( 'NONE', *, *, #37354, .F. ) ;
#41648=ADVANCED_FACE ( 'NONE', ( #8196 ), #38878, .T. ) ;
#41649=CARTESIAN_POINT ( 'NONE',  ( -21.36950656924352288, -9.026883429518402835, 73.90128804929361195 ) ) ;
#41650=CARTESIAN_POINT ( 'NONE',  ( -14.66963140629840190, -7.887024584555132556, 60.57642187187276051 ) ) ;
#41651=ORIENTED_EDGE ( 'NONE', *, *, #44238, .F. ) ;
#41652=CARTESIAN_POINT ( 'NONE',  ( -20.99144087168200912, -21.34977411167369610, 62.27617921724772998 ) ) ;
#41653=CARTESIAN_POINT ( 'NONE',  ( -24.71334378318632830, -13.26952680650525274, 59.47772536435775947 ) ) ;
#41654=CARTESIAN_POINT ( 'NONE',  ( -10.27345454978659944, -12.71824136398891980, 64.45331520391344782 ) ) ;
#41655=CARTESIAN_POINT ( 'NONE',  ( -10.45256735519816615, -15.43993469624229853, 57.56792809193251514 ) ) ;
#41656=( BOUNDED_CURVE ( )  B_SPLINE_CURVE ( 3, ( #303, #7446, #21719, #25650 ),
 .UNSPECIFIED., .F., .F. ) 
 B_SPLINE_CURVE_WITH_KNOTS ( ( 4, 4 ),
 ( 0.000000000000000000, 0.4074455897393669535 ),
 .UNSPECIFIED. ) 
 CURVE ( )  GEOMETRIC_REPRESENTATION_ITEM ( )  RATIONAL_B_SPLINE_CURVE ( ( 1.000000000000000000, 0.4567392136813300807, 0.3561768502900296007, 0.6983129098260987266 ) ) 
 REPRESENTATION_ITEM ( '' )  );
#41657=CARTESIAN_POINT ( 'NONE',  ( -21.53861794036900079, -21.02004141303368101, 72.63951040967180006 ) ) ;
#41658=CARTESIAN_POINT ( 'NONE',  ( -23.57293185872052632, -19.01568291639688724, 65.92365791119206619 ) ) ;
#41662=CARTESIAN_POINT ( 'NONE',  ( -10.56492563526530759, -13.18000101695786341, 71.20828586226983248 ) ) ;
#41664=CARTESIAN_POINT ( 'NONE',  ( -24.16627971075339332, -12.73851560842801867, 66.18757903754330130 ) ) ;
#41665=( BOUNDED_CURVE ( )  B_SPLINE_CURVE ( 3, ( #16773, #44125, #21216, #2008 ),
 .UNSPECIFIED., .F., .F. ) 
 B_SPLINE_CURVE_WITH_KNOTS ( ( 4, 4 ),
 ( 0.9074455897393635118, 1.000000000000000000 ),
 .UNSPECIFIED. ) 
 CURVE ( )  GEOMETRIC_REPRESENTATION_ITEM ( )  RATIONAL_B_SPLINE_CURVE ( ( 0.6983129098260841827, 0.7760317562606905417, 0.8765941196519958512, 1.000000000000000000 ) ) 
 REPRESENTATION_ITEM ( '' )  );
#41668=EDGE_CURVE ( 'NONE', #28824, #4171, #48386, .T. ) ;
#41669=ORIENTED_EDGE ( 'NONE', *, *, #14171, .T. ) ;
#41672=VERTEX_POINT ( 'NONE', #23935 ) ;
#41673=EDGE_CURVE ( 'NONE', #1437, #9257, #19758, .T. ) ;
#41677=CARTESIAN_POINT ( 'NONE',  ( -10.52215064345839757, -13.37195933026064232, 74.82817647370434599 ) ) ;
#41679=( BOUNDED_SURFACE ( )  B_SPLINE_SURFACE ( 3, 1, ( 
 ( #25089, #32701 ),
 ( #47729, #6614 ),
 ( #40109, #14211 ),
 ( #39617, #47498 ),
 ( #13967, #32239 ),
 ( #29016, #44064 ),
 ( #35904, #13248 ) ),
 .UNSPECIFIED., .T., .F., .F. ) 
 B_SPLINE_SURFACE_WITH_KNOTS ( ( 4, 3, 4 ),
 ( 2, 2 ),
 ( 0.000000000000000000, 0.5000000000000000000, 1.000000000000000000 ),
 ( 0.000000000000000000, 1.000000000000000000 ),
 .UNSPECIFIED. ) 
 GEOMETRIC_REPRESENTATION_ITEM ( )  RATIONAL_B_SPLINE_SURFACE ( (
 ( 1.000000000000000000, 1.000000000000000000),
 ( 0.3333333333333335369, 0.3333333333333330373),
 ( 0.3333333333333335369, 0.3333333333333330373),
 ( 1.000000000000000000, 1.000000000000000000),
 ( 0.3333333333333333703, 0.3333333333333333703),
 ( 0.3333333333333333703, 0.3333333333333333703),
 ( 1.000000000000000000, 1.000000000000000000) ) ) 
 REPRESENTATION_ITEM ( '' )  SURFACE ( )  );
#41680=CARTESIAN_POINT ( 'NONE',  ( -13.61216739602634007, -20.68217155920894967, 65.17556062011875895 ) ) ;
#41681=DIRECTION ( 'NONE',  ( -0.3478314405900341799, -0.9375570856950852239, 0.000000000000000000 ) ) ;
#41682=VECTOR ( 'NONE', #30024, 1000.000000000000227 ) ;
#41683=EDGE_LOOP ( 'NONE', ( #5025, #48165 ) ) ;
#41684=CARTESIAN_POINT ( 'NONE',  ( -13.95528965362524332, -21.40322351219866093, 72.03952346373179694 ) ) ;
#41685=CARTESIAN_POINT ( 'NONE',  ( -18.59601872632196518, -7.856991649524070809, 73.85536540707786912 ) ) ;
#41687=CARTESIAN_POINT ( 'NONE',  ( -11.47316209429933132, -11.02906371526824536, 57.20903242655475651 ) ) ;
#41690=CARTESIAN_POINT ( 'NONE',  ( -24.47432067347917695, -14.77756146504815327, 59.52828185648635184 ) ) ;
#41693=ORIENTED_EDGE ( 'NONE', *, *, #31431, .F. ) ;
#41694=CARTESIAN_POINT ( 'NONE',  ( -23.20398631485561225, -10.10837353526244087, 63.21039459454670606 ) ) ;
#41699=CARTESIAN_POINT ( 'NONE',  ( -16.11719258475605443, -7.932175852977164432, 63.67011080781733057 ) ) ;
#41700=CARTESIAN_POINT ( 'NONE',  ( -24.47405849404658795, -12.40054206295432770, 73.28579645182460922 ) ) ;
#41702=CARTESIAN_POINT ( 'NONE',  ( -11.08030728566740741, -11.72680384936461806, 74.97328630331448096 ) ) ;
#41703=CARTESIAN_POINT ( 'NONE',  ( -15.81235419205221504, -7.945607373518417837, 67.42535135806457447 ) ) ;
#41706=CARTESIAN_POINT ( 'NONE',  ( -23.93425983466340057, -11.18667287686709777, 70.03177400573818545 ) ) ;
#41707=CARTESIAN_POINT ( 'NONE',  ( -10.47914967500843986, -15.69558290523237076, 64.57941926453548831 ) ) ;
#41709=ORIENTED_EDGE ( 'NONE', *, *, #47185, .F. ) ;
#41710=ADVANCED_FACE ( 'NONE', ( #4982 ), #3637, .T. ) ;
#41711=CARTESIAN_POINT ( 'NONE',  ( -11.03962565240155591, -10.96946996027528876, 60.81852449360508928 ) ) ;
#41712=ORIENTED_EDGE ( 'NONE', *, *, #37651, .F. ) ;
#41713=CARTESIAN_POINT ( 'NONE',  ( -24.43817019563415371, -15.55591454009146979, 69.53307225875056474 ) ) ;
#41716=CARTESIAN_POINT ( 'NONE',  ( -18.41501299910237677, -20.23286350246260312, 53.88362224778186516 ) ) ;
#41718=CARTESIAN_POINT ( 'NONE',  ( -16.95423314674965098, -22.24437505095468026, 72.31543220464045874 ) ) ;
#41719=CARTESIAN_POINT ( 'NONE',  ( -17.26457240846633923, -7.760713630915982542, 70.50507891880883449 ) ) ;
#41720=CARTESIAN_POINT ( 'NONE',  ( -18.33614212499659502, -22.20322161997698629, 68.92240557158177694 ) ) ;
#41725=CARTESIAN_POINT ( 'NONE',  ( -16.01003035779492834, -7.894338788008341545, 70.75422978485266867 ) ) ;
#41726=DIRECTION ( 'NONE',  ( 0.3109111061729913916, 0.9504389954427825415, 3.354176643444177759E-08 ) ) ;
#41727=EDGE_LOOP ( 'NONE', ( #42638, #19841, #40192, #16798, #39629 ) ) ;
#41728=VERTEX_POINT ( 'NONE', #35956 ) ;
#41730=EDGE_CURVE ( 'NONE', #1862, #21555, #28592, .T. ) ;
#41734=CARTESIAN_POINT ( 'NONE',  ( -10.52991701743181174, -16.02177613136639067, 67.97767831076122036 ) ) ;
#41735=CARTESIAN_POINT ( 'NONE',  ( -18.96529421678551230, -7.929577530235508043, 66.90631605115711977 ) ) ;
#41740=EDGE_CURVE ( 'NONE', #43099, #7039, #10808, .T. ) ;
#41742=DIRECTION ( 'NONE',  ( -6.023555224489876859E-06, 1.003033500230846996E-05, -0.9999999999315546395 ) ) ;
#41743=ADVANCED_FACE ( 'NONE', ( #9155 ), #1998, .T. ) ;
#41746=CARTESIAN_POINT ( 'NONE',  ( -24.30048669258562200, -16.36410883687464946, 59.42332431756338451 ) ) ;
#41750=CARTESIAN_POINT ( 'NONE',  ( -22.17046091269999764, -9.065891900838490614, 59.83515915777798710 ) ) ;
#41751=CARTESIAN_POINT ( 'NONE',  ( -13.65684165595416921, -8.849801312179289781, 56.98439896120441261 ) ) ;
#41752=CARTESIAN_POINT ( 'NONE',  ( -12.53241260230162624, -9.190070326428815051, 74.42584683763180919 ) ) ;
#41753=LINE ( 'NONE', #31144, #255 ) ;
#41755=VECTOR ( 'NONE', #11167, 1000.000000000000000 ) ;
#41758=LINE ( 'NONE', #4329, #31299 ) ;
#41759=( BOUNDED_CURVE ( )  B_SPLINE_CURVE ( 3, ( #29220, #2860, #28500, #17633 ),
 .UNSPECIFIED., .F., .F. ) 
 B_SPLINE_CURVE_WITH_KNOTS ( ( 4, 4 ),
 ( 0.4074455897393630122, 0.5000000000000000000 ),
 .UNSPECIFIED. ) 
 CURVE ( )  GEOMETRIC_REPRESENTATION_ITEM ( )  RATIONAL_B_SPLINE_CURVE ( ( 0.6983129098260898449, 0.7760317562606893205, 0.8765941196519910772, 0.9999999999999903411 ) ) 
 REPRESENTATION_ITEM ( '' )  );
#41760=DIRECTION ( 'NONE',  ( -0.6973657521612036669, 0.7167154300785205656, -1.015100525525034718E-08 ) ) ;
#41761=CARTESIAN_POINT ( 'NONE',  ( -24.48057421083657914, -17.19850309837678637, 72.98312409556710634 ) ) ;
#41763=CARTESIAN_POINT ( 'NONE',  ( -10.55442330881768775, -17.69226200592865794, 68.27438864859273338 ) ) ;
#41764=CARTESIAN_POINT ( 'NONE',  ( -10.97586111044497947, -17.65935802862028936, 71.56718190231987364 ) ) ;
#41766=FACE_BOUND ( 'NONE', #33677, .T. ) ;
#41770=CARTESIAN_POINT ( 'NONE',  ( -21.18000274887674905, -20.77541536365158592, 69.05450184741354747 ) ) ;
#41773=CARTESIAN_POINT ( 'NONE',  ( -21.61813247623101830, -8.651786778886961571, 73.71633474065167491 ) ) ;
#41774=ORIENTED_EDGE ( 'NONE', *, *, #43521, .T. ) ;
#41776=DIRECTION ( 'NONE',  ( -0.2122660683108583690, 0.9772119095896469876, -7.504255179299140299E-08 ) ) ;
#41777=CARTESIAN_POINT ( 'NONE',  ( -22.96794543296044466, -10.53327132317364168, 63.30015916732239845 ) ) ;
#41778=DIRECTION ( 'NONE',  ( -0.9660698163281070672, -0.2582810677919976095, 5.363434502754640132E-08 ) ) ;
#41780=VECTOR ( 'NONE', #32050, 1000.000000000000114 ) ;
#41781=CARTESIAN_POINT ( 'NONE',  ( -21.95523322170430092, -8.895446802377390938, 66.77654591769551473 ) ) ;
#41782=ORIENTED_EDGE ( 'NONE', *, *, #14808, .T. ) ;
#41783=ORIENTED_EDGE ( 'NONE', *, *, #30783, .T. ) ;
#41786=CARTESIAN_POINT ( 'NONE',  ( -23.30963478160716562, -18.69084381296369557, 69.30844128244088154 ) ) ;
#41788=CARTESIAN_POINT ( 'NONE',  ( -21.18842005097459591, -20.71103373205295028, 69.05450136001277883 ) ) ;
#41789=CARTESIAN_POINT ( 'NONE',  ( -23.46741973463711872, -19.16603908095663655, 62.53902270128352825 ) ) ;
#41790=EDGE_CURVE ( 'NONE', #41056, #44086, #19632, .T. ) ;
#41791=CARTESIAN_POINT ( 'NONE',  ( -12.41310947992116098, -19.76871611099698001, 61.68206578716802113 ) ) ;
#41793=CARTESIAN_POINT ( 'NONE',  ( -22.56207008003183745, -19.63703213565221262, 72.92928497383269359 ) ) ;
#41794=ORIENTED_EDGE ( 'NONE', *, *, #23257, .T. ) ;
#41795=EDGE_LOOP ( 'NONE', ( #14839, #44717 ) ) ;
#41796=CARTESIAN_POINT ( 'NONE',  ( -12.26752988409003642, -16.72227946798956921, 54.07175714974876968 ) ) ;
#41797=ADVANCED_FACE ( 'NONE', ( #24893 ), #43934, .T. ) ;
#41799=CARTESIAN_POINT ( 'NONE',  ( -10.36816553299425792, -14.63937932467125691, 64.54370954096965818 ) ) ;
#41800=LINE ( 'NONE', #8081, #4801 ) ;
#41801=CARTESIAN_POINT ( 'NONE',  ( -23.30963478160716562, -18.69084381296369912, 69.30844128244088154 ) ) ;
#41802=ORIENTED_EDGE ( 'NONE', *, *, #8824, .T. ) ;
#41804=EDGE_CURVE ( 'NONE', #9176, #45877, #6108, .T. ) ;
#41806=VECTOR ( 'NONE', #6781, 1000.000000000000114 ) ;
#41807=CARTESIAN_POINT ( 'NONE',  ( -16.05912236108952129, -21.67647341356571999, 58.47512757527289295 ) ) ;
#41808=CARTESIAN_POINT ( 'NONE',  ( -12.32278866559117780, -19.67576434477648917, 61.41150688479135766 ) ) ;
#41809=EDGE_CURVE ( 'NONE', #22777, #45931, #36663, .T. ) ;
#41811=CARTESIAN_POINT ( 'NONE',  ( -15.17058439935471092, -21.43790227555238559, 68.64763166194532573 ) ) ;
#41812=EDGE_CURVE ( 'NONE', #5311, #44029, #48563, .T. ) ;
#41813=( BOUNDED_CURVE ( )  B_SPLINE_CURVE ( 3, ( #8027, #7775, #1095, #4315 ),
 .UNSPECIFIED., .F., .F. ) 
 B_SPLINE_CURVE_WITH_KNOTS ( ( 4, 4 ),
 ( 0.000000000000000000, 0.4074455897393656212 ),
 .UNSPECIFIED. ) 
 CURVE ( )  GEOMETRIC_REPRESENTATION_ITEM ( )  RATIONAL_B_SPLINE_CURVE ( ( 1.000000000000000000, 0.4567392136813327452, 0.3561768502900305999, 0.6983129098260936196 ) ) 
 REPRESENTATION_ITEM ( '' )  );
#41814=ORIENTED_EDGE ( 'NONE', *, *, #24280, .F. ) ;
#41816=CARTESIAN_POINT ( 'NONE',  ( -10.66703363856100317, -12.79807828486586629, 64.26836111018113229 ) ) ;
#41817=CARTESIAN_POINT ( 'NONE',  ( -22.81479297205375190, -19.95148388737573697, 72.74376929014212578 ) ) ;
#41820=CARTESIAN_POINT ( 'NONE',  ( -10.61708496520324552, -12.96040230030987850, 71.30008833185628703 ) ) ;
#41821=DIRECTION ( 'NONE',  ( 9.632611942272803284E-07, -3.816342176806251797E-07, -0.9999999999994633182 ) ) ;
#41823=ORIENTED_EDGE ( 'NONE', *, *, #46096, .T. ) ;
#41825=( BOUNDED_CURVE ( )  B_SPLINE_CURVE ( 3, ( #29338, #2980, #25634, #48284 ),
 .UNSPECIFIED., .F., .F. ) 
 B_SPLINE_CURVE_WITH_KNOTS ( ( 4, 4 ),
 ( 0.5000000000000000000, 0.9074455897393705062 ),
 .UNSPECIFIED. ) 
 CURVE ( )  GEOMETRIC_REPRESENTATION_ITEM ( )  RATIONAL_B_SPLINE_CURVE ( ( 1.000000000000006883, 0.4567392136813273606, 0.3561768502900237721, 0.6983129098261032786 ) ) 
 REPRESENTATION_ITEM ( '' )  );
#41826=ORIENTED_EDGE ( 'NONE', *, *, #43935, .F. ) ;
#41827=CARTESIAN_POINT ( 'NONE',  ( -10.48742572850251520, -13.50628733207679666, 71.36395466173868840 ) ) ;
#41828=FACE_OUTER_BOUND ( 'NONE', #6897, .T. ) ;
#41829=ORIENTED_EDGE ( 'NONE', *, *, #39131, .T. ) ;
#41834=VERTEX_POINT ( 'NONE', #14490 ) ;
#41835=CARTESIAN_POINT ( 'NONE',  ( -17.87628565292757088, -21.84483846147477237, 61.88095697920203264 ) ) ;
#41837=CARTESIAN_POINT ( 'NONE',  ( -11.42391642618174785, -11.20395052909733735, 57.40006283751519334 ) ) ;
#41838=ORIENTED_EDGE ( 'NONE', *, *, #405, .F. ) ;
#41839=CARTESIAN_POINT ( 'NONE',  ( -22.68646480449111635, -20.08284195570847430, 69.35913425646373298 ) ) ;
#41840=CARTESIAN_POINT ( 'NONE',  ( -21.78913961794832588, -8.771810275399618106, 70.24637145832762997 ) ) ;
#41842=ORIENTED_EDGE ( 'NONE', *, *, #11665, .F. ) ;
#41843=VERTEX_POINT ( 'NONE', #3201 ) ;
#41845=CARTESIAN_POINT ( 'NONE',  ( -10.48742572850251520, -13.50628733207679666, 71.36395466173868840 ) ) ;
#41846=CARTESIAN_POINT ( 'NONE',  ( -10.78031428196279329, -11.32923628920978310, 53.49999999999994316 ) ) ;
#41848=CARTESIAN_POINT ( 'NONE',  ( -20.38078961538757028, -7.970959937923086436, 70.50746246719650401 ) ) ;
#41850=CARTESIAN_POINT ( 'NONE',  ( -12.10905746339987132, -9.588700880036457264, 57.28209702652397795 ) ) ;
#41851=CARTESIAN_POINT ( 'NONE',  ( -17.59331746331979929, -7.761237803891376963, 63.55057029381061540 ) ) ;
#41852=CARTESIAN_POINT ( 'NONE',  ( -9.975186738464962843, -14.94398050308648784, 74.97495774971199012 ) ) ;
#41854=DIRECTION ( 'NONE',  ( -0.9577883914167873991, -0.2682351919075509628, 0.1033986416233889233 ) ) ;
#41855=CARTESIAN_POINT ( 'NONE',  ( -24.53780051168580911, -12.59584816521350348, 69.95738404390658616 ) ) ;
#41856=CARTESIAN_POINT ( 'NONE',  ( -14.87949561415316424, -21.38794988972642841, 65.40596695917321313 ) ) ;
#41858=ORIENTED_EDGE ( 'NONE', *, *, #6993, .T. ) ;
#41862=CARTESIAN_POINT ( 'NONE',  ( -13.33790141638613314, -21.03862562311502060, 61.71635090507787424 ) ) ;
#41863=CARTESIAN_POINT ( 'NONE',  ( -10.17814040529963826, -13.07751228953917533, 71.40839792250820039 ) ) ;
#41864=ADVANCED_FACE ( 'NONE', ( #3693 ), #17959, .T. ) ;
#41865=ORIENTED_EDGE ( 'NONE', *, *, #26076, .F. ) ;
#41866=CARTESIAN_POINT ( 'NONE',  ( -10.52991701743181174, -16.02177613136639067, 67.97767831076122036 ) ) ;
#41867=( BOUNDED_CURVE ( )  B_SPLINE_CURVE ( 3, ( #32881, #13680, #32655, #31935 ),
 .UNSPECIFIED., .F., .F. ) 
 B_SPLINE_CURVE_WITH_KNOTS ( ( 4, 4 ),
 ( 0.5000000000000000000, 0.9074455897393652881 ),
 .UNSPECIFIED. ) 
 CURVE ( )  GEOMETRIC_REPRESENTATION_ITEM ( )  RATIONAL_B_SPLINE_CURVE ( ( 1.000000000000018430, 0.4567392136813394066, 0.3561768502900201638, 0.6983129098260804080 ) ) 
 REPRESENTATION_ITEM ( '' )  );
#41868=EDGE_CURVE ( 'NONE', #31985, #31794, #12013, .T. ) ;
#41870=VERTEX_POINT ( 'NONE', #29546 ) ;
#41871=CARTESIAN_POINT ( 'NONE',  ( -10.90187802848681109, -12.12302927398623353, 74.55840406006809928 ) ) ;
#41873=B_SPLINE_CURVE_WITH_KNOTS ( 'NONE', 1,
 ( #1021, #30102 ),
 .UNSPECIFIED., .F., .F.,
 ( 2, 2 ),
 ( 0.000000000000000000, 1.000000000000000000 ),
 .UNSPECIFIED. ) ;
#41874=CARTESIAN_POINT ( 'NONE',  ( -14.37051197998799523, -8.445983692038035784, 74.34387349308116200 ) ) ;
#41875=ORIENTED_EDGE ( 'NONE', *, *, #32677, .T. ) ;
#41876=CARTESIAN_POINT ( 'NONE',  ( -17.39761409878557785, -7.809256622337199971, 67.02039592144427615 ) ) ;
#41879=FACE_OUTER_BOUND ( 'NONE', #22112, .T. ) ;
#41880=CARTESIAN_POINT ( 'NONE',  ( -20.49047903802489756, -8.516432955688220119, 63.61121494929229669 ) ) ;
#41881=ORIENTED_EDGE ( 'NONE', *, *, #23888, .T. ) ;
#41882=CARTESIAN_POINT ( 'NONE',  ( -13.54792730259346456, -8.920061342218058797, 57.25495614889487683 ) ) ;
#41885=CARTESIAN_POINT ( 'NONE',  ( -21.40280876628366968, -21.10781420246748041, 69.25438953298345268 ) ) ;
#41886=CARTESIAN_POINT ( 'NONE',  ( -11.32522400900782067, -11.27219014254736074, 60.96413645226084554 ) ) ;
#41890=CARTESIAN_POINT ( 'NONE',  ( -23.44980260057078070, -18.46889688393208573, 72.76368236443251192 ) ) ;
#41891=CARTESIAN_POINT ( 'NONE',  ( -24.45577199812615632, -12.20047074031916168, 54.27966884056650088 ) ) ;
#41892=CARTESIAN_POINT ( 'NONE',  ( -24.18825283819140992, -13.00726010212983574, 63.05937419120780163 ) ) ;
#41893=ORIENTED_EDGE ( 'NONE', *, *, #20662, .T. ) ;
#41895=LINE ( 'NONE', #8172, #23581 ) ;
#41896=CARTESIAN_POINT ( 'NONE',  ( -14.53996353315453405, -7.939311612974331744, 60.43341030124493329 ) ) ;
#41897=ORIENTED_EDGE ( 'NONE', *, *, #22694, .T. ) ;
#41898=CARTESIAN_POINT ( 'NONE',  ( -15.34465393633500696, -21.54586957516256263, 68.86120835375241711 ) ) ;
#41900=LINE ( 'NONE', #19244, #27385 ) ;
#41902=CARTESIAN_POINT ( 'NONE',  ( -14.35241195940507808, -8.021096776717739019, 67.44630344931481147 ) ) ;
#41903=CARTESIAN_POINT ( 'NONE',  ( -24.28619334359350290, -16.42731978468327014, 59.13804568661029037 ) ) ;
#41904=CARTESIAN_POINT ( 'NONE',  ( -16.39155704513022016, -21.78318439201321866, 61.75568132354042916 ) ) ;
#41905=VERTEX_POINT ( 'NONE', #9 ) ;
#41907=CARTESIAN_POINT ( 'NONE',  ( -14.44842434502374573, -8.417926551829491899, 67.25975083404114230 ) ) ;
#41908=CARTESIAN_POINT ( 'NONE',  ( -10.51276550655336273, -13.39960300793130621, 71.41648339266447465 ) ) ;
#41910=CARTESIAN_POINT ( 'NONE',  ( -19.98813031515369332, -21.37641424997302053, 72.70478737316020101 ) ) ;
#41914=ORIENTED_EDGE ( 'NONE', *, *, #37911, .F. ) ;
#41917=CARTESIAN_POINT ( 'NONE',  ( -11.56806251476610115, -18.73522173559940995, 65.03234934376791898 ) ) ;
#41918=CARTESIAN_POINT ( 'NONE',  ( -10.02107422201081732, -13.96720754792729480, 57.56169656168945181 ) ) ;
#41919=B_SPLINE_CURVE_WITH_KNOTS ( 'NONE', 3,
 ( #41615, #15239, #11086, #37656, #34448, #37909, #30305, #41862, #14732, #22174 ),
 .UNSPECIFIED., .F., .F.,
 ( 4, 2, 2, 2, 4 ),
 ( 0.1272669073658578009, 0.2522669073463363332, 0.3772669073268148932, 0.5022669073072933976, 0.6272669072877719021 ),
 .UNSPECIFIED. ) ;
#41920=EDGE_CURVE ( 'NONE', #30823, #32996, #16701, .T. ) ;
#41921=CARTESIAN_POINT ( 'NONE',  ( -13.41559485503361948, -8.529420403834853559, 57.08472365561223683 ) ) ;
#41922=CARTESIAN_POINT ( 'NONE',  ( -16.16379449968008331, -22.15191876840708929, 58.47080954035841671 ) ) ;
#41923=AXIS2_PLACEMENT_3D ( 'NONE', #5789, #5552, #2075 ) ;
#41928=CARTESIAN_POINT ( 'NONE',  ( -17.61671342162341958, -7.361684265168443098, 63.65082775983518815 ) ) ;
#41931=CARTESIAN_POINT ( 'NONE',  ( -15.38465892218781050, -7.643789270862604290, 74.22985656858331538 ) ) ;
#41932=VERTEX_POINT ( 'NONE', #41613 ) ;
#41933=CARTESIAN_POINT ( 'NONE',  ( -22.92560359444879836, -19.23055950467793096, 62.49839992038752712 ) ) ;
#41934=CARTESIAN_POINT ( 'NONE',  ( -22.49057859776916857, -20.27125474133809391, 65.89760026996282249 ) ) ;
#41936=ORIENTED_EDGE ( 'NONE', *, *, #47454, .T. ) ;
#41937=CARTESIAN_POINT ( 'NONE',  ( -24.47217469393258327, -14.64471774706559515, 62.86296487297660462 ) ) ;
#41939=( BOUNDED_SURFACE ( )  B_SPLINE_SURFACE ( 3, 1, ( 
 ( #3978, #42314 ),
 ( #30989, #43033 ),
 ( #35395, #9311 ),
 ( #24329, #9072 ),
 ( #42797, #38851 ),
 ( #1673, #24581 ),
 ( #24086, #39088 ) ),
 .UNSPECIFIED., .T., .F., .F. ) 
 B_SPLINE_SURFACE_WITH_KNOTS ( ( 4, 3, 4 ),
 ( 2, 2 ),
 ( 0.000000000000000000, 0.5000000000000000000, 1.000000000000000000 ),
 ( 0.000000000000000000, 1.000000000000000000 ),
 .UNSPECIFIED. ) 
 GEOMETRIC_REPRESENTATION_ITEM ( )  RATIONAL_B_SPLINE_SURFACE ( (
 ( 1.000000000000000000, 1.000000000000000000),
 ( 0.3333333333333335369, 0.3333333333333330373),
 ( 0.3333333333333335369, 0.3333333333333330373),
 ( 1.000000000000000000, 1.000000000000000000),
 ( 0.3333333333333333703, 0.3333333333333333703),
 ( 0.3333333333333333703, 0.3333333333333333703),
 ( 1.000000000000000000, 1.000000000000000000) ) ) 
 REPRESENTATION_ITEM ( '' )  SURFACE ( )  );
#41940=EDGE_CURVE ( 'NONE', #2243, #21441, #32585, .T. ) ;
#41941=CARTESIAN_POINT ( 'NONE',  ( -14.52849927865251267, -21.67364703532615877, 58.30584490887105886 ) ) ;
#41942=FACE_OUTER_BOUND ( 'NONE', #17286, .T. ) ;
#41945=CARTESIAN_POINT ( 'NONE',  ( -16.06904265174829405, -7.890656434512189676, 63.82011029958098192 ) ) ;
#41946=EDGE_CURVE ( 'NONE', #44255, #3166, #39654, .T. ) ;
#41947=DIRECTION ( 'NONE',  ( -6.816999857788696862E-06, -9.113320819891793432E-06, -0.9999999999352379154 ) ) ;
#41953=ORIENTED_EDGE ( 'NONE', *, *, #5297, .F. ) ;
#41955=CARTESIAN_POINT ( 'NONE',  ( -11.03619655160677304, -10.97525948075760560, 60.80168914678925063 ) ) ;
#41957=CARTESIAN_POINT ( 'NONE',  ( -23.23616409499838653, -18.79948708312782557, 65.82389430043846801 ) ) ;
#41958=CARTESIAN_POINT ( 'NONE',  ( -12.79553473267226771, -20.06053405000708878, 68.52760710243867948 ) ) ;
#41960=( BOUNDED_SURFACE ( )  B_SPLINE_SURFACE ( 3, 1, ( 
 ( #32733, #2697 ),
 ( #33438, #48479 ),
 ( #47757, #6403 ),
 ( #11069, #10347 ),
 ( #21433, #40854 ),
 ( #30039, #44814 ),
 ( #37138, #14471 ) ),
 .UNSPECIFIED., .T., .F., .F. ) 
 B_SPLINE_SURFACE_WITH_KNOTS ( ( 4, 3, 4 ),
 ( 2, 2 ),
 ( 0.000000000000000000, 0.5000000000000000000, 1.000000000000000000 ),
 ( 0.000000000000000000, 1.000000000000000000 ),
 .UNSPECIFIED. ) 
 GEOMETRIC_REPRESENTATION_ITEM ( )  RATIONAL_B_SPLINE_SURFACE ( (
 ( 1.000000000000000000, 1.000000000000000000),
 ( 0.3333333333333335369, 0.3333333333333330373),
 ( 0.3333333333333335369, 0.3333333333333330373),
 ( 1.000000000000000000, 1.000000000000000000),
 ( 0.3333333333333333703, 0.3333333333333333703),
 ( 0.3333333333333333703, 0.3333333333333333703),
 ( 1.000000000000000000, 1.000000000000000000) ) ) 
 REPRESENTATION_ITEM ( '' )  SURFACE ( )  );
#41961=ORIENTED_EDGE ( 'NONE', *, *, #15106, .F. ) ;
#41962=( BOUNDED_CURVE ( )  B_SPLINE_CURVE ( 3, ( #2302, #5771, #20778, #17310 ),
 .UNSPECIFIED., .F., .F. ) 
 B_SPLINE_CURVE_WITH_KNOTS ( ( 4, 4 ),
 ( 0.9074455897393700621, 1.000000000000000000 ),
 .UNSPECIFIED. ) 
 CURVE ( )  GEOMETRIC_REPRESENTATION_ITEM ( )  RATIONAL_B_SPLINE_CURVE ( ( 0.6983129098261124934, 0.7760317562607149666, 0.8765941196520108392, 1.000000000000000000 ) ) 
 REPRESENTATION_ITEM ( '' )  );
#41963=CARTESIAN_POINT ( 'NONE',  ( -14.78754745127378456, -8.270772244812135909, 60.61996282000563241 ) ) ;
#41964=CARTESIAN_POINT ( 'NONE',  ( -24.42401755266412522, -14.76532053153747448, 59.52834928196978126 ) ) ;
#41965=CARTESIAN_POINT ( 'NONE',  ( -24.02253934063158880, -11.35034036425029136, 66.61552819682387394 ) ) ;
#41966=B_SPLINE_CURVE_WITH_KNOTS ( 'NONE', 1,
 ( #31860, #17787 ),
 .UNSPECIFIED., .F., .F.,
 ( 2, 2 ),
 ( 0.000000000000000000, 1.000000000000000000 ),
 .UNSPECIFIED. ) ;
#41967=VERTEX_POINT ( 'NONE', #15479 ) ;
#41971=CARTESIAN_POINT ( 'NONE',  ( -10.00731251637046881, -14.10555026099538978, 61.10316585833331260 ) ) ;
#41972=DIRECTION ( 'NONE',  ( -0.9986807914369958405, 0.05134858142905002198, -1.286972153835537669E-09 ) ) ;
#41973=CARTESIAN_POINT ( 'NONE',  ( -23.16941533403626607, -18.80811654971253688, 62.46292810888792957 ) ) ;
#41974=( BOUNDED_CURVE ( )  B_SPLINE_CURVE ( 3, ( #7912, #34218, #505, #15748 ),
 .UNSPECIFIED., .F., .F. ) 
 B_SPLINE_CURVE_WITH_KNOTS ( ( 4, 4 ),
 ( 0.000000000000000000, 0.4074455897393670645 ),
 .UNSPECIFIED. ) 
 CURVE ( )  GEOMETRIC_REPRESENTATION_ITEM ( )  RATIONAL_B_SPLINE_CURVE ( ( 1.000000000000000000, 0.4567392136813321346, 0.3561768502900303779, 0.6983129098260947298 ) ) 
 REPRESENTATION_ITEM ( '' )  );
#41979=CARTESIAN_POINT ( 'NONE',  ( -21.06702863216100496, -20.84540773593990792, 65.86981821684420879 ) ) ;
#41980=CARTESIAN_POINT ( 'NONE',  ( -20.38154718419116662, -8.406214666052791884, 70.66588945595221105 ) ) ;
#41982=CARTESIAN_POINT ( 'NONE',  ( -17.84905175390062837, -22.24782703323402444, 58.51898120184483076 ) ) ;
#41983=CARTESIAN_POINT ( 'NONE',  ( -20.54394416162392289, -8.483752705004535599, 59.72636470710568091 ) ) ;
#41985=CARTESIAN_POINT ( 'NONE',  ( -9.976559278833523337, -14.59036342035520306, 67.97144843379662404 ) ) ;
#41986=CARTESIAN_POINT ( 'NONE',  ( -24.78881009142557090, -15.93819564886128148, 66.17669525438618905 ) ) ;
#41988=CARTESIAN_POINT ( 'NONE',  ( -24.05420634179087358, -17.20676946999824608, 69.69867738674849988 ) ) ;
#41990=ORIENTED_EDGE ( 'NONE', *, *, #32703, .F. ) ;
#41991=CARTESIAN_POINT ( 'NONE',  ( -22.22371030936713510, -9.111184089457765367, 59.90666523727240644 ) ) ;
#41992=DIRECTION ( 'NONE',  ( -0.9848822020395749943, 0.1732254256905498002, 7.367703375004543066E-08 ) ) ;
#41993=DIRECTION ( 'NONE',  ( -3.549360974554993999E-17, 6.371834667797928663E-18, 1.000000000000000000 ) ) ;
#41994=AXIS2_PLACEMENT_3D ( 'NONE', #13148, #28195, #9245 ) ;
#41995=EDGE_LOOP ( 'NONE', ( #4456, #29290 ) ) ;
#41996=CARTESIAN_POINT ( 'NONE',  ( -10.69985271022639317, -16.93744915505940085, 61.57231810286263141 ) ) ;
#41997=CARTESIAN_POINT ( 'NONE',  ( -14.60479643987598841, -7.913168514039711887, 60.50491717424539218 ) ) ;
#41998=CARTESIAN_POINT ( 'NONE',  ( -14.74690658000796439, -21.27702444416618732, 58.16617884968206198 ) ) ;
#41999=CARTESIAN_POINT ( 'NONE',  ( -24.49036105318029755, -17.16975618249231061, 73.00523289078640232 ) ) ;
#42002=CARTESIAN_POINT ( 'NONE',  ( -17.78619188034219079, -22.25052443322864448, 58.52740643916145302 ) ) ;
#42004=FACE_BOUND ( 'NONE', #11051, .T. ) ;
#42007=EDGE_CURVE ( 'NONE', #27678, #22721, #45806, .T. ) ;
#42008=LINE ( 'NONE', #38283, #32886 ) ;
#42009=CARTESIAN_POINT ( 'NONE',  ( -19.11145865927415954, -7.964113456900453691, 63.43089235103782642 ) ) ;
#42011=FACE_OUTER_BOUND ( 'NONE', #32833, .T. ) ;
#42013=CARTESIAN_POINT ( 'NONE',  ( -12.08002995027803372, -10.28786569443740717, 67.49896886176594535 ) ) ;
#42015=CARTESIAN_POINT ( 'NONE',  ( -11.45751978572037011, -19.27057081285444085, 71.87181161472111057 ) ) ;
#42016=CARTESIAN_POINT ( 'NONE',  ( -22.96794631393402142, -10.53327243508824473, 63.14356316969981009 ) ) ;
#42017=ORIENTED_EDGE ( 'NONE', *, *, #37351, .F. ) ;
#42018=ADVANCED_FACE ( 'NONE', ( #4671 ), #15974, .T. ) ;
#42019=ADVANCED_FACE ( 'NONE', ( #12058 ), #34702, .T. ) ;
#42020=CARTESIAN_POINT ( 'NONE',  ( -12.74662852849665207, -9.010439419175657605, 70.97208472523765010 ) ) ;
#42021=ORIENTED_EDGE ( 'NONE', *, *, #13321, .F. ) ;
#42022=ORIENTED_EDGE ( 'NONE', *, *, #41319, .F. ) ;
#42023=ORIENTED_EDGE ( 'NONE', *, *, #47009, .T. ) ;
#42025=DIRECTION ( 'NONE',  ( 0.8394943004421987487, -0.3114503813636534946, 0.4452504682462423702 ) ) ;
#42026=CARTESIAN_POINT ( 'NONE',  ( -24.16171209271585596, -12.91020206353950250, 66.60246698658390585 ) ) ;
#42027=CARTESIAN_POINT ( 'NONE',  ( -11.81148223110008821, -9.909859460634582007, 64.18947707955818771 ) ) ;
#42031=VECTOR ( 'NONE', #4293, 1000.000000000000114 ) ;
#42032=CARTESIAN_POINT ( 'NONE',  ( -19.50843993236927432, -21.96177808838975665, 62.11008241541560437 ) ) ;
#42033=ADVANCED_FACE ( 'NONE', ( #23640 ), #8364, .F. ) ;
#42035=CARTESIAN_POINT ( 'NONE',  ( -10.40687472791218049, -14.09964931664121579, 64.80292589203708076 ) ) ;
#42037=CARTESIAN_POINT ( 'NONE',  ( -19.67335841558337961, -21.43805762741428111, 65.75020853001484511 ) ) ;
#42038=ORIENTED_EDGE ( 'NONE', *, *, #16823, .T. ) ;
#42041=CARTESIAN_POINT ( 'NONE',  ( -21.57995947450667984, -9.113990939708573435, 70.14604673427196246 ) ) ;
#42044=( BOUNDED_CURVE ( )  B_SPLINE_CURVE ( 3, ( #12641, #47361, #31843, #43170 ),
 .UNSPECIFIED., .F., .F. ) 
 B_SPLINE_CURVE_WITH_KNOTS ( ( 4, 4 ),
 ( 0.000000000000000000, 0.4074455897393667314 ),
 .UNSPECIFIED. ) 
 CURVE ( )  GEOMETRIC_REPRESENTATION_ITEM ( )  RATIONAL_B_SPLINE_CURVE ( ( 1.000000000000000000, 0.4567392136813263059, 0.3561768502900282130, 0.6983129098261057210 ) ) 
 REPRESENTATION_ITEM ( '' )  );
#42045=B_SPLINE_CURVE_WITH_KNOTS ( 'NONE', 3,
 ( #28122, #1057, #45884, #27880, #12139, #23959, #38471, #4755, #16054, #15819 ),
 .UNSPECIFIED., .F., .F.,
 ( 4, 2, 2, 2, 4 ),
 ( 0.000000000000000000, 0.2500000000000000000, 0.5000000000000000000, 0.7500000000000000000, 1.000000000000000000 ),
 .UNSPECIFIED. ) ;
#42046=EDGE_LOOP ( 'NONE', ( #24051, #25859 ) ) ;
#42047=DIRECTION ( 'NONE',  ( -0.2196488028684550897, -0.9755790093059856227, 7.835600157697874713E-08 ) ) ;
#42048=B_SPLINE_CURVE_WITH_KNOTS ( 'NONE', 1,
 ( #19687, #45077 ),
 .UNSPECIFIED., .F., .F.,
 ( 2, 2 ),
 ( 0.000000000000000000, 1.000000000000000000 ),
 .UNSPECIFIED. ) ;
#42049=CARTESIAN_POINT ( 'NONE',  ( -11.83425018566923370, -19.11833757169930692, 68.37256453262955347 ) ) ;
#42050=CARTESIAN_POINT ( 'NONE',  ( -12.55788482626217650, -9.703832430577184809, 57.50424130074089391 ) ) ;
#42053=CARTESIAN_POINT ( 'NONE',  ( -17.19167086870822203, -7.760035283349824731, 66.90551000485606892 ) ) ;
#42055=VERTEX_POINT ( 'NONE', #16209 ) ;
#42056=CARTESIAN_POINT ( 'NONE',  ( -10.00747133761319141, -14.10395761772617362, 60.96175355949325336 ) ) ;
#42057=ORIENTED_EDGE ( 'NONE', *, *, #19176, .T. ) ;
#42059=CARTESIAN_POINT ( 'NONE',  ( -23.45029294355628480, -11.15024590387849557, 73.66193277021260144 ) ) ;
#42060=CARTESIAN_POINT ( 'NONE',  ( -22.02664077354800654, -9.468686367811812943, 59.72730992479275614 ) ) ;
#42063=CARTESIAN_POINT ( 'NONE',  ( -16.32745258320347759, -21.77369344365219561, 61.77040269689842944 ) ) ;
#42067=VERTEX_POINT ( 'NONE', #46995 ) ;
#42068=CARTESIAN_POINT ( 'NONE',  ( -22.12470610600313137, -9.029191726191170275, 63.36966517759014295 ) ) ;
#42070=DIRECTION ( 'NONE',  ( 0.9789991564298999860, 0.2038642972899921690, -4.410747590293462207E-08 ) ) ;
#42071=CARTESIAN_POINT ( 'NONE',  ( -10.95381465013825206, -17.48043978162002077, 68.39721944380028162 ) ) ;
#42072=VERTEX_POINT ( 'NONE', #39850 ) ;
#42074=EDGE_CURVE ( 'NONE', #3341, #47047, #34316, .T. ) ;
#42075=CARTESIAN_POINT ( 'NONE',  ( -23.32804039107871574, -19.35299860258280447, 59.08399415320680959 ) ) ;
#42076=VERTEX_POINT ( 'NONE', #13493 ) ;
#42079=CARTESIAN_POINT ( 'NONE',  ( -24.84680101036319400, -14.17012173819833798, 69.81308644732062874 ) ) ;
#42080=CARTESIAN_POINT ( 'NONE',  ( -16.06904075904983031, -7.890656793283918446, 63.97011029956861705 ) ) ;
#42084=CARTESIAN_POINT ( 'NONE',  ( -24.82750207115152463, -13.97654542584719373, 73.30766806548945169 ) ) ;
#42086=CARTESIAN_POINT ( 'NONE',  ( -10.76785811675247118, -12.48515291162924434, 57.61385273545094066 ) ) ;
#42087=CARTESIAN_POINT ( 'NONE',  ( -10.56255612388957665, -16.44405857821975658, 71.65570096763067909 ) ) ;
#42088=ORIENTED_EDGE ( 'NONE', *, *, #39607, .F. ) ;
#42090=CARTESIAN_POINT ( 'NONE',  ( -13.88293403466071396, -20.90532716339074781, 68.60625136993937190 ) ) ;
#42091=EDGE_CURVE ( 'NONE', #13885, #4171, #45513, .T. ) ;
#42093=CARTESIAN_POINT ( 'NONE',  ( -20.88270717056239789, -21.40782548341276481, 58.82970473467946704 ) ) ;
#42094=B_SPLINE_CURVE_WITH_KNOTS ( 'NONE', 1,
 ( #43572, #9835 ),
 .UNSPECIFIED., .F., .F.,
 ( 2, 2 ),
 ( 0.000000000000000000, 1.000000000000000000 ),
 .UNSPECIFIED. ) ;
#42095=( BOUNDED_CURVE ( )  B_SPLINE_CURVE ( 3, ( #5749, #28626, #17528, #13817 ),
 .UNSPECIFIED., .F., .F. ) 
 B_SPLINE_CURVE_WITH_KNOTS ( ( 4, 4 ),
 ( 0.9074455897393666204, 1.000000000000000000 ),
 .UNSPECIFIED. ) 
 CURVE ( )  GEOMETRIC_REPRESENTATION_ITEM ( )  RATIONAL_B_SPLINE_CURVE ( ( 0.6983129098261068313, 0.7760317562607100816, 0.8765941196520078416, 1.000000000000000000 ) ) 
 REPRESENTATION_ITEM ( '' )  );
#42098=ORIENTED_EDGE ( 'NONE', *, *, #41390, .T. ) ;
#42099=DIRECTION ( 'NONE',  ( 0.9999889394985579383, 0.004703284017506803583, -7.734398264755851970E-09 ) ) ;
#42100=VECTOR ( 'NONE', #14769, 1000.000000000000227 ) ;
#42101=CARTESIAN_POINT ( 'NONE',  ( -23.78676244964941233, -10.93361294341921131, 73.54688584860882372 ) ) ;
#42102=DIRECTION ( 'NONE',  ( 0.4599824152910791941, 0.8879280250239793837, 2.250728352126283350E-08 ) ) ;
#42105=( BOUNDED_CURVE ( )  B_SPLINE_CURVE ( 3, ( #3100, #18108, #48164, #14395 ),
 .UNSPECIFIED., .F., .F. ) 
 B_SPLINE_CURVE_WITH_KNOTS ( ( 4, 4 ),
 ( 0.9074455897393750581, 1.000000000000000000 ),
 .UNSPECIFIED. ) 
 CURVE ( )  GEOMETRIC_REPRESENTATION_ITEM ( )  RATIONAL_B_SPLINE_CURVE ( ( 0.6983129098261150469, 0.7760317562607171871, 0.8765941196520121714, 1.000000000000000000 ) ) 
 REPRESENTATION_ITEM ( '' )  );
#42107=CARTESIAN_POINT ( 'NONE',  ( -24.80746943141735983, -15.80390768895026987, 69.57661537956182940 ) ) ;
#42109=CARTESIAN_POINT ( 'NONE',  ( -12.93275540070710505, -20.17844446062794717, 71.87941766543936239 ) ) ;
#42110=CARTESIAN_POINT ( 'NONE',  ( -22.20320178312271153, -19.92390373660361291, 65.70421731406698029 ) ) ;
#42112=ORIENTED_EDGE ( 'NONE', *, *, #12516, .F. ) ;
#42115=CARTESIAN_POINT ( 'NONE',  ( -17.26457240846633923, -7.760713630915982542, 70.50507891880883449 ) ) ;
#42118=CARTESIAN_POINT ( 'NONE',  ( -13.35685073114381716, -8.567315923767541364, 57.01321801328607108 ) ) ;
#42119=EDGE_CURVE ( 'NONE', #34596, #30663, #43836, .T. ) ;
#42122=CARTESIAN_POINT ( 'NONE',  ( -10.33431758219403207, -12.52035302217920254, 60.98348881056122650 ) ) ;
#42123=CARTESIAN_POINT ( 'NONE',  ( -19.10460565471617755, -7.550450307296652674, 63.54433857513910056 ) ) ;
#42124=B_SPLINE_CURVE_WITH_KNOTS ( 'NONE', 1,
 ( #12910, #24258 ),
 .UNSPECIFIED., .F., .F.,
 ( 2, 2 ),
 ( 0.000000000000000000, 1.000000000000000000 ),
 .UNSPECIFIED. ) ;
#42125=CARTESIAN_POINT ( 'NONE',  ( -15.22312280068192081, -21.51522583983519255, 61.79167741754957177 ) ) ;
#42126=ORIENTED_EDGE ( 'NONE', *, *, #12398, .T. ) ;
#42128=CARTESIAN_POINT ( 'NONE',  ( -13.06884191565359643, -20.85448943349606665, 58.23305466536662323 ) ) ;
#42132=CARTESIAN_POINT ( 'NONE',  ( -24.77723895724858494, -16.00713575449774595, 66.24820309305337673 ) ) ;
#42133=ORIENTED_EDGE ( 'NONE', *, *, #3673, .F. ) ;
#42135=EDGE_CURVE ( 'NONE', #27147, #7125, #43759, .T. ) ;
#42136=CARTESIAN_POINT ( 'NONE',  ( -14.25677688785123109, -8.066017148268395331, 67.40975083916667643 ) ) ;
#42137=CARTESIAN_POINT ( 'NONE',  ( -24.29232294273250758, -16.16103065725259214, 62.59328677063434299 ) ) ;
#42138=ORIENTED_EDGE ( 'NONE', *, *, #33351, .F. ) ;
#42139=CARTESIAN_POINT ( 'NONE',  ( -10.00117635412376593, -15.44487469174752903, 57.68297500625912733 ) ) ;
#42140=CARTESIAN_POINT ( 'NONE',  ( -15.81515823392193631, -7.534963144122849066, 67.24733145614881380 ) ) ;
#42143=CARTESIAN_POINT ( 'NONE',  ( -21.89130958583942288, -9.354787850460871468, 63.20625856529903075 ) ) ;
#42144=CARTESIAN_POINT ( 'NONE',  ( -14.36817892824948650, -8.455618309860652104, 67.54503025475185041 ) ) ;
#42146=CARTESIAN_POINT ( 'NONE',  ( -16.36796100389485176, -21.77969089362421684, 61.75568160946304630 ) ) ;
#42147=ORIENTED_EDGE ( 'NONE', *, *, #6369, .T. ) ;
#42149=EDGE_CURVE ( 'NONE', #45248, #14239, #31496, .T. ) ;
#42152=CARTESIAN_POINT ( 'NONE',  ( -11.01197672498281044, -17.74032467813711733, 71.85246142747087106 ) ) ;
#42154=CARTESIAN_POINT ( 'NONE',  ( -17.44318359119074913, -7.759083889314800864, 67.02599349837787202 ) ) ;
#42155=ADVANCED_FACE ( 'NONE', ( #39369 ), #121, .T. ) ;
#42156=CARTESIAN_POINT ( 'NONE',  ( -19.70639753248355319, -21.90109403227812379, 65.57990909513159750 ) ) ;
#42158=ORIENTED_EDGE ( 'NONE', *, *, #30237, .F. ) ;
#42160=ORIENTED_EDGE ( 'NONE', *, *, #31851, .F. ) ;
#42161=CARTESIAN_POINT ( 'NONE',  ( -11.21783104652298846, -18.93062367394879431, 64.93202350587574756 ) ) ;
#42162=CARTESIAN_POINT ( 'NONE',  ( -10.02995829593802668, -13.89786868041111667, 57.63320316755233819 ) ) ;
#42163=EDGE_LOOP ( 'NONE', ( #35348, #41442 ) ) ;
#42164=B_SPLINE_CURVE_WITH_KNOTS ( 'NONE', 3,
 ( #39879, #2691, #7322, #25350, #43594, #6153, #22322, #3606, #3867, #41523 ),
 .UNSPECIFIED., .F., .F.,
 ( 4, 2, 2, 2, 4 ),
 ( 0.1272669073658169447, 0.2522669073463095213, 0.3772669073268021256, 0.5022669073072946189, 0.6272669072877872232 ),
 .UNSPECIFIED. ) ;
#42165=CARTESIAN_POINT ( 'NONE',  ( -10.43726483381679415, -14.35454136775383382, 68.04727144194282573 ) ) ;
#42167=CARTESIAN_POINT ( 'NONE',  ( -15.84754116039521676, -7.934039430420517292, 63.87830746700826268 ) ) ;
#42168=DIRECTION ( 'NONE',  ( -5.731567514496413899E-31, -1.020425574103664789E-16, -1.000000000000000000 ) ) ;
#42169=EDGE_LOOP ( 'NONE', ( #41581, #12613 ) ) ;
#42170=CARTESIAN_POINT ( 'NONE',  ( -23.83080496556880945, -17.75212211224490133, 59.28906343887996400 ) ) ;
#42171=CARTESIAN_POINT ( 'NONE',  ( -23.86921235852081580, -8.358587496134095574, 54.49999999999995026 ) ) ;
#42172=ORIENTED_EDGE ( 'NONE', *, *, #23876, .F. ) ;
#42175=CARTESIAN_POINT ( 'NONE',  ( -23.76644255318129595, -11.73037447993928239, 62.95778050648025470 ) ) ;
#42176=ORIENTED_EDGE ( 'NONE', *, *, #16330, .T. ) ;
#42177=CARTESIAN_POINT ( 'NONE',  ( -11.10300703817161327, -10.86615712478015539, 57.39398594787093089 ) ) ;
#42178=CARTESIAN_POINT ( 'NONE',  ( -22.47920019561985328, -20.28188657713170073, 65.88234471252430069 ) ) ;
#42179=CARTESIAN_POINT ( 'NONE',  ( -15.53265176333180619, -21.60105060138385014, 72.33103357390284316 ) ) ;
#42180=VERTEX_POINT ( 'NONE', #17180 ) ;
#42181=CARTESIAN_POINT ( 'NONE',  ( -10.66703313327717417, -12.79807994555918782, 64.56836111017611302 ) ) ;
#42183=B_SPLINE_CURVE_WITH_KNOTS ( 'NONE', 1,
 ( #42086, #16688 ),
 .UNSPECIFIED., .F., .F.,
 ( 2, 2 ),
 ( 0.000000000000000000, 1.000000000000000000 ),
 .UNSPECIFIED. ) ;
#42184=CARTESIAN_POINT ( 'NONE',  ( -15.25351580106674376, -21.52054300433004386, 72.13755606438517987 ) ) ;
#42185=CARTESIAN_POINT ( 'NONE',  ( -21.24554520941113367, -21.20453976546471608, 65.76949229983627276 ) ) ;
#42186=CARTESIAN_POINT ( 'NONE',  ( -14.79922817013080483, -7.836842635312091687, 57.03495431467663224 ) ) ;
#42187=DIRECTION ( 'NONE',  ( -0.1922068328301544116, -0.9813544382196450755, 7.804899501296266931E-08 ) ) ;
#42188=CARTESIAN_POINT ( 'NONE',  ( -22.75539019595754908, -10.19575032747719412, 66.82710158566565894 ) ) ;
#42189=CARTESIAN_POINT ( 'NONE',  ( -20.88397215374023119, -20.89444276828103142, 62.40006029053370895 ) ) ;
#42192=ORIENTED_EDGE ( 'NONE', *, *, #227, .T. ) ;
#42193=EDGE_CURVE ( 'NONE', #1317, #20133, #18436, .T. ) ;
#42194=DIRECTION ( 'NONE',  ( 0.1675476790616295675, -0.9858639740050658684, 1.222863418168464292E-17 ) ) ;
#42195=CARTESIAN_POINT ( 'NONE',  ( -10.47120130798260185, -17.48512196787819661, 64.73401085767241625 ) ) ;
#42201=CARTESIAN_POINT ( 'NONE',  ( -18.46885980906216318, -22.18634193242058572, 68.92859349268570668 ) ) ;
#42203=DIRECTION ( 'NONE',  ( 0.5327540375067998379, 0.8462701315302333382, 7.203825861310634525E-08 ) ) ;
#42206=CARTESIAN_POINT ( 'NONE',  ( -10.08886380456056742, -16.11191617737164705, 68.07744192415786699 ) ) ;
#42208=CARTESIAN_POINT ( 'NONE',  ( -15.62222905942471840, -7.993050613273783966, 70.89517703929612935 ) ) ;
#42210=CARTESIAN_POINT ( 'NONE',  ( -12.86542566280920319, -8.916737054783007821, 67.47919149430154562 ) ) ;
#42211=CARTESIAN_POINT ( 'NONE',  ( -10.37560970945560967, -14.44337087574636769, 61.07388280500082800 ) ) ;
#42214=ORIENTED_EDGE ( 'NONE', *, *, #21074, .F. ) ;
#42215=ORIENTED_EDGE ( 'NONE', *, *, #30180, .F. ) ;
#42217=CARTESIAN_POINT ( 'NONE',  ( -14.07539642552819359, -8.605278304397881328, 74.19954655214911554 ) ) ;
#42218=CARTESIAN_POINT ( 'NONE',  ( -23.34080049944153856, -11.06854047984963962, 73.55296409646045674 ) ) ;
#42219=DIRECTION ( 'NONE',  ( -0.1738928961406289164, 0.9847645711904029486, 7.871847295470929299E-08 ) ) ;
#42220=EDGE_CURVE ( 'NONE', #34559, #44694, #4863, .T. ) ;
#42221=EDGE_CURVE ( 'NONE', #43276, #31666, #23798, .T. ) ;
#42222=B_SPLINE_CURVE_WITH_KNOTS ( 'NONE', 1,
 ( #33409, #19830 ),
 .UNSPECIFIED., .F., .F.,
 ( 2, 2 ),
 ( 0.000000000000000000, 1.000000000000000000 ),
 .UNSPECIFIED. ) ;
#42223=CARTESIAN_POINT ( 'NONE',  ( -17.39128687056474121, -21.86710222072322907, 58.54986106076864161 ) ) ;
#42225=CARTESIAN_POINT ( 'NONE',  ( -20.88289085685542545, -8.210692395643533814, 59.88479313977884289 ) ) ;
#42227=CARTESIAN_POINT ( 'NONE',  ( -11.60526899143904345, -18.79015832504765626, 68.23161775275829655 ) ) ;
#42228=( BOUNDED_CURVE ( )  B_SPLINE_CURVE ( 3, ( #43533, #44498, #39818, #32898 ),
 .UNSPECIFIED., .F., .F. ) 
 B_SPLINE_CURVE_WITH_KNOTS ( ( 4, 4 ),
 ( 0.4074455897393627901, 0.5000000000000000000 ),
 .UNSPECIFIED. ) 
 CURVE ( )  GEOMETRIC_REPRESENTATION_ITEM ( )  RATIONAL_B_SPLINE_CURVE ( ( 0.6983129098260937306, 0.7760317562606900976, 0.8765941196519897449, 0.9999999999999861222 ) ) 
 REPRESENTATION_ITEM ( '' )  );
#42229=ORIENTED_EDGE ( 'NONE', *, *, #39961, .F. ) ;
#42230=CARTESIAN_POINT ( 'NONE',  ( -24.41687585628244506, -14.48898472626409273, 66.18292730085975961 ) ) ;
#42231=DIRECTION ( 'NONE',  ( 0.4182840851231335866, -0.9083162577718748576, 8.112345261759808545E-09 ) ) ;
#42234=ORIENTED_EDGE ( 'NONE', *, *, #35518, .T. ) ;
#42235=CARTESIAN_POINT ( 'NONE',  ( -13.30482829320324534, -21.01685844473519182, 61.62372190405099559 ) ) ;
#42236=CARTESIAN_POINT ( 'NONE',  ( -9.974527725170556636, -14.89026794202819204, 74.99790105621293890 ) ) ;
#42238=CARTESIAN_POINT ( 'NONE',  ( -18.13127753087942295, -22.22561600718755770, 65.53870465771630904 ) ) ;
#42239=VERTEX_POINT ( 'NONE', #7101 ) ;
#42240=B_SPLINE_CURVE_WITH_KNOTS ( 'NONE', 1,
 ( #35839, #2124 ),
 .UNSPECIFIED., .F., .F.,
 ( 2, 2 ),
 ( 0.000000000000000000, 1.000000000000000000 ),
 .UNSPECIFIED. ) ;
#42241=CARTESIAN_POINT ( 'NONE',  ( -10.00824906877580567, -15.52305002423542390, 57.68980053291110721 ) ) ;
#42242=AXIS2_PLACEMENT_3D ( 'NONE', #46665, #12677, #12912 ) ;
#42243=CARTESIAN_POINT ( 'NONE',  ( -15.11795752579537400, -21.47139868945932051, 65.40596679997382523 ) ) ;
#42244=CARTESIAN_POINT ( 'NONE',  ( -15.11195812866605692, -21.41632606413040918, 65.10596681519622564 ) ) ;
#42246=CARTESIAN_POINT ( 'NONE',  ( -21.57940561823839332, -9.104090476609597360, 63.34720799502051847 ) ) ;
#42247=FACE_OUTER_BOUND ( 'NONE', #11066, .T. ) ;
#42248=( BOUNDED_CURVE ( )  B_SPLINE_CURVE ( 3, ( #41327, #27282, #4633, #18923 ),
 .UNSPECIFIED., .F., .F. ) 
 B_SPLINE_CURVE_WITH_KNOTS ( ( 4, 4 ),
 ( 0.4074455897269660953, 0.5000000000000000000 ),
 .UNSPECIFIED. ) 
 CURVE ( )  GEOMETRIC_REPRESENTATION_ITEM ( )  RATIONAL_B_SPLINE_CURVE ( ( 0.6983129097948570507, 0.7760317562337696318, 0.8765941196354886111, 1.000000000000025535 ) ) 
 REPRESENTATION_ITEM ( '' )  );
#42252=CARTESIAN_POINT ( 'NONE',  ( -11.44438386955935272, -18.44830926459003351, 57.91600554991716621 ) ) ;
#42256=CARTESIAN_POINT ( 'NONE',  ( -24.35389707626741185, -16.10709931453380861, 62.87856533165624029 ) ) ;
#42257=ORIENTED_EDGE ( 'NONE', *, *, #35715, .F. ) ;
#42258=CARTESIAN_POINT ( 'NONE',  ( -11.49911252271374273, -19.32675654123934095, 71.80030491464860631 ) ) ;
#42259=CARTESIAN_POINT ( 'NONE',  ( -16.71219879347879100, -22.22520166962337740, 68.81065243885818461 ) ) ;
#42260=VERTEX_POINT ( 'NONE', #7351 ) ;
#42261=B_SPLINE_CURVE_WITH_KNOTS ( 'NONE', 1,
 ( #21359, #44256 ),
 .UNSPECIFIED., .F., .F.,
 ( 2, 2 ),
 ( 0.000000000000000000, 1.000000000000000000 ),
 .UNSPECIFIED. ) ;
#42263=( BOUNDED_CURVE ( )  B_SPLINE_CURVE ( 3, ( #47080, #17263, #47331, #16779 ),
 .UNSPECIFIED., .F., .F. ) 
 B_SPLINE_CURVE_WITH_KNOTS ( ( 4, 4 ),
 ( 0.4074455897393777226, 0.5000000000000000000 ),
 .UNSPECIFIED. ) 
 CURVE ( )  GEOMETRIC_REPRESENTATION_ITEM ( )  RATIONAL_B_SPLINE_CURVE ( ( 0.6983129098261363632, 0.7760317562607240705, 0.8765941196520085077, 0.9999999999999816813 ) ) 
 REPRESENTATION_ITEM ( '' )  );
#42264=ADVANCED_FACE ( 'NONE', ( #22349 ), #6844, .T. ) ;
#42265=ORIENTED_EDGE ( 'NONE', *, *, #37906, .F. ) ;
#42268=CARTESIAN_POINT ( 'NONE',  ( -10.03035355355731006, -15.72374577095404824, 61.22284339518546403 ) ) ;
#42269=CARTESIAN_POINT ( 'NONE',  ( -18.50931870666621037, -21.77518001355031529, 72.28510940651260341 ) ) ;
#42271=CARTESIAN_POINT ( 'NONE',  ( -21.30258078786002329, -8.981766571127032250, 73.90128699495393505 ) ) ;
#42272=CARTESIAN_POINT ( 'NONE',  ( -10.25351306168449383, -12.78524163461458762, 64.38180785400611228 ) ) ;
#42273=CARTESIAN_POINT ( 'NONE',  ( -12.49693318139922482, -20.39741725237024284, 71.94620299007212338 ) ) ;
#42278=CARTESIAN_POINT ( 'NONE',  ( -19.80301260837064703, -21.44571507605098404, 69.23482476707422961 ) ) ;
#42279=DIRECTION ( 'NONE',  ( 5.329554274754248866E-07, 1.313503380136696700E-06, 0.9999999999989952482 ) ) ;
#42280=VECTOR ( 'NONE', #45053, 1000.000000000000000 ) ;
#42281=CARTESIAN_POINT ( 'NONE',  ( -14.86627107493491984, -7.811969877679347363, 56.96504568426624360 ) ) ;
#42282=EDGE_LOOP ( 'NONE', ( #39271, #8777, #2096, #21997, #25453 ) ) ;
#42284=EDGE_CURVE ( 'NONE', #27092, #46437, #22039, .T. ) ;
#42285=EDGE_LOOP ( 'NONE', ( #23895, #39359, #33462, #20493, #5957 ) ) ;
#42286=EDGE_CURVE ( 'NONE', #3865, #34178, #45139, .T. ) ;
#42287=ADVANCED_FACE ( 'NONE', ( #18638 ), #20229, .T. ) ;
#42288=CARTESIAN_POINT ( 'NONE',  ( -21.52726260838264949, -9.076274878514672295, 70.13132538915753855 ) ) ;
#42289=CARTESIAN_POINT ( 'NONE',  ( -17.32045713178291280, -7.809913985087237442, 67.03542077588672043 ) ) ;
#42290=VERTEX_POINT ( 'NONE', #45029 ) ;
#42292=CARTESIAN_POINT ( 'NONE',  ( -10.76216126260078987, -17.12512740823429525, 65.04228012599854480 ) ) ;
#42293=CARTESIAN_POINT ( 'NONE',  ( -12.64905295888074299, -9.611711778639854487, 57.23368232919959553 ) ) ;
#42294=APPLICATION_CONTEXT ( 'automotive_design' ) ;
#42296=AXIS2_PLACEMENT_3D ( 'NONE', #10850, #47564, #13796 ) ;
#42297=CARTESIAN_POINT ( 'NONE',  ( -15.97587070454731517, -21.71254611733878193, 58.37765857771692879 ) ) ;
#42299=VERTEX_POINT ( 'NONE', #38577 ) ;
#42303=EDGE_LOOP ( 'NONE', ( #34750, #38291, #34689, #2199, #44985 ) ) ;
#42304=CARTESIAN_POINT ( 'NONE',  ( -14.99706723701585354, -21.85287888328288375, 65.29092001793476641 ) ) ;
#42308=CARTESIAN_POINT ( 'NONE',  ( -23.84761965343929901, -12.02338239010575194, 59.59308729769960422 ) ) ;
#42309=ADVANCED_FACE ( 'NONE', ( #30965 ), #22596, .T. ) ;
#42311=ORIENTED_EDGE ( 'NONE', *, *, #20396, .F. ) ;
#42312=CARTESIAN_POINT ( 'NONE',  ( -10.84896266223257122, -17.37486770053218521, 71.71150890757306229 ) ) ;
#42314=CARTESIAN_POINT ( 'NONE',  ( -20.88270717056239789, -21.40782548341276481, 58.82970473467946704 ) ) ;
#42315=CARTESIAN_POINT ( 'NONE',  ( -10.92393577332946641, -17.40806695695071227, 68.38105336835567982 ) ) ;
#42319=B_SPLINE_CURVE_WITH_KNOTS ( 'NONE', 3,
 ( #32477, #35905, #24370, #6127, #13731, #17677, #17915, #40343, #32240, #6374 ),
 .UNSPECIFIED., .F., .F.,
 ( 4, 2, 2, 2, 4 ),
 ( 0.000000000000000000, 0.2500000000000000000, 0.5000000000000000000, 0.7500000000000000000, 1.000000000000000000 ),
 .UNSPECIFIED. ) ;
#42322=ORIENTED_EDGE ( 'NONE', *, *, #39671, .T. ) ;
#42323=CARTESIAN_POINT ( 'NONE',  ( -10.49015519723160850, -15.76906674594861002, 61.11077061167396351 ) ) ;
#42324=CARTESIAN_POINT ( 'NONE',  ( -10.16786014542261007, -13.12079378898483384, 71.25182636653194379 ) ) ;
#42325=EDGE_CURVE ( 'NONE', #41967, #7285, #20817, .T. ) ;
#42328=CARTESIAN_POINT ( 'NONE',  ( -12.34455782425648351, -9.992743752570305560, 57.19821645454700842 ) ) ;
#42329=CARTESIAN_POINT ( 'NONE',  ( -23.65624121974494543, -11.51332442490695129, 66.42214514605623776 ) ) ;
#42331=CARTESIAN_POINT ( 'NONE',  ( -23.77562434277295367, -17.86939608417919345, 59.01850491586762359 ) ) ;
#42333=ORIENTED_EDGE ( 'NONE', *, *, #30788, .T. ) ;
#42334=CARTESIAN_POINT ( 'NONE',  ( -11.46310342473229049, -11.03940158154180651, 61.09374645412970750 ) ) ;
#42336=( BOUNDED_CURVE ( )  B_SPLINE_CURVE ( 3, ( #9226, #23769, #24250, #39256 ),
 .UNSPECIFIED., .F., .F. ) 
 B_SPLINE_CURVE_WITH_KNOTS ( ( 4, 4 ),
 ( 0.9074455897393661763, 1.000000000000000000 ),
 .UNSPECIFIED. ) 
 CURVE ( )  GEOMETRIC_REPRESENTATION_ITEM ( )  RATIONAL_B_SPLINE_CURVE ( ( 0.6983129098260806300, 0.7760317562606875441, 0.8765941196519939638, 1.000000000000000000 ) ) 
 REPRESENTATION_ITEM ( '' )  );
#42337=CARTESIAN_POINT ( 'NONE',  ( -18.79049830835916524, -7.892586073225762000, 70.38540174208183942 ) ) ;
#42340=VERTEX_POINT ( 'NONE', #45757 ) ;
#42341=EDGE_LOOP ( 'NONE', ( #22168, #5692, #28661, #35457, #5643 ) ) ;
#42342=EDGE_CURVE ( 'NONE', #33146, #31985, #851, .T. ) ;
#42345=DIRECTION ( 'NONE',  ( -3.298726454030011118E-06, 1.683524824177191357E-06, 0.9999999999931419303 ) ) ;
#42346=CARTESIAN_POINT ( 'NONE',  ( -15.82259855879412846, -7.533287975791289171, 67.25511890406325222 ) ) ;
#42349=CARTESIAN_POINT ( 'NONE',  ( -24.45714095472541771, -14.31630891555218987, 69.66747352629326429 ) ) ;
#42351=ADVANCED_FACE ( 'NONE', ( #18904 ), #7593, .T. ) ;
#42352=CARTESIAN_POINT ( 'NONE',  ( -24.41553149706675896, -15.71832598455623398, 69.81835354388927328 ) ) ;
#42353=ORIENTED_EDGE ( 'NONE', *, *, #18957, .F. ) ;
#42354=EDGE_CURVE ( 'NONE', #34358, #14163, #41386, .T. ) ;
#42355=CARTESIAN_POINT ( 'NONE',  ( -24.31477923169101629, -16.30090137217950996, 59.40860294853779777 ) ) ;
#42356=EDGE_CURVE ( 'NONE', #34511, #34680, #46982, .T. ) ;
#42357=CARTESIAN_POINT ( 'NONE',  ( -24.22219984651093583, -16.48362222048029579, 59.19502791767319394 ) ) ;
#42358=EDGE_LOOP ( 'NONE', ( #8284, #26977 ) ) ;
#42359=CARTESIAN_POINT ( 'NONE',  ( -20.37524731190853799, -7.968593674222963053, 70.35826172290288127 ) ) ;
#42361=CYLINDRICAL_SURFACE ( 'NONE', #12282, 0.1500000000000061562 ) ;
#42364=CARTESIAN_POINT ( 'NONE',  ( -24.29299122354570883, -17.69571185755203757, 62.58705726155704951 ) ) ;
#42365=FACE_OUTER_BOUND ( 'NONE', #19237, .T. ) ;
#42368=AXIS2_PLACEMENT_3D ( 'NONE', #3467, #40414, #29090 ) ;
#42369=CARTESIAN_POINT ( 'NONE',  ( -15.47894645291934523, -21.58867816219044755, 68.46104220717563749 ) ) ;
#42371=FACE_OUTER_BOUND ( 'NONE', #21121, .T. ) ;
#42372=CARTESIAN_POINT ( 'NONE',  ( -14.86587017669673649, -21.80700303724089295, 61.74945191855038473 ) ) ;
#42373=ORIENTED_EDGE ( 'NONE', *, *, #25985, .T. ) ;
#42374=DIRECTION ( 'NONE',  ( -5.731567514496413899E-31, -1.020425574103664789E-16, -1.000000000000000000 ) ) ;
#42375=VECTOR ( 'NONE', #37688, 1000.000000000000114 ) ;
#42376=CIRCLE ( 'NONE', #41602, 6.899999999999999467 ) ;
#42377=CARTESIAN_POINT ( 'NONE',  ( -11.89466307818281798, -10.43082414681992276, 74.85374085024349711 ) ) ;
#42379=CARTESIAN_POINT ( 'NONE',  ( -20.49479342634786505, -8.021289690749126677, 66.94137462304620101 ) ) ;
#42380=CYLINDRICAL_SURFACE ( 'NONE', #5929, 0.1500000000000010769 ) ;
#42381=ORIENTED_EDGE ( 'NONE', *, *, #43261, .T. ) ;
#42383=CARTESIAN_POINT ( 'NONE',  ( -15.43182990062313564, -8.046249867383863830, 74.36513541778452918 ) ) ;
#42384=CARTESIAN_POINT ( 'NONE',  ( -14.60628068055246942, -7.912570010659592867, 60.36350377317607752 ) ) ;
#42386=CARTESIAN_POINT ( 'NONE',  ( -22.38767768884900988, -19.81996202295057330, 65.58933089874275879 ) ) ;
#42387=CARTESIAN_POINT ( 'NONE',  ( -23.98503169607928953, -17.39005800936845603, 66.22885190747201989 ) ) ;
#42390=CARTESIAN_POINT ( 'NONE',  ( -17.33515886584969223, -7.808492153737893737, 70.56206024376236030 ) ) ;
#42393=CARTESIAN_POINT ( 'NONE',  ( -23.55000801791835485, -19.04907288299056489, 65.93115295761097627 ) ) ;
#42395=ORIENTED_EDGE ( 'NONE', *, *, #27682, .T. ) ;
#42396=CARTESIAN_POINT ( 'NONE',  ( -10.02191625022346955, -15.65273779443635327, 61.15293638507743168 ) ) ;
#42397=CARTESIAN_POINT ( 'NONE',  ( -19.23866243364646422, -21.62168334911581269, 58.52507384657483414 ) ) ;
#42398=CARTESIAN_POINT ( 'NONE',  ( -23.95290610889346539, -17.47904830382568875, 69.50519765973122333 ) ) ;
#42401=B_SPLINE_CURVE_WITH_KNOTS ( 'NONE', 3,
 ( #25594, #48009, #10103, #21438, #25126, #40144, #10818, #32738, #33204, #40859 ),
 .UNSPECIFIED., .F., .F.,
 ( 4, 2, 2, 2, 4 ),
 ( 0.000000000000000000, 0.2500000000000000000, 0.5000000000000000000, 0.7500000000000000000, 1.000000000000000000 ),
 .UNSPECIFIED. ) ;
#42402=EDGE_CURVE ( 'NONE', #26226, #4075, #8690, .T. ) ;
#42403=( BOUNDED_CURVE ( )  B_SPLINE_CURVE ( 3, ( #9224, #39006, #2307, #27923 ),
 .UNSPECIFIED., .F., .F. ) 
 B_SPLINE_CURVE_WITH_KNOTS ( ( 4, 4 ),
 ( 0.000000000000000000, 0.4074455897393611248 ),
 .UNSPECIFIED. ) 
 CURVE ( )  GEOMETRIC_REPRESENTATION_ITEM ( )  RATIONAL_B_SPLINE_CURVE ( ( 1.000000000000000000, 0.4567392136813394066, 0.3561768502900330979, 0.6983129098260809631 ) ) 
 REPRESENTATION_ITEM ( '' )  );
#42404=ORIENTED_EDGE ( 'NONE', *, *, #1526, .F. ) ;
#42405=VERTEX_POINT ( 'NONE', #11512 ) ;
#42408=EDGE_CURVE ( 'NONE', #26785, #25255, #34152, .T. ) ;
#42409=CARTESIAN_POINT ( 'NONE',  ( -11.97744758732939019, -9.726227503278199293, 60.75906873251374662 ) ) ;
#42411=CARTESIAN_POINT ( 'NONE',  ( -21.80947398209100285, -9.353160252369512762, 63.49153755919518005 ) ) ;
#42413=ORIENTED_EDGE ( 'NONE', *, *, #9077, .T. ) ;
#42415=CARTESIAN_POINT ( 'NONE',  ( -10.43414264852987117, -14.42617553249795392, 68.14183543910880303 ) ) ;
#42416=CARTESIAN_POINT ( 'NONE',  ( -18.53202070066404517, -7.846807721809618386, 73.84064401782792686 ) ) ;
#42417=ORIENTED_EDGE ( 'NONE', *, *, #23639, .F. ) ;
#42418=EDGE_CURVE ( 'NONE', #33406, #27678, #5147, .T. ) ;
#42419=CARTESIAN_POINT ( 'NONE',  ( -23.89931086185965370, -17.60652826309538099, 59.21198374917257468 ) ) ;
#42421=CARTESIAN_POINT ( 'NONE',  ( -23.18182585610446722, -10.73448348362502536, 59.90203689567525913 ) ) ;
#42424=CARTESIAN_POINT ( 'NONE',  ( -19.86401518824997225, -21.42384811948916834, 69.22010401872219632 ) ) ;
#42425=CARTESIAN_POINT ( 'NONE',  ( -17.54757171063225485, -7.760139436107405864, 63.84497264672818773 ) ) ;
#42427=B_SPLINE_CURVE_WITH_KNOTS ( 'NONE', 3,
 ( #22251, #6749, #37490, #37242, #6989, #18539, #37007, #44669, #29893, #40471 ),
 .UNSPECIFIED., .F., .F.,
 ( 4, 2, 2, 2, 4 ),
 ( 0.000000000000000000, 0.2500000000000000000, 0.5000000000000000000, 0.7500000000000000000, 1.000000000000000000 ),
 .UNSPECIFIED. ) ;
#42428=CARTESIAN_POINT ( 'NONE',  ( -24.47559319016939483, -14.50700548578266513, 59.39867536442299212 ) ) ;
#42429=CARTESIAN_POINT ( 'NONE',  ( -23.35776552503721959, -18.61638513218611735, 69.59371953224538743 ) ) ;
#42430=EDGE_LOOP ( 'NONE', ( #21511, #28729 ) ) ;
#42432=CARTESIAN_POINT ( 'NONE',  ( -19.64830701089596232, -21.50306318240866332, 61.99503448598593280 ) ) ;
#42433=ADVANCED_FACE ( 'NONE', ( #46937 ), #20359, .T. ) ;
#42437=CARTESIAN_POINT ( 'NONE',  ( -16.02724774380223849, -7.491242405164911133, 63.78515641179975404 ) ) ;
#42438=DIRECTION ( 'NONE',  ( -0.9441784275685842776, 0.3294345108122634369, 1.993146885055995131E-08 ) ) ;
#42444=AXIS2_PLACEMENT_3D ( 'NONE', #17447, #36621, #28543 ) ;
#42446=ORIENTED_EDGE ( 'NONE', *, *, #31951, .T. ) ;
#42450=CARTESIAN_POINT ( 'NONE',  ( -24.32886716615087153, -16.23426984194678724, 62.60800820172418923 ) ) ;
#42452=CARTESIAN_POINT ( 'NONE',  ( -24.80446278886646283, -15.82547754058744083, 69.63283851078359987 ) ) ;
#42454=CARTESIAN_POINT ( 'NONE',  ( -24.42312040261578687, -14.69246961071934798, 59.35186350302572578 ) ) ;
#42455=CARTESIAN_POINT ( 'NONE',  ( -24.03326526335923319, -11.37062187434330873, 66.56181149773966865 ) ) ;
#42456=VERTEX_POINT ( 'NONE', #12950 ) ;
#42457=CARTESIAN_POINT ( 'NONE',  ( -23.87620549320321572, -17.65941701095796645, 66.03537195726408981 ) ) ;
#42462=CARTESIAN_POINT ( 'NONE',  ( -24.86426575691346486, -14.42665972991787271, 66.33292729196470816 ) ) ;
#42464=ORIENTED_EDGE ( 'NONE', *, *, #23257, .F. ) ;
#42465=ORIENTED_EDGE ( 'NONE', *, *, #48385, .T. ) ;
#42467=LINE ( 'NONE', #35301, #38996 ) ;
#42468=CARTESIAN_POINT ( 'NONE',  ( -15.69205246790211561, -7.972184624072811587, 74.49474465824219749 ) ) ;
#42470=CARTESIAN_POINT ( 'NONE',  ( -20.38775279631941473, -8.467419115199003699, 66.78104087472024730 ) ) ;
#42471=EDGE_CURVE ( 'NONE', #27235, #21456, #31978, .T. ) ;
#42476=ORIENTED_EDGE ( 'NONE', *, *, #35855, .F. ) ;
#42477=CARTESIAN_POINT ( 'NONE',  ( -22.39908541082256832, -19.73366760896285399, 69.45952680249732225 ) ) ;
#42481=EDGE_CURVE ( 'NONE', #48003, #22219, #10184, .T. ) ;
#42482=CARTESIAN_POINT ( 'NONE',  ( -21.94242186726961208, -9.397052521110282441, 60.00699132926281010 ) ) ;
#42483=DIRECTION ( 'NONE',  ( -0.9687793358424796608, 0.2479245821708770392, 7.674369900078814127E-17 ) ) ;
#42485=FACE_OUTER_BOUND ( 'NONE', #29965, .T. ) ;
#42486=B_SPLINE_CURVE_WITH_KNOTS ( 'NONE', 1,
 ( #33533, #37233 ),
 .UNSPECIFIED., .F., .F.,
 ( 2, 2 ),
 ( 0.000000000000000000, 1.000000000000000000 ),
 .UNSPECIFIED. ) ;
#42489=EDGE_CURVE ( 'NONE', #3333, #21578, #38823, .T. ) ;
#42490=LINE ( 'NONE', #12914, #21909 ) ;
#42491=CARTESIAN_POINT ( 'NONE',  ( -12.14425506381237341, -10.13739722748950634, 64.32914326607961186 ) ) ;
#42492=EDGE_LOOP ( 'NONE', ( #39567, #20107, #12025, #37396, #32432 ) ) ;
#42493=CARTESIAN_POINT ( 'NONE',  ( -10.33531725737393181, -17.10115422170377641, 57.87255955594724810 ) ) ;
#42494=CARTESIAN_POINT ( 'NONE',  ( -11.55573786329523855, -10.21941616939416342, 71.15388509157428132 ) ) ;
#42496=FACE_BOUND ( 'NONE', #4159, .T. ) ;
#42498=CARTESIAN_POINT ( 'NONE',  ( -11.40678069298109953, -18.38590894181533031, 58.09249207256556247 ) ) ;
#42499=CARTESIAN_POINT ( 'NONE',  ( -15.88656107989463706, -7.980151544674868980, 67.14007279409138107 ) ) ;
#42501=ORIENTED_EDGE ( 'NONE', *, *, #41673, .T. ) ;
#42502=CARTESIAN_POINT ( 'NONE',  ( -17.42409385541300892, -14.80920654474439502, 75.49999999999994316 ) ) ;
#42503=ORIENTED_EDGE ( 'NONE', *, *, #2656, .F. ) ;
#42504=CARTESIAN_POINT ( 'NONE',  ( -20.09319558404390449, -21.76479983661718265, 72.52761822131290614 ) ) ;
#42505=CARTESIAN_POINT ( 'NONE',  ( -13.26878207226084783, -9.173970493528688763, 67.49015956650667647 ) ) ;
#42506=EDGE_CURVE ( 'NONE', #2636, #35967, #1879, .T. ) ;
#42507=B_SPLINE_CURVE_WITH_KNOTS ( 'NONE', 1,
 ( #3233, #19231 ),
 .UNSPECIFIED., .F., .F.,
 ( 2, 2 ),
 ( 0.000000000000000000, 1.000000000000000000 ),
 .UNSPECIFIED. ) ;
#42508=ORIENTED_EDGE ( 'NONE', *, *, #240, .T. ) ;
#42509=CARTESIAN_POINT ( 'NONE',  ( -20.10030204730919223, -21.76202525863913451, 72.51983304728076973 ) ) ;
#42510=ADVANCED_FACE ( 'NONE', ( #35603 ), #31921, .T. ) ;
#42511=CARTESIAN_POINT ( 'NONE',  ( -13.27770465421436619, -9.107456272842560097, 64.20946529204060482 ) ) ;
#42516=( NAMED_UNIT ( * ) PLANE_ANGLE_UNIT ( ) SI_UNIT ( $, .RADIAN. ) );
#42518=EDGE_CURVE ( 'NONE', #26697, #25255, #44370, .T. ) ;
#42519=CARTESIAN_POINT ( 'NONE',  ( -17.36015840614627592, -7.359395087992972151, 67.20535029649403214 ) ) ;
#42520=CARTESIAN_POINT ( 'NONE',  ( -10.27345486655506868, -12.71824029969684844, 64.45331411623358520 ) ) ;
#42521=CARTESIAN_POINT ( 'NONE',  ( -16.34431749418946822, -22.18055063995905130, 61.95556900725736682 ) ) ;
#42522=VECTOR ( 'NONE', #42709, 1000.000000000000114 ) ;
#42523=ORIENTED_EDGE ( 'NONE', *, *, #15545, .F. ) ;
#42526=CARTESIAN_POINT ( 'NONE',  ( -11.47484201153877237, -11.01958276889226518, 60.97886048380778590 ) ) ;
#42527=B_SPLINE_CURVE_WITH_KNOTS ( 'NONE', 1,
 ( #5642, #20651 ),
 .UNSPECIFIED., .F., .F.,
 ( 2, 2 ),
 ( 0.000000000000000000, 1.000000000000000000 ),
 .UNSPECIFIED. ) ;
#42529=VECTOR ( 'NONE', #664, 1000.000000000000114 ) ;
#42530=CARTESIAN_POINT ( 'NONE',  ( -19.72840181597629439, -21.41912346864951999, 65.53774255715215702 ) ) ;
#42531=VERTEX_POINT ( 'NONE', #43001 ) ;
#42532=( BOUNDED_CURVE ( )  B_SPLINE_CURVE ( 3, ( #4279, #26686, #5012, #45404 ),
 .UNSPECIFIED., .F., .F. ) 
 B_SPLINE_CURVE_WITH_KNOTS ( ( 4, 4 ),
 ( 0.5000000000000000000, 0.9074455897393640669 ),
 .UNSPECIFIED. ) 
 CURVE ( )  GEOMETRIC_REPRESENTATION_ITEM ( )  RATIONAL_B_SPLINE_CURVE ( ( 0.9999999999999942268, 0.4567392136813319681, 0.3561768502900342082, 0.6983129098260947298 ) ) 
 REPRESENTATION_ITEM ( '' )  );
#42534=EDGE_LOOP ( 'NONE', ( #20045, #17211, #34919, #41361 ) ) ;
#42535=DIRECTION ( 'NONE',  ( -5.468526094916624094E-08, -8.832527036150760808E-06, 0.9999999999609917589 ) ) ;
#42536=CARTESIAN_POINT ( 'NONE',  ( -16.06050865347321732, -9.480920197610746669, 53.49999999999995026 ) ) ;
#42537=CARTESIAN_POINT ( 'NONE',  ( -12.43502688619039453, -19.72161029367247309, 65.05601852582830702 ) ) ;
#42540=( BOUNDED_SURFACE ( )  B_SPLINE_SURFACE ( 3, 1, ( 
 ( #42651, #46335 ),
 ( #12589, #2228 ),
 ( #39900, #43372 ),
 ( #13056, #12829 ),
 ( #28087, #35704 ),
 ( #35472, #31550 ),
 ( #47306, #39659 ) ),
 .UNSPECIFIED., .T., .F., .F. ) 
 B_SPLINE_SURFACE_WITH_KNOTS ( ( 4, 3, 4 ),
 ( 2, 2 ),
 ( 0.000000000000000000, 0.5000000000000000000, 1.000000000000000000 ),
 ( 0.000000000000000000, 1.000000000000000000 ),
 .UNSPECIFIED. ) 
 GEOMETRIC_REPRESENTATION_ITEM ( )  RATIONAL_B_SPLINE_SURFACE ( (
 ( 1.000000000000000000, 1.000000000000000000),
 ( 0.3333333333333335369, 0.3333333333333330373),
 ( 0.3333333333333335369, 0.3333333333333330373),
 ( 1.000000000000000000, 1.000000000000000000),
 ( 0.3333333333333333703, 0.3333333333333333703),
 ( 0.3333333333333333703, 0.3333333333333333703),
 ( 1.000000000000000000, 1.000000000000000000) ) ) 
 REPRESENTATION_ITEM ( '' )  SURFACE ( )  );
#42543=CARTESIAN_POINT ( 'NONE',  ( -10.40174226954351866, -17.29724918936392442, 61.34238429002267878 ) ) ;
#42544=CARTESIAN_POINT ( 'NONE',  ( -10.85841931818429629, -17.37798394237199062, 64.91267318220633342 ) ) ;
#42545=CARTESIAN_POINT ( 'NONE',  ( -13.00141362859484673, -9.318806420380903788, 70.85485155228010967 ) ) ;
#42546=EDGE_CURVE ( 'NONE', #20698, #38947, #2062, .T. ) ;
#42547=AXIS2_PLACEMENT_3D ( 'NONE', #16619, #20330, #34605 ) ;
#42548=ORIENTED_EDGE ( 'NONE', *, *, #27944, .F. ) ;
#42549=LINE ( 'NONE', #4623, #32036 ) ;
#42550=CARTESIAN_POINT ( 'NONE',  ( -24.82391033454606699, -15.67355493173947956, 73.12586871779123499 ) ) ;
#42551=CARTESIAN_POINT ( 'NONE',  ( -23.41977899678227004, -11.19648470850049904, 73.36193302072521760 ) ) ;
#42552=ORIENTED_EDGE ( 'NONE', *, *, #23410, .F. ) ;
#42553=CARTESIAN_POINT ( 'NONE',  ( -10.00037608677762258, -14.17511115329010707, 61.03165943758897782 ) ) ;
#42555=( BOUNDED_SURFACE ( )  B_SPLINE_SURFACE ( 3, 1, ( 
 ( #38899, #20186 ),
 ( #35197, #16480 ),
 ( #31516, #12793 ),
 ( #27814, #24133 ),
 ( #7799, #14889 ),
 ( #33867, #7308 ),
 ( #22816, #26492 ) ),
 .UNSPECIFIED., .T., .F., .F. ) 
 B_SPLINE_SURFACE_WITH_KNOTS ( ( 4, 3, 4 ),
 ( 2, 2 ),
 ( 0.000000000000000000, 0.5000000000000000000, 1.000000000000000000 ),
 ( 0.000000000000000000, 1.000000000000000000 ),
 .UNSPECIFIED. ) 
 GEOMETRIC_REPRESENTATION_ITEM ( )  RATIONAL_B_SPLINE_SURFACE ( (
 ( 1.000000000000000000, 1.000000000000000000),
 ( 0.3333333333333335369, 0.3333333333333330373),
 ( 0.3333333333333335369, 0.3333333333333330373),
 ( 1.000000000000000000, 1.000000000000000000),
 ( 0.3333333333333333703, 0.3333333333333333703),
 ( 0.3333333333333333703, 0.3333333333333333703),
 ( 1.000000000000000000, 1.000000000000000000) ) ) 
 REPRESENTATION_ITEM ( '' )  SURFACE ( )  );
#42557=CARTESIAN_POINT ( 'NONE',  ( -23.43898735819080059, -11.13148316174488528, 73.65633489482847551 ) ) ;
#42559=CARTESIAN_POINT ( 'NONE',  ( -21.99178500617274779, -9.439039195359631762, 59.72171213140594404 ) ) ;
#42561=CARTESIAN_POINT ( 'NONE',  ( -16.72330486927764426, -21.83230113783351101, 61.91134987066439521 ) ) ;
#42563=PLANE ( 'NONE',  #39911 ) ;
#42565=ORIENTED_EDGE ( 'NONE', *, *, #31932, .T. ) ;
#42566=CARTESIAN_POINT ( 'NONE',  ( -23.77562434277295367, -17.86939608417919345, 59.01850491586762359 ) ) ;
#42568=DIRECTION ( 'NONE',  ( -0.8402231219892289937, 0.5322911103758086737, 0.1033986416233890204 ) ) ;
#42569=CARTESIAN_POINT ( 'NONE',  ( -17.84735443592641602, -7.371153788697909270, 60.19565345827741965 ) ) ;
#42570=FACE_OUTER_BOUND ( 'NONE', #21756, .T. ) ;
#42571=ADVANCED_FACE ( 'NONE', ( #19062 ), #11928, .T. ) ;
#42573=CARTESIAN_POINT ( 'NONE',  ( -10.37600963001940713, -14.53000751884195374, 64.59623758275894545 ) ) ;
#42574=ADVANCED_FACE ( 'NONE', ( #38498 ), #3265, .T. ) ;
#42575=LINE ( 'NONE', #42803, #43220 ) ;
#42576=EDGE_CURVE ( 'NONE', #25499, #20428, #19546, .T. ) ;
#42578=EDGE_CURVE ( 'NONE', #33105, #19220, #31608, .T. ) ;
#42579=VECTOR ( 'NONE', #26007, 1000.000000000000227 ) ;
#42580=ORIENTED_EDGE ( 'NONE', *, *, #7105, .T. ) ;
#42581=ORIENTED_EDGE ( 'NONE', *, *, #1273, .F. ) ;
#42582=CARTESIAN_POINT ( 'NONE',  ( -19.34161870936485883, -22.00820632818791012, 58.67507381970625602 ) ) ;
#42583=CARTESIAN_POINT ( 'NONE',  ( -13.12790236870489302, -8.721809449924828428, 64.09601920791236296 ) ) ;
#42586=CARTESIAN_POINT ( 'NONE',  ( -24.45714095472541771, -14.31630891555219165, 69.66747352629326429 ) ) ;
#42587=FACE_OUTER_BOUND ( 'NONE', #33778, .T. ) ;
#42588=CARTESIAN_POINT ( 'NONE',  ( -23.28150713458464338, -18.64225386619112257, 69.59372035755308161 ) ) ;
#42589=LINE ( 'NONE', #8851, #8013 ) ;
#42590=ORIENTED_EDGE ( 'NONE', *, *, #17498, .F. ) ;
#42592=AXIS2_PLACEMENT_3D ( 'NONE', #31252, #15730, #45807 ) ;
#42593=CARTESIAN_POINT ( 'NONE',  ( -22.80481760130283675, -10.24931098477615166, 70.42667203218238114 ) ) ;
#42595=CARTESIAN_POINT ( 'NONE',  ( -23.68216640822461372, -11.66929755891756670, 66.61141575710782092 ) ) ;
#42597=CARTESIAN_POINT ( 'NONE',  ( -12.50766613833179974, -19.86205114983803810, 64.86674886870797252 ) ) ;
#42598=VECTOR ( 'NONE', #37728, 1000.000000000000114 ) ;
#42600=EDGE_CURVE ( 'NONE', #47353, #17705, #15182, .T. ) ;
#42602=CARTESIAN_POINT ( 'NONE',  ( -21.68499379980493913, -9.192514338196572155, 66.96149992326067490 ) ) ;
#42604=CARTESIAN_POINT ( 'NONE',  ( -24.16424020987968646, -16.88652737071335252, 72.76847378359866525 ) ) ;
#42605=AXIS2_PLACEMENT_3D ( 'NONE', #43195, #35057, #35303 ) ;
#42606=ORIENTED_EDGE ( 'NONE', *, *, #30513, .T. ) ;
#42607=CARTESIAN_POINT ( 'NONE',  ( -24.84240844029834250, -14.11474841844398043, 69.76619977786306492 ) ) ;
#42608=B_SPLINE_CURVE_WITH_KNOTS ( 'NONE', 3,
 ( #14733, #15482, #26346, #48497, #3697, #29805, #41863, #34449, #739, #15733 ),
 .UNSPECIFIED., .F., .F.,
 ( 4, 2, 2, 2, 4 ),
 ( 0.1272669073657639871, 0.2522669073462675549, 0.3772669073267711504, 0.5022669073072747459, 0.6272669072877783414 ),
 .UNSPECIFIED. ) ;
#42611=CARTESIAN_POINT ( 'NONE',  ( -22.10541318350566442, -20.01527617504624601, 65.77591942924708235 ) ) ;
#42612=ORIENTED_EDGE ( 'NONE', *, *, #9134, .F. ) ;
#42617=CARTESIAN_POINT ( 'NONE',  ( -10.42411290126982060, -14.77598683159526161, 71.34285171099139689 ) ) ;
#42618=ORIENTED_EDGE ( 'NONE', *, *, #41120, .T. ) ;
#42619=CARTESIAN_POINT ( 'NONE',  ( -19.41474841345058522, -21.52018966427049307, 62.29503644830997189 ) ) ;
#42623=CARTESIAN_POINT ( 'NONE',  ( -23.19916440516392697, -19.59445054535707698, 53.49999999999994316 ) ) ;
#42624=CARTESIAN_POINT ( 'NONE',  ( -24.07098297129566333, -12.61366397057463118, 73.54225587970537958 ) ) ;
#42625=CARTESIAN_POINT ( 'NONE',  ( -22.25094433143537387, -9.134348456342106459, 59.87171212369386097 ) ) ;
#42627=CYLINDRICAL_SURFACE ( 'NONE', #12911, 0.1500000000000073774 ) ;
#42629=CARTESIAN_POINT ( 'NONE',  ( -11.63496427220788121, -10.77921706672702129, 74.43884596448377522 ) ) ;
#42631=CARTESIAN_POINT ( 'NONE',  ( -24.44055745662519641, -14.11932379769929113, 73.13743607903229815 ) ) ;
#42632=ADVANCED_FACE ( 'NONE', ( #4778 ), #30163, .T. ) ;
#42633=ADVANCED_FACE ( 'NONE', ( #34806 ), #25270, .T. ) ;
#42634=ORIENTED_EDGE ( 'NONE', *, *, #21730, .F. ) ;
#42636=CARTESIAN_POINT ( 'NONE',  ( -10.42334091404133645, -15.64104667191196540, 61.33789045260129313 ) ) ;
#42637=CARTESIAN_POINT ( 'NONE',  ( -17.92193097897699872, -21.84160713959417421, 62.17535923543129428 ) ) ;
#42638=ORIENTED_EDGE ( 'NONE', *, *, #48466, .F. ) ;
#42639=CARTESIAN_POINT ( 'NONE',  ( -15.54840433177174397, -8.005034934413657766, 67.29574103338339341 ) ) ;
#42640=CYLINDRICAL_SURFACE ( 'NONE', #30303, 0.1500000000000026590 ) ;
#42641=CARTESIAN_POINT ( 'NONE',  ( -10.29167786474582869, -12.65701390312483809, 64.37561959354262342 ) ) ;
#42642=CARTESIAN_POINT ( 'NONE',  ( -13.43773910423563400, -20.62433115109003268, 58.33177939114180788 ) ) ;
#42645=VERTEX_POINT ( 'NONE', #46867 ) ;
#42646=ADVANCED_FACE ( 'NONE', ( #35533 ), #39960, .T. ) ;
#42647=ADVANCED_FACE ( 'NONE', ( #5514 ), #47109, .T. ) ;
#42648=B_SPLINE_CURVE_WITH_KNOTS ( 'NONE', 1,
 ( #45012, #11257 ),
 .UNSPECIFIED., .F., .F.,
 ( 2, 2 ),
 ( 0.000000000000000000, 1.000000000000000000 ),
 .UNSPECIFIED. ) ;
#42651=CARTESIAN_POINT ( 'NONE',  ( -12.76547314785493192, -9.517330534081262172, 74.60450883341005124 ) ) ;
#42652=CARTESIAN_POINT ( 'NONE',  ( -21.43549133165072362, -9.072522135161841916, 70.41667131949601810 ) ) ;
#42653=ORIENTED_EDGE ( 'NONE', *, *, #7099, .T. ) ;
#42654=ORIENTED_EDGE ( 'NONE', *, *, #47634, .F. ) ;
#42656=ORIENTED_EDGE ( 'NONE', *, *, #33718, .T. ) ;
#42658=CARTESIAN_POINT ( 'NONE',  ( -11.96606040034933471, -9.738391814011444936, 60.75192256564785254 ) ) ;
#42659=CARTESIAN_POINT ( 'NONE',  ( -24.10581758648508099, -12.72203489083164740, 70.07242970654482406 ) ) ;
#42660=ORIENTED_EDGE ( 'NONE', *, *, #1013, .T. ) ;
#42662=CARTESIAN_POINT ( 'NONE',  ( -22.69190674372240935, -10.11825871574920654, 73.78161098756908132 ) ) ;
#42663=ORIENTED_EDGE ( 'NONE', *, *, #4722, .F. ) ;
#42664=CARTESIAN_POINT ( 'NONE',  ( -10.64068610965668960, -17.88985431858020547, 71.72751587850088129 ) ) ;
#42665=CARTESIAN_POINT ( 'NONE',  ( -23.78474288321120511, -17.73496378845812771, 62.54531179860746448 ) ) ;
#42666=B_SPLINE_CURVE_WITH_KNOTS ( 'NONE', 1,
 ( #2261, #6202 ),
 .UNSPECIFIED., .F., .F.,
 ( 2, 2 ),
 ( 0.000000000000000000, 1.000000000000000000 ),
 .UNSPECIFIED. ) ;
#42668=CARTESIAN_POINT ( 'NONE',  ( -19.90433039125390025, -21.83431899736824988, 69.04987161812600505 ) ) ;
#42669=CARTESIAN_POINT ( 'NONE',  ( -10.60399421354195404, -13.23188019733764520, 71.50828540008092205 ) ) ;
#42670=ORIENTED_EDGE ( 'NONE', *, *, #22164, .F. ) ;
#42672=CARTESIAN_POINT ( 'NONE',  ( -18.14263071100308977, -21.82253481906295178, 65.64532146769309406 ) ) ;
#42674=CARTESIAN_POINT ( 'NONE',  ( -17.84735443592641602, -7.371153788697909270, 60.19565345827741965 ) ) ;
#42675=CARTESIAN_POINT ( 'NONE',  ( -14.66790711817407278, -21.29843871104708342, 58.18089935161520287 ) ) ;
#42676=( BOUNDED_CURVE ( )  B_SPLINE_CURVE ( 3, ( #32197, #32894, #36825, #47689 ),
 .UNSPECIFIED., .F., .F. ) 
 B_SPLINE_CURVE_WITH_KNOTS ( ( 4, 4 ),
 ( 0.4074455897393675086, 0.5000000000000000000 ),
 .UNSPECIFIED. ) 
 CURVE ( )  GEOMETRIC_REPRESENTATION_ITEM ( )  RATIONAL_B_SPLINE_CURVE ( ( 0.6983129098261046108, 0.7760317562607000896, 0.8765941196519961842, 0.9999999999999872324 ) ) 
 REPRESENTATION_ITEM ( '' )  );
#42677=CARTESIAN_POINT ( 'NONE',  ( -14.58539460706017543, -21.69719740599226654, 58.36606672081529013 ) ) ;
#42678=CARTESIAN_POINT ( 'NONE',  ( -24.17899278864585355, -11.66673636667039027, 59.66731167108189737 ) ) ;
#42679=CARTESIAN_POINT ( 'NONE',  ( -24.36818545036879868, -13.92577592638252604, 73.34944830282202588 ) ) ;
#42680=ORIENTED_EDGE ( 'NONE', *, *, #4920, .F. ) ;
#42681=CARTESIAN_POINT ( 'NONE',  ( -22.37985709289073455, -19.82347726015160205, 69.17417989525732480 ) ) ;
#42684=CARTESIAN_POINT ( 'NONE',  ( -24.46812100523181144, -14.51191712007779699, 66.19764790277996269 ) ) ;
#42689=CARTESIAN_POINT ( 'NONE',  ( -12.23220189640646538, -19.57856266540686718, 58.07682373937821296 ) ) ;
#42692=CARTESIAN_POINT ( 'NONE',  ( -14.95029678367283665, -21.83651174838278664, 65.20622428847848084 ) ) ;
#42693=CARTESIAN_POINT ( 'NONE',  ( -21.06713455244400635, -20.85430592508659586, 72.66879606033384675 ) ) ;
#42695=CARTESIAN_POINT ( 'NONE',  ( -16.99688961111671404, -22.24707068558670642, 72.28730467040716690 ) ) ;
#42698=( BOUNDED_CURVE ( )  B_SPLINE_CURVE ( 3, ( #35049, #16575, #20042, #27675 ),
 .UNSPECIFIED., .F., .F. ) 
 B_SPLINE_CURVE_WITH_KNOTS ( ( 4, 4 ),
 ( 4.712388980384689674, 4.921828490624009511 ),
 .UNSPECIFIED. ) 
 CURVE ( )  GEOMETRIC_REPRESENTATION_ITEM ( )  RATIONAL_B_SPLINE_CURVE ( ( 1.000000000000000000, 0.9963479302455154896, 0.9963479302455154896, 1.000000000000000000 ) ) 
 REPRESENTATION_ITEM ( '' )  );
#42699=FACE_OUTER_BOUND ( 'NONE', #27501, .T. ) ;
#42700=ADVANCED_FACE ( 'NONE', ( #42699 ), #20531, .T. ) ;
#42701=CARTESIAN_POINT ( 'NONE',  ( -11.96194199484143539, -9.742791280557115741, 60.60272182217008208 ) ) ;
#42702=B_SPLINE_CURVE_WITH_KNOTS ( 'NONE', 3,
 ( #30015, #11294, #21878, #10796, #25815, #29024, #18172, #14222, #3914, #3406 ),
 .UNSPECIFIED., .F., .F.,
 ( 4, 2, 2, 2, 4 ),
 ( 0.1272669073658190264, 0.2522669073463195133, 0.3772669073268200002, 0.5022669073073204871, 0.6272669072878209739 ),
 .UNSPECIFIED. ) ;
#42703=VERTEX_POINT ( 'NONE', #16317 ) ;
#42706=EDGE_CURVE ( 'NONE', #25610, #41313, #30318, .T. ) ;
#42707=CARTESIAN_POINT ( 'NONE',  ( -23.97043363090852353, -12.17094895590152426, 59.62668449103946955 ) ) ;
#42709=DIRECTION ( 'NONE',  ( 0.05202058437830280740, -0.9986460127597464043, 1.657953767687799580E-08 ) ) ;
#42712=ORIENTED_EDGE ( 'NONE', *, *, #3759, .F. ) ;
#42714=CARTESIAN_POINT ( 'NONE',  ( -16.93941734680482725, -7.775588144984237005, 74.24546186738449194 ) ) ;
#42715=AXIS2_PLACEMENT_3D ( 'NONE', #15613, #11950, #41742 ) ;
#42716=CARTESIAN_POINT ( 'NONE',  ( -17.76701911439868198, -7.767511358351252504, 60.38060761803046006 ) ) ;
#42717=CARTESIAN_POINT ( 'NONE',  ( -22.91217743940941176, -10.46398633218385399, 59.71089353488221718 ) ) ;
#42718=CARTESIAN_POINT ( 'NONE',  ( -13.90804716676048258, -20.86209139562971160, 68.45625137333186672 ) ) ;
#42719=ORIENTED_EDGE ( 'NONE', *, *, #47198, .T. ) ;
#42720=CARTESIAN_POINT ( 'NONE',  ( -18.69700338743018264, -7.871300468185871146, 66.90071501288184663 ) ) ;
#42721=CARTESIAN_POINT ( 'NONE',  ( -24.10335570753463230, -17.07466383872621307, 69.29851186845237976 ) ) ;
#42722=ORIENTED_EDGE ( 'NONE', *, *, #26807, .T. ) ;
#42723=CARTESIAN_POINT ( 'NONE',  ( -23.71561414012218094, -17.99693426085591952, 59.41867086777731544 ) ) ;
#42726=CARTESIAN_POINT ( 'NONE',  ( -13.36456289509512096, -21.05617294863179723, 61.69363177936434539 ) ) ;
#42727=CARTESIAN_POINT ( 'NONE',  ( -10.40245588357037043, -14.17414831712846990, 61.20349182037644198 ) ) ;
#42729=CARTESIAN_POINT ( 'NONE',  ( -12.00971705810820467, -9.691755786776280246, 60.67422651510300113 ) ) ;
#42731=EDGE_CURVE ( 'NONE', #13213, #19324, #13352, .T. ) ;
#42732=CARTESIAN_POINT ( 'NONE',  ( -15.09544305450467938, -21.46351983957133669, 65.40596681500470311 ) ) ;
#42733=CARTESIAN_POINT ( 'NONE',  ( -22.57359528252793623, -19.55088050636924990, 72.71688684016393722 ) ) ;
#42734=VERTEX_POINT ( 'NONE', #43429 ) ;
#42736=CARTESIAN_POINT ( 'NONE',  ( -20.83870870799843900, -21.43061845379169839, 58.74500915750943619 ) ) ;
#42738=CARTESIAN_POINT ( 'NONE',  ( -11.17855889551124982, -18.87086522978130532, 64.86211687253867808 ) ) ;
#42740=CARTESIAN_POINT ( 'NONE',  ( -17.06206538396918404, -7.760525543569854356, 67.17606901500077754 ) ) ;
#42743=VERTEX_POINT ( 'NONE', #46389 ) ;
#42744=CARTESIAN_POINT ( 'NONE',  ( -10.67379822573247949, -12.95623351948692381, 64.37722118855614895 ) ) ;
#42745=ORIENTED_EDGE ( 'NONE', *, *, #10036, .F. ) ;
#42746=CARTESIAN_POINT ( 'NONE',  ( -11.15046514442954972, -11.70398196082027376, 67.69152635070139468 ) ) ;
#42747=CARTESIAN_POINT ( 'NONE',  ( -22.90877211956182435, -10.45951156430351503, 63.07186031186947872 ) ) ;
#42748=ORIENTED_EDGE ( 'NONE', *, *, #38654, .F. ) ;
#42749=CARTESIAN_POINT ( 'NONE',  ( -20.52762626839951210, -8.534807245883811788, 63.61121513079540080 ) ) ;
#42750=FACE_BOUND ( 'NONE', #6674, .T. ) ;
#42751=EDGE_LOOP ( 'NONE', ( #26124, #21570, #42322, #34700, #24674 ) ) ;
#42753=VERTEX_POINT ( 'NONE', #16568 ) ;
#42755=CARTESIAN_POINT ( 'NONE',  ( -10.38377074815290868, -15.30802594933397920, 61.18222038349547631 ) ) ;
#42756=EDGE_CURVE ( 'NONE', #2663, #6207, #14873, .T. ) ;
#42758=CARTESIAN_POINT ( 'NONE',  ( -22.81815734205171964, -10.26415160585916020, 70.10358578328691692 ) ) ;
#42759=CARTESIAN_POINT ( 'NONE',  ( -22.48114071483173149, -19.64927648862363796, 72.94400547034429394 ) ) ;
#42760=LINE ( 'NONE', #9030, #834 ) ;
#42765=CARTESIAN_POINT ( 'NONE',  ( -21.59804090337381410, -20.98026344205569771, 72.70941702861115630 ) ) ;
#42766=CARTESIAN_POINT ( 'NONE',  ( -24.87406538417882729, -14.83278061336772069, 59.44289023857400167 ) ) ;
#42767=DIRECTION ( 'NONE',  ( -6.059369603295153624E-06, 3.309764060044371102E-06, 0.9999999999761648439 ) ) ;
#42775=ORIENTED_EDGE ( 'NONE', *, *, #13124, .F. ) ;
#42776=CARTESIAN_POINT ( 'NONE',  ( -12.68532267716109985, -9.060482739934947460, 71.03420753023118550 ) ) ;
#42777=FACE_OUTER_BOUND ( 'NONE', #17997, .T. ) ;
#42778=B_SPLINE_CURVE_WITH_KNOTS ( 'NONE', 1,
 ( #4085, #22532 ),
 .UNSPECIFIED., .F., .F.,
 ( 2, 2 ),
 ( 0.000000000000000000, 1.000000000000000000 ),
 .UNSPECIFIED. ) ;
#42779=CARTESIAN_POINT ( 'NONE',  ( -22.06352374043166265, -8.980015506435984562, 63.37649162950052784 ) ) ;
#42780=CARTESIAN_POINT ( 'NONE',  ( -14.40111994560675690, -7.999901138345907547, 63.95012236324505750 ) ) ;
#42781=VERTEX_POINT ( 'NONE', #39231 ) ;
#42782=CARTESIAN_POINT ( 'NONE',  ( -23.41977742916776251, -11.19648202114625235, 73.66193302070908544 ) ) ;
#42783=EDGE_CURVE ( 'NONE', #46985, #8086, #28809, .T. ) ;
#42784=CARTESIAN_POINT ( 'NONE',  ( -12.39907312731801525, -20.30942516702692657, 68.44319146479406868 ) ) ;
#42785=ORIENTED_EDGE ( 'NONE', *, *, #2373, .T. ) ;
#42787=ORIENTED_EDGE ( 'NONE', *, *, #6461, .T. ) ;
#42788=CARTESIAN_POINT ( 'NONE',  ( -9.974824918456654643, -14.70410907813601220, 71.42759073425887095 ) ) ;
#42789=CARTESIAN_POINT ( 'NONE',  ( -9.975093131592752016, -14.93635113986534257, 74.98274190467411415 ) ) ;
#42790=EDGE_LOOP ( 'NONE', ( #23469, #27312, #2311, #22772, #26633 ) ) ;
#42792=CARTESIAN_POINT ( 'NONE',  ( -19.97164353606484255, -21.81018995992316079, 69.11977899231902711 ) ) ;
#42793=CARTESIAN_POINT ( 'NONE',  ( -14.21162209046732805, -8.087226629722726656, 67.39828596402958283 ) ) ;
#42794=CARTESIAN_POINT ( 'NONE',  ( -9.975583804105555785, -14.65598652642324673, 71.44287259100559595 ) ) ;
#42796=CARTESIAN_POINT ( 'NONE',  ( -17.42409385541300892, -14.80920654474439679, 47.99999999999994316 ) ) ;
#42797=CARTESIAN_POINT ( 'NONE',  ( -20.36919052476639180, -21.22336078664356407, 58.78908032405391992 ) ) ;
#42798=CARTESIAN_POINT ( 'NONE',  ( -10.08052694344373812, -16.06451652471636748, 68.09272548404199199 ) ) ;
#42800=EDGE_CURVE ( 'NONE', #11228, #19229, #26659, .T. ) ;
#42801=CARTESIAN_POINT ( 'NONE',  ( -24.61605457543312525, -12.86511826566283290, 66.41751344402152313 ) ) ;
#42803=CARTESIAN_POINT ( 'NONE',  ( -8.621879165042305004, -16.10189953769286575, 53.49999999999995026 ) ) ;
#42805=ORIENTED_EDGE ( 'NONE', *, *, #33172, .F. ) ;
#42807=CARTESIAN_POINT ( 'NONE',  ( -23.44680839214612789, -18.37680329023430303, 72.77870615285404199 ) ) ;
#42809=CARTESIAN_POINT ( 'NONE',  ( -10.99575410903449679, -18.57485570963264010, 57.85068653066719691 ) ) ;
#42811=CARTESIAN_POINT ( 'NONE',  ( -24.45563495707309087, -14.29732410816288279, 69.65835052054990228 ) ) ;
#42812=( BOUNDED_CURVE ( )  B_SPLINE_CURVE ( 3, ( #16864, #21557, #43241, #17103 ),
 .UNSPECIFIED., .F., .F. ) 
 B_SPLINE_CURVE_WITH_KNOTS ( ( 4, 4 ),
 ( 0.000000000000000000, 0.4074455897393707282 ),
 .UNSPECIFIED. ) 
 CURVE ( )  GEOMETRIC_REPRESENTATION_ITEM ( )  RATIONAL_B_SPLINE_CURVE ( ( 1.000000000000000000, 0.4567392136813279713, 0.3561768502900288236, 0.6983129098261023904 ) ) 
 REPRESENTATION_ITEM ( '' )  );
#42814=CARTESIAN_POINT ( 'NONE',  ( -23.22139416215049579, -18.73524918430105046, 69.40445189021075123 ) ) ;
#42817=VERTEX_POINT ( 'NONE', #16708 ) ;
#42818=EDGE_CURVE ( 'NONE', #4674, #37124, #47749, .T. ) ;
#42819=CARTESIAN_POINT ( 'NONE',  ( -12.38751766673716581, -20.29879047900762501, 68.53646224134315901 ) ) ;
#42821=CARTESIAN_POINT ( 'NONE',  ( -13.29676203468008033, -8.606078807347360637, 57.08312357396523140 ) ) ;
#42823=CARTESIAN_POINT ( 'NONE',  ( -20.84966316371748363, -20.97445663613623523, 58.52986464729110594 ) ) ;
#42824=( BOUNDED_CURVE ( )  B_SPLINE_CURVE ( 3, ( #12770, #27784, #9088, #24099 ),
 .UNSPECIFIED., .F., .F. ) 
 B_SPLINE_CURVE_WITH_KNOTS ( ( 4, 4 ),
 ( 0.4074455897393662873, 0.5000000000000000000 ),
 .UNSPECIFIED. ) 
 CURVE ( )  GEOMETRIC_REPRESENTATION_ITEM ( )  RATIONAL_B_SPLINE_CURVE ( ( 0.6983129098260995038, 0.7760317562606738884, 0.8765941196519654310, 0.9999999999999525935 ) ) 
 REPRESENTATION_ITEM ( '' )  );
#42827=CARTESIAN_POINT ( 'NONE',  ( -23.78676244964941233, -10.93361294341921131, 73.54688584860882372 ) ) ;
#42828=CARTESIAN_POINT ( 'NONE',  ( -15.61466140752867915, -21.57136684691790407, 72.27248776654836604 ) ) ;
#42830=EDGE_CURVE ( 'NONE', #22802, #21258, #16473, .T. ) ;
#42832=ADVANCED_FACE ( 'NONE', ( #46043 ), #30028, .T. ) ;
#42833=CARTESIAN_POINT ( 'NONE',  ( -10.55741651006804993, -16.16889119771467875, 68.08653743916322298 ) ) ;
#42834=( BOUNDED_CURVE ( )  B_SPLINE_CURVE ( 3, ( #17617, #35845, #10003, #43507 ),
 .UNSPECIFIED., .F., .F. ) 
 B_SPLINE_CURVE_WITH_KNOTS ( ( 4, 4 ),
 ( 0.000000000000000000, 0.4074455897393603476 ),
 .UNSPECIFIED. ) 
 CURVE ( )  GEOMETRIC_REPRESENTATION_ITEM ( )  RATIONAL_B_SPLINE_CURVE ( ( 1.000000000000000000, 0.4567392136813374082, 0.3561768502900323208, 0.6983129098260847378 ) ) 
 REPRESENTATION_ITEM ( '' )  );
#42835=AXIS2_PLACEMENT_3D ( 'NONE', #36350, #17867, #14399 ) ;
#42836=CARTESIAN_POINT ( 'NONE',  ( -24.00901317767523935, -17.32824147414624960, 69.42811846502259243 ) ) ;
#42837=EDGE_CURVE ( 'NONE', #8500, #9814, #10183, .T. ) ;
#42841=CARTESIAN_POINT ( 'NONE',  ( -10.12358845859998624, -13.32384912816304556, 74.72171712345732431 ) ) ;
#42845=CARTESIAN_POINT ( 'NONE',  ( -13.14081611093705604, -9.205013627624930805, 70.94105531385672236 ) ) ;
#42846=ORIENTED_EDGE ( 'NONE', *, *, #44869, .T. ) ;
#42847=CARTESIAN_POINT ( 'NONE',  ( -10.01581026994268342, -14.02033193174257342, 61.07967820595483488 ) ) ;
#42848=DIRECTION ( 'NONE',  ( 1.190035119058586791E-06, 1.172070126139376962E-06, 0.9999999999986050048 ) ) ;
#42849=ORIENTED_EDGE ( 'NONE', *, *, #23366, .F. ) ;
#42850=CARTESIAN_POINT ( 'NONE',  ( -10.29788529736029012, -12.63615789972814163, 64.42982626965611814 ) ) ;
#42852=ORIENTED_EDGE ( 'NONE', *, *, #21760, .F. ) ;
#42853=CARTESIAN_POINT ( 'NONE',  ( -17.92189248921373235, -7.825646680082669171, 60.15231005022496902 ) ) ;
#42854=CARTESIAN_POINT ( 'NONE',  ( -24.10114604821131223, -12.70328962272956019, 73.31395830697397287 ) ) ;
#42855=CARTESIAN_POINT ( 'NONE',  ( -16.36834346081282732, -22.18410778960565466, 61.94063409281806543 ) ) ;
#42856=VERTEX_POINT ( 'NONE', #39124 ) ;
#42858=CARTESIAN_POINT ( 'NONE',  ( -11.47236147394688111, -10.32806163424019985, 74.55389795262664165 ) ) ;
#42860=CARTESIAN_POINT ( 'NONE',  ( -20.50148804175696782, -8.024372594274959525, 66.90291339721898112 ) ) ;
#42861=CARTESIAN_POINT ( 'NONE',  ( -20.81696265954430558, -20.93198702957875668, 62.11471400680572685 ) ) ;
#42864=CARTESIAN_POINT ( 'NONE',  ( -23.81758491572420411, -18.63389732182343650, 72.90221683627511595 ) ) ;
#42865=CARTESIAN_POINT ( 'NONE',  ( -14.42683416945219221, -8.428067588089273698, 67.40975083869261653 ) ) ;
#42866=VERTEX_POINT ( 'NONE', #5410 ) ;
#42870=CARTESIAN_POINT ( 'NONE',  ( -18.50931870666621037, -21.77518001355031529, 72.28510940651260341 ) ) ;
#42871=CARTESIAN_POINT ( 'NONE',  ( -19.82413079548422274, -21.27835043604049403, 56.49999999999994316 ) ) ;
#42872=B_SPLINE_CURVE_WITH_KNOTS ( 'NONE', 1,
 ( #43340, #47272 ),
 .UNSPECIFIED., .F., .F.,
 ( 2, 2 ),
 ( 0.000000000000000000, 1.000000000000000000 ),
 .UNSPECIFIED. ) ;
#42873=CARTESIAN_POINT ( 'NONE',  ( -10.79589914290667885, -12.39663942728299517, 60.89033620964060134 ) ) ;
#42874=CIRCLE ( 'NONE', #1201, 0.4000000000000006883 ) ;
#42876=EDGE_CURVE ( 'NONE', #46252, #9124, #3709, .T. ) ;
#42877=CARTESIAN_POINT ( 'NONE',  ( -16.65185932245351808, -21.81708442718849383, 65.51092266128213737 ) ) ;
#42879=CARTESIAN_POINT ( 'NONE',  ( -20.77150559172585886, -8.660957557044635990, 59.85741905887537939 ) ) ;
#42880=CARTESIAN_POINT ( 'NONE',  ( -11.13733870171179596, -11.61806121328041996, 67.90392505421056057 ) ) ;
#42881=CARTESIAN_POINT ( 'NONE',  ( -14.30855566557790404, -8.484641631233271752, 70.74429704309763167 ) ) ;
#42882=LINE ( 'NONE', #23930, #16652 ) ;
#42883=ORIENTED_EDGE ( 'NONE', *, *, #16356, .F. ) ;
#42884=EDGE_LOOP ( 'NONE', ( #35207, #45650, #43484, #8606, #12774 ) ) ;
#42886=CARTESIAN_POINT ( 'NONE',  ( -10.88757860859750082, -12.29993007400385352, 57.43930338741527919 ) ) ;
#42887=ORIENTED_EDGE ( 'NONE', *, *, #11483, .T. ) ;
#42888=EDGE_CURVE ( 'NONE', #44738, #21373, #27785, .T. ) ;
#42890=CARTESIAN_POINT ( 'NONE',  ( -10.01391823204708231, -15.58571177677185915, 57.68137499724732464 ) ) ;
#42891=EDGE_CURVE ( 'NONE', #20914, #35358, #32493, .T. ) ;
#42894=CARTESIAN_POINT ( 'NONE',  ( -11.16720021946830244, -11.56054808309503557, 67.91864607954204303 ) ) ;
#42895=CARTESIAN_POINT ( 'NONE',  ( -22.37985696210566999, -19.82347738784875801, 69.32417989525721680 ) ) ;
#42896=ORIENTED_EDGE ( 'NONE', *, *, #35444, .F. ) ;
#42897=CARTESIAN_POINT ( 'NONE',  ( -10.81107399027072091, -12.51381874052989751, 57.34359806747983868 ) ) ;
#42899=CARTESIAN_POINT ( 'NONE',  ( -10.12170670794182392, -13.33288566098140393, 74.85534528062055415 ) ) ;
#42900=VECTOR ( 'NONE', #39722, 1000.000000000000000 ) ;
#42901=ORIENTED_EDGE ( 'NONE', *, *, #41812, .F. ) ;
#42902=EDGE_CURVE ( 'NONE', #39181, #4870, #7837, .T. ) ;
#42903=CARTESIAN_POINT ( 'NONE',  ( -16.00544582274271477, -7.903112417841744453, 63.95538887075813506 ) ) ;
#42904=CARTESIAN_POINT ( 'NONE',  ( -12.98528529603622594, -9.327379713820903362, 74.41103219219326093 ) ) ;
#42905=CARTESIAN_POINT ( 'NONE',  ( -19.30128557755455176, -21.60500301973953086, 58.81035253397666196 ) ) ;
#42906=ORIENTED_EDGE ( 'NONE', *, *, #609, .F. ) ;
#42907=CARTESIAN_POINT ( 'NONE',  ( -24.27065772746464134, -17.74681645512229622, 62.61214498559143493 ) ) ;
#42908=CARTESIAN_POINT ( 'NONE',  ( -24.42568804997961607, -14.79584355430348097, 62.90223455604580494 ) ) ;
#42909=CARTESIAN_POINT ( 'NONE',  ( -13.62949042321701398, -8.926946430974666669, 56.96967755885751217 ) ) ;
#42910=CYLINDRICAL_SURFACE ( 'NONE', #36288, 0.1500000000000009936 ) ;
#42911=CARTESIAN_POINT ( 'NONE',  ( -20.51077986664673602, -21.09370094575390198, 58.83402211390806968 ) ) ;
#42912=VERTEX_POINT ( 'NONE', #43327 ) ;
#42913=DIRECTION ( 'NONE',  ( -0.9904243694481096316, -0.1380563957348939497, -6.973877022548522575E-08 ) ) ;
#42914=CARTESIAN_POINT ( 'NONE',  ( -11.73260633559210042, -10.00184260618991416, 67.61401560909513364 ) ) ;
#42916=CARTESIAN_POINT ( 'NONE',  ( -23.54659830298692569, -19.05403935986104003, 66.08035378328281695 ) ) ;
#42917=CARTESIAN_POINT ( 'NONE',  ( -14.14525230689395130, -20.99386949692624427, 72.21142318359106582 ) ) ;
#42920=ORIENTED_EDGE ( 'NONE', *, *, #22928, .T. ) ;
#42921=DIRECTION ( 'NONE',  ( -0.9858639740050658684, -0.1675476790616295675, 1.191395510700210208E-16 ) ) ;
#42922=CARTESIAN_POINT ( 'NONE',  ( -10.78978130820344994, -12.42417047965500743, 57.62857332104950814 ) ) ;
#42924=CARTESIAN_POINT ( 'NONE',  ( -24.27033155520888030, -13.12649183948492393, 62.98264177272948672 ) ) ;
#42925=CARTESIAN_POINT ( 'NONE',  ( -10.50429924535250414, -16.15944446069507023, 71.46222527016213633 ) ) ;
#42926=CARTESIAN_POINT ( 'NONE',  ( -22.83929682888979329, -10.29453308790038157, 66.55654356380499337 ) ) ;
#42927=CARTESIAN_POINT ( 'NONE',  ( -22.52972399543339677, -9.943266245822872662, 69.89689837695897268 ) ) ;
#42928=CARTESIAN_POINT ( 'NONE',  ( -14.78766009005058812, -21.34800739930362568, 58.45145834864037937 ) ) ;
#42930=CARTESIAN_POINT ( 'NONE',  ( -12.10369268100898132, -9.594121713099781346, 57.27430968559156810 ) ) ;
#42932=DIRECTION ( 'NONE',  ( -0.9796876409582463419, 0.2005296141562636081, 7.890952370353029293E-08 ) ) ;
#42934=CARTESIAN_POINT ( 'NONE',  ( -10.43024361443327130, -12.24190297806011962, 57.49003819789888325 ) ) ;
#42935=CARTESIAN_POINT ( 'NONE',  ( -10.39864765667697988, -15.39886713103467741, 57.57352593471627955 ) ) ;
#42936=CARTESIAN_POINT ( 'NONE',  ( -23.24966709594328051, -18.77981918306044307, 66.12389400104751758 ) ) ;
#42938=ORIENTED_EDGE ( 'NONE', *, *, #20210, .T. ) ;
#42940=AXIS2_PLACEMENT_3D ( 'NONE', #21140, #44518, #25320 ) ;
#42942=DIRECTION ( 'NONE',  ( -0.2853368233144828459, 0.3443586753093350605, 0.8944271909999156334 ) ) ;
#42943=CARTESIAN_POINT ( 'NONE',  ( -14.81535805098777736, -7.777528402031248511, 56.49999999999994316 ) ) ;
#42944=CARTESIAN_POINT ( 'NONE',  ( -11.55673057814116333, -10.21815940138198009, 71.01247170384147012 ) ) ;
#42945=CARTESIAN_POINT ( 'NONE',  ( -22.92130433334872563, -10.47544214307853672, 59.67491392133583616 ) ) ;
#42947=CARTESIAN_POINT ( 'NONE',  ( -14.02573509563205789, -20.92901172694171308, 68.68298393627175358 ) ) ;
#42948=CARTESIAN_POINT ( 'NONE',  ( -12.57210041907703335, -17.42762882506661271, 53.88362224778187226 ) ) ;
#42949=CARTESIAN_POINT ( 'NONE',  ( -24.23330780873085644, -17.83228236547056156, 62.59644069454639492 ) ) ;
#42950=ORIENTED_EDGE ( 'NONE', *, *, #2760, .T. ) ;
#42951=( BOUNDED_CURVE ( )  B_SPLINE_CURVE ( 3, ( #337, #37240, #26925, #11649 ),
 .UNSPECIFIED., .F., .F. ) 
 B_SPLINE_CURVE_WITH_KNOTS ( ( 4, 4 ),
 ( 0.9074455897393648440, 1.000000000000000000 ),
 .UNSPECIFIED. ) 
 CURVE ( )  GEOMETRIC_REPRESENTATION_ITEM ( )  RATIONAL_B_SPLINE_CURVE ( ( 0.6983129098260881795, 0.7760317562606939834, 0.8765941196519979606, 1.000000000000000000 ) ) 
 REPRESENTATION_ITEM ( '' )  );
#42953=CARTESIAN_POINT ( 'NONE',  ( -24.27033198218900978, -13.12649362337911541, 62.83264177274070050 ) ) ;
#42954=ORIENTED_EDGE ( 'NONE', *, *, #26378, .T. ) ;
#42955=ADVANCED_FACE ( 'NONE', ( #18091 ), #25994, .T. ) ;
#42956=EDGE_CURVE ( 'NONE', #33912, #35760, #33692, .T. ) ;
#42957=CARTESIAN_POINT ( 'NONE',  ( -21.29196722032537537, -20.70380199363842877, 72.53918572867779346 ) ) ;
#42958=DIRECTION ( 'NONE',  ( 8.339041846367054613E-07, 7.401746001654338994E-06, -0.9999999999722594124 ) ) ;
#42959=VERTEX_POINT ( 'NONE', #10491 ) ;
#42961=EDGE_CURVE ( 'NONE', #10578, #41130, #33430, .T. ) ;
#42962=FACE_OUTER_BOUND ( 'NONE', #17660, .T. ) ;
#42963=ADVANCED_FACE ( 'NONE', ( #41010 ), #211, .T. ) ;
#42964=DIRECTION ( 'NONE',  ( 0.2393415023380396911, -0.9709354485539016810, 6.438601123316501445E-08 ) ) ;
#42965=CARTESIAN_POINT ( 'NONE',  ( -22.58392976434795330, -19.53954411336175667, 72.83503833621796275 ) ) ;
#42966=VERTEX_POINT ( 'NONE', #15864 ) ;
#42967=CARTESIAN_POINT ( 'NONE',  ( -18.53556661698576136, -22.17591588139245573, 72.40015654177148008 ) ) ;
#42969=CARTESIAN_POINT ( 'NONE',  ( -11.32522400900782067, -11.27219014254736074, 60.96413645226084554 ) ) ;
#42970=( BOUNDED_CURVE ( )  B_SPLINE_CURVE ( 3, ( #7557, #18869, #29707, #45728 ),
 .UNSPECIFIED., .F., .F. ) 
 B_SPLINE_CURVE_WITH_KNOTS ( ( 4, 4 ),
 ( 0.5000000000000000000, 0.9074455897393707282 ),
 .UNSPECIFIED. ) 
 CURVE ( )  GEOMETRIC_REPRESENTATION_ITEM ( )  RATIONAL_B_SPLINE_CURVE ( ( 1.000000000000003553, 0.4567392136813279158, 0.3561768502900262146, 0.6983129098261022794 ) ) 
 REPRESENTATION_ITEM ( '' )  );
#42974=DIRECTION ( 'NONE',  ( -0.8356905716187447153, 0.5492005722024784209, 7.728900804118605128E-08 ) ) ;
#42976=LINE ( 'NONE', #31656, #19599 ) ;
#42977=VERTEX_POINT ( 'NONE', #26230 ) ;
#42978=B_SPLINE_CURVE_WITH_KNOTS ( 'NONE', 3,
 ( #27839, #46481, #930, #31445, #34394, #41565, #23336, #30737, #20122, #453 ),
 .UNSPECIFIED., .F., .F.,
 ( 4, 2, 2, 2, 4 ),
 ( 0.6272669072877811169, 0.7522669073073010582, 0.8772669073268211104, 1.002266907346341052, 1.127266907365860993 ),
 .UNSPECIFIED. ) ;
#42979=CARTESIAN_POINT ( 'NONE',  ( -12.10506971550441335, -10.25793058095366561, 67.78280305760789304 ) ) ;
#42980=CYLINDRICAL_SURFACE ( 'NONE', #26625, 0.1500000000000077383 ) ;
#42982=ORIENTED_EDGE ( 'NONE', *, *, #42756, .F. ) ;
#42983=CARTESIAN_POINT ( 'NONE',  ( -20.11870507851999079, -21.33255209822014820, 69.09049654866474555 ) ) ;
#42984=EDGE_LOOP ( 'NONE', ( #21840, #1238, #27284, #23718, #44607 ) ) ;
#42985=ORIENTED_EDGE ( 'NONE', *, *, #38094, .T. ) ;
#42988=CARTESIAN_POINT ( 'NONE',  ( -23.78500266573477262, -11.88707733699690827, 59.78235732566622573 ) ) ;
#42989=CARTESIAN_POINT ( 'NONE',  ( -21.33694788700791278, -9.004934622526002741, 73.60128753634342047 ) ) ;
#42991=CARTESIAN_POINT ( 'NONE',  ( -16.32275379891173372, -22.17735803940487926, 61.95579338972356709 ) ) ;
#42992=ORIENTED_EDGE ( 'NONE', *, *, #36794, .F. ) ;
#42993=ORIENTED_EDGE ( 'NONE', *, *, #41608, .F. ) ;
#42995=CARTESIAN_POINT ( 'NONE',  ( -11.47327410250610313, -11.02222997523968573, 60.77066038170728035 ) ) ;
#42996=CARTESIAN_POINT ( 'NONE',  ( -24.87380742036101466, -14.88762772862374284, 59.36583317909604318 ) ) ;
#42997=CARTESIAN_POINT ( 'NONE',  ( -23.21838898650911531, -18.73703798069015392, 65.82389378437922289 ) ) ;
#43000=VERTEX_POINT ( 'NONE', #41746 ) ;
#43001=CARTESIAN_POINT ( 'NONE',  ( -24.26499789074519597, -17.75976756996305639, 62.65856417960095825 ) ) ;
#43003=CARTESIAN_POINT ( 'NONE',  ( -12.96596534320165794, -9.347742485070138940, 70.84925352874383009 ) ) ;
#43004=CARTESIAN_POINT ( 'NONE',  ( -17.24796809485249227, -7.811422621481736606, 67.12925709854650336 ) ) ;
#43006=VERTEX_POINT ( 'NONE', #8032 ) ;
#43008=B_SPLINE_CURVE_WITH_KNOTS ( 'NONE', 3,
 ( #37992, #8446, #4276, #12377, #30873, #45887, #42679, #23732, #12143, #11911 ),
 .UNSPECIFIED., .F., .F.,
 ( 4, 2, 2, 2, 4 ),
 ( 0.000000000000000000, 0.2500000000000000000, 0.5000000000000000000, 0.7500000000000000000, 1.000000000000000000 ),
 .UNSPECIFIED. ) ;
#43009=CARTESIAN_POINT ( 'NONE',  ( -9.975583786612773451, -14.65598763567812313, 71.44287367974872893 ) ) ;
#43010=CARTESIAN_POINT ( 'NONE',  ( -18.55956930788366677, -7.446158750330262421, 74.02559786541287679 ) ) ;
#43012=EDGE_CURVE ( 'NONE', #43621, #30016, #23711, .T. ) ;
#43013=ORIENTED_EDGE ( 'NONE', *, *, #47323, .T. ) ;
#43014=CARTESIAN_POINT ( 'NONE',  ( -19.62595585458452163, -8.103479577873935469, 60.10526007146324901 ) ) ;
#43015=ADVANCED_FACE ( 'NONE', ( #14869 ), #617, .T. ) ;
#43016=CARTESIAN_POINT ( 'NONE',  ( -22.94084299836913843, -19.11815316549774479, 58.88410675570529662 ) ) ;
#43017=CARTESIAN_POINT ( 'NONE',  ( -20.13087680518396994, -7.868272569338301103, 73.82758314367622177 ) ) ;
#43018=ORIENTED_EDGE ( 'NONE', *, *, #46172, .F. ) ;
#43019=CARTESIAN_POINT ( 'NONE',  ( -19.40930774675918613, -7.628578061947676403, 60.11092995211872392 ) ) ;
#43021=CARTESIAN_POINT ( 'NONE',  ( -14.09914604623946488, -8.649277798895779412, 74.19954655170327840 ) ) ;
#43022=CARTESIAN_POINT ( 'NONE',  ( -9.974235501303020612, -14.86645057852294016, 75.05424837986554110 ) ) ;
#43024=ORIENTED_EDGE ( 'NONE', *, *, #21135, .F. ) ;
#43030=DIRECTION ( 'NONE',  ( -0.3478314405900308492, -0.9375570856950864451, 0.000000000000000000 ) ) ;
#43032=ADVANCED_FACE ( 'NONE', ( #45923 ), #18576, .T. ) ;
#43033=CARTESIAN_POINT ( 'NONE',  ( -20.94477883430487708, -21.37566986424753068, 58.75819861804361466 ) ) ;
#43034=CARTESIAN_POINT ( 'NONE',  ( -23.41700317716350810, -19.23526875778016176, 62.51553421167685087 ) ) ;
#43035=ORIENTED_EDGE ( 'NONE', *, *, #44305, .F. ) ;
#43038=VECTOR ( 'NONE', #8147, 1000.000000000000227 ) ;
#43040=ORIENTED_EDGE ( 'NONE', *, *, #36111, .T. ) ;
#43041=EDGE_LOOP ( 'NONE', ( #4226, #18300 ) ) ;
#43042=CARTESIAN_POINT ( 'NONE',  ( -13.01353397724842154, -8.804979801064929390, 64.09441804368185558 ) ) ;
#43046=CARTESIAN_POINT ( 'NONE',  ( -12.14425506381237518, -10.13739722748950634, 64.32914326607961186 ) ) ;
#43047=CARTESIAN_POINT ( 'NONE',  ( -19.28352822169459202, -22.07505156356299381, 53.49999999999994316 ) ) ;
#43048=CARTESIAN_POINT ( 'NONE',  ( -18.64414733763933896, -7.459617552211802227, 74.00210948319649162 ) ) ;
#43049=CARTESIAN_POINT ( 'NONE',  ( -23.34288328645119037, -19.33377384263253873, 59.06905932422779415 ) ) ;
#43051=VERTEX_POINT ( 'NONE', #42227 ) ;
#43052=CARTESIAN_POINT ( 'NONE',  ( -10.64512080333459387, -11.71903002653516168, 74.81486074884371362 ) ) ;
#43056=CARTESIAN_POINT ( 'NONE',  ( -13.38575581802539993, -9.030060914960570173, 60.72478133471773276 ) ) ;
#43058=ADVANCED_FACE ( 'NONE', ( #45443 ), #13303, .T. ) ;
#43061=CARTESIAN_POINT ( 'NONE',  ( -24.02298749829535751, -11.35118778494372194, 66.52940360090373417 ) ) ;
#43062=CARTESIAN_POINT ( 'NONE',  ( -17.16863824095212010, -7.760122409783657638, 67.02039628079666045 ) ) ;
#43063=CARTESIAN_POINT ( 'NONE',  ( -24.51063837352987207, -17.11019555850099039, 72.99680753360935626 ) ) ;
#43065=CARTESIAN_POINT ( 'NONE',  ( -24.41403469082061051, -14.40519231153102986, 69.76348327924310411 ) ) ;
#43068=CARTESIAN_POINT ( 'NONE',  ( -19.27972737141692861, -8.007758698492196459, 60.26092978174835935 ) ) ;
#43070=EDGE_CURVE ( 'NONE', #37096, #45761, #47378, .T. ) ;
#43071=CARTESIAN_POINT ( 'NONE',  ( -18.67229796221712590, -7.919758957113036679, 73.95137594816235094 ) ) ;
#43072=CARTESIAN_POINT ( 'NONE',  ( -11.35070632453979478, -11.22329048540824559, 57.09414325051740491 ) ) ;
#43073=ADVANCED_FACE ( 'NONE', ( #22533 ), #35330, .T. ) ;
#43075=ORIENTED_EDGE ( 'NONE', *, *, #17440, .T. ) ;
#43076=CARTESIAN_POINT ( 'NONE',  ( -10.49080373283728207, -13.84193255407867262, 57.73208522591303193 ) ) ;
#43077=ORIENTED_EDGE ( 'NONE', *, *, #37674, .T. ) ;
#43078=FACE_OUTER_BOUND ( 'NONE', #603, .T. ) ;
#43079=ADVANCED_FACE ( 'NONE', ( #5045 ), #9476, .T. ) ;
#43081=ORIENTED_EDGE ( 'NONE', *, *, #14290, .T. ) ;
#43082=CARTESIAN_POINT ( 'NONE',  ( -18.46885980906216318, -22.18634193242058572, 68.92859349268570668 ) ) ;
#43083=CARTESIAN_POINT ( 'NONE',  ( -11.42506541550659449, -10.39151053845774442, 74.61601874447606519 ) ) ;
#43084=EDGE_LOOP ( 'NONE', ( #16190, #43964, #17980, #25777, #19891 ) ) ;
#43085=CARTESIAN_POINT ( 'NONE',  ( -15.34465393633500696, -21.54586957516256263, 68.86120835375241711 ) ) ;
#43087=( BOUNDED_CURVE ( )  B_SPLINE_CURVE ( 3, ( #48028, #44120, #25384, #37160 ),
 .UNSPECIFIED., .F., .F. ) 
 B_SPLINE_CURVE_WITH_KNOTS ( ( 4, 4 ),
 ( 0.5000000000000000000, 0.9074455897393596260 ),
 .UNSPECIFIED. ) 
 CURVE ( )  GEOMETRIC_REPRESENTATION_ITEM ( )  RATIONAL_B_SPLINE_CURVE ( ( 1.000000000000005107, 0.4567392136813352987, 0.3561768502900278799, 0.6983129098260882905 ) ) 
 REPRESENTATION_ITEM ( '' )  );
#43088=CARTESIAN_POINT ( 'NONE',  ( -17.61716384397549362, -7.761810361906310796, 63.55057029321027784 ) ) ;
#43089=CARTESIAN_POINT ( 'NONE',  ( -10.90975526000855389, -17.37128585871089825, 64.91274058815852754 ) ) ;
#43090=VERTEX_POINT ( 'NONE', #31869 ) ;
#43091=LINE ( 'NONE', #16238, #38890 ) ;
#43093=CARTESIAN_POINT ( 'NONE',  ( -20.66848101912799862, -8.549761622307149977, 60.12653141481577990 ) ) ;
#43094=CARTESIAN_POINT ( 'NONE',  ( -12.30444741248500051, -20.22242042389802918, 64.98019641849691652 ) ) ;
#43095=ORIENTED_EDGE ( 'NONE', *, *, #29153, .F. ) ;
#43097=CARTESIAN_POINT ( 'NONE',  ( -11.70707196628297986, -18.84868401720091313, 68.51689578196801733 ) ) ;
#43098=CARTESIAN_POINT ( 'NONE',  ( -10.99529498506645275, -17.70292631970418640, 71.86718196782238977 ) ) ;
#43099=VERTEX_POINT ( 'NONE', #13377 ) ;
#43101=CARTESIAN_POINT ( 'NONE',  ( -21.99229891970641404, -20.18939897536854389, 65.84854503242263490 ) ) ;
#43104=CARTESIAN_POINT ( 'NONE',  ( -10.42512874152911628, -14.93649829652840744, 74.79778865176552927 ) ) ;
#43105=AXIS2_PLACEMENT_3D ( 'NONE', #38181, #19479, #27113 ) ;
#43106=EDGE_CURVE ( 'NONE', #35822, #42531, #25435, .T. ) ;
#43107=CARTESIAN_POINT ( 'NONE',  ( -11.01197672498280866, -17.74032467813711378, 71.85246142747085685 ) ) ;
#43108=CARTESIAN_POINT ( 'NONE',  ( -12.31380134045779506, -10.02538898168817916, 60.55918086676557976 ) ) ;
#43109=( BOUNDED_CURVE ( )  B_SPLINE_CURVE ( 3, ( #41162, #29106, #14531, #29591 ),
 .UNSPECIFIED., .F., .F. ) 
 B_SPLINE_CURVE_WITH_KNOTS ( ( 4, 4 ),
 ( 0.9074455897393640669, 1.000000000000000000 ),
 .UNSPECIFIED. ) 
 CURVE ( )  GEOMETRIC_REPRESENTATION_ITEM ( )  RATIONAL_B_SPLINE_CURVE ( ( 0.6983129098260918433, 0.7760317562606970920, 0.8765941196519998480, 1.000000000000000000 ) ) 
 REPRESENTATION_ITEM ( '' )  );
#43110=VECTOR ( 'NONE', #11529, 1000.000000000000114 ) ;
#43112=ADVANCED_FACE ( 'NONE', ( #12665 ), #28716, .T. ) ;
#43113=VERTEX_POINT ( 'NONE', #32115 ) ;
#43114=CARTESIAN_POINT ( 'NONE',  ( -16.52316554273587101, -21.80170452179945073, 65.24036514508233608 ) ) ;
#43116=CARTESIAN_POINT ( 'NONE',  ( -20.73702004518044717, -8.642678983225538403, 60.14125279966339832 ) ) ;
#43117=EDGE_CURVE ( 'NONE', #19371, #43552, #42336, .T. ) ;
#43119=AXIS2_PLACEMENT_3D ( 'NONE', #17750, #32324, #9909 ) ;
#43122=ORIENTED_EDGE ( 'NONE', *, *, #48055, .F. ) ;
#43123=( BOUNDED_SURFACE ( )  B_SPLINE_SURFACE ( 3, 1, ( 
 ( #2431, #2897 ),
 ( #6610, #32699 ),
 ( #43566, #32929 ),
 ( #47971, #14208 ),
 ( #21150, #13963 ),
 ( #21864, #28541 ),
 ( #9826, #29261 ) ),
 .UNSPECIFIED., .T., .F., .F. ) 
 B_SPLINE_SURFACE_WITH_KNOTS ( ( 4, 3, 4 ),
 ( 2, 2 ),
 ( 0.000000000000000000, 0.5000000000000000000, 1.000000000000000000 ),
 ( 0.000000000000000000, 1.000000000000000000 ),
 .UNSPECIFIED. ) 
 GEOMETRIC_REPRESENTATION_ITEM ( )  RATIONAL_B_SPLINE_SURFACE ( (
 ( 1.000000000000000000, 1.000000000000000000),
 ( 0.3333333333333335369, 0.3333333333333330373),
 ( 0.3333333333333335369, 0.3333333333333330373),
 ( 1.000000000000000000, 1.000000000000000000),
 ( 0.3333333333333333703, 0.3333333333333333703),
 ( 0.3333333333333333703, 0.3333333333333333703),
 ( 1.000000000000000000, 1.000000000000000000) ) ) 
 REPRESENTATION_ITEM ( '' )  SURFACE ( )  );
#43124=EDGE_LOOP ( 'NONE', ( #11677, #41156 ) ) ;
#43125=CARTESIAN_POINT ( 'NONE',  ( -11.49500183448702906, -10.99442376238782515, 57.22375354680192316 ) ) ;
#43126=CARTESIAN_POINT ( 'NONE',  ( -22.52837755674526221, -10.01897815596726282, 70.20281741071431725 ) ) ;
#43127=CARTESIAN_POINT ( 'NONE',  ( -21.69182758944758049, -9.260652778598187140, 63.30039755155743109 ) ) ;
#43128=VERTEX_POINT ( 'NONE', #35554 ) ;
#43129=CARTESIAN_POINT ( 'NONE',  ( -10.79923826878429338, -11.40118965656789030, 67.81138754266618207 ) ) ;
#43132=LINE ( 'NONE', #6440, #41780 ) ;
#43134=CARTESIAN_POINT ( 'NONE',  ( -16.97946104448713456, -21.84517140583366057, 72.46543221429990922 ) ) ;
#43137=CARTESIAN_POINT ( 'NONE',  ( -23.34611022102891553, -10.28892344017613958, 59.70865101996992053 ) ) ;
#43138=ORIENTED_EDGE ( 'NONE', *, *, #6420, .F. ) ;
#43139=CARTESIAN_POINT ( 'NONE',  ( -10.60399964645595716, -13.23185723771246280, 71.20828540032704268 ) ) ;
#43141=EDGE_LOOP ( 'NONE', ( #29666, #48707, #30550, #30480, #24432 ) ) ;
#43142=CARTESIAN_POINT ( 'NONE',  ( -11.90827771948429792, -19.81721557328689798, 58.04965466949625608 ) ) ;
#43144=B_SPLINE_CURVE_WITH_KNOTS ( 'NONE', 1,
 ( #32576, #29862 ),
 .UNSPECIFIED., .F., .F.,
 ( 2, 2 ),
 ( 0.000000000000000000, 1.000000000000000000 ),
 .UNSPECIFIED. ) ;
#43147=CARTESIAN_POINT ( 'NONE',  ( -9.975583804105555785, -14.65598652642324673, 71.44287259100559595 ) ) ;
#43149=CARTESIAN_POINT ( 'NONE',  ( -22.22619359738691003, -20.50513629785891823, 58.94938195453792673 ) ) ;
#43150=EDGE_CURVE ( 'NONE', #30656, #2574, #28893, .T. ) ;
#43152=CARTESIAN_POINT ( 'NONE',  ( -24.86242989439883289, -14.39095395922188558, 66.36788051138485400 ) ) ;
#43153=CARTESIAN_POINT ( 'NONE',  ( -10.46835810950011059, -15.59615148508074789, 61.33789074736403535 ) ) ;
#43154=CARTESIAN_POINT ( 'NONE',  ( -13.26872317195175199, -21.05283485551296607, 53.49999999999994316 ) ) ;
#43156=CARTESIAN_POINT ( 'NONE',  ( -17.44177517589205451, -7.809228866840242311, 63.74160293238216468 ) ) ;
#43157=CARTESIAN_POINT ( 'NONE',  ( -24.66525519625502127, -13.05740165471419623, 63.02602501031626048 ) ) ;
#43158=DIRECTION ( 'NONE',  ( -0.3478314405900308492, -0.9375570856950864451, 0.000000000000000000 ) ) ;
#43159=CARTESIAN_POINT ( 'NONE',  ( -17.20139249542113191, -7.812750000685961815, 70.49035839633111777 ) ) ;
#43160=CARTESIAN_POINT ( 'NONE',  ( -19.97882496985426570, -21.80761570639785063, 69.11199379919601427 ) ) ;
#43163=CARTESIAN_POINT ( 'NONE',  ( -16.48749555294751445, -7.817952760528972256, 60.50028745231125527 ) ) ;
#43164=CYLINDRICAL_SURFACE ( 'NONE', #31310, 0.1500000000000047962 ) ;
#43165=ORIENTED_EDGE ( 'NONE', *, *, #25705, .F. ) ;
#43166=FACE_OUTER_BOUND ( 'NONE', #48350, .T. ) ;
#43168=CARTESIAN_POINT ( 'NONE',  ( -12.80657247161177814, -9.477853225175101315, 70.73436560138682694 ) ) ;
#43169=CARTESIAN_POINT ( 'NONE',  ( -23.10898443554464521, -18.97874941859272724, 62.35406906767577340 ) ) ;
#43170=CARTESIAN_POINT ( 'NONE',  ( -21.36489679027069499, -8.963475500412677377, 73.60128753237400190 ) ) ;
#43171=B_SPLINE_CURVE_WITH_KNOTS ( 'NONE', 3,
 ( #17624, #17860, #6802, #17392, #32657, #2380, #13918, #9545, #44250, #32883 ),
 .UNSPECIFIED., .F., .F.,
 ( 4, 2, 2, 2, 4 ),
 ( 0.6272669072782520727, 0.7522669073001176931, 0.8772669073219834246, 1.002266907343849045, 1.127266907365714665 ),
 .UNSPECIFIED. ) ;
#43172=ORIENTED_EDGE ( 'NONE', *, *, #797, .F. ) ;
#43173=CARTESIAN_POINT ( 'NONE',  ( -22.51726247777427403, -19.68384842258191725, 72.94400547081133368 ) ) ;
#43174=EDGE_CURVE ( 'NONE', #14, #28748, #33724, .T. ) ;
#43176=CARTESIAN_POINT ( 'NONE',  ( -21.99213670719075253, -20.17946569659695299, 59.04970794435396897 ) ) ;
#43177=EDGE_CURVE ( 'NONE', #1862, #39476, #36890, .T. ) ;
#43179=ADVANCED_FACE ( 'NONE', ( #32589 ), #18724, .T. ) ;
#43183=CARTESIAN_POINT ( 'NONE',  ( -10.42804297987642670, -12.24802435162854941, 57.45140417473248107 ) ) ;
#43190=VERTEX_POINT ( 'NONE', #33052 ) ;
#43191=EDGE_LOOP ( 'NONE', ( #11209, #20936, #13347, #29677 ) ) ;
#43193=CARTESIAN_POINT ( 'NONE',  ( -21.21873014114744294, -20.75103526016286537, 69.34890365675909152 ) ) ;
#43194=B_SPLINE_CURVE_WITH_KNOTS ( 'NONE', 3,
 ( #17704, #48005, #6883, #7137, #18192, #29292, #14710, #44327, #29782, #10580 ),
 .UNSPECIFIED., .F., .F.,
 ( 4, 2, 2, 2, 4 ),
 ( 0.000000000000000000, 0.2500000000000000000, 0.5000000000000000000, 0.7500000000000000000, 1.000000000000000000 ),
 .UNSPECIFIED. ) ;
#43195=CARTESIAN_POINT ( 'NONE',  ( -12.96596438542217555, -9.347743257243967818, 70.99925352873879092 ) ) ;
#43197=FACE_OUTER_BOUND ( 'NONE', #20720, .T. ) ;
#43198=CARTESIAN_POINT ( 'NONE',  ( -12.06140467229625912, -20.05244645202335008, 53.49999999999994316 ) ) ;
#43199=EDGE_CURVE ( 'NONE', #29130, #2205, #1384, .T. ) ;
#43200=CARTESIAN_POINT ( 'NONE',  ( -10.70532053225239544, -12.67267096592666498, 61.08381491717225487 ) ) ;
#43202=CARTESIAN_POINT ( 'NONE',  ( -20.18792757799173287, -7.890760935853403879, 73.97742500291465717 ) ) ;
#43204=ORIENTED_EDGE ( 'NONE', *, *, #15741, .F. ) ;
#43205=CARTESIAN_POINT ( 'NONE',  ( -22.34470957656571599, -19.78791530553215949, 69.47417989488683077 ) ) ;
#43207=ORIENTED_EDGE ( 'NONE', *, *, #39607, .T. ) ;
#43208=CARTESIAN_POINT ( 'NONE',  ( -24.47354778464749003, -12.39902454472287197, 73.42720984402279782 ) ) ;
#43209=CYLINDRICAL_SURFACE ( 'NONE', #10062, 0.1500000000000045186 ) ;
#43212=CARTESIAN_POINT ( 'NONE',  ( -22.62394951084894146, -10.04809318868971424, 70.29706442286226320 ) ) ;
#43214=AXIS2_PLACEMENT_3D ( 'NONE', #36113, #32440, #2867 ) ;
#43215=CARTESIAN_POINT ( 'NONE',  ( -16.71957921250844592, -21.82421608262117729, 68.71032757591046902 ) ) ;
#43216=CARTESIAN_POINT ( 'NONE',  ( -19.45281838860202228, -9.697037067072807659, 53.49999999999995026 ) ) ;
#43217=ORIENTED_EDGE ( 'NONE', *, *, #27051, .F. ) ;
#43218=FACE_OUTER_BOUND ( 'NONE', #3083, .T. ) ;
#43219=CARTESIAN_POINT ( 'NONE',  ( -10.38215599771421793, -15.21658347440237513, 57.86792906985348850 ) ) ;
#43220=VECTOR ( 'NONE', #9078, 1000.000000000000227 ) ;
#43221=CIRCLE ( 'NONE', #29037, 7.500000000000001776 ) ;
#43223=PLANE ( 'NONE',  #18692 ) ;
#43226=CYLINDRICAL_SURFACE ( 'NONE', #6658, 0.1500000000000026590 ) ;
#43227=CARTESIAN_POINT ( 'NONE',  ( -16.78411603780843464, -21.83009879966275690, 68.84560651669730191 ) ) ;
#43228=ORIENTED_EDGE ( 'NONE', *, *, #40291, .F. ) ;
#43234=CARTESIAN_POINT ( 'NONE',  ( -15.06786346506120822, -21.45763672053845994, 68.66772992167511802 ) ) ;
#43237=ADVANCED_FACE ( 'NONE', ( #48326 ), #10440, .T. ) ;
#43239=ORIENTED_EDGE ( 'NONE', *, *, #8535, .T. ) ;
#43241=CARTESIAN_POINT ( 'NONE',  ( -18.88931992898283241, -7.909354906767774196, 63.43088992718812591 ) ) ;
#43242=CARTESIAN_POINT ( 'NONE',  ( -14.60689809042302834, -8.346551666329650843, 64.08978840692945766 ) ) ;
#43243=( BOUNDED_CURVE ( )  B_SPLINE_CURVE ( 3, ( #27114, #8408, #15283, #45125 ),
 .UNSPECIFIED., .F., .F. ) 
 B_SPLINE_CURVE_WITH_KNOTS ( ( 4, 4 ),
 ( 0.000000000000000000, 0.4074455897393584602 ),
 .UNSPECIFIED. ) 
 CURVE ( )  GEOMETRIC_REPRESENTATION_ITEM ( )  RATIONAL_B_SPLINE_CURVE ( ( 1.000000000000000000, 0.4567392136813362979, 0.3561768502900319322, 0.6983129098260868473 ) ) 
 REPRESENTATION_ITEM ( '' )  );
#43245=CARTESIAN_POINT ( 'NONE',  ( -24.71637841307600425, -13.28356005536694973, 59.50234599550952197 ) ) ;
#43247=ORIENTED_EDGE ( 'NONE', *, *, #33077, .F. ) ;
#43248=VERTEX_POINT ( 'NONE', #14561 ) ;
#43253=CARTESIAN_POINT ( 'NONE',  ( -21.59804090337381410, -20.98026344205569771, 72.70941702861115630 ) ) ;
#43254=DIRECTION ( 'NONE',  ( -0.3566357048164924826, 0.9342435303763381160, -8.054691247152028744E-09 ) ) ;
#43255=CARTESIAN_POINT ( 'NONE',  ( -24.09752231370279318, -16.92234466904679024, 73.07439273860526896 ) ) ;
#43258=AXIS2_PLACEMENT_3D ( 'NONE', #17830, #32852, #6291 ) ;
#43260=CARTESIAN_POINT ( 'NONE',  ( -14.79343629209028244, -21.77935231311171194, 61.82874611184421099 ) ) ;
#43261=EDGE_CURVE ( 'NONE', #4554, #21712, #37808, .T. ) ;
#43262=CARTESIAN_POINT ( 'NONE',  ( -16.33297564533955537, -22.17887142534084433, 61.90568129439025569 ) ) ;
#43263=CARTESIAN_POINT ( 'NONE',  ( -24.39763799706551950, -15.84669482609578317, 69.54779622430707775 ) ) ;
#43267=( BOUNDED_CURVE ( )  B_SPLINE_CURVE ( 3, ( #27636, #17005, #46356, #12847 ),
 .UNSPECIFIED., .F., .F. ) 
 B_SPLINE_CURVE_WITH_KNOTS ( ( 4, 4 ),
 ( 0.5000000000000000000, 0.9074455897393693959 ),
 .UNSPECIFIED. ) 
 CURVE ( )  GEOMETRIC_REPRESENTATION_ITEM ( )  RATIONAL_B_SPLINE_CURVE ( ( 1.000000000000035749, 0.4567392136813320791, 0.3561768502900052313, 0.6983129098260940637 ) ) 
 REPRESENTATION_ITEM ( '' )  );
#43268=CARTESIAN_POINT ( 'NONE',  ( -10.36968235478426870, -15.03336378326449285, 71.48349971081816534 ) ) ;
#43269=CARTESIAN_POINT ( 'NONE',  ( -11.02439547600630831, -11.97273370266293036, 74.85840233422536016 ) ) ;
#43270=CARTESIAN_POINT ( 'NONE',  ( -24.47390369988710290, -14.86621679291170928, 59.24300234023566247 ) ) ;
#43271=ORIENTED_EDGE ( 'NONE', *, *, #46225, .T. ) ;
#43273=CARTESIAN_POINT ( 'NONE',  ( -11.46043843694620179, -11.04924462883820802, 57.50903212149482613 ) ) ;
#43276=VERTEX_POINT ( 'NONE', #14811 ) ;
#43277=CARTESIAN_POINT ( 'NONE',  ( -11.73187771999763740, -10.73495407577211580, 74.66558189934212919 ) ) ;
#43278=CARTESIAN_POINT ( 'NONE',  ( -9.973358241295501969, -14.79494948476079941, 74.98434255746357735 ) ) ;
#43279=EDGE_LOOP ( 'NONE', ( #5392, #8759, #2815, #18955, #48653 ) ) ;
#43280=CARTESIAN_POINT ( 'NONE',  ( -17.39761409878557785, -7.809256622337199971, 67.02039592144427615 ) ) ;
#43281=CARTESIAN_POINT ( 'NONE',  ( -10.76785811675246940, -12.48515291162924434, 57.61385273545094066 ) ) ;
#43282=B_SPLINE_CURVE_WITH_KNOTS ( 'NONE', 1,
 ( #1229, #23173 ),
 .UNSPECIFIED., .F., .F.,
 ( 2, 2 ),
 ( 0.000000000000000000, 1.000000000000000000 ),
 .UNSPECIFIED. ) ;
#43284=CARTESIAN_POINT ( 'NONE',  ( -12.26752988409003642, -16.72227946798956921, 53.49899999999994549 ) ) ;
#43286=CARTESIAN_POINT ( 'NONE',  ( -24.17969144601942233, -17.95015662838525117, 59.04732501252154009 ) ) ;
#43287=CARTESIAN_POINT ( 'NONE',  ( -10.85795890819061427, -18.96892932606922244, 54.30803469517866944 ) ) ;
#43288=B_SPLINE_CURVE_WITH_KNOTS ( 'NONE', 1,
 ( #46726, #5614 ),
 .UNSPECIFIED., .F., .F.,
 ( 2, 2 ),
 ( 0.000000000000000000, 1.000000000000000000 ),
 .UNSPECIFIED. ) ;
#43289=CARTESIAN_POINT ( 'NONE',  ( -11.50273385864769438, -11.07591097799543256, 57.50903212538073461 ) ) ;
#43291=CARTESIAN_POINT ( 'NONE',  ( -10.61061218858606914, -11.79566089880681545, 74.69693755219159925 ) ) ;
#43293=EDGE_CURVE ( 'NONE', #29409, #9616, #18339, .T. ) ;
#43294=ORIENTED_EDGE ( 'NONE', *, *, #7330, .F. ) ;
#43295=ORIENTED_EDGE ( 'NONE', *, *, #42221, .T. ) ;
#43297=FACE_OUTER_BOUND ( 'NONE', #29483, .T. ) ;
#43298=CARTESIAN_POINT ( 'NONE',  ( -13.18473975798692877, -20.93551490194142062, 58.23145353898504339 ) ) ;
#43301=CARTESIAN_POINT ( 'NONE',  ( -12.29586577630491995, -9.966054570304006432, 64.32914351779317030 ) ) ;
#43302=CARTESIAN_POINT ( 'NONE',  ( -19.54382994836049292, -21.48060488537790746, 62.06791645429107263 ) ) ;
#43303=CARTESIAN_POINT ( 'NONE',  ( -23.62389146642398075, -18.18225743695742835, 72.91935080803692415 ) ) ;
#43305=B_SPLINE_CURVE_WITH_KNOTS ( 'NONE', 3,
 ( #18113, #6710, #14784, #14536, #13830, #7209, #36709, #33263, #25654, #33505 ),
 .UNSPECIFIED., .F., .F.,
 ( 4, 2, 2, 2, 4 ),
 ( 0.6272669072878462870, 0.7522669073073414703, 0.8772669073268366535, 1.002266907346331948, 1.127266907365827020 ),
 .UNSPECIFIED. ) ;
#43307=CARTESIAN_POINT ( 'NONE',  ( -11.26201241829012822, -11.37794026804562009, 68.03353368067536167 ) ) ;
#43308=VERTEX_POINT ( 'NONE', #8203 ) ;
#43309=ORIENTED_EDGE ( 'NONE', *, *, #39671, .F. ) ;
#43310=EDGE_CURVE ( 'NONE', #8530, #33575, #40364, .T. ) ;
#43311=CARTESIAN_POINT ( 'NONE',  ( -10.58771178721467798, -11.84651422905517926, 74.67185031923813199 ) ) ;
#43315=CARTESIAN_POINT ( 'NONE',  ( -20.62633693628556486, -21.09014860362536226, 58.65034946679929817 ) ) ;
#43316=CARTESIAN_POINT ( 'NONE',  ( -22.42700247402090241, -19.70584170416704595, 72.92783938554663337 ) ) ;
#43317=DIRECTION ( 'NONE',  ( 0.4501286257827957216, 0.8929637284072022840, -1.500157796035321876E-08 ) ) ;
#43318=ADVANCED_FACE ( 'NONE', ( #48577 ), #4259, .F. ) ;
#43319=ORIENTED_EDGE ( 'NONE', *, *, #43935, .T. ) ;
#43320=CARTESIAN_POINT ( 'NONE',  ( -20.10179291524702805, -21.76144317846600629, 72.66124644823618439 ) ) ;
#43321=CARTESIAN_POINT ( 'NONE',  ( -10.21764033814386963, -12.91954908504599331, 67.92327745040803677 ) ) ;
#43325=ORIENTED_EDGE ( 'NONE', *, *, #8088, .F. ) ;
#43327=CARTESIAN_POINT ( 'NONE',  ( -17.00410685006708178, -7.771727545396207582, 73.96018273221115180 ) ) ;
#43328=B_SPLINE_CURVE_WITH_KNOTS ( 'NONE', 1,
 ( #9584, #5876 ),
 .UNSPECIFIED., .F., .F.,
 ( 2, 2 ),
 ( 0.000000000000000000, 1.000000000000000000 ),
 .UNSPECIFIED. ) ;
#43329=CARTESIAN_POINT ( 'NONE',  ( -17.65006842549283306, -20.30456235612523841, 54.07175714974878389 ) ) ;
#43330=CARTESIAN_POINT ( 'NONE',  ( -22.37880076751769920, -9.788815724235030657, 73.68981091303635367 ) ) ;
#43332=DIRECTION ( 'NONE',  ( 1.077913161596394792E-05, -7.121115469840252016E-06, -0.9999999999165499753 ) ) ;
#43333=CARTESIAN_POINT ( 'NONE',  ( -14.79267687185098268, -7.839273151334183787, 56.97187263562120307 ) ) ;
#43335=ORIENTED_EDGE ( 'NONE', *, *, #5615, .F. ) ;
#43336=CARTESIAN_POINT ( 'NONE',  ( -20.36206934058443352, -7.962967395703286044, 70.35126086822562286 ) ) ;
#43338=CARTESIAN_POINT ( 'NONE',  ( -11.30839666586712688, -19.06371641305695519, 68.41700838957257247 ) ) ;
#43339=VERTEX_POINT ( 'NONE', #37231 ) ;
#43340=CARTESIAN_POINT ( 'NONE',  ( -16.32745258320347759, -21.77369344365219561, 61.77040269689842944 ) ) ;
#43342=B_SPLINE_CURVE_WITH_KNOTS ( 'NONE', 1,
 ( #28830, #43876 ),
 .UNSPECIFIED., .F., .F.,
 ( 2, 2 ),
 ( 0.000000000000000000, 1.000000000000000000 ),
 .UNSPECIFIED. ) ;
#43343=ORIENTED_EDGE ( 'NONE', *, *, #40676, .F. ) ;
#43345=( BOUNDED_CURVE ( )  B_SPLINE_CURVE ( 3, ( #16660, #41820, #8095, #4378 ),
 .UNSPECIFIED., .F., .F. ) 
 B_SPLINE_CURVE_WITH_KNOTS ( ( 4, 4 ),
 ( 0.5000000000000000000, 0.9074455897393636228 ),
 .UNSPECIFIED. ) 
 CURVE ( )  GEOMETRIC_REPRESENTATION_ITEM ( )  RATIONAL_B_SPLINE_CURVE ( ( 0.9999999999999772404, 0.4567392136813265835, 0.3561768502900441447, 0.6983129098261050549 ) ) 
 REPRESENTATION_ITEM ( '' )  );
#43347=CARTESIAN_POINT ( 'NONE',  ( -24.05845721068777010, -12.57644527891515551, 73.54225570276561541 ) ) ;
#43348=CARTESIAN_POINT ( 'NONE',  ( -16.29919166237813144, -22.17386956490665639, 62.01214078850637890 ) ) ;
#43350=DIRECTION ( 'NONE',  ( 1.411223637948141806E-06, 4.279116285847032870E-06, 0.9999999999898486758 ) ) ;
#43351=CARTESIAN_POINT ( 'NONE',  ( -10.81230840161673790, -17.25685697075765646, 64.64211442681141762 ) ) ;
#43352=CARTESIAN_POINT ( 'NONE',  ( -12.41315173547891959, -9.850077678253004621, 57.38935532239157311 ) ) ;
#43353=AXIS2_PLACEMENT_3D ( 'NONE', #5589, #21079, #12719 ) ;
#43354=CARTESIAN_POINT ( 'NONE',  ( -12.26752988409003642, -16.72227946798956921, 54.07175714974876968 ) ) ;
#43355=ORIENTED_EDGE ( 'NONE', *, *, #10890, .T. ) ;
#43356=ORIENTED_EDGE ( 'NONE', *, *, #46058, .F. ) ;
#43358=CARTESIAN_POINT ( 'NONE',  ( -24.09792875595538320, -17.08130417324981565, 72.88336032035921619 ) ) ;
#43359=CARTESIAN_POINT ( 'NONE',  ( -22.11771078617523401, -17.70194497944557455, 53.88362224778187226 ) ) ;
#43360=ORIENTED_EDGE ( 'NONE', *, *, #43177, .F. ) ;
#43361=CARTESIAN_POINT ( 'NONE',  ( -24.32752865423570654, -15.96790753223159598, 66.36324927017490438 ) ) ;
#43362=CARTESIAN_POINT ( 'NONE',  ( -23.25771167494501412, -18.77452406822311559, 62.35406629416942081 ) ) ;
#43364=CARTESIAN_POINT ( 'NONE',  ( -23.81923673697547272, -10.98750725051906585, 73.55531620916923430 ) ) ;
#43366=CARTESIAN_POINT ( 'NONE',  ( -12.26902398874117495, -19.54473763108856943, 58.22682373989366766 ) ) ;
#43368=ORIENTED_EDGE ( 'NONE', *, *, #19904, .T. ) ;
#43369=CARTESIAN_POINT ( 'NONE',  ( -14.90981300391231024, -21.39562377109201208, 61.63600440604547970 ) ) ;
#43370=EDGE_CURVE ( 'NONE', #34219, #33529, #45419, .T. ) ;
#43372=CARTESIAN_POINT ( 'NONE',  ( -12.52712847051791378, -9.194636617869647921, 74.36277061998997340 ) ) ;
#43373=CARTESIAN_POINT ( 'NONE',  ( -13.54291793993416348, -20.63484089686539846, 61.81646374971770541 ) ) ;
#43374=ADVANCED_FACE ( 'NONE', ( #30617 ), #11395, .T. ) ;
#43377=EDGE_CURVE ( 'NONE', #24336, #29465, #39555, .T. ) ;
#43379=DIRECTION ( 'NONE',  ( 0.6205284308219183309, 0.7841839494287597967, -8.002013567987250328E-17 ) ) ;
#43380=CARTESIAN_POINT ( 'NONE',  ( -18.53201708017407157, -7.846807123103141102, 74.14064401780551350 ) ) ;
#43382=ORIENTED_EDGE ( 'NONE', *, *, #29669, .F. ) ;
#43383=EDGE_CURVE ( 'NONE', #10750, #47624, #7235, .T. ) ;
#43384=CARTESIAN_POINT ( 'NONE',  ( -15.68502974777997316, -7.977065180327442384, 70.90989839958919561 ) ) ;
#43386=CARTESIAN_POINT ( 'NONE',  ( -10.43298842381219238, -15.77843866184169208, 57.72359922229868801 ) ) ;
#43387=EDGE_LOOP ( 'NONE', ( #27241, #18695, #41669, #8411, #16218 ) ) ;
#43390=CARTESIAN_POINT ( 'NONE',  ( -12.54407977911866290, -20.43842634917980661, 71.90630053519338105 ) ) ;
#43392=( BOUNDED_CURVE ( )  B_SPLINE_CURVE ( 3, ( #46883, #46654, #13123, #28174 ),
 .UNSPECIFIED., .F., .F. ) 
 B_SPLINE_CURVE_WITH_KNOTS ( ( 4, 4 ),
 ( 0.9074455897393605142, 1.000000000000000000 ),
 .UNSPECIFIED. ) 
 CURVE ( )  GEOMETRIC_REPRESENTATION_ITEM ( )  RATIONAL_B_SPLINE_CURVE ( ( 0.6983129098260745238, 0.7760317562606822150, 0.8765941196519907441, 1.000000000000000000 ) ) 
 REPRESENTATION_ITEM ( '' )  );
#43393=CARTESIAN_POINT ( 'NONE',  ( -23.38410589725464916, -10.33907962427212190, 59.71708035543083071 ) ) ;
#43395=CARTESIAN_POINT ( 'NONE',  ( -10.56492483649129710, -13.18000429128331596, 71.50828586225091499 ) ) ;
#43397=CARTESIAN_POINT ( 'NONE',  ( -11.91924650590474855, -19.82915612511634862, 58.12020671644349790 ) ) ;
#43402=CARTESIAN_POINT ( 'NONE',  ( -24.68275054790482770, -16.48720572190336853, 59.23837039904986312 ) ) ;
#43405=ADVANCED_FACE ( 'NONE', ( #37476 ), #22239, .T. ) ;
#43406=CARTESIAN_POINT ( 'NONE',  ( -17.73224099643095286, -22.30287356026373047, 54.27966884056655061 ) ) ;
#43410=( BOUNDED_CURVE ( )  B_SPLINE_CURVE ( 3, ( #41963, #23251, #8004, #30162 ),
 .UNSPECIFIED., .F., .F. ) 
 B_SPLINE_CURVE_WITH_KNOTS ( ( 4, 4 ),
 ( 0.9074455897393632897, 1.000000000000000000 ),
 .UNSPECIFIED. ) 
 CURVE ( )  GEOMETRIC_REPRESENTATION_ITEM ( )  RATIONAL_B_SPLINE_CURVE ( ( 0.6983129098260799639, 0.7760317562606869890, 0.8765941196519936307, 1.000000000000000000 ) ) 
 REPRESENTATION_ITEM ( '' )  );
#43411=CARTESIAN_POINT ( 'NONE',  ( -24.42668993457695592, -13.99045928592870780, 73.40799407547365263 ) ) ;
#43412=CARTESIAN_POINT ( 'NONE',  ( -11.84391856442395863, -19.03561180790773832, 71.97220474003518120 ) ) ;
#43414=CYLINDRICAL_SURFACE ( 'NONE', #28941, 0.1500000000000028533 ) ;
#43419=CARTESIAN_POINT ( 'NONE',  ( -24.83245720896766073, -15.59649170587275258, 73.04657806100746598 ) ) ;
#43420=VERTEX_POINT ( 'NONE', #31083 ) ;
#43421=CARTESIAN_POINT ( 'NONE',  ( -11.29385091374517458, -19.04286921470785288, 68.33194352083310719 ) ) ;
#43423=CARTESIAN_POINT ( 'NONE',  ( -14.50361122469707986, -8.447475796767067280, 63.86266978723202925 ) ) ;
#43424=CARTESIAN_POINT ( 'NONE',  ( -13.71338950266841472, -20.80363499509022773, 64.98628881289567971 ) ) ;
#43425=DIRECTION ( 'NONE',  ( 1.066846710266752623E-06, -9.113387007412332089E-06, -0.9999999999579038956 ) ) ;
#43427=EDGE_CURVE ( 'NONE', #30899, #48422, #6060, .T. ) ;
#43429=CARTESIAN_POINT ( 'NONE',  ( -22.63008543824757979, -10.12971389395683097, 70.01178520543939499 ) ) ;
#43430=ORIENTED_EDGE ( 'NONE', *, *, #38739, .F. ) ;
#43431=CARTESIAN_POINT ( 'NONE',  ( -15.50784783684063051, -8.076599273749138774, 74.07985659288991087 ) ) ;
#43433=CARTESIAN_POINT ( 'NONE',  ( -12.23220172533774885, -19.57856247689574403, 57.92682373937842044 ) ) ;
#43434=CARTESIAN_POINT ( 'NONE',  ( -24.18334793769576407, -17.94238558166073716, 59.12565671406948553 ) ) ;
#43435=CARTESIAN_POINT ( 'NONE',  ( -11.10681587527927938, -11.67891925637714223, 71.10332952723315714 ) ) ;
#43436=CARTESIAN_POINT ( 'NONE',  ( -16.55445166459533368, -21.75508766523052628, 65.22564429726746482 ) ) ;
#43438=ORIENTED_EDGE ( 'NONE', *, *, #44259, .T. ) ;
#43440=EDGE_CURVE ( 'NONE', #3060, #46704, #14843, .T. ) ;
#43442=EDGE_CURVE ( 'NONE', #45009, #26785, #23793, .T. ) ;
#43443=CARTESIAN_POINT ( 'NONE',  ( -15.17160733334415212, -8.120315110694912519, 74.23552617732688930 ) ) ;
#43444=ADVANCED_FACE ( 'NONE', ( #34776 ), #9166, .F. ) ;
#43445=CARTESIAN_POINT ( 'NONE',  ( -20.00946575929301474, -8.250368826910309039, 74.02096600124984604 ) ) ;
#43446=CARTESIAN_POINT ( 'NONE',  ( -14.03825670519393753, -20.93587830947642914, 68.56511064978960235 ) ) ;
#43448=CARTESIAN_POINT ( 'NONE',  ( -19.31536540323461182, -22.01519918219321781, 58.71845705497510437 ) ) ;
#43449=CARTESIAN_POINT ( 'NONE',  ( -10.40888613812686359, -14.10966362093629378, 61.06821293886368807 ) ) ;
#43450=ORIENTED_EDGE ( 'NONE', *, *, #24228, .T. ) ;
#43453=DIRECTION ( 'NONE',  ( -0.9789991564298998750, -0.2038642972899922245, 4.410747590293501250E-08 ) ) ;
#43454=ADVANCED_FACE ( 'NONE', ( #13074 ), #1690, .T. ) ;
#43455=( BOUNDED_CURVE ( )  B_SPLINE_CURVE ( 3, ( #41433, #11643, #46110, #23724 ),
 .UNSPECIFIED., .F., .F. ) 
 B_SPLINE_CURVE_WITH_KNOTS ( ( 4, 4 ),
 ( 0.000000000000000000, 0.4074455897393601256 ),
 .UNSPECIFIED. ) 
 CURVE ( )  GEOMETRIC_REPRESENTATION_ITEM ( )  RATIONAL_B_SPLINE_CURVE ( ( 1.000000000000000000, 0.4567392136813438475, 0.3561768502900347078, 0.6983129098260726364 ) ) 
 REPRESENTATION_ITEM ( '' )  );
#43456=VERTEX_POINT ( 'NONE', #39189 ) ;
#43458=CARTESIAN_POINT ( 'NONE',  ( -10.40277073914389661, -15.44443991871667343, 57.56792809063193772 ) ) ;
#43459=ADVANCED_FACE ( 'NONE', ( #23717 ), #16042, .T. ) ;
#43461=EDGE_CURVE ( 'NONE', #44694, #4434, #5477, .T. ) ;
#43462=LINE ( 'NONE', #1336, #46648 ) ;
#43467=CARTESIAN_POINT ( 'NONE',  ( -14.36817892824948473, -8.455618309860652104, 67.54503025475186462 ) ) ;
#43468=CARTESIAN_POINT ( 'NONE',  ( -22.33041860316855320, -20.41560964288588664, 62.34943852502606632 ) ) ;
#43469=CARTESIAN_POINT ( 'NONE',  ( -11.05034076241727625, -11.79557573020262318, 71.37388789199357575 ) ) ;
#43470=CARTESIAN_POINT ( 'NONE',  ( -11.29385027892729987, -19.04286830487734861, 68.33194243210506613 ) ) ;
#43472=B_SPLINE_CURVE_WITH_KNOTS ( 'NONE', 3,
 ( #31359, #12880, #46390, #31612, #20283, #38499, #23254, #46636, #4525, #27183 ),
 .UNSPECIFIED., .F., .F.,
 ( 4, 2, 2, 2, 4 ),
 ( 0.000000000000000000, 0.2500000000000000000, 0.5000000000000000000, 0.7500000000000000000, 1.000000000000000000 ),
 .UNSPECIFIED. ) ;
#43473=CARTESIAN_POINT ( 'NONE',  ( -20.32146343473794303, -8.373352561929221949, 73.86529255602565058 ) ) ;
#43474=CARTESIAN_POINT ( 'NONE',  ( -11.44117050972369221, -11.17454573989694921, 60.96269276219595667 ) ) ;
#43475=B_SPLINE_CURVE_WITH_KNOTS ( 'NONE', 1,
 ( #43502, #20841 ),
 .UNSPECIFIED., .F., .F.,
 ( 2, 2 ),
 ( 0.000000000000000000, 1.000000000000000000 ),
 .UNSPECIFIED. ) ;
#43476=CARTESIAN_POINT ( 'NONE',  ( -16.16221056564778991, -7.466773990862017207, 60.24382527849350311 ) ) ;
#43477=CARTESIAN_POINT ( 'NONE',  ( -23.46260449798628045, -11.17067817067885649, 73.51193301756617871 ) ) ;
#43478=ORIENTED_EDGE ( 'NONE', *, *, #36128, .F. ) ;
#43480=CARTESIAN_POINT ( 'NONE',  ( -20.09379292320953425, -21.76456661724738950, 72.58291472526767052 ) ) ;
#43481=CARTESIAN_POINT ( 'NONE',  ( -13.26872317195175199, -21.05283485551296607, 47.99999999999994316 ) ) ;
#43482=ORIENTED_EDGE ( 'NONE', *, *, #13189, .T. ) ;
#43483=CARTESIAN_POINT ( 'NONE',  ( -19.86401518824997225, -21.42384811948916834, 69.22010401872219632 ) ) ;
#43484=ORIENTED_EDGE ( 'NONE', *, *, #8134, .T. ) ;
#43486=ORIENTED_EDGE ( 'NONE', *, *, #27622, .T. ) ;
#43488=B_SPLINE_CURVE_WITH_KNOTS ( 'NONE', 3,
 ( #16107, #12681, #27702, #42733, #39752, #42965, #2325, #2573, #12915, #39999 ),
 .UNSPECIFIED., .F., .F.,
 ( 4, 2, 2, 2, 4 ),
 ( 0.000000000000000000, 0.2500000000000000000, 0.5000000000000000000, 0.7500000000000000000, 1.000000000000000000 ),
 .UNSPECIFIED. ) ;
#43489=CARTESIAN_POINT ( 'NONE',  ( -17.42409385541300892, -14.80920654474439679, 47.99999999999994316 ) ) ;
#43490=DIRECTION ( 'NONE',  ( 0.9640890753730593232, -0.2655790932026004803, 6.310348465037888425E-08 ) ) ;
#43493=CARTESIAN_POINT ( 'NONE',  ( -22.72031779163844689, -16.29245029320677673, 53.49999999999995026 ) ) ;
#43494=VERTEX_POINT ( 'NONE', #14268 ) ;
#43495=ORIENTED_EDGE ( 'NONE', *, *, #47646, .T. ) ;
#43497=EDGE_CURVE ( 'NONE', #40716, #29465, #14234, .T. ) ;
#43498=CARTESIAN_POINT ( 'NONE',  ( -21.06634951290973845, -21.30826427787840771, 62.29966696806321380 ) ) ;
#43499=CARTESIAN_POINT ( 'NONE',  ( -24.09293239453862512, -16.93698224962508547, 72.95624128829483368 ) ) ;
#43501=ORIENTED_EDGE ( 'NONE', *, *, #17824, .F. ) ;
#43502=CARTESIAN_POINT ( 'NONE',  ( -10.37382936219775154, -14.83089353207902228, 74.81251018390588570 ) ) ;
#43503=B_SPLINE_CURVE_WITH_KNOTS ( 'NONE', 3,
 ( #42861, #1010, #23421, #27104, #20456, #46318, #12572, #4704, #9375, #9131 ),
 .UNSPECIFIED., .F., .F.,
 ( 4, 2, 2, 2, 4 ),
 ( 0.000000000000000000, 0.2500000000000000000, 0.5000000000000000000, 0.7500000000000000000, 1.000000000000000000 ),
 .UNSPECIFIED. ) ;
#43504=LINE ( 'NONE', #28482, #32320 ) ;
#43505=VERTEX_POINT ( 'NONE', #13788 ) ;
#43506=LINE ( 'NONE', #32644, #9973 ) ;
#43507=CARTESIAN_POINT ( 'NONE',  ( -10.72552571836178181, -12.61109718544098790, 60.79853568372240602 ) ) ;
#43508=CARTESIAN_POINT ( 'NONE',  ( -20.78299823145727387, -8.610459808214880439, 59.85597358678664648 ) ) ;
#43509=ADVANCED_FACE ( 'NONE', ( #47324 ), #6433, .T. ) ;
#43510=EDGE_CURVE ( 'NONE', #4674, #37124, #46548, .T. ) ;
#43511=CARTESIAN_POINT ( 'NONE',  ( -18.85724798917316392, -7.906108138700305155, 67.18599644112759961 ) ) ;
#43512=VECTOR ( 'NONE', #44713, 1000.000000000000114 ) ;
#43513=ORIENTED_EDGE ( 'NONE', *, *, #45159, .F. ) ;
#43514=DIRECTION ( 'NONE',  ( -0.9000732436326450703, -0.4357386327795698677, 2.072980810273451787E-08 ) ) ;
#43515=CARTESIAN_POINT ( 'NONE',  ( -22.75539019595755263, -10.19575032747719590, 66.82710158566565894 ) ) ;
#43521=EDGE_CURVE ( 'NONE', #41728, #2374, #17725, .T. ) ;
#43522=EDGE_CURVE ( 'NONE', #29624, #8171, #24825, .T. ) ;
#43523=CARTESIAN_POINT ( 'NONE',  ( -10.37051006938303388, -14.56035623187037942, 74.94211941000891386 ) ) ;
#43524=ORIENTED_EDGE ( 'NONE', *, *, #30844, .T. ) ;
#43525=FACE_OUTER_BOUND ( 'NONE', #15578, .T. ) ;
#43526=CARTESIAN_POINT ( 'NONE',  ( -21.88020070643341697, -20.20778541568678932, 58.76442927266135285 ) ) ;
#43527=CARTESIAN_POINT ( 'NONE',  ( -24.46557908765160860, -17.24254831546467415, 73.13981945087590475 ) ) ;
#43528=CARTESIAN_POINT ( 'NONE',  ( -21.20587034079417776, -21.22798937808393660, 65.78465149344722818 ) ) ;
#43529=ORIENTED_EDGE ( 'NONE', *, *, #39547, .T. ) ;
#43530=CARTESIAN_POINT ( 'NONE',  ( -21.94239013569476171, -20.22099906679998327, 58.76442899523448204 ) ) ;
#43532=( BOUNDED_CURVE ( )  B_SPLINE_CURVE ( 3, ( #14840, #14354, #8001, #22509 ),
 .UNSPECIFIED., .F., .F. ) 
 B_SPLINE_CURVE_WITH_KNOTS ( ( 4, 4 ),
 ( 0.4074455897393626236, 0.5000000000000000000 ),
 .UNSPECIFIED. ) 
 CURVE ( )  GEOMETRIC_REPRESENTATION_ITEM ( )  RATIONAL_B_SPLINE_CURVE ( ( 0.6983129098260836276, 0.7760317562606876551, 0.8765941196519922984, 0.9999999999999961142 ) ) 
 REPRESENTATION_ITEM ( '' )  );
#43533=CARTESIAN_POINT ( 'NONE',  ( -14.78754716229542865, -8.270772359302402066, 60.31996282000578447 ) ) ;
#43534=CARTESIAN_POINT ( 'NONE',  ( -23.42532328873747005, -19.22384396101403681, 62.46911485589509994 ) ) ;
#43535=EDGE_LOOP ( 'NONE', ( #41293, #30133 ) ) ;
#43537=CARTESIAN_POINT ( 'NONE',  ( -24.25486363958986757, -13.06355980472538292, 63.11792038370487035 ) ) ;
#43538=EDGE_CURVE ( 'NONE', #21212, #22802, #6720, .T. ) ;
#43539=ORIENTED_EDGE ( 'NONE', *, *, #25234, .F. ) ;
#43540=ORIENTED_EDGE ( 'NONE', *, *, #42091, .T. ) ;
#43541=CARTESIAN_POINT ( 'NONE',  ( -20.66696855643225561, -21.06909979829504209, 58.94475164909854925 ) ) ;
#43542=FACE_OUTER_BOUND ( 'NONE', #26286, .T. ) ;
#43543=CARTESIAN_POINT ( 'NONE',  ( -10.02022215050942577, -15.63848034003142295, 61.17755693646328297 ) ) ;
#43545=CARTESIAN_POINT ( 'NONE',  ( -21.89218479126588335, -8.847617444388541585, 66.83866863626586508 ) ) ;
#43546=CARTESIAN_POINT ( 'NONE',  ( -24.41553149706675896, -15.71832598455623398, 69.81835354388927328 ) ) ;
#43547=( BOUNDED_CURVE ( )  B_SPLINE_CURVE ( 3, ( #17473, #32502, #31778, #39156 ),
 .UNSPECIFIED., .F., .F. ) 
 B_SPLINE_CURVE_WITH_KNOTS ( ( 4, 4 ),
 ( 0.000000000000000000, 0.4074455897393658987 ),
 .UNSPECIFIED. ) 
 CURVE ( )  GEOMETRIC_REPRESENTATION_ITEM ( )  RATIONAL_B_SPLINE_CURVE ( ( 1.000000000000000000, 0.4567392136813347991, 0.3561768502900313216, 0.6983129098260896228 ) ) 
 REPRESENTATION_ITEM ( '' )  );
#43549=CARTESIAN_POINT ( 'NONE',  ( -10.13258936719380898, -16.33817337277914561, 71.63245765104117879 ) ) ;
#43550=( BOUNDED_CURVE ( )  B_SPLINE_CURVE ( 3, ( #10432, #10903, #45145, #26175 ),
 .UNSPECIFIED., .F., .F. ) 
 B_SPLINE_CURVE_WITH_KNOTS ( ( 4, 4 ),
 ( 0.4074455897393624570, 0.5000000000000000000 ),
 .UNSPECIFIED. ) 
 CURVE ( )  GEOMETRIC_REPRESENTATION_ITEM ( )  RATIONAL_B_SPLINE_CURVE ( ( 0.6983129098261117162, 0.7760317562607033093, 0.8765941196519960732, 0.9999999999999825695 ) ) 
 REPRESENTATION_ITEM ( '' )  );
#43551=CARTESIAN_POINT ( 'NONE',  ( -18.95165573079047761, -7.922886716408846119, 70.67068327992531351 ) ) ;
#43552=VERTEX_POINT ( 'NONE', #13555 ) ;
#43553=EDGE_LOOP ( 'NONE', ( #18702, #47469 ) ) ;
#43554=CARTESIAN_POINT ( 'NONE',  ( -24.39416267077224987, -15.91966209353573802, 73.14736799148198543 ) ) ;
#43555=VECTOR ( 'NONE', #29216, 1000.000000000000000 ) ;
#43556=CARTESIAN_POINT ( 'NONE',  ( -21.91034708787274710, -20.18261625685872218, 59.06442899735736773 ) ) ;
#43557=CARTESIAN_POINT ( 'NONE',  ( -19.93475561761363934, -21.40553454266635569, 65.62053285436006433 ) ) ;
#43558=CARTESIAN_POINT ( 'NONE',  ( -13.41424841794075462, -8.530288970272771110, 57.22613703607469660 ) ) ;
#43559=CARTESIAN_POINT ( 'NONE',  ( -13.54823083431842612, -20.69819501703281617, 61.66646323538943619 ) ) ;
#43561=( BOUNDED_CURVE ( )  B_SPLINE_CURVE ( 3, ( #22603, #48447, #16098, #37601 ),
 .UNSPECIFIED., .F., .F. ) 
 B_SPLINE_CURVE_WITH_KNOTS ( ( 4, 4 ),
 ( 0.9074455897393652881, 1.000000000000000000 ),
 .UNSPECIFIED. ) 
 CURVE ( )  GEOMETRIC_REPRESENTATION_ITEM ( )  RATIONAL_B_SPLINE_CURVE ( ( 0.6983129098260858481, 0.7760317562606919850, 0.8765941196519967393, 1.000000000000000000 ) ) 
 REPRESENTATION_ITEM ( '' )  );
#43562=VERTEX_POINT ( 'NONE', #502 ) ;
#43565=CARTESIAN_POINT ( 'NONE',  ( -17.63866254341385442, -7.362211269489866261, 63.66561597723832477 ) ) ;
#43566=CARTESIAN_POINT ( 'NONE',  ( -10.44761804341386124, -15.84536169652562343, 60.92300268024614240 ) ) ;
#43567=EDGE_LOOP ( 'NONE', ( #31607, #25869, #19793, #12713, #60 ) ) ;
#43568=CARTESIAN_POINT ( 'NONE',  ( -13.71339110807025641, -20.80363600241853561, 65.13628881288371986 ) ) ;
#43572=CARTESIAN_POINT ( 'NONE',  ( -24.45714095472541771, -14.31630891555219165, 69.66747352629326429 ) ) ;
#43573=CARTESIAN_POINT ( 'NONE',  ( -10.82029165754025257, -17.28804506987337675, 68.39721911992690195 ) ) ;
#43574=ORIENTED_EDGE ( 'NONE', *, *, #24223, .F. ) ;
#43575=CARTESIAN_POINT ( 'NONE',  ( -20.87058393588507244, -20.90343486309737031, 65.65624275338501548 ) ) ;
#43576=VERTEX_POINT ( 'NONE', #4203 ) ;
#43577=AXIS2_PLACEMENT_3D ( 'NONE', #32728, #32267, #36412 ) ;
#43578=CARTESIAN_POINT ( 'NONE',  ( -23.85748962928175132, -11.92509172808648543, 59.49707787073156595 ) ) ;
#43579=EDGE_CURVE ( 'NONE', #44745, #44593, #7414, .T. ) ;
#43580=EDGE_CURVE ( 'NONE', #34640, #45327, #19210, .T. ) ;
#43582=VERTEX_POINT ( 'NONE', #26606 ) ;
#43583=CARTESIAN_POINT ( 'NONE',  ( -17.39591213481957155, -7.359259842313431221, 67.17039592573394202 ) ) ;
#43587=ORIENTED_EDGE ( 'NONE', *, *, #9551, .F. ) ;
#43590=CARTESIAN_POINT ( 'NONE',  ( -24.08343201129240185, -12.65065468682437100, 73.25842202001697956 ) ) ;
#43591=CARTESIAN_POINT ( 'NONE',  ( -10.90988520595749023, -17.37161216853074919, 64.64241850740873474 ) ) ;
#43592=EDGE_LOOP ( 'NONE', ( #20128, #18409, #498, #24427, #38096 ) ) ;
#43594=CARTESIAN_POINT ( 'NONE',  ( -10.95719248119807254, -18.50832987904905735, 57.98527366719552845 ) ) ;
#43595=CARTESIAN_POINT ( 'NONE',  ( -10.65397967773411203, -12.84193750263848521, 64.56276319717653678 ) ) ;
#43598=VERTEX_POINT ( 'NONE', #21 ) ;
#43600=CARTESIAN_POINT ( 'NONE',  ( -24.48810908846319734, -17.17637088580320537, 73.06831457992643664 ) ) ;
#43601=CARTESIAN_POINT ( 'NONE',  ( -10.98557796499954087, -17.68114198556070704, 71.86718193507100239 ) ) ;
#43603=DIRECTION ( 'NONE',  ( 4.133538118270764137E-06, -2.214839422975871337E-07, 0.9999999999914324089 ) ) ;
#43606=CARTESIAN_POINT ( 'NONE',  ( -10.60570763719787735, -17.81143699334987218, 71.68222866232767387 ) ) ;
#43607=CARTESIAN_POINT ( 'NONE',  ( -24.84449963183508459, -13.71944596863515464, 54.27966884056654351 ) ) ;
#43608=EDGE_LOOP ( 'NONE', ( #27959, #44402, #45088, #17150 ) ) ;
#43609=CARTESIAN_POINT ( 'NONE',  ( -20.88147674714181079, -8.209942860146695054, 60.02620543942160225 ) ) ;
#43610=CARTESIAN_POINT ( 'NONE',  ( -13.00788241525034827, -8.809089704718775948, 64.03133736531236764 ) ) ;
#43611=CARTESIAN_POINT ( 'NONE',  ( -24.87417961795293664, -14.80849281899037884, 59.42795564617806292 ) ) ;
#43612=LINE ( 'NONE', #5931, #2544 ) ;
#43613=VERTEX_POINT ( 'NONE', #14744 ) ;
#43615=VERTEX_POINT ( 'NONE', #45090 ) ;
#43617=AXIS2_PLACEMENT_3D ( 'NONE', #23978, #22570, #34801 ) ;
#43618=CARTESIAN_POINT ( 'NONE',  ( -10.01365112473739316, -14.04198459531795962, 61.02547148049693249 ) ) ;
#43619=B_SPLINE_CURVE_WITH_KNOTS ( 'NONE', 3,
 ( #8588, #31231, #5379, #12759, #46254, #12512, #27536, #8840, #28013, #23857 ),
 .UNSPECIFIED., .F., .F.,
 ( 4, 2, 2, 2, 4 ),
 ( 0.1272669073658264094, 0.2522669073439470777, 0.3772669073220676905, 0.5022669073001884144, 0.6272669072783090272 ),
 .UNSPECIFIED. ) ;
#43621=VERTEX_POINT ( 'NONE', #3452 ) ;
#43622=CARTESIAN_POINT ( 'NONE',  ( -24.26595340233995302, -13.32969406988797623, 59.36267925071750540 ) ) ;
#43624=EDGE_CURVE ( 'NONE', #34217, #24292, #19947, .T. ) ;
#43625=ORIENTED_EDGE ( 'NONE', *, *, #3132, .F. ) ;
#43626=CARTESIAN_POINT ( 'NONE',  ( -24.43112999227502868, -15.58634490091466951, 73.00303748142292193 ) ) ;
#43627=( BOUNDED_SURFACE ( )  B_SPLINE_SURFACE ( 3, 1, ( 
 ( #35932, #1481 ),
 ( #16967, #5189 ),
 ( #31528, #46063 ),
 ( #35209, #42858 ),
 ( #16239, #27344 ),
 ( #42377, #9373 ),
 ( #20197, #8646 ) ),
 .UNSPECIFIED., .T., .F., .F. ) 
 B_SPLINE_SURFACE_WITH_KNOTS ( ( 4, 3, 4 ),
 ( 2, 2 ),
 ( 0.000000000000000000, 0.5000000000000000000, 1.000000000000000000 ),
 ( 0.000000000000000000, 1.000000000000000000 ),
 .UNSPECIFIED. ) 
 GEOMETRIC_REPRESENTATION_ITEM ( )  RATIONAL_B_SPLINE_SURFACE ( (
 ( 1.000000000000000000, 1.000000000000000000),
 ( 0.3333333333333335369, 0.3333333333333330373),
 ( 0.3333333333333335369, 0.3333333333333330373),
 ( 1.000000000000000000, 1.000000000000000000),
 ( 0.3333333333333333703, 0.3333333333333333703),
 ( 0.3333333333333333703, 0.3333333333333333703),
 ( 1.000000000000000000, 1.000000000000000000) ) ) 
 REPRESENTATION_ITEM ( '' )  SURFACE ( )  );
#43628=CARTESIAN_POINT ( 'NONE',  ( -20.39989816187257077, -8.414049535419632520, 70.34280313098182091 ) ) ;
#43630=B_SPLINE_CURVE_WITH_KNOTS ( 'NONE', 1,
 ( #37442, #26637 ),
 .UNSPECIFIED., .F., .F.,
 ( 2, 2 ),
 ( 0.000000000000000000, 1.000000000000000000 ),
 .UNSPECIFIED. ) ;
#43631=ORIENTED_EDGE ( 'NONE', *, *, #15741, .T. ) ;
#43632=CARTESIAN_POINT ( 'NONE',  ( -11.85162103594838001, -10.49015045520576983, 71.25420998615621215 ) ) ;
#43634=CARTESIAN_POINT ( 'NONE',  ( -16.09584876169039802, -7.477806291315723719, 63.85666425603482566 ) ) ;
#43635=CARTESIAN_POINT ( 'NONE',  ( -12.36794907275616850, -19.72224022788673636, 61.54678633597969650 ) ) ;
#43636=B_SPLINE_CURVE_WITH_KNOTS ( 'NONE', 1,
 ( #41703, #34291 ),
 .UNSPECIFIED., .F., .F.,
 ( 2, 2 ),
 ( 0.000000000000000000, 1.000000000000000000 ),
 .UNSPECIFIED. ) ;
#43638=DIRECTION ( 'NONE',  ( 5.828394909737395597E-08, -1.590814177254004958E-07, -0.9999999999999855671 ) ) ;
#43639=CARTESIAN_POINT ( 'NONE',  ( -10.64854695470030599, -12.86019059820356958, 64.55364013863997741 ) ) ;
#43640=EDGE_CURVE ( 'NONE', #43552, #23522, #23402, .T. ) ;
#43642=EDGE_CURVE ( 'NONE', #30663, #26903, #11761, .T. ) ;
#43646=ORIENTED_EDGE ( 'NONE', *, *, #8609, .F. ) ;
#43648=CARTESIAN_POINT ( 'NONE',  ( -11.80131277442636240, -10.54314289786156777, 67.65463988879716339 ) ) ;
#43649=CARTESIAN_POINT ( 'NONE',  ( -16.16909865928699830, -7.465622663876843923, 60.30690150944003136 ) ) ;
#43651=CARTESIAN_POINT ( 'NONE',  ( -16.58751095051766455, -21.80939428823196025, 65.22564390318969174 ) ) ;
#43652=EDGE_CURVE ( 'NONE', #44029, #32817, #16764, .T. ) ;
#43659=CARTESIAN_POINT ( 'NONE',  ( -24.32852063849251323, -13.38246526728995001, 59.37740068604990995 ) ) ;
#43660=EDGE_LOOP ( 'NONE', ( #21217, #5566, #44956, #20831 ) ) ;
#43661=B_SPLINE_CURVE_WITH_KNOTS ( 'NONE', 3,
 ( #19984, #12830, #23441, #4729, #31307, #27850, #46336, #42652, #38934, #8912 ),
 .UNSPECIFIED., .F., .F.,
 ( 4, 2, 2, 2, 4 ),
 ( 0.000000000000000000, 0.2500000000000000000, 0.5000000000000000000, 0.7500000000000000000, 1.000000000000000000 ),
 .UNSPECIFIED. ) ;
#43663=CARTESIAN_POINT ( 'NONE',  ( -10.55855397105558779, -16.42450592920206276, 71.33261492083846633 ) ) ;
#43665=CARTESIAN_POINT ( 'NONE',  ( -23.12535468111908443, -10.01343724238356359, 66.65686954956312604 ) ) ;
#43667=CARTESIAN_POINT ( 'NONE',  ( -10.85938897953544924, -12.23054697885984510, 57.74345952600154419 ) ) ;
#43669=VERTEX_POINT ( 'NONE', #18970 ) ;
#43670=FACE_BOUND ( 'NONE', #32151, .T. ) ;
#43671=CARTESIAN_POINT ( 'NONE',  ( -24.82668569956033622, -13.96895926810607946, 73.29988393021096726 ) ) ;
#43674=ORIENTED_EDGE ( 'NONE', *, *, #18984, .F. ) ;
#43675=CARTESIAN_POINT ( 'NONE',  ( -10.38078067960954520, -14.50222210708341741, 68.15800126083217947 ) ) ;
#43676=FILL_AREA_STYLE_COLOUR ( '', #37640 ) ;
#43677=CARTESIAN_POINT ( 'NONE',  ( -17.00410561000564513, -7.771727611841390271, 74.26018273220857679 ) ) ;
#43678=CARTESIAN_POINT ( 'NONE',  ( -21.08710395203513244, -20.77481533096753452, 69.07066874357158781 ) ) ;
#43679=CARTESIAN_POINT ( 'NONE',  ( -21.41370985594940990, -18.61458953632344659, 53.88362224778186516 ) ) ;
#43680=CARTESIAN_POINT ( 'NONE',  ( -15.87557486115803052, -7.931373420853708112, 67.44007279014866185 ) ) ;
#43682=ORIENTED_EDGE ( 'NONE', *, *, #41610, .F. ) ;
#43684=CARTESIAN_POINT ( 'NONE',  ( -13.24520478104276933, -9.193358983593601153, 64.19481115367814539 ) ) ;
#43685=CARTESIAN_POINT ( 'NONE',  ( -19.24829632005326019, -7.991050106228435368, 67.04504941182814548 ) ) ;
#43686=( BOUNDED_SURFACE ( )  B_SPLINE_SURFACE ( 3, 1, ( 
 ( #25723, #21785 ),
 ( #21324, #28695 ),
 ( #44227, #14125 ),
 ( #43732, #9985 ),
 ( #47653, #40739 ),
 ( #40030, #48134 ),
 ( #13891, #28934 ) ),
 .UNSPECIFIED., .T., .F., .F. ) 
 B_SPLINE_SURFACE_WITH_KNOTS ( ( 4, 3, 4 ),
 ( 2, 2 ),
 ( 0.000000000000000000, 0.5000000000000000000, 1.000000000000000000 ),
 ( 0.000000000000000000, 1.000000000000000000 ),
 .UNSPECIFIED. ) 
 GEOMETRIC_REPRESENTATION_ITEM ( )  RATIONAL_B_SPLINE_SURFACE ( (
 ( 1.000000000000000000, 1.000000000000000000),
 ( 0.3333333333333335369, 0.3333333333333330373),
 ( 0.3333333333333335369, 0.3333333333333330373),
 ( 1.000000000000000000, 1.000000000000000000),
 ( 0.3333333333333333703, 0.3333333333333333703),
 ( 0.3333333333333333703, 0.3333333333333333703),
 ( 1.000000000000000000, 1.000000000000000000) ) ) 
 REPRESENTATION_ITEM ( '' )  SURFACE ( )  );
#43687=ADVANCED_FACE ( 'NONE', ( #33975 ), #13678, .T. ) ;
#43691=ORIENTED_EDGE ( 'NONE', *, *, #10858, .T. ) ;
#43692=CARTESIAN_POINT ( 'NONE',  ( -21.05173877328207510, -20.79594606475588137, 65.86988551343767995 ) ) ;
#43693=CARTESIAN_POINT ( 'NONE',  ( -21.02116742812006223, -20.87599269455877860, 61.99982634431184181 ) ) ;
#43696=( BOUNDED_CURVE ( )  B_SPLINE_CURVE ( 3, ( #34338, #8760, #26735, #19581 ),
 .UNSPECIFIED., .F., .F. ) 
 B_SPLINE_CURVE_WITH_KNOTS ( ( 4, 4 ),
 ( 0.9074455897393663983, 1.000000000000000000 ),
 .UNSPECIFIED. ) 
 CURVE ( )  GEOMETRIC_REPRESENTATION_ITEM ( )  RATIONAL_B_SPLINE_CURVE ( ( 0.6983129098261007250, 0.7760317562607048636, 0.8765941196520046219, 1.000000000000000000 ) ) 
 REPRESENTATION_ITEM ( '' )  );
#43697=CARTESIAN_POINT ( 'NONE',  ( -18.54053647975129238, -21.77400351277580270, 68.81514511891278119 ) ) ;
#43699=CARTESIAN_POINT ( 'NONE',  ( -18.98390459359973548, -7.933620001262258192, 66.91543923465640376 ) ) ;
#43701=ORIENTED_EDGE ( 'NONE', *, *, #4051, .F. ) ;
#43703=EDGE_CURVE ( 'NONE', #956, #4771, #18338, .T. ) ;
#43704=CARTESIAN_POINT ( 'NONE',  ( -23.33759372854072822, -18.55733037075456693, 72.83538601489385655 ) ) ;
#43705=CYLINDRICAL_SURFACE ( 'NONE', #1452, 0.1500000000000056566 ) ;
#43706=CARTESIAN_POINT ( 'NONE',  ( -10.77407439928238908, -17.16094721493464093, 57.89580409822232099 ) ) ;
#43707=ORIENTED_EDGE ( 'NONE', *, *, #31645, .F. ) ;
#43708=CARTESIAN_POINT ( 'NONE',  ( -22.38400238879419391, -20.36826089713532895, 62.41934470639706944 ) ) ;
#43709=CARTESIAN_POINT ( 'NONE',  ( -24.53780083649505173, -12.59584922708229904, 69.95738295622972203 ) ) ;
#43710=ADVANCED_FACE ( 'NONE', ( #31753 ), #1215, .T. ) ;
#43712=DIRECTION ( 'NONE',  ( -1.770046493635803029E-07, 8.183081527205841035E-08, 0.9999999999999809042 ) ) ;
#43713=B_SPLINE_CURVE_WITH_KNOTS ( 'NONE', 3,
 ( #30915, #35311, #12424, #5047, #27444, #28181, #12186, #42477, #24252, #43205 ),
 .UNSPECIFIED., .F., .F.,
 ( 4, 2, 2, 2, 4 ),
 ( 0.000000000000000000, 0.2500000000000000000, 0.5000000000000000000, 0.7500000000000000000, 1.000000000000000000 ),
 .UNSPECIFIED. ) ;
#43714=CARTESIAN_POINT ( 'NONE',  ( -11.42622084110231029, -18.51434063454204093, 61.27710833181471628 ) ) ;
#43715=CARTESIAN_POINT ( 'NONE',  ( -23.04635137988585214, -19.07596084359022726, 65.96822594231640835 ) ) ;
#43717=CARTESIAN_POINT ( 'NONE',  ( -24.34788207851723740, -17.55975901192373811, 66.12074161205516987 ) ) ;
#43719=CARTESIAN_POINT ( 'NONE',  ( -20.15980875465224997, -21.73879204183439029, 72.59752904776686933 ) ) ;
#43720=CARTESIAN_POINT ( 'NONE',  ( -10.00117625416208433, -15.44487358686203571, 57.68297391752145842 ) ) ;
#43721=B_SPLINE_CURVE_WITH_KNOTS ( 'NONE', 1,
 ( #18241, #2745 ),
 .UNSPECIFIED., .F., .F.,
 ( 2, 2 ),
 ( 0.000000000000000000, 1.000000000000000000 ),
 .UNSPECIFIED. ) ;
#43722=EDGE_LOOP ( 'NONE', ( #43976, #26760 ) ) ;
#43726=VERTEX_POINT ( 'NONE', #5413 ) ;
#43727=VERTEX_POINT ( 'NONE', #42355 ) ;
#43728=CARTESIAN_POINT ( 'NONE',  ( -18.76558283008973049, -7.480892646508040755, 70.55563411965815135 ) ) ;
#43729=CARTESIAN_POINT ( 'NONE',  ( -23.19494587819374942, -18.77118419879135303, 66.12389430422854275 ) ) ;
#43730=DIRECTION ( 'NONE',  ( 0.09855345062332551698, 0.9951317587989213509, 3.188559572831062401E-08 ) ) ;
#43731=EDGE_CURVE ( 'NONE', #35167, #16426, #8312, .T. ) ;
#43732=CARTESIAN_POINT ( 'NONE',  ( -13.01616685277437391, -9.306763517318227485, 70.86397465682092900 ) ) ;
#43733=ADVANCED_FACE ( 'NONE', ( #1719 ), #20433, .T. ) ;
#43734=ORIENTED_EDGE ( 'NONE', *, *, #31173, .F. ) ;
#43735=ORIENTED_EDGE ( 'NONE', *, *, #44535, .T. ) ;
#43737=B_SPLINE_CURVE_WITH_KNOTS ( 'NONE', 3,
 ( #44361, #6677, #29822, #21934, #32995, #29327, #14505, #18226, #44133, #11103 ),
 .UNSPECIFIED., .F., .F.,
 ( 4, 2, 2, 2, 4 ),
 ( 0.000000000000000000, 0.2500000000000000000, 0.5000000000000000000, 0.7500000000000000000, 1.000000000000000000 ),
 .UNSPECIFIED. ) ;
#43738=EDGE_CURVE ( 'NONE', #23048, #25893, #45926, .T. ) ;
#43739=CARTESIAN_POINT ( 'NONE',  ( -24.87381043567631878, -14.88698653629387003, 59.42112968367225534 ) ) ;
#43740=CARTESIAN_POINT ( 'NONE',  ( -23.70015231925135168, -18.82353928378165975, 69.47867257277708575 ) ) ;
#43742=VERTEX_POINT ( 'NONE', #27085 ) ;
#43743=CARTESIAN_POINT ( 'NONE',  ( -23.85748962928175132, -11.92509172808648543, 59.49707787073156595 ) ) ;
#43744=DIRECTION ( 'NONE',  ( 3.549360974554993999E-17, -6.371834667797928663E-18, -1.000000000000000000 ) ) ;
#43745=ORIENTED_EDGE ( 'NONE', *, *, #20153, .T. ) ;
#43747=VECTOR ( 'NONE', #17923, 1000.000000000000227 ) ;
#43748=AXIS2_PLACEMENT_3D ( 'NONE', #24489, #39247, #9940 ) ;
#43749=ORIENTED_EDGE ( 'NONE', *, *, #33091, .F. ) ;
#43751=DIRECTION ( 'NONE',  ( -5.731567514496413899E-31, -1.020425574103664789E-16, -1.000000000000000000 ) ) ;
#43752=CARTESIAN_POINT ( 'NONE',  ( -18.97054410961560578, -7.521390078327941708, 67.08567059339527816 ) ) ;
#43753=VERTEX_POINT ( 'NONE', #34715 ) ;
#43754=DIRECTION ( 'NONE',  ( 6.312331213287273068E-07, 6.220915576652692866E-06, 0.9999999999804508599 ) ) ;
#43756=CARTESIAN_POINT ( 'NONE',  ( -19.23866564181064831, -21.62168251543363695, 58.82507384655652771 ) ) ;
#43759=B_SPLINE_CURVE_WITH_KNOTS ( 'NONE', 1,
 ( #2176, #6117 ),
 .UNSPECIFIED., .F., .F.,
 ( 2, 2 ),
 ( 0.000000000000000000, 1.000000000000000000 ),
 .UNSPECIFIED. ) ;
#43760=CARTESIAN_POINT ( 'NONE',  ( -24.85346453946240786, -14.25412306239375049, 69.90921191474365060 ) ) ;
#43761=EDGE_LOOP ( 'NONE', ( #16625, #21358 ) ) ;
#43762=CARTESIAN_POINT ( 'NONE',  ( -13.26809664353323726, -20.51382390604332784, 61.66079502706314486 ) ) ;
#43763=CARTESIAN_POINT ( 'NONE',  ( -9.974215871585233373, -14.86485004610319827, 74.91283608227215041 ) ) ;
#43764=ORIENTED_EDGE ( 'NONE', *, *, #43863, .T. ) ;
#43765=EDGE_CURVE ( 'NONE', #35674, #38958, #15986, .T. ) ;
#43766=CARTESIAN_POINT ( 'NONE',  ( -22.51726263819124441, -19.68384825699994423, 72.79400547081151274 ) ) ;
#43767=FACE_OUTER_BOUND ( 'NONE', #6105, .T. ) ;
#43768=CARTESIAN_POINT ( 'NONE',  ( -13.26948432366006969, -9.109728530933422164, 60.32461385657482822 ) ) ;
#43769=CARTESIAN_POINT ( 'NONE',  ( -13.47245400663725690, -21.12492667118925382, 65.10133491818508844 ) ) ;
#43771=CARTESIAN_POINT ( 'NONE',  ( -18.11889279746774051, -21.82488571228486052, 65.49532159284275679 ) ) ;
#43772=CARTESIAN_POINT ( 'NONE',  ( -19.03203220252169459, -7.534746275656669212, 67.09410107843321214 ) ) ;
#43775=CARTESIAN_POINT ( 'NONE',  ( -9.979672921070292801, -14.51892525773737574, 67.90154210966345261 ) ) ;
#43776=CARTESIAN_POINT ( 'NONE',  ( -24.77850173595669503, -15.99961219664241696, 66.24041782031707726 ) ) ;
#43777=ORIENTED_EDGE ( 'NONE', *, *, #38491, .F. ) ;
#43778=VERTEX_POINT ( 'NONE', #15983 ) ;
#43779=CARTESIAN_POINT ( 'NONE',  ( -14.81801217541857518, -21.30606701939088765, 58.45152577640163116 ) ) ;
#43780=CARTESIAN_POINT ( 'NONE',  ( -15.56648003470729336, -8.060123005460294365, 70.83663087793784996 ) ) ;
#43781=CARTESIAN_POINT ( 'NONE',  ( -10.03035368457962662, -15.72374687363213575, 61.22284448286259817 ) ) ;
#43782=CARTESIAN_POINT ( 'NONE',  ( -10.59051903643958958, -13.04363995460383663, 74.82250634059326444 ) ) ;
#43783=CARTESIAN_POINT ( 'NONE',  ( -19.45112228907181873, -7.640138419055735319, 60.08376115775335791 ) ) ;
#43784=CARTESIAN_POINT ( 'NONE',  ( -21.18398602608336745, -21.24092397535611809, 65.69958545398036165 ) ) ;
#43785=CARTESIAN_POINT ( 'NONE',  ( -12.40538917401127961, -20.31523793222865493, 68.52152763170285255 ) ) ;
#43786=CARTESIAN_POINT ( 'NONE',  ( -20.50783594841701785, -8.027295835816985914, 66.96599399791791996 ) ) ;
#43787=ADVANCED_FACE ( 'NONE', ( #31029 ), #46046, .T. ) ;
#43790=VERTEX_POINT ( 'NONE', #17917 ) ;
#43791=ORIENTED_EDGE ( 'NONE', *, *, #6136, .T. ) ;
#43792=CARTESIAN_POINT ( 'NONE',  ( -24.83263366448169762, -15.59490076022755112, 73.18799035805197661 ) ) ;
#43793=EDGE_CURVE ( 'NONE', #26823, #24042, #21804, .T. ) ;
#43795=CARTESIAN_POINT ( 'NONE',  ( -19.86472783040103707, -8.248401445373296781, 73.94770042502594265 ) ) ;
#43800=B_SPLINE_CURVE_WITH_KNOTS ( 'NONE', 1,
 ( #24686, #25399 ),
 .UNSPECIFIED., .F., .F.,
 ( 2, 2 ),
 ( 0.000000000000000000, 1.000000000000000000 ),
 .UNSPECIFIED. ) ;
#43802=ORIENTED_EDGE ( 'NONE', *, *, #11617, .T. ) ;
#43803=B_SPLINE_CURVE_WITH_KNOTS ( 'NONE', 1,
 ( #34196, #33962 ),
 .UNSPECIFIED., .F., .F.,
 ( 2, 2 ),
 ( 0.000000000000000000, 1.000000000000000000 ),
 .UNSPECIFIED. ) ;
#43804=CARTESIAN_POINT ( 'NONE',  ( -15.22312280068192081, -21.51522583983519255, 61.79167741754957177 ) ) ;
#43805=CARTESIAN_POINT ( 'NONE',  ( -19.96591064584176323, -21.38508948087614669, 72.40478736589766129 ) ) ;
#43807=CARTESIAN_POINT ( 'NONE',  ( -10.42257993575900876, -15.70014684107950842, 68.12200980565171449 ) ) ;
#43809=CARTESIAN_POINT ( 'NONE',  ( -10.59785598015707819, -16.35919899344940021, 71.55636283569445766 ) ) ;
#43813=( BOUNDED_CURVE ( )  B_SPLINE_CURVE ( 3, ( #7755, #4059, #19058, #7004 ),
 .UNSPECIFIED., .F., .F. ) 
 B_SPLINE_CURVE_WITH_KNOTS ( ( 4, 4 ),
 ( 0.000000000000000000, 0.4074455897393629566 ),
 .UNSPECIFIED. ) 
 CURVE ( )  GEOMETRIC_REPRESENTATION_ITEM ( )  RATIONAL_B_SPLINE_CURVE ( ( 1.000000000000000000, 0.4567392136813327452, 0.3561768502900305999, 0.6983129098260936196 ) ) 
 REPRESENTATION_ITEM ( '' )  );
#43814=B_SPLINE_CURVE_WITH_KNOTS ( 'NONE', 3,
 ( #43720, #40015, #17097, #21310, #24763, #24530, #36302, #2585, #32619, #13880 ),
 .UNSPECIFIED., .F., .F.,
 ( 4, 2, 2, 2, 4 ),
 ( 0.1272669073658393990, 0.2522669073463166267, 0.3772669073267939099, 0.5022669073072711932, 0.6272669072877483654 ),
 .UNSPECIFIED. ) ;
#43815=B_SPLINE_CURVE_WITH_KNOTS ( 'NONE', 3,
 ( #10178, #5518, #12886, #1566, #13114, #46640, #24480, #24719, #5986, #5271 ),
 .UNSPECIFIED., .F., .F.,
 ( 4, 2, 2, 2, 4 ),
 ( 0.000000000000000000, 0.2500000000000000000, 0.5000000000000000000, 0.7500000000000000000, 1.000000000000000000 ),
 .UNSPECIFIED. ) ;
#43818=CARTESIAN_POINT ( 'NONE',  ( -23.04658630743911374, -18.97915095201261337, 59.11083934693237296 ) ) ;
#43821=ORIENTED_EDGE ( 'NONE', *, *, #15261, .T. ) ;
#43823=CARTESIAN_POINT ( 'NONE',  ( -10.23610968374255314, -12.85046669463587143, 67.85336945107273721 ) ) ;
#43824=B_SPLINE_CURVE_WITH_KNOTS ( 'NONE', 3,
 ( #21357, #5617, #32431, #47452, #20627, #35622, #26198, #104, #11179, #3531 ),
 .UNSPECIFIED., .F., .F.,
 ( 4, 2, 2, 2, 4 ),
 ( 0.1272669073658526662, 0.2522669073488176261, 0.3772669073317826416, 0.5022669073147476571, 0.6272669072977126170 ),
 .UNSPECIFIED. ) ;
#43825=ORIENTED_EDGE ( 'NONE', *, *, #5122, .T. ) ;
#43830=ORIENTED_EDGE ( 'NONE', *, *, #25635, .T. ) ;
#43832=CARTESIAN_POINT ( 'NONE',  ( -15.95707209241614422, -7.504986913482371236, 63.85506412386598640 ) ) ;
#43833=( BOUNDED_CURVE ( )  B_SPLINE_CURVE ( 3, ( #46789, #27585, #13517, #47021 ),
 .UNSPECIFIED., .F., .F. ) 
 B_SPLINE_CURVE_WITH_KNOTS ( ( 4, 4 ),
 ( 0.5000000000000000000, 0.9074455897393661763 ),
 .UNSPECIFIED. ) 
 CURVE ( )  GEOMETRIC_REPRESENTATION_ITEM ( )  RATIONAL_B_SPLINE_CURVE ( ( 1.000000000000021982, 0.4567392136813435144, 0.3561768502900192201, 0.6983129098260727474 ) ) 
 REPRESENTATION_ITEM ( '' )  );
#43834=CARTESIAN_POINT ( 'NONE',  ( -23.52949419687348964, -11.28347464189849703, 70.17738639980606763 ) ) ;
#43836=( BOUNDED_CURVE ( )  B_SPLINE_CURVE ( 3, ( #21147, #16703, #24360, #9099 ),
 .UNSPECIFIED., .F., .F. ) 
 B_SPLINE_CURVE_WITH_KNOTS ( ( 4, 4 ),
 ( 0.4074455897393593484, 0.5000000000000000000 ),
 .UNSPECIFIED. ) 
 CURVE ( )  GEOMETRIC_REPRESENTATION_ITEM ( )  RATIONAL_B_SPLINE_CURVE ( ( 0.6983129098260878465, 0.7760317562606910968, 0.8765941196519944079, 0.9999999999999958922 ) ) 
 REPRESENTATION_ITEM ( '' )  );
#43837=FACE_OUTER_BOUND ( 'NONE', #32597, .T. ) ;
#43839=CARTESIAN_POINT ( 'NONE',  ( -10.66703313327717417, -12.79807994555918960, 64.56836111017611302 ) ) ;
#43840=LINE ( 'NONE', #17469, #24805 ) ;
#43841=ORIENTED_EDGE ( 'NONE', *, *, #30300, .T. ) ;
#43844=DIRECTION ( 'NONE',  ( 0.8651630202045380580, -0.5014907262059380422, -5.433021001198017416E-08 ) ) ;
#43845=ORIENTED_EDGE ( 'NONE', *, *, #15982, .T. ) ;
#43846=FACE_OUTER_BOUND ( 'NONE', #35522, .T. ) ;
#43848=FACE_OUTER_BOUND ( 'NONE', #30245, .T. ) ;
#43850=CARTESIAN_POINT ( 'NONE',  ( -12.31380156693488992, -10.02538874655004442, 60.85918086676540639 ) ) ;
#43851=( BOUNDED_CURVE ( )  B_SPLINE_CURVE ( 3, ( #47673, #9777, #1649, #13911 ),
 .UNSPECIFIED., .F., .F. ) 
 B_SPLINE_CURVE_WITH_KNOTS ( ( 4, 4 ),
 ( 0.4074455897393667869, 0.5000000000000000000 ),
 .UNSPECIFIED. ) 
 CURVE ( )  GEOMETRIC_REPRESENTATION_ITEM ( )  RATIONAL_B_SPLINE_CURVE ( ( 0.6983129098261057210, 0.7760317562607094155, 0.8765941196520075085, 1.000000000000000222 ) ) 
 REPRESENTATION_ITEM ( '' )  );
#43853=CARTESIAN_POINT ( 'NONE',  ( -20.90753508896134960, -8.676468725517494818, 60.25614029449676678 ) ) ;
#43858=CARTESIAN_POINT ( 'NONE',  ( -16.58248652804564927, -22.21164012696474899, 65.34751608897319386 ) ) ;
#43860=ORIENTED_EDGE ( 'NONE', *, *, #22282, .F. ) ;
#43862=EDGE_CURVE ( 'NONE', #47879, #13276, #13252, .T. ) ;
#43863=EDGE_CURVE ( 'NONE', #39854, #3501, #26860, .T. ) ;
#43864=ORIENTED_EDGE ( 'NONE', *, *, #17843, .F. ) ;
#43865=CARTESIAN_POINT ( 'NONE',  ( -17.38762135442090795, -7.756298984960698917, 63.43568405917763897 ) ) ;
#43867=CARTESIAN_POINT ( 'NONE',  ( -15.49415903819706486, -8.028509590827587417, 74.22985659018391402 ) ) ;
#43869=ADVANCED_FACE ( 'NONE', ( #21405 ), #40113, .T. ) ;
#43872=CARTESIAN_POINT ( 'NONE',  ( -23.96075645138428456, -17.45014240273063066, 65.94357239682317129 ) ) ;
#43873=DIRECTION ( 'NONE',  ( 0.7800143876985550229, -0.6257615799833393666, 5.505484597913564244E-08 ) ) ;
#43874=EDGE_CURVE ( 'NONE', #34219, #18401, #23611, .T. ) ;
#43876=CARTESIAN_POINT ( 'NONE',  ( -20.88270815654435353, -21.40782497263450068, 58.82970582236164603 ) ) ;
#43877=CARTESIAN_POINT ( 'NONE',  ( -24.47368665962210343, -14.70950332193510413, 62.72768537250228604 ) ) ;
#43878=CARTESIAN_POINT ( 'NONE',  ( -23.34190511704397153, -19.33504077159632573, 58.92764702605110472 ) ) ;
#43879=ORIENTED_EDGE ( 'NONE', *, *, #25362, .T. ) ;
#43880=CARTESIAN_POINT ( 'NONE',  ( -20.00946575929301474, -8.250368826910309039, 74.02096600124984604 ) ) ;
#43881=ORIENTED_EDGE ( 'NONE', *, *, #40676, .T. ) ;
#43886=CARTESIAN_POINT ( 'NONE',  ( -13.71339271347209454, -20.80363700974684349, 65.28628881287176000 ) ) ;
#43888=DIRECTION ( 'NONE',  ( -5.731567514496413899E-31, -1.020425574103664789E-16, -1.000000000000000000 ) ) ;
#43890=CARTESIAN_POINT ( 'NONE',  ( -17.77921064978749044, -22.25082400685520057, 58.59048811498988840 ) ) ;
#43893=CARTESIAN_POINT ( 'NONE',  ( -10.20197030601470090, -12.78660143320473175, 53.49999999999994316 ) ) ;
#43895=AXIS2_PLACEMENT_3D ( 'NONE', #16483, #31519, #999 ) ;
#43896=CARTESIAN_POINT ( 'NONE',  ( -22.94085434386056832, -9.802298134861713308, 70.19673941016031904 ) ) ;
#43900=ORIENTED_EDGE ( 'NONE', *, *, #6496, .F. ) ;
#43902=CARTESIAN_POINT ( 'NONE',  ( -10.39215589072981416, -14.30487699944780289, 64.68803863382906627 ) ) ;
#43903=CARTESIAN_POINT ( 'NONE',  ( -24.83263366448169762, -15.59490076022755112, 73.18799035805197661 ) ) ;
#43904=ORIENTED_EDGE ( 'NONE', *, *, #12413, .T. ) ;
#43905=CARTESIAN_POINT ( 'NONE',  ( -10.38025826595154477, -14.36272272558099772, 71.47215414551031643 ) ) ;
#43906=CARTESIAN_POINT ( 'NONE',  ( -10.14660727810982976, -16.40665786317032371, 71.56094979796495181 ) ) ;
#43907=CARTESIAN_POINT ( 'NONE',  ( -11.77456283875730136, -18.94252740843654337, 71.68685932468078192 ) ) ;
#43908=CARTESIAN_POINT ( 'NONE',  ( -17.90690210039477392, -22.24367211215778539, 61.99819018155271522 ) ) ;
#43909=CARTESIAN_POINT ( 'NONE',  ( -19.30746897944592888, -7.600422969554355923, 60.07437648108736994 ) ) ;
#43910=CARTESIAN_POINT ( 'NONE',  ( -14.66790711817407278, -21.29843871104708342, 58.18089935161520287 ) ) ;
#43911=EDGE_CURVE ( 'NONE', #1220, #42912, #24984, .T. ) ;
#43912=CARTESIAN_POINT ( 'NONE',  ( -15.53265176333180619, -21.60105060138385369, 72.33103357390284316 ) ) ;
#43913=FACE_OUTER_BOUND ( 'NONE', #24939, .T. ) ;
#43914=AXIS2_PLACEMENT_3D ( 'NONE', #13668, #25269, #2838 ) ;
#43915=CARTESIAN_POINT ( 'NONE',  ( -12.15399301493812878, -9.543295845094297292, 57.20440096431307353 ) ) ;
#43916=PLANE ( 'NONE',  #46036 ) ;
#43917=CARTESIAN_POINT ( 'NONE',  ( -20.75775239920833215, -8.146595409969087598, 63.56767435313065562 ) ) ;
#43918=EDGE_CURVE ( 'NONE', #47684, #5480, #20109, .T. ) ;
#43919=ORIENTED_EDGE ( 'NONE', *, *, #34986, .T. ) ;
#43920=FACE_OUTER_BOUND ( 'NONE', #46323, .T. ) ;
#43921=CARTESIAN_POINT ( 'NONE',  ( -11.54914866798053197, -18.61512550936221544, 61.46813926877504031 ) ) ;
#43922=CARTESIAN_POINT ( 'NONE',  ( -24.39703051400040223, -17.43244739030124890, 69.60678083904183211 ) ) ;
#43924=DIRECTION ( 'NONE',  ( -5.731567514496413899E-31, -1.020425574103664789E-16, -1.000000000000000000 ) ) ;
#43925=DIRECTION ( 'NONE',  ( -5.731567514496413899E-31, -1.020425574103664789E-16, -1.000000000000000000 ) ) ;
#43926=ORIENTED_EDGE ( 'NONE', *, *, #16103, .T. ) ;
#43927=ORIENTED_EDGE ( 'NONE', *, *, #24330, .F. ) ;
#43929=B_SPLINE_CURVE_WITH_KNOTS ( 'NONE', 1,
 ( #45929, #31875 ),
 .UNSPECIFIED., .F., .F.,
 ( 2, 2 ),
 ( 0.000000000000000000, 1.000000000000000000 ),
 .UNSPECIFIED. ) ;
#43930=CARTESIAN_POINT ( 'NONE',  ( -21.18000576974785787, -20.77541348745421246, 69.35450184739246993 ) ) ;
#43931=EDGE_CURVE ( 'NONE', #7278, #39540, #14737, .T. ) ;
#43934=( BOUNDED_SURFACE ( )  B_SPLINE_SURFACE ( 3, 1, ( 
 ( #32291, #39907 ),
 ( #17488, #47061 ),
 ( #24174, #40156 ),
 ( #20225, #21200 ),
 ( #13779, #47546 ),
 ( #35237, #28099 ),
 ( #1512, #39177 ) ),
 .UNSPECIFIED., .T., .F., .F. ) 
 B_SPLINE_SURFACE_WITH_KNOTS ( ( 4, 3, 4 ),
 ( 2, 2 ),
 ( 0.000000000000000000, 0.5000000000000000000, 1.000000000000000000 ),
 ( 0.000000000000000000, 1.000000000000000000 ),
 .UNSPECIFIED. ) 
 GEOMETRIC_REPRESENTATION_ITEM ( )  RATIONAL_B_SPLINE_SURFACE ( (
 ( 1.000000000000000000, 1.000000000000000000),
 ( 0.3333333333333335369, 0.3333333333333330373),
 ( 0.3333333333333335369, 0.3333333333333330373),
 ( 1.000000000000000000, 1.000000000000000000),
 ( 0.3333333333333333703, 0.3333333333333333703),
 ( 0.3333333333333333703, 0.3333333333333333703),
 ( 1.000000000000000000, 1.000000000000000000) ) ) 
 REPRESENTATION_ITEM ( '' )  SURFACE ( )  );
#43935=EDGE_CURVE ( 'NONE', #33529, #45391, #7603, .T. ) ;
#43937=CARTESIAN_POINT ( 'NONE',  ( -15.35760563471625595, -7.651489246766129071, 74.27259798395405710 ) ) ;
#43938=FACE_OUTER_BOUND ( 'NONE', #21267, .T. ) ;
#43940=B_SPLINE_CURVE_WITH_KNOTS ( 'NONE', 1,
 ( #24288, #16867 ),
 .UNSPECIFIED., .F., .F.,
 ( 2, 2 ),
 ( 0.000000000000000000, 1.000000000000000000 ),
 .UNSPECIFIED. ) ;
#43941=CARTESIAN_POINT ( 'NONE',  ( -19.36879887743637241, -22.00096660050156672, 58.71781517422923002 ) ) ;
#43944=VERTEX_POINT ( 'NONE', #33661 ) ;
#43946=CYLINDRICAL_SURFACE ( 'NONE', #40078, 0.1499999999999973577 ) ;
#43947=ORIENTED_EDGE ( 'NONE', *, *, #35992, .F. ) ;
#43948=LINE ( 'NONE', #28901, #17342 ) ;
#43950=CARTESIAN_POINT ( 'NONE',  ( -9.979298953853202647, -14.52750539432568289, 67.97987381442376886 ) ) ;
#43951=ORIENTED_EDGE ( 'NONE', *, *, #45081, .T. ) ;
#43952=CARTESIAN_POINT ( 'NONE',  ( -10.70366717127368084, -11.59369238842668359, 71.13214950009151494 ) ) ;
#43955=CARTESIAN_POINT ( 'NONE',  ( -24.10584592916820057, -12.56049825913868645, 73.24225570139947195 ) ) ;
#43956=ORIENTED_EDGE ( 'NONE', *, *, #27691, .F. ) ;
#43959=CARTESIAN_POINT ( 'NONE',  ( -24.90891992605694227, -15.28604896337863472, 53.49999999999994316 ) ) ;
#43961=CARTESIAN_POINT ( 'NONE',  ( -15.41904748403203484, -7.634001509309876532, 74.19490257054667381 ) ) ;
#43962=CARTESIAN_POINT ( 'NONE',  ( -16.19792114999740562, -7.866354181730329742, 60.48556343814865954 ) ) ;
#43963=CARTESIAN_POINT ( 'NONE',  ( -24.69822986944709697, -13.19963441799314197, 59.54763197719577761 ) ) ;
#43964=ORIENTED_EDGE ( 'NONE', *, *, #9469, .T. ) ;
#43965=CARTESIAN_POINT ( 'NONE',  ( -14.92957361138602579, -21.82925975653312278, 65.22101252026929785 ) ) ;
#43967=CARTESIAN_POINT ( 'NONE',  ( -12.98382639084827694, -18.07753951239978463, 53.69233794759168887 ) ) ;
#43968=CARTESIAN_POINT ( 'NONE',  ( -13.38109212034142992, -20.52372131538385958, 58.34650125919424823 ) ) ;
#43969=EDGE_CURVE ( 'NONE', #43790, #10474, #15433, .T. ) ;
#43971=CARTESIAN_POINT ( 'NONE',  ( -19.81318675137362462, -21.38895278651759568, 69.23482470049566473 ) ) ;
#43976=ORIENTED_EDGE ( 'NONE', *, *, #35710, .T. ) ;
#43979=CARTESIAN_POINT ( 'NONE',  ( -12.90907418246050575, -8.883084357830009381, 67.55755565527715589 ) ) ;
#43980=( BOUNDED_CURVE ( )  B_SPLINE_CURVE ( 3, ( #16682, #31722, #13470, #28516 ),
 .UNSPECIFIED., .F., .F. ) 
 B_SPLINE_CURVE_WITH_KNOTS ( ( 4, 4 ),
 ( 0.000000000000000000, 0.4074455897393656212 ),
 .UNSPECIFIED. ) 
 CURVE ( )  GEOMETRIC_REPRESENTATION_ITEM ( )  RATIONAL_B_SPLINE_CURVE ( ( 1.000000000000000000, 0.4567392136813311909, 0.3561768502900300448, 0.6983129098260966172 ) ) 
 REPRESENTATION_ITEM ( '' )  );
#43981=FACE_OUTER_BOUND ( 'NONE', #19056, .T. ) ;
#43984=EDGE_LOOP ( 'NONE', ( #34072, #43207, #45409, #46557, #48661 ) ) ;
#43986=EDGE_CURVE ( 'NONE', #20830, #5461, #3644, .T. ) ;
#43988=DIRECTION ( 'NONE',  ( -5.888300610989836252E-06, -9.662809626516592716E-06, 0.9999999999359789893 ) ) ;
#43989=EDGE_CURVE ( 'NONE', #33222, #45841, #31887, .T. ) ;
#43993=EDGE_CURVE ( 'NONE', #17461, #42531, #13023, .T. ) ;
#43994=CARTESIAN_POINT ( 'NONE',  ( -15.66808075433818992, -21.64011062311675815, 71.93086697972334775 ) ) ;
#43996=CARTESIAN_POINT ( 'NONE',  ( -24.87424715294626054, -14.79413390388218374, 59.40333630874831528 ) ) ;
#43997=EDGE_CURVE ( 'NONE', #5768, #22634, #21538, .T. ) ;
#43998=ORIENTED_EDGE ( 'NONE', *, *, #39188, .F. ) ;
#43999=CARTESIAN_POINT ( 'NONE',  ( -11.24765613265417841, -11.51409684124195998, 67.63481256405479769 ) ) ;
#44002=ORIENTED_EDGE ( 'NONE', *, *, #16957, .T. ) ;
#44003=CYLINDRICAL_SURFACE ( 'NONE', #17393, 0.1500000000000066835 ) ;
#44004=CARTESIAN_POINT ( 'NONE',  ( -16.34000564509899078, -21.72481133989910163, 58.35873513796175160 ) ) ;
#44005=CARTESIAN_POINT ( 'NONE',  ( -9.994167848590823411, -14.26249844466068772, 64.48829615640673296 ) ) ;
#44008=CARTESIAN_POINT ( 'NONE',  ( -14.72778380697173617, -21.32322314059157264, 58.16617885012794886 ) ) ;
#44011=ORIENTED_EDGE ( 'NONE', *, *, #320, .F. ) ;
#44012=CARTESIAN_POINT ( 'NONE',  ( -21.92320759141193776, -20.24164808600927046, 62.32619241939052301 ) ) ;
#44013=CARTESIAN_POINT ( 'NONE',  ( -23.88415220289344276, -17.63235127459526908, 62.62360984996717406 ) ) ;
#44014=DIRECTION ( 'NONE',  ( 0.4468359692653126602, -0.01837434545035531233, 0.8944271909999156334 ) ) ;
#44015=ADVANCED_FACE ( 'NONE', ( #3157 ), #36871, .T. ) ;
#44017=FACE_OUTER_BOUND ( 'NONE', #29706, .T. ) ;
#44018=ORIENTED_EDGE ( 'NONE', *, *, #20435, .T. ) ;
#44019=CARTESIAN_POINT ( 'NONE',  ( -19.70296738327746056, -7.644578391088470148, 53.76227901944321275 ) ) ;
#44020=CARTESIAN_POINT ( 'NONE',  ( -13.59294679993987565, -20.73687756253419678, 68.60058253670568718 ) ) ;
#44021=CARTESIAN_POINT ( 'NONE',  ( -13.12596155740353154, -8.723179898376328012, 60.55294873703923031 ) ) ;
#44022=CARTESIAN_POINT ( 'NONE',  ( -14.25068859620041017, -8.513811488652077486, 70.72957628655862550 ) ) ;
#44023=ORIENTED_EDGE ( 'NONE', *, *, #15125, .T. ) ;
#44026=CARTESIAN_POINT ( 'NONE',  ( -14.74982318541341364, -21.33234577674026156, 58.46617888512912486 ) ) ;
#44027=EDGE_CURVE ( 'NONE', #15877, #45956, #35039, .T. ) ;
#44028=CARTESIAN_POINT ( 'NONE',  ( -21.54693431995308828, -8.603789849366368259, 73.76162071728887781 ) ) ;
#44029=VERTEX_POINT ( 'NONE', #37114 ) ;
#44031=FACE_OUTER_BOUND ( 'NONE', #3309, .T. ) ;
#44033=ORIENTED_EDGE ( 'NONE', *, *, #36793, .T. ) ;
#44036=CARTESIAN_POINT ( 'NONE',  ( -13.12613471901881113, -20.89454346209081947, 58.16154795605982031 ) ) ;
#44037=B_SPLINE_CURVE_WITH_KNOTS ( 'NONE', 3,
 ( #28813, #10353, #25366, #29296, #47535, #21666, #44333, #6648, #17947, #36655 ),
 .UNSPECIFIED., .F., .F.,
 ( 4, 2, 2, 2, 4 ),
 ( 0.6272669072782339761, 0.7522669073001400086, 0.8772669073220461522, 1.002266907343952296, 1.127266907365858328 ),
 .UNSPECIFIED. ) ;
#44039=CARTESIAN_POINT ( 'NONE',  ( -23.89200535028185612, -11.11192396016905448, 70.07706043178237110 ) ) ;
#44040=DIRECTION ( 'NONE',  ( -5.828394480008251615E-08, 1.590814170208496341E-07, 0.9999999999999855671 ) ) ;
#44041=CARTESIAN_POINT ( 'NONE',  ( -13.04382658994076927, -9.348978013824847721, 67.45230756976776831 ) ) ;
#44042=EDGE_CURVE ( 'NONE', #33165, #27092, #15197, .T. ) ;
#44043=CARTESIAN_POINT ( 'NONE',  ( -14.80768872953871629, -21.78479300179184719, 61.81317360619090095 ) ) ;
#44044=VECTOR ( 'NONE', #23865, 1000.000000000000227 ) ;
#44045=ORIENTED_EDGE ( 'NONE', *, *, #72, .T. ) ;
#44046=ORIENTED_EDGE ( 'NONE', *, *, #15111, .T. ) ;
#44047=B_SPLINE_CURVE_WITH_KNOTS ( 'NONE', 1,
 ( #32575, #10181 ),
 .UNSPECIFIED., .F., .F.,
 ( 2, 2 ),
 ( 0.000000000000000000, 1.000000000000000000 ),
 .UNSPECIFIED. ) ;
#44048=CYLINDRICAL_SURFACE ( 'NONE', #28898, 0.1500000000000047962 ) ;
#44049=DIRECTION ( 'NONE',  ( 0.03181436478788692013, 0.9994937949748079475, 6.982004199025367595E-09 ) ) ;
#44052=CARTESIAN_POINT ( 'NONE',  ( -10.38277322391999746, -14.45650603033957005, 67.86359899216145664 ) ) ;
#44055=VERTEX_POINT ( 'NONE', #18166 ) ;
#44057=CARTESIAN_POINT ( 'NONE',  ( -22.05923734882601295, -20.05472318235705131, 62.53439162613685909 ) ) ;
#44060=ADVANCED_FACE ( 'NONE', ( #37864 ), #29757, .T. ) ;
#44062=CARTESIAN_POINT ( 'NONE',  ( -11.21783165637758550, -18.93062460193366192, 64.93202459354702683 ) ) ;
#44064=CARTESIAN_POINT ( 'NONE',  ( -13.47381639519378105, -21.12577003491056260, 65.24274829841968426 ) ) ;
#44065=AXIS2_PLACEMENT_3D ( 'NONE', #43019, #24075, #38838 ) ;
#44068=EDGE_CURVE ( 'NONE', #1136, #8232, #39477, .T. ) ;
#44069=CARTESIAN_POINT ( 'NONE',  ( -21.42336380182764088, -21.09487415076890215, 69.23945570945444672 ) ) ;
#44071=DIRECTION ( 'NONE',  ( 0.4683180279402421875, -0.8835599723313410925, 4.589753183357165266E-08 ) ) ;
#44073=EDGE_CURVE ( 'NONE', #19236, #38546, #11454, .T. ) ;
#44076=FACE_OUTER_BOUND ( 'NONE', #10492, .T. ) ;
#44077=ORIENTED_EDGE ( 'NONE', *, *, #29778, .F. ) ;
#44078=EDGE_CURVE ( 'NONE', #40518, #10306, #2488, .T. ) ;
#44086=VERTEX_POINT ( 'NONE', #9053 ) ;
#44087=CARTESIAN_POINT ( 'NONE',  ( -24.23813412381375088, -12.99935709875259526, 66.31718868320673721 ) ) ;
#44088=CARTESIAN_POINT ( 'NONE',  ( -17.11594671439511828, -7.315539529225058679, 53.49999999999994316 ) ) ;
#44089=CARTESIAN_POINT ( 'NONE',  ( -23.08280660609100465, -10.60377317445056811, 59.61675562601556067 ) ) ;
#44090=ORIENTED_EDGE ( 'NONE', *, *, #29312, .F. ) ;
#44093=CARTESIAN_POINT ( 'NONE',  ( -11.07857854458970692, -11.73724703412850623, 71.08860870961423473 ) ) ;
#44095=B_SPLINE_CURVE_WITH_KNOTS ( 'NONE', 1,
 ( #26844, #27798 ),
 .UNSPECIFIED., .F., .F.,
 ( 2, 2 ),
 ( 0.000000000000000000, 1.000000000000000000 ),
 .UNSPECIFIED. ) ;
#44096=CARTESIAN_POINT ( 'NONE',  ( -19.47262290702580501, -4.225005811476141737, 54.49999999999995026 ) ) ;
#44098=CARTESIAN_POINT ( 'NONE',  ( -24.08907123645992243, -11.48026457312919391, 63.13713595337925000 ) ) ;
#44099=CARTESIAN_POINT ( 'NONE',  ( -13.75915741662262270, -20.84105630778929097, 72.07040738930723478 ) ) ;
#44100=CARTESIAN_POINT ( 'NONE',  ( -20.52989715560836714, -8.037455129638530593, 66.98092865364507986 ) ) ;
#44103=CARTESIAN_POINT ( 'NONE',  ( -21.96070222398937943, -20.20571033069026257, 59.06442882800701710 ) ) ;
#44104=EDGE_CURVE ( 'NONE', #300, #28014, #23590, .T. ) ;
#44105=CARTESIAN_POINT ( 'NONE',  ( -13.97628689860590079, -8.204186434626230096, 70.84302338899487950 ) ) ;
#44106=AXIS2_PLACEMENT_3D ( 'NONE', #44365, #33480, #40643 ) ;
#44111=ORIENTED_EDGE ( 'NONE', *, *, #8078, .T. ) ;
#44112=CARTESIAN_POINT ( 'NONE',  ( -16.96883228653983267, -7.373121007882340372, 74.16007052498633811 ) ) ;
#44113=CARTESIAN_POINT ( 'NONE',  ( -23.66704192603476287, -11.64274840793925136, 63.23752948021675735 ) ) ;
#44114=FACE_OUTER_BOUND ( 'NONE', #45671, .T. ) ;
#44115=CARTESIAN_POINT ( 'NONE',  ( -11.66853631837921057, -18.88083403034671193, 68.51129807381201431 ) ) ;
#44116=VECTOR ( 'NONE', #17432, 1000.000000000000227 ) ;
#44117=( BOUNDED_CURVE ( )  B_SPLINE_CURVE ( 3, ( #37832, #15405, #33631, #19126 ),
 .UNSPECIFIED., .F., .F. ) 
 B_SPLINE_CURVE_WITH_KNOTS ( ( 4, 4 ),
 ( 4.712388980384689674, 4.921828490623996188 ),
 .UNSPECIFIED. ) 
 CURVE ( )  GEOMETRIC_REPRESENTATION_ITEM ( )  RATIONAL_B_SPLINE_CURVE ( ( 1.000000000000000000, 0.9963479302455159337, 0.9963479302455159337, 1.000000000000000000 ) ) 
 REPRESENTATION_ITEM ( '' )  );
#44118=ORIENTED_EDGE ( 'NONE', *, *, #8514, .F. ) ;
#44119=DIRECTION ( 'NONE',  ( -0.6973657521612036669, 0.7167154300785205656, -1.015100525525034718E-08 ) ) ;
#44120=CARTESIAN_POINT ( 'NONE',  ( -13.68776306357628236, -20.79195502325622158, 68.54805381681681808 ) ) ;
#44121=AXIS2_PLACEMENT_3D ( 'NONE', #3578, #41993, #41497 ) ;
#44124=CARTESIAN_POINT ( 'NONE',  ( -19.70639647806698136, -21.90109437720271757, 65.57990800639531415 ) ) ;
#44125=CARTESIAN_POINT ( 'NONE',  ( -16.80787187392568782, -21.83226421674134343, 68.99560634640492651 ) ) ;
#44126=ORIENTED_EDGE ( 'NONE', *, *, #27739, .F. ) ;
#44127=( BOUNDED_CURVE ( )  B_SPLINE_CURVE ( 3, ( #18951, #45311, #4190, #45559 ),
 .UNSPECIFIED., .F., .F. ) 
 B_SPLINE_CURVE_WITH_KNOTS ( ( 4, 4 ),
 ( 0.4074455897393688963, 0.5000000000000000000 ),
 .UNSPECIFIED. ) 
 CURVE ( )  GEOMETRIC_REPRESENTATION_ITEM ( )  RATIONAL_B_SPLINE_CURVE ( ( 0.6983129098261010581, 0.7760317562607195185, 0.8765941196520234957, 1.000000000000022871 ) ) 
 REPRESENTATION_ITEM ( '' )  );
#44128=CARTESIAN_POINT ( 'NONE',  ( -19.45281838860202228, -9.697037067072804106, 54.07175714974879099 ) ) ;
#44129=VERTEX_POINT ( 'NONE', #42782 ) ;
#44130=CARTESIAN_POINT ( 'NONE',  ( -19.33060681123161828, -8.018134805169733426, 63.52269467617171728 ) ) ;
#44131=CARTESIAN_POINT ( 'NONE',  ( -13.54822921233619226, -20.69819393533649077, 61.51646323540209949 ) ) ;
#44132=AXIS2_PLACEMENT_3D ( 'NONE', #3889, #3382, #14673 ) ;
#44133=CARTESIAN_POINT ( 'NONE',  ( -24.39889571797764845, -14.21434815047959255, 69.95275261040420389 ) ) ;
#44134=EDGE_LOOP ( 'NONE', ( #40633, #31186, #47279, #43247, #14446 ) ) ;
#44135=CARTESIAN_POINT ( 'NONE',  ( -24.17712593706266233, -17.95560904427356519, 59.19652577575318730 ) ) ;
#44136=EDGE_CURVE ( 'NONE', #32972, #29603, #44804, .T. ) ;
#44137=EDGE_CURVE ( 'NONE', #11451, #39638, #27029, .T. ) ;
#44138=CARTESIAN_POINT ( 'NONE',  ( -24.47405849404658795, -12.40054206295432770, 73.28579645182460922 ) ) ;
#44140=AXIS2_PLACEMENT_3D ( 'NONE', #14699, #11056, #26079 ) ;
#44141=CARTESIAN_POINT ( 'NONE',  ( -24.86251202286899442, -14.39255128295101471, 66.22646819999783929 ) ) ;
#44145=CARTESIAN_POINT ( 'NONE',  ( -22.79734409636068904, -10.24514240368273477, 66.54182257473807738 ) ) ;
#44146=( BOUNDED_CURVE ( )  B_SPLINE_CURVE ( 3, ( #31817, #23955, #9667, #28373 ),
 .UNSPECIFIED., .F., .F. ) 
 B_SPLINE_CURVE_WITH_KNOTS ( ( 4, 4 ),
 ( 0.000000000000000000, 0.4074455897393651216 ),
 .UNSPECIFIED. ) 
 CURVE ( )  GEOMETRIC_REPRESENTATION_ITEM ( )  RATIONAL_B_SPLINE_CURVE ( ( 1.000000000000000000, 0.4567392136813256953, 0.3561768502900279909, 0.6983129098261068313 ) ) 
 REPRESENTATION_ITEM ( '' )  );
#44147=FACE_OUTER_BOUND ( 'NONE', #3884, .T. ) ;
#44151=CARTESIAN_POINT ( 'NONE',  ( -13.19650781164887832, -20.94374207671370058, 58.20683400836775689 ) ) ;
#44152=CARTESIAN_POINT ( 'NONE',  ( -16.16379340615718618, -22.15191857530921382, 58.47080845268740035 ) ) ;
#44153=CARTESIAN_POINT ( 'NONE',  ( -24.26463774145634034, -13.10332622516414069, 63.13264148103307605 ) ) ;
#44154=EDGE_LOOP ( 'NONE', ( #46104, #36216, #14469, #43204, #31220 ) ) ;
#44156=CARTESIAN_POINT ( 'NONE',  ( -11.46028008028683942, -18.56947564720590194, 61.56238700194530367 ) ) ;
#44157=CARTESIAN_POINT ( 'NONE',  ( -10.47613650077225600, -13.59292889141194216, 74.88637490168683541 ) ) ;
#44158=ORIENTED_EDGE ( 'NONE', *, *, #35349, .T. ) ;
#44159=CARTESIAN_POINT ( 'NONE',  ( -23.99387123153590551, -11.29613222128559258, 66.46568589023691231 ) ) ;
#44161=CARTESIAN_POINT ( 'NONE',  ( -24.19351354463141845, -13.02564601667185151, 66.31863419436056972 ) ) ;
#44162=CARTESIAN_POINT ( 'NONE',  ( -11.77467277675836321, -9.951459619914194477, 64.14259051640634368 ) ) ;
#44163=CARTESIAN_POINT ( 'NONE',  ( -12.15470796376391682, -20.07677110164151557, 61.51023378490003068 ) ) ;
#44165=FACE_BOUND ( 'NONE', #8302, .T. ) ;
#44166=CARTESIAN_POINT ( 'NONE',  ( -24.82750195234013191, -13.97654432178796569, 73.30766915316792165 ) ) ;
#44167=LINE ( 'NONE', #18009, #5119 ) ;
#44168=CARTESIAN_POINT ( 'NONE',  ( -11.49500183448702906, -10.99442376238782515, 57.22375354680192316 ) ) ;
#44169=EDGE_CURVE ( 'NONE', #40684, #25938, #38855, .T. ) ;
#44170=VERTEX_POINT ( 'NONE', #35132 ) ;
#44173=DIRECTION ( 'NONE',  ( 3.549360974554993999E-17, -6.371834667797928663E-18, -1.000000000000000000 ) ) ;
#44174=DIRECTION ( 'NONE',  ( -2.083496777882594458E-06, 1.347747145367441676E-07, 0.9999999999978204102 ) ) ;
#44175=CARTESIAN_POINT ( 'NONE',  ( -20.82683693055541596, -21.43676851416161355, 58.83813467579677337 ) ) ;
#44176=CARTESIAN_POINT ( 'NONE',  ( -11.22470860480879118, -11.43539691024457206, 71.23293728648457090 ) ) ;
#44177=CARTESIAN_POINT ( 'NONE',  ( -16.46055793053448113, -21.74386666130517298, 65.45394323774524992 ) ) ;
#44178=ORIENTED_EDGE ( 'NONE', *, *, #30490, .F. ) ;
#44179=EDGE_LOOP ( 'NONE', ( #30517, #28504, #8853, #41104, #23654 ) ) ;
#44182=CARTESIAN_POINT ( 'NONE',  ( -17.13276323845814630, -21.80314153100133723, 72.35646425281650806 ) ) ;
#44183=AXIS2_PLACEMENT_3D ( 'NONE', #587, #15582, #30645 ) ;
#44184=CARTESIAN_POINT ( 'NONE',  ( -20.11563963094288354, -8.345964892081962461, 73.94926364880660685 ) ) ;
#44185=B_SPLINE_CURVE_WITH_KNOTS ( 'NONE', 3,
 ( #29586, #298, #11125, #41396, #26381, #7688, #47, #10405, #48292, #2992 ),
 .UNSPECIFIED., .F., .F.,
 ( 4, 2, 2, 2, 4 ),
 ( 0.000000000000000000, 0.2500000000000000000, 0.5000000000000000000, 0.7500000000000000000, 1.000000000000000000 ),
 .UNSPECIFIED. ) ;
#44186=CARTESIAN_POINT ( 'NONE',  ( -15.42576764927216892, -7.632088794545897947, 74.25798431274822065 ) ) ;
#44190=CARTESIAN_POINT ( 'NONE',  ( -19.37616851487812752, -21.99900361761337919, 58.71002773933979313 ) ) ;
#44196=ORIENTED_EDGE ( 'NONE', *, *, #27398, .F. ) ;
#44197=CARTESIAN_POINT ( 'NONE',  ( -21.35412623182586955, -20.66579906811421452, 68.93961316870652922 ) ) ;
#44198=DIRECTION ( 'NONE',  ( -1.069446448411283641E-06, 1.103879804260444988E-06, -0.9999999999988188337 ) ) ;
#44199=ORIENTED_EDGE ( 'NONE', *, *, #32345, .F. ) ;
#44201=EDGE_CURVE ( 'NONE', #34833, #42067, #26565, .T. ) ;
#44204=CARTESIAN_POINT ( 'NONE',  ( -15.28291064399146215, -21.52618758091310980, 68.57592918174772478 ) ) ;
#44205=ORIENTED_EDGE ( 'NONE', *, *, #33934, .F. ) ;
#44206=DIRECTION ( 'NONE',  ( 0.9774082387306983755, -0.2113602016968848529, 7.903122840289807171E-08 ) ) ;
#44208=CARTESIAN_POINT ( 'NONE',  ( -23.83043773139749533, -11.86620498678314561, 59.78235732590890450 ) ) ;
#44209=EDGE_CURVE ( 'NONE', #20573, #13987, #42549, .T. ) ;
#44211=CARTESIAN_POINT ( 'NONE',  ( -11.73296596577226936, -10.64774513788296240, 74.72412863062541533 ) ) ;
#44212=EDGE_CURVE ( 'NONE', #34242, #1270, #39072, .T. ) ;
#44214=CARTESIAN_POINT ( 'NONE',  ( -12.05806040642128707, -10.23620046216302448, 67.51368956197082127 ) ) ;
#44216=CARTESIAN_POINT ( 'NONE',  ( -15.03427660820159772, -21.44211488324610571, 65.12068745241758450 ) ) ;
#44217=EDGE_CURVE ( 'NONE', #10695, #13075, #43345, .T. ) ;
#44218=DIRECTION ( 'NONE',  ( -0.9893521221787096032, 0.1455416721783832079, 6.188545272020285247E-08 ) ) ;
#44222=VERTEX_POINT ( 'NONE', #19396 ) ;
#44223=ORIENTED_EDGE ( 'NONE', *, *, #28098, .F. ) ;
#44224=CARTESIAN_POINT ( 'NONE',  ( -16.19813999035177332, -21.75179513556690480, 58.28585572029249562 ) ) ;
#44226=DIRECTION ( 'NONE',  ( -3.827383491158052452E-06, 8.363078748037870009E-06, 0.9999999999577049437 ) ) ;
#44227=CARTESIAN_POINT ( 'NONE',  ( -12.80657247161177814, -9.477853225175101315, 70.73436560138682694 ) ) ;
#44228=ORIENTED_EDGE ( 'NONE', *, *, #3571, .T. ) ;
#44229=ORIENTED_EDGE ( 'NONE', *, *, #28706, .T. ) ;
#44235=CARTESIAN_POINT ( 'NONE',  ( -17.42409385541300892, -14.80920654474439324, 53.49899999999994549 ) ) ;
#44236=CYLINDRICAL_SURFACE ( 'NONE', #30746, 0.1500000000000035749 ) ;
#44237=DIRECTION ( 'NONE',  ( -2.872222159185455981E-06, 2.507089443456002334E-06, 0.9999999999927324801 ) ) ;
#44238=EDGE_CURVE ( 'NONE', #32800, #2641, #1257, .T. ) ;
#44240=CARTESIAN_POINT ( 'NONE',  ( -10.42334066387008029, -15.64104445138816324, 61.03789045260960933 ) ) ;
#44242=CARTESIAN_POINT ( 'NONE',  ( -20.83700022493356130, -19.12221826660257307, 53.49999999999995026 ) ) ;
#44243=CARTESIAN_POINT ( 'NONE',  ( -15.12736045941317897, -21.89643407171298151, 68.69097498501147925 ) ) ;
#44244=CARTESIAN_POINT ( 'NONE',  ( -24.42364817991657588, -14.92042613324309208, 59.52683630610148668 ) ) ;
#44245=VERTEX_POINT ( 'NONE', #30740 ) ;
#44246=CARTESIAN_POINT ( 'NONE',  ( -24.09823712565756182, -12.53788967028716783, 73.54225559392006062 ) ) ;
#44248=LINE ( 'NONE', #22066, #23708 ) ;
#44249=VERTEX_POINT ( 'NONE', #45767 ) ;
#44250=CARTESIAN_POINT ( 'NONE',  ( -24.82559196212071484, -15.65839247127784972, 73.11029605187583513 ) ) ;
#44251=CYLINDRICAL_SURFACE ( 'NONE', #3808, 0.1500000000000073774 ) ;
#44252=CARTESIAN_POINT ( 'NONE',  ( -10.96921284960095377, -11.97350354382807680, 74.84368195529052059 ) ) ;
#44253=ORIENTED_EDGE ( 'NONE', *, *, #31751, .F. ) ;
#44254=CARTESIAN_POINT ( 'NONE',  ( -13.24006525392636391, -20.97423447465198976, 61.70301720779925603 ) ) ;
#44255=VERTEX_POINT ( 'NONE', #5838 ) ;
#44256=CARTESIAN_POINT ( 'NONE',  ( -12.40538999107997498, -20.31523868419091272, 68.52152871938794476 ) ) ;
#44257=CARTESIAN_POINT ( 'NONE',  ( -13.77338061488629073, -21.30427811955188844, 68.56969753575143045 ) ) ;
#44258=CARTESIAN_POINT ( 'NONE',  ( -24.42003622094757276, -14.56910621572103715, 62.99831180156633081 ) ) ;
#44259=EDGE_CURVE ( 'NONE', #11465, #30525, #26950, .T. ) ;
#44262=CARTESIAN_POINT ( 'NONE',  ( -24.18037252889021005, -17.94870914462638822, 59.18873732074431615 ) ) ;
#44263=ADVANCED_FACE ( 'NONE', ( #21347 ), #9542, .T. ) ;
#44264=CARTESIAN_POINT ( 'NONE',  ( -18.99427849551180358, -7.526545565697431606, 67.10060551660288297 ) ) ;
#44265=( BOUNDED_CURVE ( )  B_SPLINE_CURVE ( 3, ( #11282, #19147, #33920, #34647 ),
 .UNSPECIFIED., .F., .F. ) 
 B_SPLINE_CURVE_WITH_KNOTS ( ( 4, 4 ),
 ( 0.000000000000000000, 0.4074455897393777226 ),
 .UNSPECIFIED. ) 
 CURVE ( )  GEOMETRIC_REPRESENTATION_ITEM ( )  RATIONAL_B_SPLINE_CURVE ( ( 1.000000000000000000, 0.4567392136813100967, 0.3561768502900222177, 0.6983129098261363632 ) ) 
 REPRESENTATION_ITEM ( '' )  );
#44266=CARTESIAN_POINT ( 'NONE',  ( -15.35181094580836358, -7.653138554841501850, 74.12339718037890179 ) ) ;
#44268=CARTESIAN_POINT ( 'NONE',  ( -10.37795889460693033, -14.56696403379599403, 68.14328054657653411 ) ) ;
#44269=ADVANCED_FACE ( 'NONE', ( #9292 ), #29813, .T. ) ;
#44270=CARTESIAN_POINT ( 'NONE',  ( -12.23301264461619553, -10.03852782535897958, 60.84446034103241630 ) ) ;
#44271=EDGE_LOOP ( 'NONE', ( #40049, #12156, #41121, #938, #28689 ) ) ;
#44273=CARTESIAN_POINT ( 'NONE',  ( -14.99555751708010121, -21.85235056220836469, 65.14950770721691242 ) ) ;
#44274=CARTESIAN_POINT ( 'NONE',  ( -19.88526120935579655, -21.36290167704760279, 72.68255599050156945 ) ) ;
#44275=CARTESIAN_POINT ( 'NONE',  ( -15.82259855879412846, -7.533287975791289171, 67.25511890406325222 ) ) ;
#44276=CARTESIAN_POINT ( 'NONE',  ( -23.89200535028185612, -11.11192396016905448, 70.07706043178237110 ) ) ;
#44278=CARTESIAN_POINT ( 'NONE',  ( -24.23813412381375088, -12.99935709875259526, 66.31718868320673721 ) ) ;
#44281=( BOUNDED_SURFACE ( )  B_SPLINE_SURFACE ( 3, 1, ( 
 ( #4139, #442 ),
 ( #15417, #30486 ),
 ( #45499, #11757 ),
 ( #41801, #8082 ),
 ( #38083, #670 ),
 ( #19378, #31917 ),
 ( #39782, #43740 ) ),
 .UNSPECIFIED., .T., .F., .F. ) 
 B_SPLINE_SURFACE_WITH_KNOTS ( ( 4, 3, 4 ),
 ( 2, 2 ),
 ( 0.000000000000000000, 0.5000000000000000000, 1.000000000000000000 ),
 ( 0.000000000000000000, 1.000000000000000000 ),
 .UNSPECIFIED. ) 
 GEOMETRIC_REPRESENTATION_ITEM ( )  RATIONAL_B_SPLINE_SURFACE ( (
 ( 1.000000000000000000, 1.000000000000000000),
 ( 0.3333333333333335369, 0.3333333333333330373),
 ( 0.3333333333333335369, 0.3333333333333330373),
 ( 1.000000000000000000, 1.000000000000000000),
 ( 0.3333333333333333703, 0.3333333333333333703),
 ( 0.3333333333333333703, 0.3333333333333333703),
 ( 1.000000000000000000, 1.000000000000000000) ) ) 
 REPRESENTATION_ITEM ( '' )  SURFACE ( )  );
#44282=ORIENTED_EDGE ( 'NONE', *, *, #1704, .F. ) ;
#44284=CARTESIAN_POINT ( 'NONE',  ( -13.43921731646364925, -8.993429882417945720, 60.43950277494440826 ) ) ;
#44286=CARTESIAN_POINT ( 'NONE',  ( -23.76176040870155148, -11.71284927192775527, 66.51394613547601864 ) ) ;
#44287=CARTESIAN_POINT ( 'NONE',  ( -13.88539965413766453, -8.253282245057402378, 74.34954655571560522 ) ) ;
#44291=VERTEX_POINT ( 'NONE', #9780 ) ;
#44292=CARTESIAN_POINT ( 'NONE',  ( -24.33858675457341292, -15.90816096490859088, 69.60477842452804964 ) ) ;
#44294=AXIS2_PLACEMENT_3D ( 'NONE', #34834, #7787, #1106 ) ;
#44295=PLANE ( 'NONE',  #22958 ) ;
#44296=CARTESIAN_POINT ( 'NONE',  ( -11.17079691907060202, -18.85905423163385564, 64.90853625290334605 ) ) ;
#44300=CARTESIAN_POINT ( 'NONE',  ( -23.85820194903862657, -17.69173191509663567, 62.48833042115954584 ) ) ;
#44301=ORIENTED_EDGE ( 'NONE', *, *, #5603, .T. ) ;
#44302=CARTESIAN_POINT ( 'NONE',  ( -24.20371252810814866, -12.87440185077122834, 66.58774614429587757 ) ) ;
#44303=CARTESIAN_POINT ( 'NONE',  ( -21.34582024633207098, -20.66775256773563285, 72.67446429491059234 ) ) ;
#44304=ORIENTED_EDGE ( 'NONE', *, *, #43461, .F. ) ;
#44305=EDGE_CURVE ( 'NONE', #9970, #6766, #6067, .T. ) ;
#44306=FACE_OUTER_BOUND ( 'NONE', #25755, .T. ) ;
#44307=ORIENTED_EDGE ( 'NONE', *, *, #30238, .F. ) ;
#44308=CARTESIAN_POINT ( 'NONE',  ( -21.71330648800491048, -9.209429688968461036, 70.43132803184890633 ) ) ;
#44309=CARTESIAN_POINT ( 'NONE',  ( -24.31477923169101629, -16.30090137217950996, 59.40860294853779777 ) ) ;
#44310=VERTEX_POINT ( 'NONE', #2130 ) ;
#44311=CARTESIAN_POINT ( 'NONE',  ( -18.42425741750128765, -21.73782862702753249, 72.30127622548401689 ) ) ;
#44312=CARTESIAN_POINT ( 'NONE',  ( -24.40650426928521100, -17.40698345136521752, 69.56339792804031674 ) ) ;
#44314=ORIENTED_EDGE ( 'NONE', *, *, #13950, .T. ) ;
#44315=CARTESIAN_POINT ( 'NONE',  ( -18.71756812234623979, -7.929749856837892352, 70.67068030594712980 ) ) ;
#44316=CARTESIAN_POINT ( 'NONE',  ( -11.11213569393138023, -18.76700539655533362, 61.41564285493458897 ) ) ;
#44317=CARTESIAN_POINT ( 'NONE',  ( -21.59705452237689371, -8.637577456526162933, 73.80139960705861313 ) ) ;
#44319=CARTESIAN_POINT ( 'NONE',  ( -13.51260394713023416, -21.14978044785226530, 65.18617648760555028 ) ) ;
#44321=DIRECTION ( 'NONE',  ( 0.8839923186919885767, -0.4675014229855998793, 2.842058574697910297E-08 ) ) ;
#44323=AXIS2_PLACEMENT_3D ( 'NONE', #6986, #44920, #17568 ) ;
#44324=ORIENTED_EDGE ( 'NONE', *, *, #21760, .T. ) ;
#44325=ORIENTED_EDGE ( 'NONE', *, *, #24068, .F. ) ;
#44326=CARTESIAN_POINT ( 'NONE',  ( -22.57893663749957369, -9.999394138389963160, 73.49633153340955971 ) ) ;
#44327=CARTESIAN_POINT ( 'NONE',  ( -16.93043456194158125, -7.826573929305837396, 74.24552922955767542 ) ) ;
#44328=CARTESIAN_POINT ( 'NONE',  ( -11.44771684537310463, -11.06942230959719176, 57.50903181645943363 ) ) ;
#44329=ADVANCED_FACE ( 'NONE', ( #17856 ), #32879, .T. ) ;
#44331=CARTESIAN_POINT ( 'NONE',  ( -23.21283114448125673, -10.11939864774917908, 63.25681283445349123 ) ) ;
#44332=CARTESIAN_POINT ( 'NONE',  ( -12.90227214125716237, -8.888328675545798419, 67.63588728319849963 ) ) ;
#44333=CARTESIAN_POINT ( 'NONE',  ( -23.68746034620986762, -18.84317387556108514, 69.39348344656710310 ) ) ;
#44334=DIRECTION ( 'NONE',  ( -5.517078746805382707E-07, -1.257343593493847808E-06, -0.9999999999990573096 ) ) ;
#44335=ORIENTED_EDGE ( 'NONE', *, *, #27122, .F. ) ;
#44336=DIRECTION ( 'NONE',  ( 2.696738943264045022E-06, 1.002714486673431828E-05, 0.9999999999460920108 ) ) ;
#44337=CARTESIAN_POINT ( 'NONE',  ( -18.31357640787765462, -21.80286941108919763, 68.81514702304139064 ) ) ;
#44339=EDGE_CURVE ( 'NONE', #20830, #21555, #36339, .T. ) ;
#44341=VERTEX_POINT ( 'NONE', #35614 ) ;
#44343=ADVANCED_FACE ( 'NONE', ( #31931 ), #39562, .T. ) ;
#44346=CARTESIAN_POINT ( 'NONE',  ( -10.00655543316878493, -14.11314255069943258, 61.09538170931386958 ) ) ;
#44347=CARTESIAN_POINT ( 'NONE',  ( -24.30515140815569097, -13.27439714384899183, 59.65708100345488418 ) ) ;
#44348=( BOUNDED_CURVE ( )  B_SPLINE_CURVE ( 3, ( #3185, #6163, #21189, #29533 ),
 .UNSPECIFIED., .F., .F. ) 
 B_SPLINE_CURVE_WITH_KNOTS ( ( 4, 4 ),
 ( 0.9074455897393657322, 1.000000000000000000 ),
 .UNSPECIFIED. ) 
 CURVE ( )  GEOMETRIC_REPRESENTATION_ITEM ( )  RATIONAL_B_SPLINE_CURVE ( ( 0.6983129098260905110, 0.7760317562606959818, 0.8765941196519991818, 1.000000000000000000 ) ) 
 REPRESENTATION_ITEM ( '' )  );
#44350=CARTESIAN_POINT ( 'NONE',  ( -12.50766578132126838, -19.86205079821699471, 65.16674886870754335 ) ) ;
#44351=FACE_OUTER_BOUND ( 'NONE', #28787, .T. ) ;
#44355=CARTESIAN_POINT ( 'NONE',  ( -19.69975549639545420, -21.90326680182264596, 65.64298972507442897 ) ) ;
#44356=CARTESIAN_POINT ( 'NONE',  ( -22.87867891474110849, -19.28048576922455837, 59.29899440274890310 ) ) ;
#44359=VERTEX_POINT ( 'NONE', #29947 ) ;
#44360=CARTESIAN_POINT ( 'NONE',  ( -10.46561413896930581, -17.47044525196274734, 64.82728164928992953 ) ) ;
#44361=CARTESIAN_POINT ( 'NONE',  ( -24.40217300928714650, -14.25566238011515274, 69.65275273531472067 ) ) ;
#44362=ORIENTED_EDGE ( 'NONE', *, *, #12621, .F. ) ;
#44363=CARTESIAN_POINT ( 'NONE',  ( -10.41336640449534734, -12.28884930470453085, 57.47857332146136855 ) ) ;
#44364=CARTESIAN_POINT ( 'NONE',  ( -20.03165646395635591, -8.259115988876370551, 73.72096593878789861 ) ) ;
#44365=CARTESIAN_POINT ( 'NONE',  ( -12.64995480627295521, -19.99670077279894898, 68.48657438322858582 ) ) ;
#44366=CARTESIAN_POINT ( 'NONE',  ( -24.01844669341070926, -17.32505205508840262, 62.62928254837112974 ) ) ;
#44368=DIRECTION ( 'NONE',  ( 0.9271861211590526342, 0.3746009833543293421, -1.005599061620490611E-08 ) ) ;
#44369=ORIENTED_EDGE ( 'NONE', *, *, #16880, .F. ) ;
#44370=B_SPLINE_CURVE_WITH_KNOTS ( 'NONE', 3,
 ( #46218, #8807, #23823, #5102, #9278, #20112, #35120, #39057, #1640, #16650 ),
 .UNSPECIFIED., .F., .F.,
 ( 4, 2, 2, 2, 4 ),
 ( 0.000000000000000000, 0.2500000000000000000, 0.5000000000000000000, 0.7500000000000000000, 1.000000000000000000 ),
 .UNSPECIFIED. ) ;
#44371=DIRECTION ( 'NONE',  ( 0.9048399035850772654, 0.4257519804770707461, 1.330923649722295902E-08 ) ) ;
#44372=DIRECTION ( 'NONE',  ( -0.9529680021988313765, 0.3030709269876716849, 3.918663088761644638E-08 ) ) ;
#44374=DIRECTION ( 'NONE',  ( -0.9893521221787096032, 0.1455416721783832079, 6.188545272020283923E-08 ) ) ;
#44376=CARTESIAN_POINT ( 'NONE',  ( -13.35969120262891430, -20.57410711936033820, 61.60826610285024429 ) ) ;
#44379=VERTEX_POINT ( 'NONE', #14153 ) ;
#44381=CARTESIAN_POINT ( 'NONE',  ( -9.974456273375457371, -14.72748566909688073, 71.51278126739182994 ) ) ;
#44382=EDGE_LOOP ( 'NONE', ( #41709, #48056, #31600, #39410, #39115 ) ) ;
#44384=CARTESIAN_POINT ( 'NONE',  ( -24.16575310113231012, -12.74704012323608104, 70.07243002239954421 ) ) ;
#44386=FACE_BOUND ( 'NONE', #43553, .T. ) ;
#44387=CARTESIAN_POINT ( 'NONE',  ( -24.82598972713961771, -13.96249193466810823, 73.26124986525175586 ) ) ;
#44388=CARTESIAN_POINT ( 'NONE',  ( -10.42462062184586635, -14.89508117765250361, 75.09778901762284420 ) ) ;
#44389=VECTOR ( 'NONE', #17822, 1000.000000000000227 ) ;
#44395=CARTESIAN_POINT ( 'NONE',  ( -24.69822963474414479, -13.19963333263893190, 59.54763306486673713 ) ) ;
#44396=DIRECTION ( 'NONE',  ( -0.3037135924646501839, 0.9527633776296273727, 2.170275161112374231E-08 ) ) ;
#44397=CARTESIAN_POINT ( 'NONE',  ( -12.00790786851990610, -10.29148984397945377, 63.91425679989585973 ) ) ;
#44398=( BOUNDED_CURVE ( )  B_SPLINE_CURVE ( 3, ( #9301, #42059, #42557, #27995 ),
 .UNSPECIFIED., .F., .F. ) 
 B_SPLINE_CURVE_WITH_KNOTS ( ( 4, 4 ),
 ( 0.9074455897393648440, 1.000000000000000000 ),
 .UNSPECIFIED. ) 
 CURVE ( )  GEOMETRIC_REPRESENTATION_ITEM ( )  RATIONAL_B_SPLINE_CURVE ( ( 0.6983129098260973944, 0.7760317562607019770, 0.8765941196520028456, 1.000000000000000000 ) ) 
 REPRESENTATION_ITEM ( '' )  );
#44399=CARTESIAN_POINT ( 'NONE',  ( -14.66790711817407278, -21.29843871104708342, 58.18089935161520287 ) ) ;
#44400=CARTESIAN_POINT ( 'NONE',  ( -16.59344411340201475, -21.75974756046277747, 65.22564390621562325 ) ) ;
#44402=ORIENTED_EDGE ( 'NONE', *, *, #41307, .F. ) ;
#44403=ORIENTED_EDGE ( 'NONE', *, *, #20671, .F. ) ;
#44405=EDGE_LOOP ( 'NONE', ( #17719, #21087, #38440, #3755, #3271 ) ) ;
#44406=ADVANCED_FACE ( 'NONE', ( #11462 ), #7302, .T. ) ;
#44407=EDGE_CURVE ( 'NONE', #45657, #26697, #26005, .T. ) ;
#44408=CARTESIAN_POINT ( 'NONE',  ( -17.43166586245951422, -7.359124596637800053, 67.13544155391683432 ) ) ;
#44409=CARTESIAN_POINT ( 'NONE',  ( -18.85724798917316392, -7.906108138700305155, 67.18599644112759961 ) ) ;
#44410=( BOUNDED_CURVE ( )  B_SPLINE_CURVE ( 3, ( #10111, #25132, #7397, #41115 ),
 .UNSPECIFIED., .F., .F. ) 
 B_SPLINE_CURVE_WITH_KNOTS ( ( 4, 4 ),
 ( 0.5000000000000000000, 0.9074455897393650661 ),
 .UNSPECIFIED. ) 
 CURVE ( )  GEOMETRIC_REPRESENTATION_ITEM ( )  RATIONAL_B_SPLINE_CURVE ( ( 1.000000000000001998, 0.4567392136813319681, 0.3561768502900288791, 0.6983129098260947298 ) ) 
 REPRESENTATION_ITEM ( '' )  );
#44412=CARTESIAN_POINT ( 'NONE',  ( -12.96596534320165972, -9.347742485070138940, 70.84925352874383009 ) ) ;
#44413=ORIENTED_EDGE ( 'NONE', *, *, #44679, .T. ) ;
#44414=CARTESIAN_POINT ( 'NONE',  ( -13.65828898514496537, -20.76952646431350757, 65.00101022825411690 ) ) ;
#44416=ORIENTED_EDGE ( 'NONE', *, *, #39823, .F. ) ;
#44417=CARTESIAN_POINT ( 'NONE',  ( -10.37185532365394813, -14.67000050818549184, 74.88959094244134462 ) ) ;
#44419=( BOUNDED_SURFACE ( )  B_SPLINE_SURFACE ( 3, 1, ( 
 ( #47322, #28600 ),
 ( #47068, #9887 ),
 ( #9408, #39186 ),
 ( #13554, #39675 ),
 ( #5476, #5947 ),
 ( #39440, #36442 ),
 ( #2244, #36211 ) ),
 .UNSPECIFIED., .T., .F., .F. ) 
 B_SPLINE_SURFACE_WITH_KNOTS ( ( 4, 3, 4 ),
 ( 2, 2 ),
 ( 0.000000000000000000, 0.5000000000000000000, 1.000000000000000000 ),
 ( 0.000000000000000000, 1.000000000000000000 ),
 .UNSPECIFIED. ) 
 GEOMETRIC_REPRESENTATION_ITEM ( )  RATIONAL_B_SPLINE_SURFACE ( (
 ( 1.000000000000000000, 1.000000000000000000),
 ( 0.3333333333333335369, 0.3333333333333330373),
 ( 0.3333333333333335369, 0.3333333333333330373),
 ( 1.000000000000000000, 1.000000000000000000),
 ( 0.3333333333333333703, 0.3333333333333333703),
 ( 0.3333333333333333703, 0.3333333333333333703),
 ( 1.000000000000000000, 1.000000000000000000) ) ) 
 REPRESENTATION_ITEM ( '' )  SURFACE ( )  );
#44420=VECTOR ( 'NONE', #39169, 1000.000000000000000 ) ;
#44421=ORIENTED_EDGE ( 'NONE', *, *, #35121, .T. ) ;
#44422=CARTESIAN_POINT ( 'NONE',  ( -10.55151165865014384, -17.68520938540437371, 68.28217272534745064 ) ) ;
#44423=CARTESIAN_POINT ( 'NONE',  ( -15.12990733413706224, -8.194132228790286021, 57.03926990816982112 ) ) ;
#44424=CARTESIAN_POINT ( 'NONE',  ( -23.42631727757699878, -10.39480074052133141, 59.78858809748042091 ) ) ;
#44427=EDGE_CURVE ( 'NONE', #18572, #32337, #16855, .T. ) ;
#44428=VECTOR ( 'NONE', #30694, 1000.000000000000227 ) ;
#44430=CARTESIAN_POINT ( 'NONE',  ( -19.50843993236927432, -21.96177808838975665, 62.11008241541560437 ) ) ;
#44432=ORIENTED_EDGE ( 'NONE', *, *, #6754, .T. ) ;
#44433=B_SPLINE_CURVE_WITH_KNOTS ( 'NONE', 1,
 ( #42143, #8407 ),
 .UNSPECIFIED., .F., .F.,
 ( 2, 2 ),
 ( 0.000000000000000000, 1.000000000000000000 ),
 .UNSPECIFIED. ) ;
#44434=B_SPLINE_CURVE_WITH_KNOTS ( 'NONE', 3,
 ( #17656, #43783, #28523, #2647, #36366, #6348, #21379, #4969, #17161, #10291 ),
 .UNSPECIFIED., .F., .F.,
 ( 4, 2, 2, 2, 4 ),
 ( 0.1272669073658063144, 0.2522669073463020273, 0.3772669073267977957, 0.5022669073072935086, 0.6272669072877892216 ),
 .UNSPECIFIED. ) ;
#44436=CYLINDRICAL_SURFACE ( 'NONE', #22341, 0.1500000000000077383 ) ;
#44437=CARTESIAN_POINT ( 'NONE',  ( -23.66220297886838964, -18.88224728823589160, 69.55017934013164904 ) ) ;
#44440=CARTESIAN_POINT ( 'NONE',  ( -24.66692207690629246, -13.06418342283853562, 63.08910124536953390 ) ) ;
#44449=ORIENTED_EDGE ( 'NONE', *, *, #35898, .F. ) ;
#44451=CARTESIAN_POINT ( 'NONE',  ( -18.78945352633789057, -7.485380791038083181, 70.57056797142773519 ) ) ;
#44452=CARTESIAN_POINT ( 'NONE',  ( -15.93209805084403641, -7.970058305397211385, 63.77896932425708343 ) ) ;
#44453=CARTESIAN_POINT ( 'NONE',  ( -22.63668070846305724, -10.06225679001389040, 70.30618742561198076 ) ) ;
#44454=ORIENTED_EDGE ( 'NONE', *, *, #26599, .F. ) ;
#44455=ORIENTED_EDGE ( 'NONE', *, *, #40850, .F. ) ;
#44458=VECTOR ( 'NONE', #24532, 1000.000000000000114 ) ;
#44461=EDGE_CURVE ( 'NONE', #2275, #31856, #6505, .T. ) ;
#44462=EDGE_CURVE ( 'NONE', #19538, #1406, #25335, .T. ) ;
#44463=ORIENTED_EDGE ( 'NONE', *, *, #6592, .T. ) ;
#44466=CARTESIAN_POINT ( 'NONE',  ( -22.21932263989193856, -19.98213852671348434, 69.26597955412674423 ) ) ;
#44467=EDGE_CURVE ( 'NONE', #14528, #19458, #46455, .T. ) ;
#44468=CARTESIAN_POINT ( 'NONE',  ( -23.59167324040609870, -11.49507535768466227, 70.00283877229584562 ) ) ;
#44471=EDGE_LOOP ( 'NONE', ( #30801, #22318, #11740, #3902, #4883 ) ) ;
#44473=DIRECTION ( 'NONE',  ( 0.3506977235573930929, -0.2775087506578172158, 0.8944271909999157444 ) ) ;
#44474=CARTESIAN_POINT ( 'NONE',  ( -10.13751350317288669, -13.25697809452625009, 74.93463578866538910 ) ) ;
#44475=CARTESIAN_POINT ( 'NONE',  ( -21.59170415179237423, -20.98450529054885649, 72.71720556543249359 ) ) ;
#44476=EDGE_CURVE ( 'NONE', #12076, #21448, #44710, .T. ) ;
#44477=ORIENTED_EDGE ( 'NONE', *, *, #9661, .T. ) ;
#44478=CARTESIAN_POINT ( 'NONE',  ( -10.66137368835686416, -12.80659570974005668, 60.68364890423993785 ) ) ;
#44479=CARTESIAN_POINT ( 'NONE',  ( -15.33343222186064914, -21.95989685909981404, 72.23913770967520520 ) ) ;
#44480=B_SPLINE_CURVE_WITH_KNOTS ( 'NONE', 3,
 ( #32602, #37003, #10926, #40960, #3290, #18289, #13859, #40245, #33296, #6511 ),
 .UNSPECIFIED., .F., .F.,
 ( 4, 2, 2, 2, 4 ),
 ( 0.6272669072877791185, 0.7522669073073000590, 0.8772669073268208884, 1.002266907346341718, 1.127266907365862769 ),
 .UNSPECIFIED. ) ;
#44481=CARTESIAN_POINT ( 'NONE',  ( -19.42260780150576949, -7.632255095345715112, 60.06118752816730222 ) ) ;
#44482=CARTESIAN_POINT ( 'NONE',  ( -23.80321479583337307, -17.81075880182941873, 59.30378417737343710 ) ) ;
#44483=ORIENTED_EDGE ( 'NONE', *, *, #40281, .T. ) ;
#44484=CARTESIAN_POINT ( 'NONE',  ( -10.55151208239364635, -17.68521041179895548, 68.28217381303441869 ) ) ;
#44485=CARTESIAN_POINT ( 'NONE',  ( -21.39967327233876304, -20.63170314183283693, 72.80974286114339122 ) ) ;
#44486=CARTESIAN_POINT ( 'NONE',  ( -9.995738443926455830, -14.24059931954510816, 64.50308448303212572 ) ) ;
#44488=AXIS2_PLACEMENT_3D ( 'NONE', #21731, #48079, #37456 ) ;
#44489=FACE_BOUND ( 'NONE', #13190, .T. ) ;
#44490=ORIENTED_EDGE ( 'NONE', *, *, #12413, .F. ) ;
#44491=CARTESIAN_POINT ( 'NONE',  ( -18.24929096724884658, -21.81104555038653103, 68.82986815895560540 ) ) ;
#44493=CARTESIAN_POINT ( 'NONE',  ( -24.42122182511307571, -14.60447249519721069, 62.71296493455815124 ) ) ;
#44494=CARTESIAN_POINT ( 'NONE',  ( -10.02995815481606634, -13.89786978184575794, 57.63320425522585566 ) ) ;
#44495=ORIENTED_EDGE ( 'NONE', *, *, #23751, .F. ) ;
#44496=CARTESIAN_POINT ( 'NONE',  ( -23.83080496556880945, -17.75212211224490133, 59.28906343887996400 ) ) ;
#44498=CARTESIAN_POINT ( 'NONE',  ( -14.80966956416942004, -8.261851763560979833, 60.31996279529170835 ) ) ;
#44501=CARTESIAN_POINT ( 'NONE',  ( -11.21311628236200875, -18.92344944615173929, 64.85368745296808868 ) ) ;
#44504=ORIENTED_EDGE ( 'NONE', *, *, #47532, .T. ) ;
#44506=DIRECTION ( 'NONE',  ( 0.1261685609230673022, 0.9920088176193797569, 5.058037262945178882E-08 ) ) ;
#44507=CARTESIAN_POINT ( 'NONE',  ( -23.46741973463711872, -19.16603908095663655, 62.53902270128352825 ) ) ;
#44508=CARTESIAN_POINT ( 'NONE',  ( -16.52316554273587101, -21.80170452179945073, 65.24036514508233608 ) ) ;
#44510=CARTESIAN_POINT ( 'NONE',  ( -12.31054139703831041, -19.59141238940855700, 61.62508423592262119 ) ) ;
#44514=ORIENTED_EDGE ( 'NONE', *, *, #1090, .T. ) ;
#44515=EDGE_CURVE ( 'NONE', #3477, #48343, #7115, .T. ) ;
#44516=CARTESIAN_POINT ( 'NONE',  ( -10.18401502636761968, -13.05277926903019470, 71.32333192088977114 ) ) ;
#44518=DIRECTION ( 'NONE',  ( 0.9243256318339804212, -0.3816046728418208134, 8.614662760012533852E-09 ) ) ;
#44519=CARTESIAN_POINT ( 'NONE',  ( -23.00454255336054743, -10.50046069577333441, 59.88731295783226471 ) ) ;
#44520=ORIENTED_EDGE ( 'NONE', *, *, #35624, .F. ) ;
#44523=EDGE_LOOP ( 'NONE', ( #44432, #29436, #26433, #20458 ) ) ;
#44527=CARTESIAN_POINT ( 'NONE',  ( -15.55648817577099585, -8.010769314271311003, 74.09457776258329886 ) ) ;
#44528=EDGE_CURVE ( 'NONE', #45590, #13240, #9179, .T. ) ;
#44529=ORIENTED_EDGE ( 'NONE', *, *, #7835, .T. ) ;
#44531=CARTESIAN_POINT ( 'NONE',  ( -23.04367355717579713, -10.55211556811382678, 59.90203429191419104 ) ) ;
#44532=CARTESIAN_POINT ( 'NONE',  ( -21.53458130032788986, -9.143176798465843191, 66.77035947577643071 ) ) ;
#44533=VERTEX_POINT ( 'NONE', #15627 ) ;
#44534=DIRECTION ( 'NONE',  ( -3.964551025433374905E-06, -2.747358590626761473E-07, 0.9999999999921033167 ) ) ;
#44535=EDGE_CURVE ( 'NONE', #10306, #7586, #22363, .T. ) ;
#44536=( BOUNDED_CURVE ( )  B_SPLINE_CURVE ( 3, ( #26741, #37064, #22550, #3345 ),
 .UNSPECIFIED., .F., .F. ) 
 B_SPLINE_CURVE_WITH_KNOTS ( ( 4, 4 ),
 ( 0.4074455897393638448, 0.5000000000000000000 ),
 .UNSPECIFIED. ) 
 CURVE ( )  GEOMETRIC_REPRESENTATION_ITEM ( )  RATIONAL_B_SPLINE_CURVE ( ( 0.6983129098260937306, 0.7760317562607014219, 0.8765941196520041778, 1.000000000000003997 ) ) 
 REPRESENTATION_ITEM ( '' )  );
#44537=FACE_OUTER_BOUND ( 'NONE', #15940, .T. ) ;
#44539=CARTESIAN_POINT ( 'NONE',  ( -11.15769964539508941, -11.68856008149023218, 71.10477494218005745 ) ) ;
#44540=ORIENTED_EDGE ( 'NONE', *, *, #17044, .T. ) ;
#44542=VERTEX_POINT ( 'NONE', #27879 ) ;
#44544=CARTESIAN_POINT ( 'NONE',  ( -11.43475638805646710, -10.37850985603223286, 74.54546699258546028 ) ) ;
#44546=FACE_OUTER_BOUND ( 'NONE', #23352, .T. ) ;
#44547=CARTESIAN_POINT ( 'NONE',  ( -19.70639753248355319, -21.90109403227812379, 65.57990909513159750 ) ) ;
#44548=CARTESIAN_POINT ( 'NONE',  ( -13.43921408130402817, -8.993432070331126127, 60.73950277491898220 ) ) ;
#44549=ORIENTED_EDGE ( 'NONE', *, *, #28391, .F. ) ;
#44550=CARTESIAN_POINT ( 'NONE',  ( -19.89102460414330054, -21.83908858431354716, 69.09628976311167037 ) ) ;
#44551=( BOUNDED_CURVE ( )  B_SPLINE_CURVE ( 3, ( #45669, #23248, #19298, #4772 ),
 .UNSPECIFIED., .F., .F. ) 
 B_SPLINE_CURVE_WITH_KNOTS ( ( 4, 4 ),
 ( 0.9074455897393679527, 1.000000000000000000 ),
 .UNSPECIFIED. ) 
 CURVE ( )  GEOMETRIC_REPRESENTATION_ITEM ( )  RATIONAL_B_SPLINE_CURVE ( ( 0.6983129098260973944, 0.7760317562607019770, 0.8765941196520028456, 1.000000000000000000 ) ) 
 REPRESENTATION_ITEM ( '' )  );
#44553=CARTESIAN_POINT ( 'NONE',  ( -18.59487950719992000, -7.451777622494494047, 73.99064398808116039 ) ) ;
#44555=ORIENTED_EDGE ( 'NONE', *, *, #15590, .T. ) ;
#44556=VERTEX_POINT ( 'NONE', #5236 ) ;
#44557=CARTESIAN_POINT ( 'NONE',  ( -22.79960313759534074, -9.650943445293346912, 73.66656413195866548 ) ) ;
#44558=FACE_OUTER_BOUND ( 'NONE', #31597, .T. ) ;
#44559=CARTESIAN_POINT ( 'NONE',  ( -17.78823904182716120, -7.818684512505932993, 60.38060768393231825 ) ) ;
#44561=CARTESIAN_POINT ( 'NONE',  ( -10.78898398081525301, -17.19290454168847404, 61.44271037915215317 ) ) ;
#44562=EDGE_CURVE ( 'NONE', #25852, #36933, #47054, .T. ) ;
#44566=ORIENTED_EDGE ( 'NONE', *, *, #25240, .F. ) ;
#44567=CARTESIAN_POINT ( 'NONE',  ( -20.88289085685542545, -8.210692395643533814, 59.88479313977884289 ) ) ;
#44568=DIRECTION ( 'NONE',  ( 0.000000000000000000, 0.000000000000000000, 1.000000000000000000 ) ) ;
#44569=CARTESIAN_POINT ( 'NONE',  ( -24.47304815678895196, -15.04811744431364140, 59.65788834854969735 ) ) ;
#44570=CARTESIAN_POINT ( 'NONE',  ( -23.74619254753875808, -11.68933987248222550, 63.10218278636759237 ) ) ;
#44571=ORIENTED_EDGE ( 'NONE', *, *, #22040, .F. ) ;
#44572=ORIENTED_EDGE ( 'NONE', *, *, #46365, .F. ) ;
#44573=CARTESIAN_POINT ( 'NONE',  ( -17.72634082312590920, -21.85272461445201486, 58.40553378267873796 ) ) ;
#44576=CARTESIAN_POINT ( 'NONE',  ( -10.72552546848295485, -12.61109793159036485, 61.09853568372136579 ) ) ;
#44577=DIRECTION ( 'NONE',  ( -1.371991812172399310E-08, 1.272593380608347342E-06, -0.9999999999991900923 ) ) ;
#44580=CARTESIAN_POINT ( 'NONE',  ( -24.46903964301072421, -12.38562919627177727, 73.38079058079814843 ) ) ;
#44583=EDGE_CURVE ( 'NONE', #35456, #46448, #15375, .T. ) ;
#44584=CARTESIAN_POINT ( 'NONE',  ( -12.63291411399994146, -9.103221862242449447, 74.50578369661835154 ) ) ;
#44586=CARTESIAN_POINT ( 'NONE',  ( -22.38400238879419391, -20.36826089713532895, 62.41934470639706944 ) ) ;
#44590=CARTESIAN_POINT ( 'NONE',  ( -24.77697371742066679, -16.00871596996390167, 66.10678971410503380 ) ) ;
#44592=LINE ( 'NONE', #21929, #7895 ) ;
#44593=VERTEX_POINT ( 'NONE', #46840 ) ;
#44594=CARTESIAN_POINT ( 'NONE',  ( -23.81233663663554978, -10.97605585942814344, 73.46219060175555171 ) ) ;
#44595=CYLINDRICAL_SURFACE ( 'NONE', #42296, 0.1500000000000022704 ) ;
#44597=CARTESIAN_POINT ( 'NONE',  ( -21.36284794767689377, -21.13297080501056513, 69.16954792666395235 ) ) ;
#44598=CARTESIAN_POINT ( 'NONE',  ( -10.31379496977684340, -12.58270390103710668, 64.45491433821949556 ) ) ;
#44599=B_SPLINE_CURVE_WITH_KNOTS ( 'NONE', 1,
 ( #28381, #35264 ),
 .UNSPECIFIED., .F., .F.,
 ( 2, 2 ),
 ( 0.000000000000000000, 1.000000000000000000 ),
 .UNSPECIFIED. ) ;
#44601=CARTESIAN_POINT ( 'NONE',  ( -14.37840813110883254, -8.506458304712115392, 67.27477558708663707 ) ) ;
#44602=EDGE_CURVE ( 'NONE', #10578, #11221, #41758, .T. ) ;
#44603=CARTESIAN_POINT ( 'NONE',  ( -10.56879219357104915, -13.14797678187891528, 74.97817813415294097 ) ) ;
#44605=DIRECTION ( 'NONE',  ( 1.487365700889503844E-06, -6.376425446390537491E-07, -0.9999999999986906030 ) ) ;
#44606=B_SPLINE_CURVE_WITH_KNOTS ( 'NONE', 1,
 ( #17139, #32433 ),
 .UNSPECIFIED., .F., .F.,
 ( 2, 2 ),
 ( 0.000000000000000000, 1.000000000000000000 ),
 .UNSPECIFIED. ) ;
#44607=ORIENTED_EDGE ( 'NONE', *, *, #41030, .F. ) ;
#44609=ADVANCED_FACE ( 'NONE', ( #36455 ), #1772, .T. ) ;
#44610=DIRECTION ( 'NONE',  ( -0.9410372374137780938, -0.3383029970317210644, -1.029646047569396398E-09 ) ) ;
#44612=CARTESIAN_POINT ( 'NONE',  ( -24.83132749654373939, -14.01209333255521727, 73.27271506205273965 ) ) ;
#44613=CARTESIAN_POINT ( 'NONE',  ( -16.09495291808068274, -22.13976250616876840, 58.54231521589509413 ) ) ;
#44614=CARTESIAN_POINT ( 'NONE',  ( -22.79960237261627398, -9.650942640399760464, 73.66656521964461035 ) ) ;
#44616=ORIENTED_EDGE ( 'NONE', *, *, #41302, .T. ) ;
#44618=CARTESIAN_POINT ( 'NONE',  ( -9.974839262372155346, -14.70319952471188074, 71.52771478739579436 ) ) ;
#44619=ORIENTED_EDGE ( 'NONE', *, *, #38739, .T. ) ;
#44621=CARTESIAN_POINT ( 'NONE',  ( -11.77456497187086093, -18.94253032688613914, 71.98685932465902226 ) ) ;
#44622=CARTESIAN_POINT ( 'NONE',  ( -11.36794959886231915, -18.31963617796164812, 57.80714594517343841 ) ) ;
#44623=CARTESIAN_POINT ( 'NONE',  ( -11.59701759869595072, -18.68823990753973163, 65.04707024129098158 ) ) ;
#44624=CARTESIAN_POINT ( 'NONE',  ( -12.10487669921564446, -20.02548830339394925, 61.44032727821130635 ) ) ;
#44625=CARTESIAN_POINT ( 'NONE',  ( -11.20995753719673438, -18.14677381299707548, 58.10714798773844336 ) ) ;
#44626=CARTESIAN_POINT ( 'NONE',  ( -24.82596573341765733, -13.96226896445660515, 73.28304862000281616 ) ) ;
#44628=DIRECTION ( 'NONE',  ( 5.215802034766747424E-06, -6.671378398269898551E-06, -0.9999999999641441262 ) ) ;
#44629=AXIS2_PLACEMENT_3D ( 'NONE', #42895, #24183, #38708 ) ;
#44631=ORIENTED_EDGE ( 'NONE', *, *, #37906, .T. ) ;
#44632=CARTESIAN_POINT ( 'NONE',  ( -20.37299714182665866, -8.405577154986387356, 67.08104082189564110 ) ) ;
#44635=VECTOR ( 'NONE', #24737, 1000.000000000000114 ) ;
#44636=CARTESIAN_POINT ( 'NONE',  ( -11.06319317263454849, -11.76086512588999256, 67.82684465229463910 ) ) ;
#44637=DIRECTION ( 'NONE',  ( -1.504942875245327186E-06, 3.061075853171912725E-06, -0.9999999999941825424 ) ) ;
#44638=CARTESIAN_POINT ( 'NONE',  ( -14.60635853056651001, -21.70587488938233278, 58.20971981907628390 ) ) ;
#44641=ORIENTED_EDGE ( 'NONE', *, *, #33378, .F. ) ;
#44642=B_SPLINE_CURVE_WITH_KNOTS ( 'NONE', 3,
 ( #41178, #15056, #48312, #18267, #4918, #48560, #67, #971, #7218, #30114 ),
 .UNSPECIFIED., .F., .F.,
 ( 4, 2, 2, 2, 4 ),
 ( 0.000000000000000000, 0.2500000000000000000, 0.5000000000000000000, 0.7500000000000000000, 1.000000000000000000 ),
 .UNSPECIFIED. ) ;
#44644=ORIENTED_EDGE ( 'NONE', *, *, #47253, .F. ) ;
#44645=FACE_OUTER_BOUND ( 'NONE', #4810, .T. ) ;
#44647=EDGE_CURVE ( 'NONE', #3049, #48304, #21468, .T. ) ;
#44648=CARTESIAN_POINT ( 'NONE',  ( -18.34560609025200861, -9.386954687716537293, 54.07175714974878389 ) ) ;
#44649=CARTESIAN_POINT ( 'NONE',  ( -16.16221656818315466, -22.15164012088281709, 58.32939616168999208 ) ) ;
#44651=EDGE_CURVE ( 'NONE', #828, #40875, #30122, .T. ) ;
#44652=CARTESIAN_POINT ( 'NONE',  ( -24.37710591498809265, -15.61986392179586147, 73.00303784453015510 ) ) ;
#44654=CARTESIAN_POINT ( 'NONE',  ( -12.45873566688477929, -9.804017486950373339, 57.10407583662104258 ) ) ;
#44655=ORIENTED_EDGE ( 'NONE', *, *, #35548, .T. ) ;
#44656=CARTESIAN_POINT ( 'NONE',  ( -22.31965859069846658, -20.42511761535959636, 62.37405793546869148 ) ) ;
#44657=DIRECTION ( 'NONE',  ( -0.8356905716187447153, 0.5492005722024784209, 7.728900804118605128E-08 ) ) ;
#44661=CARTESIAN_POINT ( 'NONE',  ( -19.57699507595987143, -21.94144279212693860, 62.17998934563075153 ) ) ;
#44662=PLANE ( 'NONE',  #34619 ) ;
#44663=CARTESIAN_POINT ( 'NONE',  ( -13.06813783877040791, -9.265530354883376063, 67.66470656304637998 ) ) ;
#44664=VERTEX_POINT ( 'NONE', #47797 ) ;
#44668=ADVANCED_FACE ( 'NONE', ( #20978 ), #28233, .T. ) ;
#44669=CARTESIAN_POINT ( 'NONE',  ( -15.03805483313293756, -21.39046390026760847, 65.38980090007645174 ) ) ;
#44670=CARTESIAN_POINT ( 'NONE',  ( -10.57818832626110250, -17.74982580657420428, 68.21066696669559803 ) ) ;
#44671=ORIENTED_EDGE ( 'NONE', *, *, #36790, .F. ) ;
#44672=CARTESIAN_POINT ( 'NONE',  ( -24.66733291767277692, -16.55538881886969804, 59.30987817879385915 ) ) ;
#44675=CARTESIAN_POINT ( 'NONE',  ( -15.40901097238366546, -21.51335240779075875, 72.32958917352875972 ) ) ;
#44676=EDGE_CURVE ( 'NONE', #26011, #17474, #24118, .T. ) ;
#44677=CARTESIAN_POINT ( 'NONE',  ( -18.05298600948144028, -21.78095894789524678, 61.94824011654481666 ) ) ;
#44678=EDGE_CURVE ( 'NONE', #545, #40496, #6798, .T. ) ;
#44679=EDGE_CURVE ( 'NONE', #24975, #25942, #11846, .T. ) ;
#44680=CARTESIAN_POINT ( 'NONE',  ( -11.89466307818281798, -10.43082414681992276, 74.85374085024349711 ) ) ;
#44682=ORIENTED_EDGE ( 'NONE', *, *, #18299, .T. ) ;
#44683=CARTESIAN_POINT ( 'NONE',  ( -17.70776835051902864, -22.25388969026799657, 58.52057945155585372 ) ) ;
#44684=CARTESIAN_POINT ( 'NONE',  ( -14.66630222544868900, -8.320656262913127321, 63.80450889863892172 ) ) ;
#44686=FACE_OUTER_BOUND ( 'NONE', #31177, .T. ) ;
#44687=CARTESIAN_POINT ( 'NONE',  ( -22.59024966566153125, -10.08387632041895188, 73.55331295946989201 ) ) ;
#44688=CARTESIAN_POINT ( 'NONE',  ( -17.19811928533322387, -9.313850733363548073, 53.49899999999994549 ) ) ;
#44689=( BOUNDED_SURFACE ( )  B_SPLINE_SURFACE ( 3, 1, ( 
 ( #301, #19000 ),
 ( #15773, #30345 ),
 ( #45842, #12098 ),
 ( #27110, #42139 ),
 ( #38424, #4713 ),
 ( #1017, #47037 ),
 ( #46573, #38679 ) ),
 .UNSPECIFIED., .T., .F., .F. ) 
 B_SPLINE_SURFACE_WITH_KNOTS ( ( 4, 3, 4 ),
 ( 2, 2 ),
 ( 0.000000000000000000, 0.5000000000000000000, 1.000000000000000000 ),
 ( 0.000000000000000000, 1.000000000000000000 ),
 .UNSPECIFIED. ) 
 GEOMETRIC_REPRESENTATION_ITEM ( )  RATIONAL_B_SPLINE_SURFACE ( (
 ( 1.000000000000000000, 1.000000000000000000),
 ( 0.3333333333333335369, 0.3333333333333330373),
 ( 0.3333333333333335369, 0.3333333333333330373),
 ( 1.000000000000000000, 1.000000000000000000),
 ( 0.3333333333333333703, 0.3333333333333333703),
 ( 0.3333333333333333703, 0.3333333333333333703),
 ( 1.000000000000000000, 1.000000000000000000) ) ) 
 REPRESENTATION_ITEM ( '' )  SURFACE ( )  );
#44690=ORIENTED_EDGE ( 'NONE', *, *, #31833, .T. ) ;
#44691=CARTESIAN_POINT ( 'NONE',  ( -10.05751352497363271, -15.92131473292516119, 64.70045725156860783 ) ) ;
#44692=CARTESIAN_POINT ( 'NONE',  ( -18.40644494809068377, -22.19428016187509911, 68.93701928270169788 ) ) ;
#44693=ORIENTED_EDGE ( 'NONE', *, *, #47895, .F. ) ;
#44694=VERTEX_POINT ( 'NONE', #17268 ) ;
#44697=CARTESIAN_POINT ( 'NONE',  ( -18.83586040784625126, -7.494106175837369044, 70.48572642001049360 ) ) ;
#44698=DIRECTION ( 'NONE',  ( -0.4439273849576848563, -0.8960627639203804229, 9.143653603063735118E-17 ) ) ;
#44699=CARTESIAN_POINT ( 'NONE',  ( -14.03247011961845203, -8.175865378139491213, 70.85144881067481037 ) ) ;
#44700=DIRECTION ( 'NONE',  ( 4.556087729312554466E-06, -5.696494005668992306E-06, 0.9999999999733959477 ) ) ;
#44701=( BOUNDED_CURVE ( )  B_SPLINE_CURVE ( 3, ( #25585, #11063, #48230, #19858 ),
 .UNSPECIFIED., .F., .F. ) 
 B_SPLINE_CURVE_WITH_KNOTS ( ( 4, 4 ),
 ( 0.9074455897393648440, 1.000000000000000000 ),
 .UNSPECIFIED. ) 
 CURVE ( )  GEOMETRIC_REPRESENTATION_ITEM ( )  RATIONAL_B_SPLINE_CURVE ( ( 0.6983129098261178225, 0.7760317562607195185, 0.8765941196520136147, 1.000000000000000000 ) ) 
 REPRESENTATION_ITEM ( '' )  );
#44703=ORIENTED_EDGE ( 'NONE', *, *, #11375, .F. ) ;
#44706=EDGE_CURVE ( 'NONE', #46361, #25757, #39989, .T. ) ;
#44708=CARTESIAN_POINT ( 'NONE',  ( -11.33665496402021411, -18.36534999539612301, 58.10714572920461052 ) ) ;
#44710=B_SPLINE_CURVE_WITH_KNOTS ( 'NONE', 3,
 ( #41502, #7792, #40767, #22063, #7051, #42908, #20503, #13085, #28120, #46612 ),
 .UNSPECIFIED., .F., .F.,
 ( 4, 2, 2, 2, 4 ),
 ( 0.000000000000000000, 0.2500000000000000000, 0.5000000000000000000, 0.7500000000000000000, 1.000000000000000000 ),
 .UNSPECIFIED. ) ;
#44712=ORIENTED_EDGE ( 'NONE', *, *, #38457, .T. ) ;
#44713=DIRECTION ( 'NONE',  ( 0.5088156898428700670, 0.8608754809899750171, 5.922709712265242817E-08 ) ) ;
#44715=CARTESIAN_POINT ( 'NONE',  ( -23.83043768205027035, -11.86620487761972420, 59.63235732590894855 ) ) ;
#44716=CARTESIAN_POINT ( 'NONE',  ( -23.58371748462962714, -11.48100147700675855, 70.12040655271316325 ) ) ;
#44717=ORIENTED_EDGE ( 'NONE', *, *, #23675, .T. ) ;
#44718=CARTESIAN_POINT ( 'NONE',  ( -23.05949083151958590, -18.96177719399141282, 62.35406924025621578 ) ) ;
#44722=CARTESIAN_POINT ( 'NONE',  ( -10.57818832626110250, -17.74982580657420428, 68.21066696669559803 ) ) ;
#44723=CARTESIAN_POINT ( 'NONE',  ( -11.38156967460460223, -11.17705904596687105, 60.68445599065120177 ) ) ;
#44725=CARTESIAN_POINT ( 'NONE',  ( -18.94833620235381133, -7.977059930319036596, 67.20071832652779165 ) ) ;
#44726=CARTESIAN_POINT ( 'NONE',  ( -22.77174232103692830, -19.99646445987193388, 72.80547028276266985 ) ) ;
#44728=CYLINDRICAL_SURFACE ( 'NONE', #23513, 0.1500000000000013267 ) ;
#44729=CARTESIAN_POINT ( 'NONE',  ( -21.34582186320181307, -20.66775149956831115, 72.82446429489806405 ) ) ;
#44730=EDGE_LOOP ( 'NONE', ( #34158, #42373 ) ) ;
#44731=CARTESIAN_POINT ( 'NONE',  ( -17.56322643164902431, -15.18422937902243142, 47.99999999999994316 ) ) ;
#44732=CARTESIAN_POINT ( 'NONE',  ( -17.14371526033637849, -7.364357988229939700, 70.66752758873944629 ) ) ;
#44734=AXIS2_PLACEMENT_3D ( 'NONE', #1291, #2270, #17276 ) ;
#44735=CARTESIAN_POINT ( 'NONE',  ( -12.64043014238784046, -19.91972699092798038, 65.09348316439465520 ) ) ;
#44736=ORIENTED_EDGE ( 'NONE', *, *, #25568, .T. ) ;
#44737=FACE_BOUND ( 'NONE', #15690, .T. ) ;
#44738=VERTEX_POINT ( 'NONE', #11841 ) ;
#44739=EDGE_CURVE ( 'NONE', #17093, #25305, #9701, .T. ) ;
#44741=CARTESIAN_POINT ( 'NONE',  ( -22.09027712961677636, -20.02729522806141915, 62.23439146821721124 ) ) ;
#44742=FACE_OUTER_BOUND ( 'NONE', #24453, .T. ) ;
#44745=VERTEX_POINT ( 'NONE', #44853 ) ;
#44746=CARTESIAN_POINT ( 'NONE',  ( -18.53202070066404161, -7.846807721809618386, 73.84064401782792686 ) ) ;
#44748=VERTEX_POINT ( 'NONE', #15754 ) ;
#44750=CARTESIAN_POINT ( 'NONE',  ( -14.91432061146141663, -8.212540298998538546, 63.93411529719415398 ) ) ;
#44751=ORIENTED_EDGE ( 'NONE', *, *, #18895, .F. ) ;
#44752=CARTESIAN_POINT ( 'NONE',  ( -21.65613231742964473, -20.94137680209911423, 72.63791026777079196 ) ) ;
#44753=EDGE_CURVE ( 'NONE', #11637, #3920, #33985, .T. ) ;
#44755=CARTESIAN_POINT ( 'NONE',  ( -10.98359684359402699, -17.55162065409421501, 68.11224428658677255 ) ) ;
#44759=CARTESIAN_POINT ( 'NONE',  ( -22.23802305151986403, -19.89335697136803205, 69.36344962027256145 ) ) ;
#44760=CARTESIAN_POINT ( 'NONE',  ( -13.05029276218966672, -20.34859559109395377, 71.96220867596423432 ) ) ;
#44761=FACE_OUTER_BOUND ( 'NONE', #5286, .T. ) ;
#44762=B_SPLINE_CURVE_WITH_KNOTS ( 'NONE', 3,
 ( #41840, #48727, #14966, #45060, #26319, #22632, #33943, #15216, #37628, #30277 ),
 .UNSPECIFIED., .F., .F.,
 ( 4, 2, 2, 2, 4 ),
 ( 0.1272669073658116712, 0.2522669073463083000, 0.3772669073268050122, 0.5022669073073016133, 0.6272669072877983254 ),
 .UNSPECIFIED. ) ;
#44763=DIRECTION ( 'NONE',  ( 3.811252424767960347E-06, 6.838859004561632622E-06, 0.9999999999693520714 ) ) ;
#44764=CARTESIAN_POINT ( 'NONE',  ( -14.23114467316514897, -8.578028860463618344, 74.31027642345760853 ) ) ;
#44765=CARTESIAN_POINT ( 'NONE',  ( -22.28538024775887294, -19.92612572838908491, 72.78833238834644703 ) ) ;
#44768=CARTESIAN_POINT ( 'NONE',  ( -12.08372859862091708, -10.28366800835667760, 64.13800404418488199 ) ) ;
#44769=EDGE_CURVE ( 'NONE', #5353, #33324, #38271, .T. ) ;
#44770=CARTESIAN_POINT ( 'NONE',  ( -23.12535539932854078, -10.01343808792704237, 66.65686846082743955 ) ) ;
#44773=CARTESIAN_POINT ( 'NONE',  ( -10.38360249164154325, -14.43747963625415309, 67.87272197508832505 ) ) ;
#44774=CARTESIAN_POINT ( 'NONE',  ( -14.99706828511980916, -21.85287925006270626, 65.29092110561946072 ) ) ;
#44775=ORIENTED_EDGE ( 'NONE', *, *, #48198, .F. ) ;
#44777=AXIS2_PLACEMENT_3D ( 'NONE', #22695, #26881, #769 ) ;
#44779=CARTESIAN_POINT ( 'NONE',  ( -24.35706328060247827, -15.77560928887050373, 69.53307488759497801 ) ) ;
#44780=CARTESIAN_POINT ( 'NONE',  ( -13.60238447927381777, -8.884931327198675177, 57.11967755504965538 ) ) ;
#44781=LINE ( 'NONE', #7595, #11867 ) ;
#44784=CARTESIAN_POINT ( 'NONE',  ( -15.87557675045462169, -7.931373007531637320, 67.29007279016111909 ) ) ;
#44785=DIRECTION ( 'NONE',  ( -1.070267892829395584E-05, -6.715522050485540099E-06, 0.9999999999201771850 ) ) ;
#44786=EDGE_LOOP ( 'NONE', ( #39987, #21174, #15436, #21694, #20399 ) ) ;
#44787=CARTESIAN_POINT ( 'NONE',  ( -15.18490717705548398, -21.44146708918249544, 65.12099149998387304 ) ) ;
#44788=CARTESIAN_POINT ( 'NONE',  ( -10.13086764262007655, -16.32976185473646424, 71.55412051275166618 ) ) ;
#44791=VERTEX_POINT ( 'NONE', #19222 ) ;
#44792=CARTESIAN_POINT ( 'NONE',  ( -10.31364510401727053, -17.03300888149450998, 57.80265138661536639 ) ) ;
#44793=CARTESIAN_POINT ( 'NONE',  ( -17.56717507065399531, -7.360494836047319467, 63.73552460944732445 ) ) ;
#44794=VERTEX_POINT ( 'NONE', #15501 ) ;
#44795=ADVANCED_FACE ( 'NONE', ( #26129 ), #29825, .T. ) ;
#44797=CARTESIAN_POINT ( 'NONE',  ( -10.44916082259175916, -15.83527127794237188, 64.80771589743309846 ) ) ;
#44798=VECTOR ( 'NONE', #38952, 1000.000000000000000 ) ;
#44799=ORIENTED_EDGE ( 'NONE', *, *, #1094, .T. ) ;
#44802=CARTESIAN_POINT ( 'NONE',  ( -23.89200535028185612, -11.11192396016905448, 70.07706043178237110 ) ) ;
#44804=B_SPLINE_CURVE_WITH_KNOTS ( 'NONE', 3,
 ( #16164, #15686, #12248, #27270, #1398, #8326, #4877, #19888, #20125, #34891 ),
 .UNSPECIFIED., .F., .F.,
 ( 4, 2, 2, 2, 4 ),
 ( 0.000000000000000000, 0.2500000000000000000, 0.5000000000000000000, 0.7500000000000000000, 1.000000000000000000 ),
 .UNSPECIFIED. ) ;
#44805=CARTESIAN_POINT ( 'NONE',  ( -23.08487763607990928, -19.01185175973044039, 62.36879011380454330 ) ) ;
#44806=VECTOR ( 'NONE', #36654, 1000.000000000000114 ) ;
#44808=CARTESIAN_POINT ( 'NONE',  ( -20.66848101912799862, -8.549761622307149977, 60.12653141481577990 ) ) ;
#44813=CARTESIAN_POINT ( 'NONE',  ( -23.38410589725464916, -10.33907962427212190, 59.71708035543083071 ) ) ;
#44814=CARTESIAN_POINT ( 'NONE',  ( -24.68310392741195258, -16.48564297948346891, 59.37978378043003147 ) ) ;
#44818=ADVANCED_FACE ( 'NONE', ( #760 ), #37175, .T. ) ;
#44819=CARTESIAN_POINT ( 'NONE',  ( -7.433578433745469560, -16.27641334846635246, 54.54971261817296835 ) ) ;
#44820=FACE_OUTER_BOUND ( 'NONE', #2346, .T. ) ;
#44821=CARTESIAN_POINT ( 'NONE',  ( -16.94458633259734270, -7.374567983260779336, 74.14513688882354359 ) ) ;
#44823=ORIENTED_EDGE ( 'NONE', *, *, #35977, .F. ) ;
#44827=CARTESIAN_POINT ( 'NONE',  ( -10.20197030601470090, -12.78660143320473175, 53.49999999999994316 ) ) ;
#44828=ORIENTED_EDGE ( 'NONE', *, *, #31564, .T. ) ;
#44829=VERTEX_POINT ( 'NONE', #48518 ) ;
#44834=CARTESIAN_POINT ( 'NONE',  ( -13.83108299072750391, -21.33561835983412891, 72.04112301026525245 ) ) ;
#44835=( BOUNDED_CURVE ( )  B_SPLINE_CURVE ( 3, ( #33594, #26728, #18337, #11222 ),
 .UNSPECIFIED., .F., .F. ) 
 B_SPLINE_CURVE_WITH_KNOTS ( ( 4, 4 ),
 ( 0.5000000000000000000, 0.9074455897393695070 ),
 .UNSPECIFIED. ) 
 CURVE ( )  GEOMETRIC_REPRESENTATION_ITEM ( )  RATIONAL_B_SPLINE_CURVE ( ( 0.9999999999999745759, 0.4567392136813185344, 0.3561768502900429789, 0.6983129098261203760 ) ) 
 REPRESENTATION_ITEM ( '' )  );
#44836=ORIENTED_EDGE ( 'NONE', *, *, #7063, .F. ) ;
#44838=CARTESIAN_POINT ( 'NONE',  ( -24.64621740481133116, -16.83181165628401033, 54.27966884056654351 ) ) ;
#44839=DIRECTION ( 'NONE',  ( 0.9562635972186041000, -0.2925062950340273638, 4.666065131241568958E-08 ) ) ;
#44841=CARTESIAN_POINT ( 'NONE',  ( -22.78678303852979070, -9.565966637465479039, 47.99999999999994316 ) ) ;
#44843=CARTESIAN_POINT ( 'NONE',  ( -14.60689764421331738, -8.346551857622413806, 63.78978840692985131 ) ) ;
#44844=CARTESIAN_POINT ( 'NONE',  ( -14.07539681412750987, -8.605278097683306981, 74.49954655214880006 ) ) ;
#44845=EDGE_CURVE ( 'NONE', #19358, #24660, #14753, .T. ) ;
#44848=( BOUNDED_CURVE ( )  B_SPLINE_CURVE ( 3, ( #4263, #3772, #23466, #34278 ),
 .UNSPECIFIED., .F., .F. ) 
 B_SPLINE_CURVE_WITH_KNOTS ( ( 4, 4 ),
 ( 0.000000000000000000, 0.4074455897393673975 ),
 .UNSPECIFIED. ) 
 CURVE ( )  GEOMETRIC_REPRESENTATION_ITEM ( )  RATIONAL_B_SPLINE_CURVE ( ( 1.000000000000000000, 0.4567392136813307468, 0.3561768502900298783, 0.6983129098260973944 ) ) 
 REPRESENTATION_ITEM ( '' )  );
#44849=ORIENTED_EDGE ( 'NONE', *, *, #13606, .T. ) ;
#44850=CARTESIAN_POINT ( 'NONE',  ( -19.57699507595987143, -21.94144279212693860, 62.17998934563075153 ) ) ;
#44851=DIRECTION ( 'NONE',  ( 0.9687793358424813261, -0.2479245821708705166, 1.273414158200120423E-16 ) ) ;
#44852=VERTEX_POINT ( 'NONE', #18719 ) ;
#44853=CARTESIAN_POINT ( 'NONE',  ( -11.25989433568915032, -11.38792842781904469, 64.44882039367774951 ) ) ;
#44856=CARTESIAN_POINT ( 'NONE',  ( -24.86969121598721344, -14.53217971827670496, 66.36947994509128534 ) ) ;
#44858=B_SPLINE_CURVE_WITH_KNOTS ( 'NONE', 3,
 ( #2923, #10807, #17466, #44550, #14704, #32950, #48470, #2689, #9852, #40365 ),
 .UNSPECIFIED., .F., .F.,
 ( 4, 2, 2, 2, 4 ),
 ( 0.1272669073658279915, 0.2522669073463119638, 0.3772669073267959083, 0.5022669073072799639, 0.6272669072877639085 ),
 .UNSPECIFIED. ) ;
#44859=CARTESIAN_POINT ( 'NONE',  ( -24.18470913683765389, -12.80901137141652768, 69.78715111652664405 ) ) ;
#44860=ORIENTED_EDGE ( 'NONE', *, *, #33297, .T. ) ;
#44862=CARTESIAN_POINT ( 'NONE',  ( -22.65122085952885556, -20.11767465994831738, 69.27443734771573247 ) ) ;
#44864=B_SPLINE_CURVE_WITH_KNOTS ( 'NONE', 1,
 ( #4267, #95 ),
 .UNSPECIFIED., .F., .F.,
 ( 2, 2 ),
 ( 0.000000000000000000, 1.000000000000000000 ),
 .UNSPECIFIED. ) ;
#44865=FACE_OUTER_BOUND ( 'NONE', #148, .T. ) ;
#44866=CARTESIAN_POINT ( 'NONE',  ( -23.76916757952739090, -18.71361706205413000, 72.88651372856567434 ) ) ;
#44868=VERTEX_POINT ( 'NONE', #30 ) ;
#44869=EDGE_CURVE ( 'NONE', #16178, #23498, #5377, .T. ) ;
#44870=VECTOR ( 'NONE', #37067, 1000.000000000000227 ) ;
#44873=VERTEX_POINT ( 'NONE', #16959 ) ;
#44874=CYLINDRICAL_SURFACE ( 'NONE', #24339, 0.1500000000000050460 ) ;
#44875=DIRECTION ( 'NONE',  ( 0.3668819201507681482, -0.9245033139891514207, 0.1033986416233890204 ) ) ;
#44876=DIRECTION ( 'NONE',  ( -5.731567514496413899E-31, -1.020425574103664789E-16, -1.000000000000000000 ) ) ;
#44877=CARTESIAN_POINT ( 'NONE',  ( -20.71604796063133591, -8.125966986502412226, 63.41097886120039817 ) ) ;
#44880=CYLINDRICAL_SURFACE ( 'NONE', #4685, 7.000000000000000888 ) ;
#44882=AXIS2_PLACEMENT_3D ( 'NONE', #24721, #43924, #33037 ) ;
#44883=CARTESIAN_POINT ( 'NONE',  ( -10.42413885153580644, -14.85581157485834503, 74.79778936448731486 ) ) ;
#44886=CARTESIAN_POINT ( 'NONE',  ( -16.65537394168718421, -21.76815631184664213, 68.92390547312155036 ) ) ;
#44887=EDGE_LOOP ( 'NONE', ( #22885, #33640, #27378, #13948, #17870 ) ) ;
#44888=LINE ( 'NONE', #33508, #39242 ) ;
#44889=CARTESIAN_POINT ( 'NONE',  ( -10.38752013045322009, -14.36951432065623813, 64.67331771650336236 ) ) ;
#44892=CARTESIAN_POINT ( 'NONE',  ( -17.92193066645248578, -21.84160715981037981, 62.02535923543162966 ) ) ;
#44894=ADVANCED_FACE ( 'NONE', ( #42365 ), #20331, .T. ) ;
#44895=CARTESIAN_POINT ( 'NONE',  ( -21.65914559189701194, -18.31838547852702703, 54.07175714974879099 ) ) ;
#44897=ORIENTED_EDGE ( 'NONE', *, *, #6264, .F. ) ;
#44903=AXIS2_PLACEMENT_3D ( 'NONE', #9762, #27736, #9039 ) ;
#44904=CARTESIAN_POINT ( 'NONE',  ( -15.37363155966973061, -7.646927905176254647, 74.27974431700636160 ) ) ;
#44908=FACE_OUTER_BOUND ( 'NONE', #3757, .T. ) ;
#44909=CARTESIAN_POINT ( 'NONE',  ( -17.56717507065399531, -7.360494836047319467, 63.73552460944732445 ) ) ;
#44911=CARTESIAN_POINT ( 'NONE',  ( -14.97035482569482312, -21.41873484682592377, 61.92128389535452015 ) ) ;
#44912=EDGE_CURVE ( 'NONE', #5348, #36746, #41117, .T. ) ;
#44914=DIRECTION ( 'NONE',  ( 0.2465957053274518418, 0.9635866743705491233, 0.1033986416233889788 ) ) ;
#44915=ORIENTED_EDGE ( 'NONE', *, *, #31712, .F. ) ;
#44916=CARTESIAN_POINT ( 'NONE',  ( -17.95491883169589542, -21.84291603085813804, 58.40553388833760096 ) ) ;
#44918=CARTESIAN_POINT ( 'NONE',  ( -13.71338950266841294, -20.80363499509022773, 64.98628881289567971 ) ) ;
#44919=VERTEX_POINT ( 'NONE', #1468 ) ;
#44920=DIRECTION ( 'NONE',  ( 0.04287186434519785205, 0.9990805789562555717, -2.806673972535357682E-09 ) ) ;
#44921=CARTESIAN_POINT ( 'NONE',  ( -24.73385245812551503, -16.24793116159999684, 62.74328673523763200 ) ) ;
#44923=B_SPLINE_CURVE_WITH_KNOTS ( 'NONE', 1,
 ( #14459, #32259 ),
 .UNSPECIFIED., .F., .F.,
 ( 2, 2 ),
 ( 0.000000000000000000, 1.000000000000000000 ),
 .UNSPECIFIED. ) ;
#44924=LINE ( 'NONE', #14103, #36067 ) ;
#44925=CARTESIAN_POINT ( 'NONE',  ( -10.52422472645684870, -17.61911478008853749, 68.21226617000660042 ) ) ;
#44927=CARTESIAN_POINT ( 'NONE',  ( -24.69816866750256779, -16.41902046076232935, 59.16686479676427979 ) ) ;
#44930=DIRECTION ( 'NONE',  ( -0.8507615431891571989, 0.5255518971808581519, 6.876821558984484920E-08 ) ) ;
#44933=ORIENTED_EDGE ( 'NONE', *, *, #13658, .T. ) ;
#44934=DIRECTION ( 'NONE',  ( -0.1464579420318390668, 0.9892168979631277281, 7.284849527811297202E-08 ) ) ;
#44936=EDGE_LOOP ( 'NONE', ( #592, #7687, #25358, #25314, #40851 ) ) ;
#44937=CARTESIAN_POINT ( 'NONE',  ( -17.42409385541300892, -14.80920654474439679, 47.99999999999994316 ) ) ;
#44938=( BOUNDED_CURVE ( )  B_SPLINE_CURVE ( 3, ( #42397, #8666, #38690, #4973 ),
 .UNSPECIFIED., .F., .T. ) 
 B_SPLINE_CURVE_WITH_KNOTS ( ( 4, 4 ),
 ( 0.4074455897393651216, 0.5000000000000000000 ),
 .UNSPECIFIED. ) 
 CURVE ( )  GEOMETRIC_REPRESENTATION_ITEM ( )  RATIONAL_B_SPLINE_CURVE ( ( 0.6983129098261068313, 0.7760317562606926511, 0.8765941196519854151, 0.9999999999999723554 ) ) 
 REPRESENTATION_ITEM ( '' )  );
#44939=CARTESIAN_POINT ( 'NONE',  ( -15.43373621257565276, -8.098073005819149017, 74.09488064067743096 ) ) ;
#44941=ORIENTED_EDGE ( 'NONE', *, *, #35110, .F. ) ;
#44942=CARTESIAN_POINT ( 'NONE',  ( -10.37569183047413723, -14.65229009179183883, 71.33342454697773860 ) ) ;
#44943=ADVANCED_FACE ( 'NONE', ( #19954 ), #34726, .T. ) ;
#44945=ORIENTED_EDGE ( 'NONE', *, *, #24280, .T. ) ;
#44946=ORIENTED_EDGE ( 'NONE', *, *, #22764, .T. ) ;
#44948=ADVANCED_FACE ( 'NONE', ( #1958 ), #12559, .T. ) ;
#44950=CARTESIAN_POINT ( 'NONE',  ( -18.84272689959381353, -7.495397202044052243, 70.54880819107169998 ) ) ;
#44952=CARTESIAN_POINT ( 'NONE',  ( -15.62222905942472018, -7.993050613273783966, 70.89517703929612935 ) ) ;
#44953=CARTESIAN_POINT ( 'NONE',  ( -13.60894707410760240, -8.877133421815647907, 60.85439169328856934 ) ) ;
#44955=ORIENTED_EDGE ( 'NONE', *, *, #40561, .T. ) ;
#44956=ORIENTED_EDGE ( 'NONE', *, *, #43986, .T. ) ;
#44958=CARTESIAN_POINT ( 'NONE',  ( -10.44647900978708321, -14.24909228104994696, 60.99109301640115177 ) ) ;
#44959=AXIS2_PLACEMENT_3D ( 'NONE', #39371, #42102, #42345 ) ;
#44962=EDGE_CURVE ( 'NONE', #4699, #4476, #31273, .T. ) ;
#44965=EDGE_CURVE ( 'NONE', #46955, #47542, #18431, .T. ) ;
#44966=EDGE_CURVE ( 'NONE', #10001, #656, #42872, .T. ) ;
#44969=CARTESIAN_POINT ( 'NONE',  ( -18.76338093351206382, -7.938521699473153781, 67.00957693643654522 ) ) ;
#44970=CARTESIAN_POINT ( 'NONE',  ( -24.38756562526642213, -15.91227465074932290, 66.34852784166324113 ) ) ;
#44971=ORIENTED_EDGE ( 'NONE', *, *, #10402, .T. ) ;
#44973=ORIENTED_EDGE ( 'NONE', *, *, #35384, .F. ) ;
#44974=AXIS2_PLACEMENT_3D ( 'NONE', #16651, #2608, #17609 ) ;
#44976=CARTESIAN_POINT ( 'NONE',  ( -18.26831436342312287, -21.75822329804466904, 69.11514735239036611 ) ) ;
#44977=CARTESIAN_POINT ( 'NONE',  ( -24.40169278593617008, -17.41991595014878769, 69.51365538212004935 ) ) ;
#44978=CARTESIAN_POINT ( 'NONE',  ( -13.43773910423563400, -20.62433115109003268, 58.33177939114180788 ) ) ;
#44979=AXIS2_PLACEMENT_3D ( 'NONE', #45072, #48241, #48011 ) ;
#44980=ORIENTED_EDGE ( 'NONE', *, *, #34215, .F. ) ;
#44982=( BOUNDED_CURVE ( )  B_SPLINE_CURVE ( 3, ( #19241, #15520, #34243, #34004 ),
 .UNSPECIFIED., .F., .F. ) 
 B_SPLINE_CURVE_WITH_KNOTS ( ( 4, 4 ),
 ( 0.9074455897393650661, 1.000000000000000000 ),
 .UNSPECIFIED. ) 
 CURVE ( )  GEOMETRIC_REPRESENTATION_ITEM ( )  RATIONAL_B_SPLINE_CURVE ( ( 0.6983129098260931755, 0.7760317562606983133, 0.8765941196520006251, 1.000000000000000000 ) ) 
 REPRESENTATION_ITEM ( '' )  );
#44984=FACE_OUTER_BOUND ( 'NONE', #16101, .T. ) ;
#44985=ORIENTED_EDGE ( 'NONE', *, *, #8873, .F. ) ;
#44987=CARTESIAN_POINT ( 'NONE',  ( -17.22281210278579167, -7.361840297529252730, 70.60540404266352255 ) ) ;
#44988=CARTESIAN_POINT ( 'NONE',  ( -10.74028706782022269, -11.51804935604180358, 71.25007375637602536 ) ) ;
#44989=FACE_BOUND ( 'NONE', #9895, .T. ) ;
#44990=ORIENTED_EDGE ( 'NONE', *, *, #28274, .T. ) ;
#44991=CARTESIAN_POINT ( 'NONE',  ( -10.56492523587830235, -13.18000265412059058, 71.35828586226037373 ) ) ;
#44992=CARTESIAN_POINT ( 'NONE',  ( -10.81230840161673967, -17.25685697075765646, 64.64211442681141762 ) ) ;
#44994=CARTESIAN_POINT ( 'NONE',  ( -24.41709716369935990, -14.49630903675724625, 62.82182603900851348 ) ) ;
#44996=ORIENTED_EDGE ( 'NONE', *, *, #43793, .F. ) ;
#44998=VECTOR ( 'NONE', #39852, 999.9999999999998863 ) ;
#44999=ORIENTED_EDGE ( 'NONE', *, *, #17162, .T. ) ;
#45000=CARTESIAN_POINT ( 'NONE',  ( -12.69197368675297355, -9.055053595461757254, 70.95587035088203720 ) ) ;
#45002=DIRECTION ( 'NONE',  ( 0.9811758422909349076, 0.1931164583992469319, 7.863147543881890502E-08 ) ) ;
#45004=CARTESIAN_POINT ( 'NONE',  ( -16.14077005943513399, -22.14785303186519627, 58.38561932509040986 ) ) ;
#45005=( BOUNDED_SURFACE ( )  B_SPLINE_SURFACE ( 3, 1, ( 
 ( #2372, #20617 ),
 ( #47441, #5605 ),
 ( #47674, #32180 ),
 ( #24067, #13439 ),
 ( #28487, #35375 ),
 ( #46716, #9778 ),
 ( #12958, #27986 ) ),
 .UNSPECIFIED., .T., .F., .F. ) 
 B_SPLINE_SURFACE_WITH_KNOTS ( ( 4, 3, 4 ),
 ( 2, 2 ),
 ( 0.000000000000000000, 0.5000000000000000000, 1.000000000000000000 ),
 ( 0.000000000000000000, 1.000000000000000000 ),
 .UNSPECIFIED. ) 
 GEOMETRIC_REPRESENTATION_ITEM ( )  RATIONAL_B_SPLINE_SURFACE ( (
 ( 1.000000000000000000, 1.000000000000000000),
 ( 0.3333333333333335369, 0.3333333333333330373),
 ( 0.3333333333333335369, 0.3333333333333330373),
 ( 1.000000000000000000, 1.000000000000000000),
 ( 0.3333333333333333703, 0.3333333333333333703),
 ( 0.3333333333333333703, 0.3333333333333333703),
 ( 1.000000000000000000, 1.000000000000000000) ) ) 
 REPRESENTATION_ITEM ( '' )  SURFACE ( )  );
#45006=CARTESIAN_POINT ( 'NONE',  ( -11.01240199294250033, -17.61815787592479055, 68.20608059829778824 ) ) ;
#45007=EDGE_CURVE ( 'NONE', #38000, #28514, #7021, .T. ) ;
#45008=ORIENTED_EDGE ( 'NONE', *, *, #7572, .T. ) ;
#45009=VERTEX_POINT ( 'NONE', #47512 ) ;
#45010=ORIENTED_EDGE ( 'NONE', *, *, #19691, .F. ) ;
#45012=CARTESIAN_POINT ( 'NONE',  ( -24.00901317767523935, -17.32824147414624960, 69.42811846502259243 ) ) ;
#45013=CARTESIAN_POINT ( 'NONE',  ( -19.35357574399719027, -22.00502143967494817, 58.62483747956095215 ) ) ;
#45014=CARTESIAN_POINT ( 'NONE',  ( -10.57910656192517784, -13.34370627372683416, 74.67817676091868861 ) ) ;
#45015=CARTESIAN_POINT ( 'NONE',  ( -10.37567211895962060, -17.22253062098360488, 61.28026218318612450 ) ) ;
#45018=EDGE_LOOP ( 'NONE', ( #33375, #38251, #39728, #7770, #32518 ) ) ;
#45019=CARTESIAN_POINT ( 'NONE',  ( -16.16063032598464133, -7.467038112641824377, 60.38523865926408263 ) ) ;
#45021=CARTESIAN_POINT ( 'NONE',  ( -10.38752013045322009, -14.36951432065623635, 64.67331771650336236 ) ) ;
#45022=CARTESIAN_POINT ( 'NONE',  ( -24.29232294273250758, -16.16103065725259214, 62.59328677063434299 ) ) ;
#45023=ORIENTED_EDGE ( 'NONE', *, *, #27266, .T. ) ;
#45025=EDGE_CURVE ( 'NONE', #30144, #748, #9972, .T. ) ;
#45028=EDGE_CURVE ( 'NONE', #15971, #33162, #23515, .T. ) ;
#45029=CARTESIAN_POINT ( 'NONE',  ( -17.56322643164902431, -15.18422937902243142, 54.49999999999994316 ) ) ;
#45030=CARTESIAN_POINT ( 'NONE',  ( -22.19874839824752044, -20.52805027805738902, 58.91442897818879487 ) ) ;
#45032=B_SPLINE_CURVE_WITH_KNOTS ( 'NONE', 3,
 ( #35260, #23475, #13086, #46613, #34787, #34533, #38962, #814, #39203, #19780 ),
 .UNSPECIFIED., .F., .F.,
 ( 4, 2, 2, 2, 4 ),
 ( 0.6272669072878143126, 0.7522669073073209312, 0.8772669073268274387, 1.002266907346333946, 1.127266907365840565 ),
 .UNSPECIFIED. ) ;
#45035=ADVANCED_FACE ( 'NONE', ( #47740 ), #32485, .T. ) ;
#45037=CARTESIAN_POINT ( 'NONE',  ( -21.79028809537168243, -9.273590339475653366, 63.47681654923867711 ) ) ;
#45038=CARTESIAN_POINT ( 'NONE',  ( -10.47425521701617157, -17.49314416303823450, 64.81234701634230078 ) ) ;
#45039=B_SPLINE_CURVE_WITH_KNOTS ( 'NONE', 3,
 ( #29770, #14231, #29283, #44316, #14701, #36886, #14460, #29519, #10804, #37126 ),
 .UNSPECIFIED., .F., .F.,
 ( 4, 2, 2, 2, 4 ),
 ( 0.6272669072877813390, 0.7522669073072901780, 0.8772669073267991280, 1.002266907346307967, 1.127266907365816806 ),
 .UNSPECIFIED. ) ;
#45041=CARTESIAN_POINT ( 'NONE',  ( -18.68183629324915174, -7.872155521403883860, 70.66508205815506471 ) ) ;
#45042=DIRECTION ( 'NONE',  ( -5.408674110437222193E-06, 4.460197095916123975E-06, 0.9999999999754265456 ) ) ;
#45043=CARTESIAN_POINT ( 'NONE',  ( -23.98503169607928953, -17.39005800936845603, 66.22885190747201989 ) ) ;
#45044=ORIENTED_EDGE ( 'NONE', *, *, #40294, .F. ) ;
#45045=CARTESIAN_POINT ( 'NONE',  ( -16.03473429733671196, -7.489776097686932310, 63.79294168612747740 ) ) ;
#45047=PLANE ( 'NONE',  #39937 ) ;
#45048=CARTESIAN_POINT ( 'NONE',  ( -12.41315146567208139, -9.850077947585075933, 57.08935532239182464 ) ) ;
#45052=ADVANCED_FACE ( 'NONE', ( #6385 ), #6144, .T. ) ;
#45053=DIRECTION ( 'NONE',  ( -5.731567514496413899E-31, -1.020425574103664789E-16, -1.000000000000000000 ) ) ;
#45055=CARTESIAN_POINT ( 'NONE',  ( -22.09234508783963236, -20.09219152016766685, 62.38439162497947166 ) ) ;
#45056=CARTESIAN_POINT ( 'NONE',  ( -10.61330258792943226, -12.98832159324075874, 68.03832347271723791 ) ) ;
#45059=CARTESIAN_POINT ( 'NONE',  ( -12.64905295888074299, -9.611711778639854487, 57.23368232919959553 ) ) ;
#45060=CARTESIAN_POINT ( 'NONE',  ( -21.80063255203189243, -8.780035963955921119, 70.29279082220594432 ) ) ;
#45061=CARTESIAN_POINT ( 'NONE',  ( -24.38497043871102576, -15.94922339405466971, 62.80148391248476258 ) ) ;
#45062=ORIENTED_EDGE ( 'NONE', *, *, #22335, .F. ) ;
#45063=ORIENTED_EDGE ( 'NONE', *, *, #38998, .T. ) ;
#45064=DIRECTION ( 'NONE',  ( 1.277734862359329272E-05, 2.482875502418557358E-06, 0.9999999999152874297 ) ) ;
#45069=CARTESIAN_POINT ( 'NONE',  ( -24.82002243867330549, -13.90704071453223456, 73.23616177064057808 ) ) ;
#45070=CARTESIAN_POINT ( 'NONE',  ( -11.82099675438171005, -9.899106633794131582, 64.21409753874590365 ) ) ;
#45071=CARTESIAN_POINT ( 'NONE',  ( -17.36459502086233186, -7.755746116514760757, 63.55057029956871872 ) ) ;
#45072=CARTESIAN_POINT ( 'NONE',  ( -15.28291115335697192, -21.52618774670101232, 68.72592918174676413 ) ) ;
#45074=FACE_OUTER_BOUND ( 'NONE', #4978, .T. ) ;
#45076=AXIS2_PLACEMENT_3D ( 'NONE', #8200, #42168, #41681 ) ;
#45077=CARTESIAN_POINT ( 'NONE',  ( -12.10599200002982556, -20.02663609087960239, 61.58174067880212021 ) ) ;
#45079=ORIENTED_EDGE ( 'NONE', *, *, #43863, .F. ) ;
#45080=ORIENTED_EDGE ( 'NONE', *, *, #21330, .F. ) ;
#45081=EDGE_CURVE ( 'NONE', #34284, #18372, #31685, .T. ) ;
#45083=CYLINDRICAL_SURFACE ( 'NONE', #14213, 0.1499999999999979128 ) ;
#45085=CARTESIAN_POINT ( 'NONE',  ( -23.59267638082966201, -11.50008196526012760, 66.42214495376651939 ) ) ;
#45088=ORIENTED_EDGE ( 'NONE', *, *, #46911, .T. ) ;
#45090=CARTESIAN_POINT ( 'NONE',  ( -24.49635653881819408, -12.46679777644911447, 73.35730153580948354 ) ) ;
#45091=ADVANCED_FACE ( 'NONE', ( #26309 ), #48643, .T. ) ;
#45092=CARTESIAN_POINT ( 'NONE',  ( -10.86812116641377557, -17.26293110649939777, 64.62739382021851497 ) ) ;
#45093=ORIENTED_EDGE ( 'NONE', *, *, #12273, .T. ) ;
#45094=CARTESIAN_POINT ( 'NONE',  ( -21.68606078249201730, -9.256083098098587314, 66.96150029160082795 ) ) ;
#45096=CARTESIAN_POINT ( 'NONE',  ( -11.93762650184002538, -19.84916447049328170, 58.07682373525275921 ) ) ;
#45098=ORIENTED_EDGE ( 'NONE', *, *, #20553, .F. ) ;
#45099=PLANE ( 'NONE',  #18346 ) ;
#45100=DIRECTION ( 'NONE',  ( -0.6205284308219133349, -0.7841839494287637935, 8.002013567987292236E-17 ) ) ;
#45104=CARTESIAN_POINT ( 'NONE',  ( -21.36284794767689377, -21.13297080501056513, 69.16954792666395235 ) ) ;
#45106=CARTESIAN_POINT ( 'NONE',  ( -24.43617438265181008, -15.54086213135836303, 73.29743941331763324 ) ) ;
#45107=CARTESIAN_POINT ( 'NONE',  ( -13.42200550436094453, -8.525284928264134976, 57.09250892727150273 ) ) ;
#45109=CARTESIAN_POINT ( 'NONE',  ( -19.09646890170684230, -21.60781482332639314, 58.59677732982556364 ) ) ;
#45110=CARTESIAN_POINT ( 'NONE',  ( -15.47038452772150663, -21.58309165278561537, 72.04575460769355288 ) ) ;
#45111=CARTESIAN_POINT ( 'NONE',  ( -18.24819606216845358, -21.76058716088148515, 65.41820204848704634 ) ) ;
#45112=CARTESIAN_POINT ( 'NONE',  ( -17.42409385541300892, -14.80920654474439324, 56.49999999999994316 ) ) ;
#45115=EDGE_LOOP ( 'NONE', ( #41953, #33535, #11310, #41426, #5592 ) ) ;
#45117=CARTESIAN_POINT ( 'NONE',  ( -23.99312320239454976, -11.29471777418100231, 66.60709819448160829 ) ) ;
#45119=ORIENTED_EDGE ( 'NONE', *, *, #31017, .F. ) ;
#45120=CARTESIAN_POINT ( 'NONE',  ( -24.02536246799019892, -17.13931026604683083, 72.89952639825732206 ) ) ;
#45123=CARTESIAN_POINT ( 'NONE',  ( -17.24064286951094616, -7.811500644630894108, 70.79035835121598552 ) ) ;
#45124=( BOUNDED_SURFACE ( )  B_SPLINE_SURFACE ( 3, 1, ( 
 ( #43537, #18127 ),
 ( #35871, #33142 ),
 ( #17647, #32443 ),
 ( #40315, #32675 ),
 ( #9801, #47697 ),
 ( #24814, #6585 ),
 ( #13702, #2871 ) ),
 .UNSPECIFIED., .T., .F., .F. ) 
 B_SPLINE_SURFACE_WITH_KNOTS ( ( 4, 3, 4 ),
 ( 2, 2 ),
 ( 0.000000000000000000, 0.5000000000000000000, 1.000000000000000000 ),
 ( 0.000000000000000000, 1.000000000000000000 ),
 .UNSPECIFIED. ) 
 GEOMETRIC_REPRESENTATION_ITEM ( )  RATIONAL_B_SPLINE_SURFACE ( (
 ( 1.000000000000000000, 1.000000000000000000),
 ( 0.3333333333333335369, 0.3333333333333330373),
 ( 0.3333333333333335369, 0.3333333333333330373),
 ( 1.000000000000000000, 1.000000000000000000),
 ( 0.3333333333333333703, 0.3333333333333333703),
 ( 0.3333333333333333703, 0.3333333333333333703),
 ( 1.000000000000000000, 1.000000000000000000) ) ) 
 REPRESENTATION_ITEM ( '' )  SURFACE ( )  );
#45125=CARTESIAN_POINT ( 'NONE',  ( -17.92193035392797285, -21.84160718002658541, 61.87535923543196503 ) ) ;
#45126=CARTESIAN_POINT ( 'NONE',  ( -23.59048307761029761, -18.99011851117282390, 66.00106286486899876 ) ) ;
#45127=CARTESIAN_POINT ( 'NONE',  ( -15.55171133418867235, -7.598245370416885969, 70.79485226425863686 ) ) ;
#45128=CARTESIAN_POINT ( 'NONE',  ( -16.78865592400587659, -21.78030535593112305, 68.99560651886281448 ) ) ;
#45130=CARTESIAN_POINT ( 'NONE',  ( -17.56717507065399531, -7.360494836047319467, 63.73552460944732445 ) ) ;
#45131=FACE_OUTER_BOUND ( 'NONE', #37813, .T. ) ;
#45132=CARTESIAN_POINT ( 'NONE',  ( -15.65211633649168554, -8.035537180803068225, 74.26912783389062156 ) ) ;
#45133=CARTESIAN_POINT ( 'NONE',  ( -24.28250172495594228, -13.40621956664827152, 59.64651430442704338 ) ) ;
#45134=CARTESIAN_POINT ( 'NONE',  ( -22.96375064570672819, -10.44813988596692589, 63.08658113699938497 ) ) ;
#45135=ADVANCED_FACE ( 'NONE', ( #30265 ), #45530, .T. ) ;
#45137=( BOUNDED_CURVE ( )  B_SPLINE_CURVE ( 3, ( #23653, #34216, #19212, #23161 ),
 .UNSPECIFIED., .F., .F. ) 
 B_SPLINE_CURVE_WITH_KNOTS ( ( 4, 4 ),
 ( 0.9074455897393668424, 1.000000000000000000 ),
 .UNSPECIFIED. ) 
 CURVE ( )  GEOMETRIC_REPRESENTATION_ITEM ( )  RATIONAL_B_SPLINE_CURVE ( ( 0.6983129098261089407, 0.7760317562607119690, 0.8765941196520089518, 1.000000000000000000 ) ) 
 REPRESENTATION_ITEM ( '' )  );
#45138=CARTESIAN_POINT ( 'NONE',  ( -10.68602809008750576, -16.88409676349039046, 57.70232650191087487 ) ) ;
#45139=( BOUNDED_CURVE ( )  B_SPLINE_CURVE ( 3, ( #36381, #13725, #36616, #40566 ),
 .UNSPECIFIED., .F., .F. ) 
 B_SPLINE_CURVE_WITH_KNOTS ( ( 4, 4 ),
 ( 0.9074455897393658432, 1.000000000000000000 ),
 .UNSPECIFIED. ) 
 CURVE ( )  GEOMETRIC_REPRESENTATION_ITEM ( )  RATIONAL_B_SPLINE_CURVE ( ( 0.6983129098260822953, 0.7760317562606889874, 0.8765941196519948519, 1.000000000000000000 ) ) 
 REPRESENTATION_ITEM ( '' )  );
#45145=CARTESIAN_POINT ( 'NONE',  ( -16.30697390535036106, -7.848126388226943639, 60.20588296999211764 ) ) ;
#45146=DIRECTION ( 'NONE',  ( 1.522745436688331916E-06, -7.096186242782870827E-06, 0.9999999999736625123 ) ) ;
#45147=( BOUNDED_CURVE ( )  B_SPLINE_CURVE ( 3, ( #20564, #36033, #9480, #17069 ),
 .UNSPECIFIED., .F., .F. ) 
 B_SPLINE_CURVE_WITH_KNOTS ( ( 4, 4 ),
 ( 4.712388980384690562, 4.921828490624010399 ),
 .UNSPECIFIED. ) 
 CURVE ( )  GEOMETRIC_REPRESENTATION_ITEM ( )  RATIONAL_B_SPLINE_CURVE ( ( 1.000000000000000000, 0.9963479302455154896, 0.9963479302455154896, 1.000000000000000000 ) ) 
 REPRESENTATION_ITEM ( '' )  );
#45148=CARTESIAN_POINT ( 'NONE',  ( -10.39147815561416621, -17.41829018061022438, 53.49999999999995026 ) ) ;
#45149=CARTESIAN_POINT ( 'NONE',  ( -17.85555652284939043, -7.772123375420258107, 60.09532845646905486 ) ) ;
#45150=ORIENTED_EDGE ( 'NONE', *, *, #26873, .T. ) ;
#45151=EDGE_CURVE ( 'NONE', #6217, #29130, #25361, .T. ) ;
#45152=CARTESIAN_POINT ( 'NONE',  ( -24.37280380791617418, -15.65865402563598430, 73.01920416708826167 ) ) ;
#45153=CARTESIAN_POINT ( 'NONE',  ( -18.57721099958938282, -7.853998799284704013, 73.84624222578358399 ) ) ;
#45154=EDGE_CURVE ( 'NONE', #39323, #42977, #3515, .T. ) ;
#45159=EDGE_CURVE ( 'NONE', #1846, #6762, #14957, .T. ) ;
#45161=CARTESIAN_POINT ( 'NONE',  ( -14.98927377128279126, -8.246306944878790901, 56.84999999999994458 ) ) ;
#45162=CARTESIAN_POINT ( 'NONE',  ( -23.37999588001404661, -18.58199455739222827, 69.57899840282863124 ) ) ;
#45163=EDGE_LOOP ( 'NONE', ( #39429, #37504, #29369, #25862, #16028 ) ) ;
#45164=CARTESIAN_POINT ( 'NONE',  ( -23.20805662353657439, -10.11344718840461887, 63.24902867775850268 ) ) ;
#45165=FACE_OUTER_BOUND ( 'NONE', #1016, .T. ) ;
#45167=CARTESIAN_POINT ( 'NONE',  ( -10.74628672884880132, -17.07053172313825939, 61.17215199736627795 ) ) ;
#45168=CARTESIAN_POINT ( 'NONE',  ( -21.68495691188242702, -20.43592993620880804, 58.90875877921045145 ) ) ;
#45169=EDGE_LOOP ( 'NONE', ( #44253, #11702, #17753, #19857, #6640 ) ) ;
#45170=CARTESIAN_POINT ( 'NONE',  ( -10.91133513969588087, -12.10202850713728218, 74.44351760842475585 ) ) ;
#45172=FACE_OUTER_BOUND ( 'NONE', #42884, .T. ) ;
#45179=CARTESIAN_POINT ( 'NONE',  ( -17.42409385541300892, -14.80920654474439679, 47.99999999999994316 ) ) ;
#45180=CARTESIAN_POINT ( 'NONE',  ( -14.41574869888453136, -7.993524183322376686, 63.83332938139840707 ) ) ;
#45182=CARTESIAN_POINT ( 'NONE',  ( -24.41553149706675896, -15.71832598455623398, 69.81835354388927328 ) ) ;
#45183=CARTESIAN_POINT ( 'NONE',  ( -22.59024963249656182, -10.08387628509608192, 73.70990895709888946 ) ) ;
#45185=FACE_OUTER_BOUND ( 'NONE', #34096, .T. ) ;
#45187=CARTESIAN_POINT ( 'NONE',  ( -10.42334078895570926, -15.64104556165006521, 61.18789045260545834 ) ) ;
#45188=EDGE_LOOP ( 'NONE', ( #22587, #16920, #47315, #22996, #4600 ) ) ;
#45190=CARTESIAN_POINT ( 'NONE',  ( -11.46310342473229049, -11.03940158154180651, 61.09374645412970750 ) ) ;
#45192=EDGE_CURVE ( 'NONE', #3562, #30487, #16573, .T. ) ;
#45193=CARTESIAN_POINT ( 'NONE',  ( -14.03870967672415304, -8.172720116890397790, 70.91453050697840865 ) ) ;
#45194=CARTESIAN_POINT ( 'NONE',  ( -23.19916440516392697, -19.59445054535707698, 53.49999999999994316 ) ) ;
#45195=ORIENTED_EDGE ( 'NONE', *, *, #20267, .T. ) ;
#45196=ORIENTED_EDGE ( 'NONE', *, *, #8380, .F. ) ;
#45201=CARTESIAN_POINT ( 'NONE',  ( -10.81484442788029376, -17.11524687497682251, 61.45743118925498294 ) ) ;
#45202=CARTESIAN_POINT ( 'NONE',  ( -10.52668521080748398, -13.31230368787681506, 67.89399308012602319 ) ) ;
#45205=CARTESIAN_POINT ( 'NONE',  ( -13.85534475943383370, -8.269504983759647487, 74.24308752109034515 ) ) ;
#45206=CARTESIAN_POINT ( 'NONE',  ( -24.77697371742066679, -16.00871596996390167, 66.10678971410503380 ) ) ;
#45208=PLANE ( 'NONE',  #36716 ) ;
#45209=ORIENTED_EDGE ( 'NONE', *, *, #42837, .F. ) ;
#45210=ADVANCED_FACE ( 'NONE', ( #41087 ), #22373, .T. ) ;
#45211=CARTESIAN_POINT ( 'NONE',  ( -12.59088559871646673, -9.139540839424896035, 74.45889665379543487 ) ) ;
#45214=CARTESIAN_POINT ( 'NONE',  ( -18.10866925340710409, -22.22785503003063212, 65.50678672671764957 ) ) ;
#45215=ORIENTED_EDGE ( 'NONE', *, *, #19245, .F. ) ;
#45217=CARTESIAN_POINT ( 'NONE',  ( -17.71668947275567874, -21.85613660542494685, 62.29024590482070778 ) ) ;
#45218=CARTESIAN_POINT ( 'NONE',  ( -15.31785298361350378, -21.95540353714732618, 72.16858574460090381 ) ) ;
#45219=( BOUNDED_SURFACE ( )  B_SPLINE_SURFACE ( 3, 1, ( 
 ( #26940, #20033 ),
 ( #19059, #357 ),
 ( #15341, #30400 ),
 ( #8002, #23019 ),
 ( #39475, #20759 ),
 ( #43667, #17536 ),
 ( #5509, #39712 ) ),
 .UNSPECIFIED., .T., .F., .F. ) 
 B_SPLINE_SURFACE_WITH_KNOTS ( ( 4, 3, 4 ),
 ( 2, 2 ),
 ( 0.000000000000000000, 0.5000000000000000000, 1.000000000000000000 ),
 ( 0.000000000000000000, 1.000000000000000000 ),
 .UNSPECIFIED. ) 
 GEOMETRIC_REPRESENTATION_ITEM ( )  RATIONAL_B_SPLINE_SURFACE ( (
 ( 1.000000000000000000, 1.000000000000000000),
 ( 0.3333333333333335369, 0.3333333333333330373),
 ( 0.3333333333333335369, 0.3333333333333330373),
 ( 1.000000000000000000, 1.000000000000000000),
 ( 0.3333333333333333703, 0.3333333333333333703),
 ( 0.3333333333333333703, 0.3333333333333333703),
 ( 1.000000000000000000, 1.000000000000000000) ) ) 
 REPRESENTATION_ITEM ( '' )  SURFACE ( )  );
#45220=EDGE_CURVE ( 'NONE', #9377, #20130, #1169, .T. ) ;
#45221=CARTESIAN_POINT ( 'NONE',  ( -20.13458775212509266, -8.355142810065961712, 70.25100345207583530 ) ) ;
#45223=VERTEX_POINT ( 'NONE', #15696 ) ;
#45224=CARTESIAN_POINT ( 'NONE',  ( -10.52713468165226374, -17.62616329503903856, 68.20447774248857797 ) ) ;
#45226=CARTESIAN_POINT ( 'NONE',  ( -12.65141607933757051, -19.92990444307418230, 65.05778175411948894 ) ) ;
#45227=FACE_BOUND ( 'NONE', #25157, .T. ) ;
#45229=ORIENTED_EDGE ( 'NONE', *, *, #37330, .T. ) ;
#45231=FACE_OUTER_BOUND ( 'NONE', #29489, .T. ) ;
#45233=CARTESIAN_POINT ( 'NONE',  ( -24.47432067347917695, -14.77756146504815327, 59.52828185648635184 ) ) ;
#45236=ORIENTED_EDGE ( 'NONE', *, *, #10810, .T. ) ;
#45238=CARTESIAN_POINT ( 'NONE',  ( -23.52949419687348964, -11.28347464189849525, 70.17738639980606763 ) ) ;
#45239=CARTESIAN_POINT ( 'NONE',  ( -14.92957361138602579, -21.82925975653312278, 65.22101252026929785 ) ) ;
#45241=ORIENTED_EDGE ( 'NONE', *, *, #5460, .F. ) ;
#45242=ADVANCED_FACE ( 'NONE', ( #35387 ), #12258, .T. ) ;
#45244=CARTESIAN_POINT ( 'NONE',  ( -23.08280660609100110, -10.60377317445056811, 59.61675562601556067 ) ) ;
#45245=ORIENTED_EDGE ( 'NONE', *, *, #17267, .T. ) ;
#45248=VERTEX_POINT ( 'NONE', #4887 ) ;
#45249=CARTESIAN_POINT ( 'NONE',  ( -20.38226146016681994, -7.971588334861294811, 70.36604906519886526 ) ) ;
#45250=CARTESIAN_POINT ( 'NONE',  ( -20.55988796755815073, -8.491641294495202885, 67.19592733635545301 ) ) ;
#45251=CARTESIAN_POINT ( 'NONE',  ( -19.36787201549275750, -22.00121347418323481, 58.63169058443503445 ) ) ;
#45252=CARTESIAN_POINT ( 'NONE',  ( -20.75918656682226171, -8.147304802054664563, 63.42626204841099735 ) ) ;
#45256=ORIENTED_EDGE ( 'NONE', *, *, #34052, .T. ) ;
#45258=CARTESIAN_POINT ( 'NONE',  ( -16.19792114999740562, -7.866354181730329742, 60.48556343814865954 ) ) ;
#45259=CARTESIAN_POINT ( 'NONE',  ( -13.89449342130350473, -8.248373700058229119, 74.39965851202151725 ) ) ;
#45262=ORIENTED_EDGE ( 'NONE', *, *, #24334, .T. ) ;
#45265=DIRECTION ( 'NONE',  ( 1.053901171194056067E-05, -6.708308827411335869E-06, 0.9999999999219638669 ) ) ;
#45266=FACE_OUTER_BOUND ( 'NONE', #27526, .T. ) ;
#45269=CARTESIAN_POINT ( 'NONE',  ( -20.37436612178944273, -7.968217454415653656, 70.44438632422075841 ) ) ;
#45271=EDGE_CURVE ( 'NONE', #20133, #6106, #18159, .T. ) ;
#45272=CARTESIAN_POINT ( 'NONE',  ( -14.58503208334058421, -8.356083477664656201, 64.08978844553014653 ) ) ;
#45273=ADVANCED_FACE ( 'NONE', ( #8576 ), #24787, .T. ) ;
#45275=CARTESIAN_POINT ( 'NONE',  ( -24.40658449907488148, -15.78251210865724907, 69.53307488410803217 ) ) ;
#45276=CARTESIAN_POINT ( 'NONE',  ( -10.45859239952313224, -15.89938452881993847, 64.79299464097340433 ) ) ;
#45277=DIRECTION ( 'NONE',  ( -4.924618307954601745E-06, -4.007739941247756836E-06, -0.9999999999798431238 ) ) ;
#45279=CARTESIAN_POINT ( 'NONE',  ( -24.69683998333984576, -16.42489649515229289, 59.31606561861987359 ) ) ;
#45280=( BOUNDED_CURVE ( )  B_SPLINE_CURVE ( 3, ( #11840, #8155, #30807, #45335 ),
 .UNSPECIFIED., .F., .F. ) 
 B_SPLINE_CURVE_WITH_KNOTS ( ( 4, 4 ),
 ( 0.4074455897393619574, 0.5000000000000000000 ),
 .UNSPECIFIED. ) 
 CURVE ( )  GEOMETRIC_REPRESENTATION_ITEM ( )  RATIONAL_B_SPLINE_CURVE ( ( 0.6983129098260852929, 0.7760317562606940944, 0.8765941196519998480, 1.000000000000004219 ) ) 
 REPRESENTATION_ITEM ( '' )  );
#45282=CARTESIAN_POINT ( 'NONE',  ( -17.72634082312590920, -21.85272461445201486, 58.40553378267872375 ) ) ;
#45283=CARTESIAN_POINT ( 'NONE',  ( -24.74075702715665770, -16.21285080831185965, 62.77823949964436423 ) ) ;
#45286=CARTESIAN_POINT ( 'NONE',  ( -24.10556926794565413, -12.55028678686139898, 69.65754220287278997 ) ) ;
#45287=CARTESIAN_POINT ( 'NONE',  ( -12.57408663618378952, -9.687461344359430626, 57.38935503166064933 ) ) ;
#45288=ORIENTED_EDGE ( 'NONE', *, *, #20909, .F. ) ;
#45289=FACE_OUTER_BOUND ( 'NONE', #9815, .T. ) ;
#45290=CARTESIAN_POINT ( 'NONE',  ( -22.31195342450015318, -19.82007762202811918, 65.89524982080033055 ) ) ;
#45291=CARTESIAN_POINT ( 'NONE',  ( -11.50273595086851763, -11.07590776185467263, 57.20903212540526539 ) ) ;
#45292=ORIENTED_EDGE ( 'NONE', *, *, #13189, .F. ) ;
#45295=FACE_OUTER_BOUND ( 'NONE', #25001, .T. ) ;
#45298=EDGE_CURVE ( 'NONE', #24853, #14265, #47571, .T. ) ;
#45303=CARTESIAN_POINT ( 'NONE',  ( -23.42626641412206823, -19.22254892098468204, 62.61052823878424078 ) ) ;
#45306=CARTESIAN_POINT ( 'NONE',  ( -12.49878633484568446, -19.78335800357576346, 61.46966759759297361 ) ) ;
#45308=VECTOR ( 'NONE', #12777, 1000.000000000000114 ) ;
#45309=ORIENTED_EDGE ( 'NONE', *, *, #37390, .F. ) ;
#45311=CARTESIAN_POINT ( 'NONE',  ( -10.57043792878517685, -13.15679342524445516, 71.20828613024409037 ) ) ;
#45313=ORIENTED_EDGE ( 'NONE', *, *, #31556, .T. ) ;
#45314=VERTEX_POINT ( 'NONE', #39082 ) ;
#45316=CARTESIAN_POINT ( 'NONE',  ( -7.540694356433003342, -14.17955609235691661, 53.49999999999995026 ) ) ;
#45317=PLANE ( 'NONE',  #1694 ) ;
#45318=B_SPLINE_CURVE_WITH_KNOTS ( 'NONE', 3,
 ( #10203, #33536, #48335, #22245, #18285, #40241, #17799, #40706, #10447, #29628 ),
 .UNSPECIFIED., .F., .F.,
 ( 4, 2, 2, 2, 4 ),
 ( 0.6272669072877586904, 0.7522669073072832946, 0.8772669073268077877, 1.002266907346332392, 1.127266907365856996 ),
 .UNSPECIFIED. ) ;
#45320=ORIENTED_EDGE ( 'NONE', *, *, #46494, .F. ) ;
#45321=CARTESIAN_POINT ( 'NONE',  ( -12.52591726580351228, -9.195683270288645517, 74.50418291613799227 ) ) ;
#45323=CARTESIAN_POINT ( 'NONE',  ( -10.35515617550548306, -17.16373074020370737, 61.34398415755805445 ) ) ;
#45324=EDGE_CURVE ( 'NONE', #41313, #28733, #44606, .T. ) ;
#45325=CARTESIAN_POINT ( 'NONE',  ( -22.96375064570672819, -10.44813988596692589, 63.08658113699938497 ) ) ;
#45326=CARTESIAN_POINT ( 'NONE',  ( -12.41315146567207961, -9.850077947585075933, 57.08935532239181754 ) ) ;
#45327=VERTEX_POINT ( 'NONE', #24575 ) ;
#45328=FACE_OUTER_BOUND ( 'NONE', #42282, .T. ) ;
#45331=ORIENTED_EDGE ( 'NONE', *, *, #15673, .F. ) ;
#45332=CARTESIAN_POINT ( 'NONE',  ( -10.44632879773527456, -17.41978534048111982, 64.80552118489215729 ) ) ;
#45334=ORIENTED_EDGE ( 'NONE', *, *, #47526, .T. ) ;
#45335=CARTESIAN_POINT ( 'NONE',  ( -24.42398663107514523, -15.65075326911586906, 73.01775867260030850 ) ) ;
#45338=CARTESIAN_POINT ( 'NONE',  ( -11.30361347545239958, -11.41219030243732391, 64.14882039658046153 ) ) ;
#45339=DIRECTION ( 'NONE',  ( 3.827383494395459811E-06, -8.363078745702701817E-06, -0.9999999999577049437 ) ) ;
#45340=CARTESIAN_POINT ( 'NONE',  ( -12.54253442593986456, -19.82621537833410841, 64.86674886820043184 ) ) ;
#45341=CARTESIAN_POINT ( 'NONE',  ( -15.28291166272248169, -21.52618791248891128, 68.87592918174580348 ) ) ;
#45343=CARTESIAN_POINT ( 'NONE',  ( -10.43288321166496502, -14.45853026220434323, 64.57907052596242181 ) ) ;
#45346=CARTESIAN_POINT ( 'NONE',  ( -18.64201680114630832, -7.915911148255196039, 70.65602612026023621 ) ) ;
#45347=CARTESIAN_POINT ( 'NONE',  ( -22.83373948139051990, -9.686860930601344677, 73.58186838660923001 ) ) ;
#45348=EDGE_CURVE ( 'NONE', #24292, #39358, #41759, .T. ) ;
#45349=ADVANCED_FACE ( 'NONE', ( #43525 ), #9552, .T. ) ;
#45350=ORIENTED_EDGE ( 'NONE', *, *, #1036, .F. ) ;
#45351=ORIENTED_EDGE ( 'NONE', *, *, #48333, .T. ) ;
#45352=CARTESIAN_POINT ( 'NONE',  ( -24.47354778464749003, -12.39902454472287197, 73.42720984402279782 ) ) ;
#45353=CARTESIAN_POINT ( 'NONE',  ( -11.93195840498443516, -10.38844327383712773, 70.98365212470247343 ) ) ;
#45354=EDGE_LOOP ( 'NONE', ( #12976, #15988, #40697, #10480, #42417 ) ) ;
#45355=CARTESIAN_POINT ( 'NONE',  ( -17.85555652284939043, -7.772123375420258107, 60.09532845646905486 ) ) ;
#45356=DIRECTION ( 'NONE',  ( 0.1206048672277635625, -0.4306442452895124506, 0.8944271909999158554 ) ) ;
#45357=CARTESIAN_POINT ( 'NONE',  ( -12.04630953498396018, -19.96521513636629663, 61.55825118588921896 ) ) ;
#45360=EDGE_CURVE ( 'NONE', #1918, #11910, #5225, .T. ) ;
#45361=EDGE_CURVE ( 'NONE', #12034, #22754, #6326, .T. ) ;
#45364=EDGE_CURVE ( 'NONE', #20890, #33252, #33407, .T. ) ;
#45365=CARTESIAN_POINT ( 'NONE',  ( -16.07865488608826254, -7.939723797651444315, 63.67011030349581091 ) ) ;
#45366=CARTESIAN_POINT ( 'NONE',  ( -10.99655737938916289, -18.57624151290433900, 57.99209991576458378 ) ) ;
#45368=AXIS2_PLACEMENT_3D ( 'NONE', #5716, #20723, #38946 ) ;
#45369=EDGE_LOOP ( 'NONE', ( #28669, #42265, #27006, #9664 ) ) ;
#45372=EDGE_LOOP ( 'NONE', ( #17806, #20754, #3939, #45446, #1883 ) ) ;
#45373=ADVANCED_FACE ( 'NONE', ( #24803 ), #28254, .T. ) ;
#45374=DIRECTION ( 'NONE',  ( -0.3824554607245533866, 0.9239739285077094300, -8.917814418161383551E-09 ) ) ;
#45377=B_SPLINE_CURVE_WITH_KNOTS ( 'NONE', 3,
 ( #46792, #27828, #28327, #9371, #1736, #1232, #1478, #5683, #17212, #20693 ),
 .UNSPECIFIED., .F., .F.,
 ( 4, 2, 2, 2, 4 ),
 ( 0.000000000000000000, 0.2499999999999775180, 0.4999999999999850120, 0.7499999999999924505, 1.000000000000000000 ),
 .UNSPECIFIED. ) ;
#45378=B_SPLINE_CURVE_WITH_KNOTS ( 'NONE', 3,
 ( #45610, #8175, #45120, #26150, #37946, #4460, #50, #19734, #30097, #14776 ),
 .UNSPECIFIED., .F., .F.,
 ( 4, 2, 2, 2, 4 ),
 ( 0.000000000000000000, 0.2500000000000000000, 0.5000000000000000000, 0.7500000000000000000, 1.000000000000000000 ),
 .UNSPECIFIED. ) ;
#45379=LINE ( 'NONE', #321, #11161 ) ;
#45381=ORIENTED_EDGE ( 'NONE', *, *, #41378, .T. ) ;
#45382=CARTESIAN_POINT ( 'NONE',  ( -13.53189383941936264, -21.16172133628754892, 65.02982926591782586 ) ) ;
#45384=ORIENTED_EDGE ( 'NONE', *, *, #47454, .F. ) ;
#45387=VERTEX_POINT ( 'NONE', #43280 ) ;
#45389=DIRECTION ( 'NONE',  ( 0.3163880819683242418, 0.8528035521334692559, 0.4154812667942346938 ) ) ;
#45391=VERTEX_POINT ( 'NONE', #46956 ) ;
#45392=CARTESIAN_POINT ( 'NONE',  ( -19.74917349865086180, -21.41189893251537413, 68.93482485975984275 ) ) ;
#45394=( BOUNDED_CURVE ( )  B_SPLINE_CURVE ( 3, ( #713, #18424, #30764, #33433 ),
 .UNSPECIFIED., .F., .F. ) 
 B_SPLINE_CURVE_WITH_KNOTS ( ( 4, 4 ),
 ( 0.000000000000000000, 0.4074455897393649551 ),
 .UNSPECIFIED. ) 
 CURVE ( )  GEOMETRIC_REPRESENTATION_ITEM ( )  RATIONAL_B_SPLINE_CURVE ( ( 1.000000000000000000, 0.4567392136813263059, 0.3561768502900282130, 0.6983129098261057210 ) ) 
 REPRESENTATION_ITEM ( '' )  );
#45397=CARTESIAN_POINT ( 'NONE',  ( -13.65828898514496359, -20.76952646431350757, 65.00101022825411690 ) ) ;
#45398=ORIENTED_EDGE ( 'NONE', *, *, #29543, .F. ) ;
#45399=CARTESIAN_POINT ( 'NONE',  ( -10.61641629527463770, -11.78277212779517136, 74.74335553404092991 ) ) ;
#45401=CARTESIAN_POINT ( 'NONE',  ( -10.76011155904975780, -12.66606457907365169, 61.09853557581804750 ) ) ;
#45404=CARTESIAN_POINT ( 'NONE',  ( -10.42334091404133645, -15.64104667191196185, 61.33789045260130024 ) ) ;
#45405=CARTESIAN_POINT ( 'NONE',  ( -20.85319456454439546, -20.91190956734547157, 62.11471372081155096 ) ) ;
#45408=ADVANCED_FACE ( 'NONE', ( #40304 ), #21593, .T. ) ;
#45409=ORIENTED_EDGE ( 'NONE', *, *, #44966, .T. ) ;
#45412=VERTEX_POINT ( 'NONE', #35860 ) ;
#45413=CYLINDRICAL_SURFACE ( 'NONE', #22941, 7.500000000000001776 ) ;
#45415=CARTESIAN_POINT ( 'NONE',  ( -15.09544287645192462, -21.46351977604527761, 65.10596681500476279 ) ) ;
#45417=( BOUNDED_CURVE ( )  B_SPLINE_CURVE ( 3, ( #4261, #41687, #10672, #327 ),
 .UNSPECIFIED., .F., .F. ) 
 B_SPLINE_CURVE_WITH_KNOTS ( ( 4, 4 ),
 ( 0.4074455897393671200, 0.5000000000000000000 ),
 .UNSPECIFIED. ) 
 CURVE ( )  GEOMETRIC_REPRESENTATION_ITEM ( )  RATIONAL_B_SPLINE_CURVE ( ( 0.6983129098260968393, 0.7760317562607000896, 0.8765941196520007361, 0.9999999999999978906 ) ) 
 REPRESENTATION_ITEM ( '' )  );
#45419=( BOUNDED_CURVE ( )  B_SPLINE_CURVE ( 3, ( #30129, #86, #45640, #30861 ),
 .UNSPECIFIED., .F., .F. ) 
 B_SPLINE_CURVE_WITH_KNOTS ( ( 4, 4 ),
 ( 0.000000000000000000, 0.4074455897393655657 ),
 .UNSPECIFIED. ) 
 CURVE ( )  GEOMETRIC_REPRESENTATION_ITEM ( )  RATIONAL_B_SPLINE_CURVE ( ( 1.000000000000000000, 0.4567392136813270276, 0.3561768502900284905, 0.6983129098261043888 ) ) 
 REPRESENTATION_ITEM ( '' )  );
#45420=CARTESIAN_POINT ( 'NONE',  ( -18.24929096724884658, -21.81104555038653103, 68.82986815895560540 ) ) ;
#45421=CARTESIAN_POINT ( 'NONE',  ( -20.68530789332051256, -8.558680460152096714, 60.13565450698544623 ) ) ;
#45422=EDGE_CURVE ( 'NONE', #34178, #33339, #42261, .T. ) ;
#45426=ADVANCED_FACE ( 'NONE', ( #36574 ), #33224, .T. ) ;
#45427=ADVANCED_FACE ( 'NONE', ( #26014 ), #41032, .T. ) ;
#45429=CARTESIAN_POINT ( 'NONE',  ( -10.88286923018596575, -17.43962093083235843, 68.11193994895104709 ) ) ;
#45430=CARTESIAN_POINT ( 'NONE',  ( -15.55326400670571196, -7.597850160029695488, 70.65343888371961611 ) ) ;
#45432=( BOUNDED_CURVE ( )  B_SPLINE_CURVE ( 3, ( #23153, #7404, #38386, #27076 ),
 .UNSPECIFIED., .F., .F. ) 
 B_SPLINE_CURVE_WITH_KNOTS ( ( 4, 4 ),
 ( 0.5000000000000000000, 0.9074455897393651771 ),
 .UNSPECIFIED. ) 
 CURVE ( )  GEOMETRIC_REPRESENTATION_ITEM ( )  RATIONAL_B_SPLINE_CURVE ( ( 1.000000000000007772, 0.4567392136813430703, 0.3561768502900289346, 0.6983129098260736356 ) ) 
 REPRESENTATION_ITEM ( '' )  );
#45434=ORIENTED_EDGE ( 'NONE', *, *, #17309, .T. ) ;
#45436=CARTESIAN_POINT ( 'NONE',  ( -20.31796842471441522, -7.944138697998205600, 70.29454436300783016 ) ) ;
#45438=EDGE_CURVE ( 'NONE', #34125, #19673, #10262, .T. ) ;
#45440=VECTOR ( 'NONE', #27752, 1000.000000000000227 ) ;
#45442=CARTESIAN_POINT ( 'NONE',  ( -10.56016083362581703, -13.18709213229180932, 67.62343541709479666 ) ) ;
#45443=FACE_OUTER_BOUND ( 'NONE', #14924, .T. ) ;
#45444=VERTEX_POINT ( 'NONE', #33874 ) ;
#45445=VECTOR ( 'NONE', #40194, 1000.000000000000000 ) ;
#45446=ORIENTED_EDGE ( 'NONE', *, *, #14345, .T. ) ;
#45447=CARTESIAN_POINT ( 'NONE',  ( -22.22371030936713510, -9.111184089457765367, 59.90666523727240644 ) ) ;
#45448=LINE ( 'NONE', #27209, #46229 ) ;
#45450=CARTESIAN_POINT ( 'NONE',  ( -18.12273401612753077, -22.22646211661374593, 65.46036745194116691 ) ) ;
#45452=DIRECTION ( 'NONE',  ( 0.3722980621098854748, 0.2477784351981106581, 0.8944271909999157444 ) ) ;
#45454=B_SPLINE_CURVE_WITH_KNOTS ( 'NONE', 1,
 ( #43093, #1968 ),
 .UNSPECIFIED., .F., .F.,
 ( 2, 2 ),
 ( 0.000000000000000000, 1.000000000000000000 ),
 .UNSPECIFIED. ) ;
#45456=CARTESIAN_POINT ( 'NONE',  ( -19.43641843455863238, -7.636073284130151961, 60.06818851049102648 ) ) ;
#45457=CARTESIAN_POINT ( 'NONE',  ( -19.30271816048872324, -8.014114901043837946, 60.26092997144682073 ) ) ;
#45458=ORIENTED_EDGE ( 'NONE', *, *, #25159, .F. ) ;
#45459=CARTESIAN_POINT ( 'NONE',  ( -19.53281124456648854, -21.95454890610320930, 62.19514848487217051 ) ) ;
#45462=FACE_BOUND ( 'NONE', #14403, .T. ) ;
#45464=EDGE_LOOP ( 'NONE', ( #33469, #18158, #47199, #32404, #4614 ) ) ;
#45466=CARTESIAN_POINT ( 'NONE',  ( -14.98249323814573941, -9.880861343182303358, 54.07175714974879099 ) ) ;
#45467=CARTESIAN_POINT ( 'NONE',  ( -15.17321550381910988, -21.91105134213339412, 68.67569292545161375 ) ) ;
#45468=AXIS2_PLACEMENT_3D ( 'NONE', #41200, #11169, #44198 ) ;
#45469=ORIENTED_EDGE ( 'NONE', *, *, #36048, .F. ) ;
#45471=ORIENTED_EDGE ( 'NONE', *, *, #19788, .T. ) ;
#45474=CARTESIAN_POINT ( 'NONE',  ( -16.71979392375450146, -22.22589398653607873, 68.80286503482692240 ) ) ;
#45475=CARTESIAN_POINT ( 'NONE',  ( -14.29947512317492730, -8.480563224953527879, 63.94546151666516209 ) ) ;
#45476=ORIENTED_EDGE ( 'NONE', *, *, #42576, .T. ) ;
#45479=DIRECTION ( 'NONE',  ( 0.3303050442826436783, -0.9438742382973702716, -3.829623548921168867E-09 ) ) ;
#45480=ORIENTED_EDGE ( 'NONE', *, *, #30300, .F. ) ;
#45481=ORIENTED_EDGE ( 'NONE', *, *, #6512, .T. ) ;
#45482=ORIENTED_EDGE ( 'NONE', *, *, #39329, .T. ) ;
#45483=CARTESIAN_POINT ( 'NONE',  ( -15.66808075433818992, -21.64011062311675815, 71.93086697972334775 ) ) ;
#45484=EDGE_CURVE ( 'NONE', #3450, #43669, #37553, .T. ) ;
#45485=DIRECTION ( 'NONE',  ( 0.2393415023380396911, -0.9709354485539016810, 6.438601123316501445E-08 ) ) ;
#45486=AXIS2_PLACEMENT_3D ( 'NONE', #44612, #41, #18736 ) ;
#45487=CARTESIAN_POINT ( 'NONE',  ( -21.27916101436501251, -20.65201899428944898, 69.16336101976946793 ) ) ;
#45490=CARTESIAN_POINT ( 'NONE',  ( -10.37345536002686686, -17.21617726224556932, 61.29709747334221248 ) ) ;
#45491=CARTESIAN_POINT ( 'NONE',  ( -14.10256296019058198, -8.140532706836228982, 70.84462314181931220 ) ) ;
#45493=VERTEX_POINT ( 'NONE', #7314 ) ;
#45496=CARTESIAN_POINT ( 'NONE',  ( -16.16221056564778991, -7.466773990862017207, 60.24382527849350311 ) ) ;
#45497=CARTESIAN_POINT ( 'NONE',  ( -22.53655473247544805, -20.22829521909097394, 65.88917159596024931 ) ) ;
#45498=CARTESIAN_POINT ( 'NONE',  ( -10.50393358731724369, -15.87404606333056911, 68.16695003737737579 ) ) ;
#45499=CARTESIAN_POINT ( 'NONE',  ( -23.45651108574825372, -18.46362474097727002, 69.17883092557275404 ) ) ;
#45503=ADVANCED_FACE ( 'NONE', ( #37815 ), #41512, .T. ) ;
#45504=ORIENTED_EDGE ( 'NONE', *, *, #3136, .F. ) ;
#45505=CARTESIAN_POINT ( 'NONE',  ( -10.61330328728660533, -12.98831903967553814, 67.73832347272892207 ) ) ;
#45507=AXIS2_PLACEMENT_3D ( 'NONE', #47015, #2854, #42848 ) ;
#45508=CARTESIAN_POINT ( 'NONE',  ( -12.68381388925888587, -19.95990997655619381, 68.63657438305759229 ) ) ;
#45509=( BOUNDED_SURFACE ( )  B_SPLINE_SURFACE ( 3, 1, ( 
 ( #30576, #26140 ),
 ( #23418, #30334 ),
 ( #11850, #16003 ),
 ( #33994, #292 ),
 ( #37937, #42128 ),
 ( #11597, #26627 ),
 ( #4701, #4222 ) ),
 .UNSPECIFIED., .T., .F., .F. ) 
 B_SPLINE_SURFACE_WITH_KNOTS ( ( 4, 3, 4 ),
 ( 2, 2 ),
 ( 0.000000000000000000, 0.5000000000000000000, 1.000000000000000000 ),
 ( 0.000000000000000000, 1.000000000000000000 ),
 .UNSPECIFIED. ) 
 GEOMETRIC_REPRESENTATION_ITEM ( )  RATIONAL_B_SPLINE_SURFACE ( (
 ( 1.000000000000000000, 1.000000000000000000),
 ( 0.3333333333333335369, 0.3333333333333330373),
 ( 0.3333333333333335369, 0.3333333333333330373),
 ( 1.000000000000000000, 1.000000000000000000),
 ( 0.3333333333333333703, 0.3333333333333333703),
 ( 0.3333333333333333703, 0.3333333333333333703),
 ( 1.000000000000000000, 1.000000000000000000) ) ) 
 REPRESENTATION_ITEM ( '' )  SURFACE ( )  );
#45511=ORIENTED_EDGE ( 'NONE', *, *, #25894, .F. ) ;
#45513=B_SPLINE_CURVE_WITH_KNOTS ( 'NONE', 1,
 ( #1448, #46533 ),
 .UNSPECIFIED., .F., .F.,
 ( 2, 2 ),
 ( 0.000000000000000000, 1.000000000000000000 ),
 .UNSPECIFIED. ) ;
#45514=VECTOR ( 'NONE', #22435, 1000.000000000000227 ) ;
#45515=VECTOR ( 'NONE', #47456, 1000.000000000000114 ) ;
#45516=CARTESIAN_POINT ( 'NONE',  ( -10.43073328261085386, -14.50439875238632403, 67.85800126138448718 ) ) ;
#45519=VECTOR ( 'NONE', #20016, 1000.000000000000000 ) ;
#45521=EDGE_CURVE ( 'NONE', #35971, #4639, #23501, .T. ) ;
#45522=LINE ( 'NONE', #12738, #14141 ) ;
#45527=FACE_OUTER_BOUND ( 'NONE', #913, .T. ) ;
#45529=ORIENTED_EDGE ( 'NONE', *, *, #38218, .T. ) ;
#45530=CYLINDRICAL_SURFACE ( 'NONE', #1446, 0.1500000000000006051 ) ;
#45532=CYLINDRICAL_SURFACE ( 'NONE', #1380, 0.1500000000000003553 ) ;
#45534=CARTESIAN_POINT ( 'NONE',  ( -23.90959958070817848, -11.14304846090580980, 70.04210748470214298 ) ) ;
#45535=DIRECTION ( 'NONE',  ( -1.522745435920864373E-06, 7.096186240322379876E-06, -0.9999999999736627343 ) ) ;
#45536=CARTESIAN_POINT ( 'NONE',  ( -11.48064390335815155, -11.11094769457351816, 57.20903159568930363 ) ) ;
#45537=ORIENTED_EDGE ( 'NONE', *, *, #16213, .F. ) ;
#45539=FACE_OUTER_BOUND ( 'NONE', #22204, .T. ) ;
#45540=PLANE ( 'NONE',  #48725 ) ;
#45541=ORIENTED_EDGE ( 'NONE', *, *, #35898, .T. ) ;
#45544=DIRECTION ( 'NONE',  ( -0.8875028193683940358, -0.4608022847308269609, 4.020963237607658939E-08 ) ) ;
#45546=CARTESIAN_POINT ( 'NONE',  ( -23.46741908093438767, -19.16603997859080266, 62.53902161361033052 ) ) ;
#45548=CARTESIAN_POINT ( 'NONE',  ( -20.38226043987465630, -7.971587899251926679, 70.36605015394232510 ) ) ;
#45549=DIRECTION ( 'NONE',  ( -0.9501515917649785425, -0.3117883138709295898, 1.594035198720926202E-08 ) ) ;
#45550=CARTESIAN_POINT ( 'NONE',  ( -12.16409273157858628, -9.533090607804314942, 57.22902139051024051 ) ) ;
#45551=LINE ( 'NONE', #34192, #8989 ) ;
#45553=CARTESIAN_POINT ( 'NONE',  ( -11.01266498513346015, -11.85818215851522339, 67.77431642774575948 ) ) ;
#45554=EDGE_LOOP ( 'NONE', ( #22268, #4320, #13667, #17057, #212 ) ) ;
#45555=EDGE_CURVE ( 'NONE', #32237, #26756, #34658, .T. ) ;
#45556=CARTESIAN_POINT ( 'NONE',  ( -24.39403702774331606, -17.44049340399234893, 69.52844358061491903 ) ) ;
#45557=EDGE_CURVE ( 'NONE', #19035, #39384, #29459, .T. ) ;
#45558=AXIS2_PLACEMENT_3D ( 'NONE', #17403, #21111, #13928 ) ;
#45559=CARTESIAN_POINT ( 'NONE',  ( -10.57990114081760957, -13.11695186304740979, 71.22300718686658172 ) ) ;
#45560=EDGE_CURVE ( 'NONE', #43276, #31666, #7646, .T. ) ;
#45561=CARTESIAN_POINT ( 'NONE',  ( -21.92782103781014413, -9.450273908687094604, 60.02171200090587178 ) ) ;
#45562=( BOUNDED_CURVE ( )  B_SPLINE_CURVE ( 3, ( #12868, #38975, #12633, #27655 ),
 .UNSPECIFIED., .F., .F. ) 
 B_SPLINE_CURVE_WITH_KNOTS ( ( 4, 4 ),
 ( 0.9074455897393682857, 1.000000000000000000 ),
 .UNSPECIFIED. ) 
 CURVE ( )  GEOMETRIC_REPRESENTATION_ITEM ( )  RATIONAL_B_SPLINE_CURVE ( ( 0.6983129098260908441, 0.7760317562606963149, 0.8765941196519994039, 1.000000000000000000 ) ) 
 REPRESENTATION_ITEM ( '' )  );
#45564=ORIENTED_EDGE ( 'NONE', *, *, #35114, .T. ) ;
#45565=CARTESIAN_POINT ( 'NONE',  ( -19.92070420837752565, -21.34886149063710192, 69.13710527445095977 ) ) ;
#45566=FACE_OUTER_BOUND ( 'NONE', #26209, .T. ) ;
#45567=CARTESIAN_POINT ( 'NONE',  ( -22.11925914797909343, -9.024813657292067859, 63.30658454184609241 ) ) ;
#45568=CARTESIAN_POINT ( 'NONE',  ( -15.82259855879412846, -7.533287975791289171, 67.25511890406325222 ) ) ;
#45571=B_SPLINE_CURVE_WITH_KNOTS ( 'NONE', 1,
 ( #191, #22839 ),
 .UNSPECIFIED., .F., .F.,
 ( 2, 2 ),
 ( 0.000000000000000000, 1.000000000000000000 ),
 .UNSPECIFIED. ) ;
#45572=( BOUNDED_SURFACE ( )  B_SPLINE_SURFACE ( 3, 1, ( 
 ( #35799, #16602 ),
 ( #31878, #9486 ),
 ( #39995, #46897 ),
 ( #1841, #28187 ),
 ( #39265, #16838 ),
 ( #36038, #31643 ),
 ( #46664, #24018 ) ),
 .UNSPECIFIED., .T., .F., .F. ) 
 B_SPLINE_SURFACE_WITH_KNOTS ( ( 4, 3, 4 ),
 ( 2, 2 ),
 ( 0.000000000000000000, 0.5000000000000000000, 1.000000000000000000 ),
 ( 0.000000000000000000, 1.000000000000000000 ),
 .UNSPECIFIED. ) 
 GEOMETRIC_REPRESENTATION_ITEM ( )  RATIONAL_B_SPLINE_SURFACE ( (
 ( 1.000000000000000000, 1.000000000000000000),
 ( 0.3333333333333335369, 0.3333333333333330373),
 ( 0.3333333333333335369, 0.3333333333333330373),
 ( 1.000000000000000000, 1.000000000000000000),
 ( 0.3333333333333333703, 0.3333333333333333703),
 ( 0.3333333333333333703, 0.3333333333333333703),
 ( 1.000000000000000000, 1.000000000000000000) ) ) 
 REPRESENTATION_ITEM ( '' )  SURFACE ( )  );
#45574=CARTESIAN_POINT ( 'NONE',  ( -12.99758137947571157, -9.386477775907486887, 71.14925353122600882 ) ) ;
#45575=B_SPLINE_CURVE_WITH_KNOTS ( 'NONE', 3,
 ( #11457, #6793, #33597, #7535, #21808, #14384, #3338, #7045, #10497, #33112 ),
 .UNSPECIFIED., .F., .F.,
 ( 4, 2, 2, 2, 4 ),
 ( 0.1272669073658425354, 0.2522669073463276179, 0.3772669073268126727, 0.5022669073072977275, 0.6272669072877827823 ),
 .UNSPECIFIED. ) ;
#45577=EDGE_CURVE ( 'NONE', #29452, #41905, #1084, .T. ) ;
#45578=EDGE_CURVE ( 'NONE', #26071, #32198, #8120, .T. ) ;
#45579=VERTEX_POINT ( 'NONE', #27945 ) ;
#45582=CARTESIAN_POINT ( 'NONE',  ( -22.14599188607209612, -19.97735994708842355, 65.98805141629955529 ) ) ;
#45584=CARTESIAN_POINT ( 'NONE',  ( -10.42334066387008207, -15.64104445138816679, 61.03789045260961643 ) ) ;
#45589=CYLINDRICAL_SURFACE ( 'NONE', #21064, 0.1499999999999963030 ) ;
#45590=VERTEX_POINT ( 'NONE', #38788 ) ;
#45594=CARTESIAN_POINT ( 'NONE',  ( -17.78823985852933731, -7.818684566706888717, 60.08060768393342954 ) ) ;
#45595=VECTOR ( 'NONE', #1239, 1000.000000000000114 ) ;
#45596=CARTESIAN_POINT ( 'NONE',  ( -12.06140467229625912, -20.05244645202335008, 47.99999999999994316 ) ) ;
#45597=CARTESIAN_POINT ( 'NONE',  ( -22.40450728528633206, -19.80423666046082687, 65.70421711893553152 ) ) ;
#45598=ORIENTED_EDGE ( 'NONE', *, *, #29572, .T. ) ;
#45599=CARTESIAN_POINT ( 'NONE',  ( -24.47295431262708476, -15.06807065624729169, 59.33480201725491554 ) ) ;
#45600=CARTESIAN_POINT ( 'NONE',  ( -12.81450749931373245, -9.474957484202729319, 74.31923006089486705 ) ) ;
#45601=CARTESIAN_POINT ( 'NONE',  ( -22.58065782673598321, -12.89613362149922438, 53.49999999999995026 ) ) ;
#45603=CARTESIAN_POINT ( 'NONE',  ( -22.86572475812252847, -14.01004878893095196, 53.49899999999994549 ) ) ;
#45604=ADVANCED_FACE ( 'NONE', ( #20078 ), #45721, .T. ) ;
#45605=EDGE_LOOP ( 'NONE', ( #32016, #20240, #6927, #27578, #7418 ) ) ;
#45606=EDGE_LOOP ( 'NONE', ( #20436, #46354, #10811, #31284, #33846 ) ) ;
#45607=CARTESIAN_POINT ( 'NONE',  ( -24.49858526622490373, -12.47342014262311949, 73.42038324740811106 ) ) ;
#45609=ORIENTED_EDGE ( 'NONE', *, *, #37736, .F. ) ;
#45610=CARTESIAN_POINT ( 'NONE',  ( -24.05059659118241555, -17.06519001246171996, 72.88336032079776317 ) ) ;
#45611=DIRECTION ( 'NONE',  ( 0.8398192074808117358, 0.5428661886195298436, 7.907900705247678986E-08 ) ) ;
#45613=PLANE ( 'NONE',  #2220 ) ;
#45614=CARTESIAN_POINT ( 'NONE',  ( -12.08906526520849489, -20.00921629736058804, 61.59667419651943021 ) ) ;
#45615=CARTESIAN_POINT ( 'NONE',  ( -11.40656469618873814, -19.20173789643934015, 71.84832430454555663 ) ) ;
#45618=CARTESIAN_POINT ( 'NONE',  ( -11.55573786329523855, -10.21941616939416342, 71.15388509157428132 ) ) ;
#45619=EDGE_CURVE ( 'NONE', #33140, #5827, #42008, .T. ) ;
#45624=CARTESIAN_POINT ( 'NONE',  ( -18.26345899425187369, -22.21252533677388286, 65.45876839498835409 ) ) ;
#45626=ORIENTED_EDGE ( 'NONE', *, *, #37674, .F. ) ;
#45628=CARTESIAN_POINT ( 'NONE',  ( -20.17979545193272273, -21.30158238988698116, 72.28990119599492914 ) ) ;
#45629=EDGE_LOOP ( 'NONE', ( #29345, #18560 ) ) ;
#45630=CYLINDRICAL_SURFACE ( 'NONE', #31926, 0.1499999999999992450 ) ;
#45631=CARTESIAN_POINT ( 'NONE',  ( -16.54715509603413537, -21.75405920933647863, 61.86454047598803641 ) ) ;
#45633=CARTESIAN_POINT ( 'NONE',  ( -15.84452207058844486, -7.934630762070933763, 63.67010736139238958 ) ) ;
#45634=EDGE_CURVE ( 'NONE', #40340, #4523, #20325, .T. ) ;
#45635=EDGE_CURVE ( 'NONE', #45990, #3943, #46788, .T. ) ;
#45636=DIRECTION ( 'NONE',  ( 0.1261685609230673022, 0.9920088176193797569, 5.058037262945178882E-08 ) ) ;
#45638=ORIENTED_EDGE ( 'NONE', *, *, #10646, .T. ) ;
#45639=CARTESIAN_POINT ( 'NONE',  ( -18.11889201384288128, -21.82488578508536747, 65.34532159284481168 ) ) ;
#45640=CARTESIAN_POINT ( 'NONE',  ( -24.16016232491792337, -12.71630861904342069, 66.30246503819121529 ) ) ;
#45643=CARTESIAN_POINT ( 'NONE',  ( -15.29809632361469873, -21.47854941203162937, 68.57592918283285144 ) ) ;
#45645=EDGE_CURVE ( 'NONE', #5827, #40125, #31086, .T. ) ;
#45648=CARTESIAN_POINT ( 'NONE',  ( -12.81450527785482407, -9.474959380418823685, 74.61923006088066757 ) ) ;
#45649=CARTESIAN_POINT ( 'NONE',  ( -12.55198883488284878, -12.25722835735234639, 53.49999999999995026 ) ) ;
#45650=ORIENTED_EDGE ( 'NONE', *, *, #22170, .T. ) ;
#45651=CARTESIAN_POINT ( 'NONE',  ( -10.90458911758865312, -11.20383709417547280, 64.34870811186064543 ) ) ;
#45652=CARTESIAN_POINT ( 'NONE',  ( -15.02405691534179688, -8.340062653448299557, 56.49999999999994316 ) ) ;
#45653=VECTOR ( 'NONE', #44071, 1000.000000000000114 ) ;
#45657=VERTEX_POINT ( 'NONE', #27708 ) ;
#45666=LINE ( 'NONE', #8713, #40050 ) ;
#45668=VERTEX_POINT ( 'NONE', #23788 ) ;
#45669=CARTESIAN_POINT ( 'NONE',  ( -15.68502974777997316, -7.977065180327441496, 70.90989839958919561 ) ) ;
#45671=EDGE_LOOP ( 'NONE', ( #11880, #28956, #23149, #18311, #4009 ) ) ;
#45672=PLANE ( 'NONE',  #5049 ) ;
#45673=CARTESIAN_POINT ( 'NONE',  ( -24.42421125441087071, -14.80070621231813455, 59.24300242292227381 ) ) ;
#45674=FACE_OUTER_BOUND ( 'NONE', #4306, .T. ) ;
#45675=ORIENTED_EDGE ( 'NONE', *, *, #23391, .T. ) ;
#45677=CARTESIAN_POINT ( 'NONE',  ( -10.77303304197945621, -12.62668734528506853, 61.09853568451838868 ) ) ;
#45678=CYLINDRICAL_SURFACE ( 'NONE', #30066, 0.1500000000000057676 ) ;
#45680=CARTESIAN_POINT ( 'NONE',  ( -23.10699383429526321, -18.89654842981622807, 62.35406835440843309 ) ) ;
#45681=ORIENTED_EDGE ( 'NONE', *, *, #17524, .F. ) ;
#45684=CARTESIAN_POINT ( 'NONE',  ( -22.94595275489701081, -9.807970174690861853, 70.20452678257210266 ) ) ;
#45685=AXIS2_PLACEMENT_3D ( 'NONE', #9121, #31765, #16962 ) ;
#45686=CARTESIAN_POINT ( 'NONE',  ( -24.16575310113231012, -12.74704012323608104, 70.07243002239954421 ) ) ;
#45687=DIRECTION ( 'NONE',  ( -0.7700094066334506326, -0.6380325334150297456, 6.510647142068518693E-17 ) ) ;
#45688=AXIS2_PLACEMENT_3D ( 'NONE', #33918, #210, #34154 ) ;
#45689=PRODUCT ( 'Pin Studded Brass Music Cylinder', 'Pin Studded Brass Music Cylinder', '', ( #30932 ) ) ;
#45692=CARTESIAN_POINT ( 'NONE',  ( -17.98657259272421172, -21.83703102787368167, 62.16063850355641307 ) ) ;
#45693=CARTESIAN_POINT ( 'NONE',  ( -13.91545454884148825, -8.237059506355153715, 74.45600559034086530 ) ) ;
#45694=CARTESIAN_POINT ( 'NONE',  ( -13.73934026678462850, -20.82397421667150894, 61.51646026183723137 ) ) ;
#45695=( BOUNDED_SURFACE ( )  B_SPLINE_SURFACE ( 3, 1, ( 
 ( #5151, #46755 ),
 ( #46269, #43311 ),
 ( #39598, #12998 ),
 ( #19925, #12526 ),
 ( #28029, #20161 ),
 ( #27551, #43052 ),
 ( #35648, #1930 ) ),
 .UNSPECIFIED., .T., .F., .F. ) 
 B_SPLINE_SURFACE_WITH_KNOTS ( ( 4, 3, 4 ),
 ( 2, 2 ),
 ( 0.000000000000000000, 0.5000000000000000000, 1.000000000000000000 ),
 ( 0.000000000000000000, 1.000000000000000000 ),
 .UNSPECIFIED. ) 
 GEOMETRIC_REPRESENTATION_ITEM ( )  RATIONAL_B_SPLINE_SURFACE ( (
 ( 1.000000000000000000, 1.000000000000000000),
 ( 0.3333333333333335369, 0.3333333333333330373),
 ( 0.3333333333333335369, 0.3333333333333330373),
 ( 1.000000000000000000, 1.000000000000000000),
 ( 0.3333333333333333703, 0.3333333333333333703),
 ( 0.3333333333333333703, 0.3333333333333333703),
 ( 1.000000000000000000, 1.000000000000000000) ) ) 
 REPRESENTATION_ITEM ( '' )  SURFACE ( )  );
#45696=ORIENTED_EDGE ( 'NONE', *, *, #39962, .T. ) ;
#45697=CYLINDRICAL_SURFACE ( 'NONE', #12357, 0.1500000000000026867 ) ;
#45698=ORIENTED_EDGE ( 'NONE', *, *, #2717, .F. ) ;
#45701=CARTESIAN_POINT ( 'NONE',  ( -20.98638901306355820, -20.89730141071840208, 69.35450455931557201 ) ) ;
#45702=CARTESIAN_POINT ( 'NONE',  ( -12.58002213166789041, -9.148928514680237711, 74.43427606957253317 ) ) ;
#45703=LINE ( 'NONE', #41498, #13608 ) ;
#45707=CARTESIAN_POINT ( 'NONE',  ( -17.98424483515344718, -22.23819686138322638, 61.91890007431585019 ) ) ;
#45708=CARTESIAN_POINT ( 'NONE',  ( -14.66315376424047301, -7.889636616332322383, 60.51334572945852130 ) ) ;
#45710=( BOUNDED_SURFACE ( )  B_SPLINE_SURFACE ( 3, 1, ( 
 ( #25454, #6742 ),
 ( #21757, #38713 ),
 ( #15560, #15814 ),
 ( #35011, #23470 ),
 ( #41933, #30134 ),
 ( #5000, #20009 ),
 ( #38466, #37734 ) ),
 .UNSPECIFIED., .T., .F., .F. ) 
 B_SPLINE_SURFACE_WITH_KNOTS ( ( 4, 3, 4 ),
 ( 2, 2 ),
 ( 0.000000000000000000, 0.5000000000000000000, 1.000000000000000000 ),
 ( 0.000000000000000000, 1.000000000000000000 ),
 .UNSPECIFIED. ) 
 GEOMETRIC_REPRESENTATION_ITEM ( )  RATIONAL_B_SPLINE_SURFACE ( (
 ( 1.000000000000000000, 1.000000000000000000),
 ( 0.3333333333333335369, 0.3333333333333330373),
 ( 0.3333333333333335369, 0.3333333333333330373),
 ( 1.000000000000000000, 1.000000000000000000),
 ( 0.3333333333333333703, 0.3333333333333333703),
 ( 0.3333333333333333703, 0.3333333333333333703),
 ( 1.000000000000000000, 1.000000000000000000) ) ) 
 REPRESENTATION_ITEM ( '' )  SURFACE ( )  );
#45711=CARTESIAN_POINT ( 'NONE',  ( -10.33699397268960674, -12.51219692611108236, 60.90515267099636532 ) ) ;
#45712=CARTESIAN_POINT ( 'NONE',  ( -20.88147576600584543, -8.209942340109883219, 60.02620652709861560 ) ) ;
#45713=EDGE_LOOP ( 'NONE', ( #34708, #6524, #11775, #13895, #16052 ) ) ;
#45714=CARTESIAN_POINT ( 'NONE',  ( -19.98813040044048606, -21.37641421727040125, 72.40478737316021807 ) ) ;
#45715=CARTESIAN_POINT ( 'NONE',  ( -17.78683253498428485, -22.25049694173829096, 58.58270294325748750 ) ) ;
#45716=( BOUNDED_SURFACE ( )  B_SPLINE_SURFACE ( 3, 1, ( 
 ( #26831, #37642 ),
 ( #33444, #37143 ),
 ( #14717, #25842 ),
 ( #40860, #22393 ),
 ( #7638, #3678 ),
 ( #11809, #41108 ),
 ( #29788, #10819 ) ),
 .UNSPECIFIED., .T., .F., .F. ) 
 B_SPLINE_SURFACE_WITH_KNOTS ( ( 4, 3, 4 ),
 ( 2, 2 ),
 ( 0.000000000000000000, 0.5000000000000000000, 1.000000000000000000 ),
 ( 0.000000000000000000, 1.000000000000000000 ),
 .UNSPECIFIED. ) 
 GEOMETRIC_REPRESENTATION_ITEM ( )  RATIONAL_B_SPLINE_SURFACE ( (
 ( 1.000000000000000000, 1.000000000000000000),
 ( 0.3333333333333335369, 0.3333333333333330373),
 ( 0.3333333333333335369, 0.3333333333333330373),
 ( 1.000000000000000000, 1.000000000000000000),
 ( 0.3333333333333333703, 0.3333333333333333703),
 ( 0.3333333333333333703, 0.3333333333333333703),
 ( 1.000000000000000000, 1.000000000000000000) ) ) 
 REPRESENTATION_ITEM ( '' )  SURFACE ( )  );
#45717=CARTESIAN_POINT ( 'NONE',  ( -24.33163080547450718, -17.59998302563209904, 66.09357240084537466 ) ) ;
#45720=VECTOR ( 'NONE', #8361, 1000.000000000000227 ) ;
#45721=CYLINDRICAL_SURFACE ( 'NONE', #11686, 0.1500000000000037970 ) ;
#45722=DIRECTION ( 'NONE',  ( 0.3636930986378154040, 0.9315188296557533887, -1.850371886801397658E-09 ) ) ;
#45726=CARTESIAN_POINT ( 'NONE',  ( -10.64577744754535082, -11.71757184301072563, 74.67344733366148546 ) ) ;
#45727=ORIENTED_EDGE ( 'NONE', *, *, #10028, .T. ) ;
#45728=CARTESIAN_POINT ( 'NONE',  ( -14.07539681412750809, -8.605278097683306981, 74.49954655214880006 ) ) ;
#45729=VERTEX_POINT ( 'NONE', #28916 ) ;
#45730=FACE_OUTER_BOUND ( 'NONE', #12831, .T. ) ;
#45731=CARTESIAN_POINT ( 'NONE',  ( -13.25597844349469057, -9.183841988267115397, 67.60772729950176085 ) ) ;
#45732=ORIENTED_EDGE ( 'NONE', *, *, #1294, .T. ) ;
#45734=( BOUNDED_CURVE ( )  B_SPLINE_CURVE ( 3, ( #11773, #26791, #929, #41816 ),
 .UNSPECIFIED., .F., .F. ) 
 B_SPLINE_CURVE_WITH_KNOTS ( ( 4, 4 ),
 ( 0.000000000000000000, 0.4074455897393705062 ),
 .UNSPECIFIED. ) 
 CURVE ( )  GEOMETRIC_REPRESENTATION_ITEM ( )  RATIONAL_B_SPLINE_CURVE ( ( 1.000000000000000000, 0.4567392136813268610, 0.3561768502900283795, 0.6983129098261044998 ) ) 
 REPRESENTATION_ITEM ( '' )  );
#45735=FACE_BOUND ( 'NONE', #19132, .T. ) ;
#45737=ORIENTED_EDGE ( 'NONE', *, *, #19290, .T. ) ;
#45738=EDGE_LOOP ( 'NONE', ( #11964, #16899, #11276, #29712, #29660 ) ) ;
#45741=CARTESIAN_POINT ( 'NONE',  ( -16.43513463834741728, -22.19403045546258468, 65.41219756188628764 ) ) ;
#45742=CYLINDRICAL_SURFACE ( 'NONE', #11797, 0.1500000000000009936 ) ;
#45743=CARTESIAN_POINT ( 'NONE',  ( -11.82668574982945664, -9.892677223491459060, 64.13576029842931803 ) ) ;
#45744=FACE_OUTER_BOUND ( 'NONE', #8894, .T. ) ;
#45746=ORIENTED_EDGE ( 'NONE', *, *, #47131, .T. ) ;
#45747=CARTESIAN_POINT ( 'NONE',  ( -17.65810221059773610, -7.762793303104815301, 63.56529088875731759 ) ) ;
#45748=AXIS2_PLACEMENT_3D ( 'NONE', #2378, #35616, #5610 ) ;
#45749=CARTESIAN_POINT ( 'NONE',  ( -9.990737576226866423, -14.31032742905966337, 64.43157936802064967 ) ) ;
#45751=DIRECTION ( 'NONE',  ( -0.8507615431891570879, 0.5255518971808580408, 6.876821558984483597E-08 ) ) ;
#45752=ORIENTED_EDGE ( 'NONE', *, *, #1986, .T. ) ;
#45755=ORIENTED_EDGE ( 'NONE', *, *, #18957, .T. ) ;
#45757=CARTESIAN_POINT ( 'NONE',  ( -15.74783386771837890, -7.961078896070159061, 70.62461975990308360 ) ) ;
#45758=ADVANCED_FACE ( 'NONE', ( #39520 ), #23214, .T. ) ;
#45759=CARTESIAN_POINT ( 'NONE',  ( -12.10599122619147749, -20.02663529450013513, 61.58173959111590534 ) ) ;
#45760=CARTESIAN_POINT ( 'NONE',  ( -10.47387877723939731, -13.58059689071059495, 57.59258137113961595 ) ) ;
#45761=VERTEX_POINT ( 'NONE', #39757 ) ;
#45763=CARTESIAN_POINT ( 'NONE',  ( -12.17725024227025621, -10.08844384719822429, 57.24502831558379512 ) ) ;
#45767=CARTESIAN_POINT ( 'NONE',  ( -11.04141237841800560, -11.93494539390495568, 74.85840195306853673 ) ) ;
#45769=CARTESIAN_POINT ( 'NONE',  ( -17.60317953294568127, -7.758478677834707682, 67.43528183898541783 ) ) ;
#45771=ORIENTED_EDGE ( 'NONE', *, *, #18789, .T. ) ;
#45773=ORIENTED_EDGE ( 'NONE', *, *, #38662, .T. ) ;
#45774=CARTESIAN_POINT ( 'NONE',  ( -24.71344798646422802, -16.35160113208834431, 62.77984073303771595 ) ) ;
#45775=EDGE_CURVE ( 'NONE', #31812, #1447, #4949, .T. ) ;
#45776=EDGE_LOOP ( 'NONE', ( #41566, #35930 ) ) ;
#45777=CARTESIAN_POINT ( 'NONE',  ( -24.46479343890040070, -14.44719913075708817, 66.48292729247950206 ) ) ;
#45780=B_SPLINE_CURVE_WITH_KNOTS ( 'NONE', 3,
 ( #42930, #5512, #20530, #35532, #1806, #13107, #36707, #10645, #14306, #43915 ),
 .UNSPECIFIED., .F., .F.,
 ( 4, 2, 2, 2, 4 ),
 ( 0.6272669072877762320, 0.7522669073072868473, 0.8772669073267975737, 1.002266907346308189, 1.127266907365818804 ),
 .UNSPECIFIED. ) ;
#45781=ORIENTED_EDGE ( 'NONE', *, *, #34171, .F. ) ;
#45782=CARTESIAN_POINT ( 'NONE',  ( -21.31800492490012999, -20.62620369199774117, 72.52446429884872714 ) ) ;
#45783=ADVANCED_FACE ( 'NONE', ( #13872 ), #21622, .T. ) ;
#45784=CARTESIAN_POINT ( 'NONE',  ( -16.34731059182330526, -7.892077880983075389, 60.21645166852753306 ) ) ;
#45785=DIRECTION ( 'NONE',  ( -0.9990515194385546360, -0.04354378839186318767, 1.103613758316041215E-08 ) ) ;
#45787=DIRECTION ( 'NONE',  ( -0.9410372374137779827, -0.3383029970317210644, -1.029646047569396398E-09 ) ) ;
#45788=EDGE_LOOP ( 'NONE', ( #8922, #19663, #1519, #24647 ) ) ;
#45791=CARTESIAN_POINT ( 'NONE',  ( -22.84587788576350675, -10.37951466216800966, 66.61352538834459835 ) ) ;
#45795=CARTESIAN_POINT ( 'NONE',  ( -11.51240771850610933, -10.27427218717217627, 71.08237763624090633 ) ) ;
#45796=CARTESIAN_POINT ( 'NONE',  ( -18.56710112356817532, -7.447357278511908873, 74.03338530932549588 ) ) ;
#45797=CARTESIAN_POINT ( 'NONE',  ( -12.11393208253047149, -10.17166670693309349, 64.32354556750141228 ) ) ;
#45799=EDGE_LOOP ( 'NONE', ( #42353, #43319, #25193, #42229, #46586 ) ) ;
#45800=CARTESIAN_POINT ( 'NONE',  ( -22.71059208588729561, -10.14448404190931186, 70.02650598627910483 ) ) ;
#45801=CARTESIAN_POINT ( 'NONE',  ( -10.02816200250604872, -13.91188849819191553, 57.58678490442956388 ) ) ;
#45806=LINE ( 'NONE', #19692, #24901 ) ;
#45807=DIRECTION ( 'NONE',  ( -4.734277553319870270E-07, 1.363385191780837012E-06, 0.9999999999989586108 ) ) ;
#45814=ORIENTED_EDGE ( 'NONE', *, *, #41378, .F. ) ;
#45815=EDGE_CURVE ( 'NONE', #43494, #7495, #1701, .T. ) ;
#45816=FACE_OUTER_BOUND ( 'NONE', #31200, .T. ) ;
#45817=ORIENTED_EDGE ( 'NONE', *, *, #28706, .F. ) ;
#45819=ORIENTED_EDGE ( 'NONE', *, *, #33099, .T. ) ;
#45821=EDGE_CURVE ( 'NONE', #18340, #5003, #42376, .T. ) ;
#45822=CARTESIAN_POINT ( 'NONE',  ( -19.29992334121955366, -21.55324995122935761, 58.81041981532258944 ) ) ;
#45823=ORIENTED_EDGE ( 'NONE', *, *, #19436, .T. ) ;
#45825=CARTESIAN_POINT ( 'NONE',  ( -24.27033112822875793, -13.12649005559073245, 63.13264177271827293 ) ) ;
#45829=DIRECTION ( 'NONE',  ( -5.731567514496413899E-31, -1.020425574103664789E-16, -1.000000000000000000 ) ) ;
#45830=CARTESIAN_POINT ( 'NONE',  ( -14.97035482569482312, -21.41873484682592377, 61.92128389535452015 ) ) ;
#45831=ORIENTED_EDGE ( 'NONE', *, *, #3066, .T. ) ;
#45835=CARTESIAN_POINT ( 'NONE',  ( -18.34835985623554677, -21.74804277390830975, 68.81514668082158437 ) ) ;
#45836=CARTESIAN_POINT ( 'NONE',  ( -12.74802523442671465, -20.09592109768945889, 65.02242199588995675 ) ) ;
#45837=EDGE_LOOP ( 'NONE', ( #15373, #35869, #13553, #4518, #38594 ) ) ;
#45838=ORIENTED_EDGE ( 'NONE', *, *, #18929, .T. ) ;
#45839=DIRECTION ( 'NONE',  ( 3.084459863448555673E-06, -5.853393718798201518E-06, 0.9999999999781119531 ) ) ;
#45840=LINE ( 'NONE', #38677, #46253 ) ;
#45841=VERTEX_POINT ( 'NONE', #45867 ) ;
#45842=CARTESIAN_POINT ( 'NONE',  ( -10.42131017383741032, -15.64935787052201910, 57.45304097017945111 ) ) ;
#45843=CARTESIAN_POINT ( 'NONE',  ( -15.74601971208386786, -7.550529481922165331, 67.26194484337577251 ) ) ;
#45845=CARTESIAN_POINT ( 'NONE',  ( -14.81535805098777736, -7.777528402031244958, 75.49999999999994316 ) ) ;
#45846=( BOUNDED_CURVE ( )  B_SPLINE_CURVE ( 3, ( #39073, #694, #38592, #5114 ),
 .UNSPECIFIED., .F., .F. ) 
 B_SPLINE_CURVE_WITH_KNOTS ( ( 4, 4 ),
 ( 4.712388980384689674, 4.921828490624008623 ),
 .UNSPECIFIED. ) 
 CURVE ( )  GEOMETRIC_REPRESENTATION_ITEM ( )  RATIONAL_B_SPLINE_CURVE ( ( 1.000000000000000000, 0.9963479302455156006, 0.9963479302455156006, 1.000000000000000000 ) ) 
 REPRESENTATION_ITEM ( '' )  );
#45847=EDGE_CURVE ( 'NONE', #43944, #1710, #34518, .T. ) ;
#45848=CARTESIAN_POINT ( 'NONE',  ( -14.28769015366465567, -8.051497000463099241, 67.51620991724109899 ) ) ;
#45851=EDGE_CURVE ( 'NONE', #27306, #7306, #9891, .T. ) ;
#45853=CARTESIAN_POINT ( 'NONE',  ( -24.39511741622861507, -15.44614315551445571, 73.22977031223102529 ) ) ;
#45856=CARTESIAN_POINT ( 'NONE',  ( -10.63004074901718532, -12.92571453866564823, 67.75304464120749515 ) ) ;
#45858=CARTESIAN_POINT ( 'NONE',  ( -15.88655729437939534, -7.980152340574909076, 67.44007279406643818 ) ) ;
#45859=( BOUNDED_SURFACE ( )  B_SPLINE_SURFACE ( 3, 1, ( 
 ( #32218, #16690 ),
 ( #2414, #47234 ),
 ( #10048, #25721 ),
 ( #5148, #28025 ),
 ( #31730, #46519 ),
 ( #27786, #46752 ),
 ( #12994, #43049 ) ),
 .UNSPECIFIED., .T., .F., .F. ) 
 B_SPLINE_SURFACE_WITH_KNOTS ( ( 4, 3, 4 ),
 ( 2, 2 ),
 ( 0.000000000000000000, 0.5000000000000000000, 1.000000000000000000 ),
 ( 0.000000000000000000, 1.000000000000000000 ),
 .UNSPECIFIED. ) 
 GEOMETRIC_REPRESENTATION_ITEM ( )  RATIONAL_B_SPLINE_SURFACE ( (
 ( 1.000000000000000000, 1.000000000000000000),
 ( 0.3333333333333335369, 0.3333333333333330373),
 ( 0.3333333333333335369, 0.3333333333333330373),
 ( 1.000000000000000000, 1.000000000000000000),
 ( 0.3333333333333333703, 0.3333333333333333703),
 ( 0.3333333333333333703, 0.3333333333333333703),
 ( 1.000000000000000000, 1.000000000000000000) ) ) 
 REPRESENTATION_ITEM ( '' )  SURFACE ( )  );
#45862=FACE_OUTER_BOUND ( 'NONE', #13216, .T. ) ;
#45863=ORIENTED_EDGE ( 'NONE', *, *, #12060, .T. ) ;
#45864=CARTESIAN_POINT ( 'NONE',  ( -11.21783104652298846, -18.93062367394879431, 64.93202350587574756 ) ) ;
#45866=ORIENTED_EDGE ( 'NONE', *, *, #26341, .T. ) ;
#45867=CARTESIAN_POINT ( 'NONE',  ( -10.40888626530166405, -14.10966241957602385, 60.91821293886854249 ) ) ;
#45868=CARTESIAN_POINT ( 'NONE',  ( -13.61216655543990584, -20.68217103177308047, 65.09702080378529843 ) ) ;
#45869=CARTESIAN_POINT ( 'NONE',  ( -16.91855125566938511, -22.24212016642244905, 72.28047911973106920 ) ) ;
#45872=CARTESIAN_POINT ( 'NONE',  ( -20.90293659130012216, -8.221317335593040454, 60.04114024615370937 ) ) ;
#45873=DIRECTION ( 'NONE',  ( 0.8467008005855419794, -0.3141239757129650201, 0.4294460177601872597 ) ) ;
#45874=ORIENTED_EDGE ( 'NONE', *, *, #18454, .T. ) ;
#45876=CARTESIAN_POINT ( 'NONE',  ( -23.93244369146852080, -17.39065619829227671, 69.60266770082890275 ) ) ;
#45877=VERTEX_POINT ( 'NONE', #46098 ) ;
#45879=CARTESIAN_POINT ( 'NONE',  ( -22.20824715029565866, -20.52011977224520223, 58.86419268801586924 ) ) ;
#45881=CARTESIAN_POINT ( 'NONE',  ( -24.00920687666620168, -12.43512006407420145, 73.35111597096941694 ) ) ;
#45883=CARTESIAN_POINT ( 'NONE',  ( -23.25280541480605834, -10.16922674724575693, 63.17911852083285851 ) ) ;
#45884=CARTESIAN_POINT ( 'NONE',  ( -17.80126953765676845, -21.79909748901075517, 58.42055855158453426 ) ) ;
#45885=CARTESIAN_POINT ( 'NONE',  ( -23.58616520728616806, -18.99640775243969060, 66.00884813586510802 ) ) ;
#45887=CARTESIAN_POINT ( 'NONE',  ( -24.36621887139804699, -13.91093020482227693, 73.31374677385069560 ) ) ;
#45888=CARTESIAN_POINT ( 'NONE',  ( -10.42052617248403124, -15.61735782369945547, 61.03789063027900141 ) ) ;
#45889=CYLINDRICAL_SURFACE ( 'NONE', #36778, 0.1499999999999963585 ) ;
#45890=CARTESIAN_POINT ( 'NONE',  ( -24.25171713147202368, -16.35308467727669068, 59.12332432120680181 ) ) ;
#45891=CARTESIAN_POINT ( 'NONE',  ( -14.90981300391230846, -21.39562377109201208, 61.63600440604547970 ) ) ;
#45893=ORIENTED_EDGE ( 'NONE', *, *, #46915, .T. ) ;
#45895=CARTESIAN_POINT ( 'NONE',  ( -10.47936380272204104, -17.50656370757942781, 64.78772765493845043 ) ) ;
#45897=CARTESIAN_POINT ( 'NONE',  ( -16.17793336889135603, -22.15441545345155205, 58.44618891099874958 ) ) ;
#45899=LINE ( 'NONE', #4776, #36775 ) ;
#45900=ORIENTED_EDGE ( 'NONE', *, *, #21553, .T. ) ;
#45901=CARTESIAN_POINT ( 'NONE',  ( -23.65624121974494898, -11.51332442490695307, 66.42214514605623776 ) ) ;
#45904=CARTESIAN_POINT ( 'NONE',  ( -23.51785719624223958, -11.36449344406884343, 70.19210750610864125 ) ) ;
#45905=EDGE_CURVE ( 'NONE', #34665, #7279, #7545, .T. ) ;
#45906=EDGE_CURVE ( 'NONE', #29749, #4669, #48355, .T. ) ;
#45907=ORIENTED_EDGE ( 'NONE', *, *, #26113, .F. ) ;
#45909=CARTESIAN_POINT ( 'NONE',  ( -13.29699920919266631, -9.093425021029217348, 63.90946558901772079 ) ) ;
#45910=CARTESIAN_POINT ( 'NONE',  ( -24.39403702774331606, -17.44049340399234893, 69.52844358061491903 ) ) ;
#45911=CARTESIAN_POINT ( 'NONE',  ( -24.55620591900586902, -12.65601924842659720, 69.96581314741867175 ) ) ;
#45912=CARTESIAN_POINT ( 'NONE',  ( -23.23616624490289340, -18.79948399208958776, 66.12389430041484673 ) ) ;
#45913=CARTESIAN_POINT ( 'NONE',  ( -10.84300597751149553, -17.34773470226564029, 61.15743043792785016 ) ) ;
#45915=ORIENTED_EDGE ( 'NONE', *, *, #44515, .T. ) ;
#45917=CARTESIAN_POINT ( 'NONE',  ( -11.93102662126159785, -10.47028825497329585, 70.96893105764984000 ) ) ;
#45918=CARTESIAN_POINT ( 'NONE',  ( -24.15877587438482976, -12.72423012542946807, 70.07242983926148838 ) ) ;
#45919=CARTESIAN_POINT ( 'NONE',  ( -18.52416312356643147, -7.896186446804856374, 73.84064402154488960 ) ) ;
#45921=EDGE_CURVE ( 'NONE', #7173, #10403, #39913, .T. ) ;
#45922=CARTESIAN_POINT ( 'NONE',  ( -12.77796340496265692, -17.75258416873320400, 54.07175714974880520 ) ) ;
#45923=FACE_OUTER_BOUND ( 'NONE', #34183, .T. ) ;
#45924=VERTEX_POINT ( 'NONE', #21207 ) ;
#45925=CARTESIAN_POINT ( 'NONE',  ( -24.32852063849251323, -13.38246526728995001, 59.37740068604990995 ) ) ;
#45926=B_SPLINE_CURVE_WITH_KNOTS ( 'NONE', 1,
 ( #8628, #27326 ),
 .UNSPECIFIED., .F., .F.,
 ( 2, 2 ),
 ( 0.000000000000000000, 1.000000000000000000 ),
 .UNSPECIFIED. ) ;
#45928=EDGE_LOOP ( 'NONE', ( #43707, #26727, #14003, #27997, #36034 ) ) ;
#45929=CARTESIAN_POINT ( 'NONE',  ( -22.96481576609224717, -19.16891988936071556, 58.89882756593014790 ) ) ;
#45931=VERTEX_POINT ( 'NONE', #20721 ) ;
#45932=CARTESIAN_POINT ( 'NONE',  ( -13.24261801534493088, -8.643248549050911222, 60.55454889300790455 ) ) ;
#45935=DIRECTION ( 'NONE',  ( 0.9271861211590526342, 0.3746009833543293421, -1.005599061620490611E-08 ) ) ;
#45937=CARTESIAN_POINT ( 'NONE',  ( -10.39693166811831304, -15.37990016280386740, 57.58264896457095006 ) ) ;
#45938=CARTESIAN_POINT ( 'NONE',  ( -20.94465790601859467, -8.243431112063134947, 59.95629843672877257 ) ) ;
#45939=ORIENTED_EDGE ( 'NONE', *, *, #21406, .F. ) ;
#45940=CARTESIAN_POINT ( 'NONE',  ( -21.79028809537168243, -9.273590339475653366, 63.47681654923867711 ) ) ;
#45941=FACE_OUTER_BOUND ( 'NONE', #45799, .T. ) ;
#45943=FACE_BOUND ( 'NONE', #26490, .T. ) ;
#45945=CARTESIAN_POINT ( 'NONE',  ( -11.36794959886231915, -18.31963617796164812, 57.80714594517343841 ) ) ;
#45946=CARTESIAN_POINT ( 'NONE',  ( -19.98813035779708969, -21.37641423362171267, 72.55478737316022375 ) ) ;
#45947=DIRECTION ( 'NONE',  ( -0.9584484254710481377, -0.2852658684667118139, 3.516456354099036190E-08 ) ) ;
#45950=VERTEX_POINT ( 'NONE', #29313 ) ;
#45951=CARTESIAN_POINT ( 'NONE',  ( -11.95727733380162050, -19.27338395605723420, 71.84252737392968413 ) ) ;
#45952=CARTESIAN_POINT ( 'NONE',  ( -22.90877043182983286, -10.45950943414446854, 63.37186031185718349 ) ) ;
#45954=CARTESIAN_POINT ( 'NONE',  ( -24.32852063849251323, -13.38246526728995001, 59.37740068604990995 ) ) ;
#45955=FACE_BOUND ( 'NONE', #23278, .T. ) ;
#45956=VERTEX_POINT ( 'NONE', #32983 ) ;
#45957=EDGE_CURVE ( 'NONE', #40380, #2617, #28533, .T. ) ;
#45958=ORIENTED_EDGE ( 'NONE', *, *, #38080, .T. ) ;
#45959=ORIENTED_EDGE ( 'NONE', *, *, #26194, .F. ) ;
#45960=CARTESIAN_POINT ( 'NONE',  ( -17.71668947275567874, -21.85613660542494685, 62.29024590482070778 ) ) ;
#45961=CARTESIAN_POINT ( 'NONE',  ( -13.73970969606274473, -20.76112332560825990, 65.28628881671112083 ) ) ;
#45963=CARTESIAN_POINT ( 'NONE',  ( -14.51896086823277443, -8.440036041935664812, 67.27591678782368945 ) ) ;
#45964=CARTESIAN_POINT ( 'NONE',  ( -19.28939461086542906, -8.062307027802660286, 60.26092997386343342 ) ) ;
#45965=VERTEX_POINT ( 'NONE', #43384 ) ;
#45969=EDGE_CURVE ( 'NONE', #18851, #1251, #10120, .T. ) ;
#45972=EDGE_CURVE ( 'NONE', #8735, #26020, #12243, .T. ) ;
#45973=CARTESIAN_POINT ( 'NONE',  ( -11.82605070163061534, -9.893394921550459742, 64.22188489775784603 ) ) ;
#45974=PLANE ( 'NONE',  #31509 ) ;
#45975=CARTESIAN_POINT ( 'NONE',  ( -19.63985863958091116, -21.44939509270802702, 65.76486191116302393 ) ) ;
#45976=EDGE_CURVE ( 'NONE', #39245, #12574, #29071, .T. ) ;
#45978=( BOUNDED_CURVE ( )  B_SPLINE_CURVE ( 3, ( #2168, #47958, #6107, #3135 ),
 .UNSPECIFIED., .F., .F. ) 
 B_SPLINE_CURVE_WITH_KNOTS ( ( 4, 4 ),
 ( 0.000000000000000000, 0.4074455897393572390 ),
 .UNSPECIFIED. ) 
 CURVE ( )  GEOMETRIC_REPRESENTATION_ITEM ( )  RATIONAL_B_SPLINE_CURVE ( ( 1.000000000000000000, 0.4567392136813397396, 0.3561768502900331534, 0.6983129098260801859 ) ) 
 REPRESENTATION_ITEM ( '' )  );
#45980=ORIENTED_EDGE ( 'NONE', *, *, #42518, .F. ) ;
#45981=CARTESIAN_POINT ( 'NONE',  ( -16.16816684335524457, -21.69572884791061540, 58.58585623285081567 ) ) ;
#45983=CARTESIAN_POINT ( 'NONE',  ( -24.46043589294705001, -17.25765543095130639, 73.02302651788181720 ) ) ;
#45985=B_SPLINE_CURVE_WITH_KNOTS ( 'NONE', 3,
 ( #47343, #1790, #31339, #17274, #5496, #43156, #46617, #28385, #39458, #32321 ),
 .UNSPECIFIED., .F., .F.,
 ( 4, 2, 2, 2, 4 ),
 ( 0.000000000000000000, 0.2500000000000000000, 0.5000000000000000000, 0.7500000000000000000, 1.000000000000000000 ),
 .UNSPECIFIED. ) ;
#45987=( BOUNDED_CURVE ( )  B_SPLINE_CURVE ( 3, ( #43677, #9930, #24949, #36258 ),
 .UNSPECIFIED., .F., .F. ) 
 B_SPLINE_CURVE_WITH_KNOTS ( ( 4, 4 ),
 ( 0.9074455897393653991, 1.000000000000000000 ),
 .UNSPECIFIED. ) 
 CURVE ( )  GEOMETRIC_REPRESENTATION_ITEM ( )  RATIONAL_B_SPLINE_CURVE ( ( 0.6983129098261022794, 0.7760317562607061959, 0.8765941196520053991, 1.000000000000000000 ) ) 
 REPRESENTATION_ITEM ( '' )  );
#45988=CARTESIAN_POINT ( 'NONE',  ( -10.42579980212244983, -14.65467349332582714, 68.04903362315590698 ) ) ;
#45990=VERTEX_POINT ( 'NONE', #35719 ) ;
#45991=CARTESIAN_POINT ( 'NONE',  ( -14.67111564601650997, -7.886426081561471513, 60.43500846974642116 ) ) ;
#45994=ORIENTED_EDGE ( 'NONE', *, *, #1154, .T. ) ;
#45995=CARTESIAN_POINT ( 'NONE',  ( -16.04111743724699224, -7.488525900945328218, 63.83157579393176917 ) ) ;
#45996=( BOUNDED_CURVE ( )  B_SPLINE_CURVE ( 3, ( #11050, #26073, #41085, #44309 ),
 .UNSPECIFIED., .F., .F. ) 
 B_SPLINE_CURVE_WITH_KNOTS ( ( 4, 4 ),
 ( 0.9074455897393604031, 1.000000000000000000 ),
 .UNSPECIFIED. ) 
 CURVE ( )  GEOMETRIC_REPRESENTATION_ITEM ( )  RATIONAL_B_SPLINE_CURVE ( ( 0.6983129098260856260, 0.7760317562606918740, 0.8765941196519966283, 1.000000000000000000 ) ) 
 REPRESENTATION_ITEM ( '' )  );
#45999=CARTESIAN_POINT ( 'NONE',  ( -9.974456273375457371, -14.72748566909688073, 71.51278126739182994 ) ) ;
#46000=CARTESIAN_POINT ( 'NONE',  ( -23.77487038158592014, -11.74745262826995429, 62.96690348473899235 ) ) ;
#46002=CARTESIAN_POINT ( 'NONE',  ( -18.57089378905319421, -22.17041224548506406, 72.43510938007564448 ) ) ;
#46003=CARTESIAN_POINT ( 'NONE',  ( -11.02242957576233451, -11.85532881267382166, 74.57312195644870201 ) ) ;
#46005=CARTESIAN_POINT ( 'NONE',  ( -16.19814190158817269, -21.75179548504963023, 58.43585572027992470 ) ) ;
#46006=EDGE_LOOP ( 'NONE', ( #1960, #43802 ) ) ;
#46007=CARTESIAN_POINT ( 'NONE',  ( -9.996765541055841808, -14.22627829241283770, 64.52770499853964736 ) ) ;
#46009=CARTESIAN_POINT ( 'NONE',  ( -15.11368083008136587, -21.89207339945041753, 68.71559548072659140 ) ) ;
#46011=CARTESIAN_POINT ( 'NONE',  ( -19.63868610202945675, -21.50238589859430149, 65.76486200656573544 ) ) ;
#46012=CARTESIAN_POINT ( 'NONE',  ( -11.07857809310684338, -11.73724795245126273, 71.38860870961248395 ) ) ;
#46013=ORIENTED_EDGE ( 'NONE', *, *, #35841, .F. ) ;
#46014=CARTESIAN_POINT ( 'NONE',  ( -15.82259747647940173, -7.533288219471245384, 67.25511999279136433 ) ) ;
#46015=CARTESIAN_POINT ( 'NONE',  ( -11.31808814922340822, -18.33929587155208552, 61.69199689979424051 ) ) ;
#46017=ORIENTED_EDGE ( 'NONE', *, *, #48609, .F. ) ;
#46018=ORIENTED_EDGE ( 'NONE', *, *, #41035, .F. ) ;
#46021=CARTESIAN_POINT ( 'NONE',  ( -10.37743123699495307, -15.12446308634721603, 74.79778699417029486 ) ) ;
#46023=CARTESIAN_POINT ( 'NONE',  ( -12.43267529144301520, -19.71710391272808849, 61.39678636628809727 ) ) ;
#46024=CARTESIAN_POINT ( 'NONE',  ( -24.05420634179087358, -17.20676946999824608, 69.69867738674849988 ) ) ;
#46025=CARTESIAN_POINT ( 'NONE',  ( -10.37394849890712401, -14.76283852923608286, 71.61310637325181006 ) ) ;
#46026=ORIENTED_EDGE ( 'NONE', *, *, #40392, .F. ) ;
#46027=ORIENTED_EDGE ( 'NONE', *, *, #16553, .F. ) ;
#46028=CARTESIAN_POINT ( 'NONE',  ( -22.62394951084894146, -10.04809318868971424, 70.29706442286226320 ) ) ;
#46030=EDGE_CURVE ( 'NONE', #14825, #10444, #4654, .T. ) ;
#46031=CARTESIAN_POINT ( 'NONE',  ( -14.60783614669699304, -21.70648650955843806, 58.35113213314874514 ) ) ;
#46033=CARTESIAN_POINT ( 'NONE',  ( -18.90456104531098092, -7.507023198961870314, 70.55723427638547207 ) ) ;
#46034=ADVANCED_FACE ( 'NONE', ( #19203 ), #37660, .T. ) ;
#46035=ORIENTED_EDGE ( 'NONE', *, *, #3136, .T. ) ;
#46036=AXIS2_PLACEMENT_3D ( 'NONE', #14307, #48548, #44628 ) ;
#46037=ORIENTED_EDGE ( 'NONE', *, *, #42135, .T. ) ;
#46038=DIRECTION ( 'NONE',  ( 0.06357898915123888495, -0.9979768094191902028, 2.038786632797724544E-16 ) ) ;
#46039=CARTESIAN_POINT ( 'NONE',  ( -14.93767672275562575, -21.83209540852061181, 65.29934976567700744 ) ) ;
#46042=EDGE_LOOP ( 'NONE', ( #30900, #14438 ) ) ;
#46043=FACE_OUTER_BOUND ( 'NONE', #45188, .T. ) ;
#46046=CYLINDRICAL_SURFACE ( 'NONE', #36710, 0.1500000000000007716 ) ;
#46047=DIRECTION ( 'NONE',  ( 0.8507615431891570879, -0.5255518971808580408, -6.876821557926347540E-08 ) ) ;
#46048=VERTEX_POINT ( 'NONE', #7656 ) ;
#46049=CARTESIAN_POINT ( 'NONE',  ( -23.65754020941666269, -18.88946062594842701, 69.47184773153367132 ) ) ;
#46050=EDGE_LOOP ( 'NONE', ( #9227, #10057 ) ) ;
#46051=CYLINDRICAL_SURFACE ( 'NONE', #7112, 0.1500000000000061007 ) ;
#46052=FACE_OUTER_BOUND ( 'NONE', #6388, .T. ) ;
#46053=ORIENTED_EDGE ( 'NONE', *, *, #17440, .F. ) ;
#46054=CARTESIAN_POINT ( 'NONE',  ( -23.96654618570108042, -17.44381333609114648, 62.35872369075587329 ) ) ;
#46057=CARTESIAN_POINT ( 'NONE',  ( -11.97955916273614285, -10.40884600102296176, 70.98509759323277990 ) ) ;
#46058=EDGE_CURVE ( 'NONE', #4721, #5613, #16325, .T. ) ;
#46059=CARTESIAN_POINT ( 'NONE',  ( -19.24190786459753610, -7.584296138276666710, 63.54593947706258206 ) ) ;
#46060=LINE ( 'NONE', #7677, #38405 ) ;
#46062=PLANE ( 'NONE',  #16840 ) ;
#46063=CARTESIAN_POINT ( 'NONE',  ( -11.43058294688041165, -10.38410865082031442, 74.48239070398270201 ) ) ;
#46066=PLANE ( 'NONE',  #1479 ) ;
#46067=DIRECTION ( 'NONE',  ( -1.069388061899112173E-05, 2.778940573026428581E-06, 0.9999999999389591609 ) ) ;
#46068=VERTEX_POINT ( 'NONE', #30062 ) ;
#46070=CARTESIAN_POINT ( 'NONE',  ( -15.35027035934970918, -7.653577032698213323, 74.26481056556292515 ) ) ;
#46071=CARTESIAN_POINT ( 'NONE',  ( -24.37683887807358118, -15.97618392648307761, 66.36324926629207255 ) ) ;
#46072=ORIENTED_EDGE ( 'NONE', *, *, #26113, .T. ) ;
#46073=CARTESIAN_POINT ( 'NONE',  ( -22.48237781098097798, -19.73147542146173450, 65.85988959519353614 ) ) ;
#46074=CYLINDRICAL_SURFACE ( 'NONE', #5891, 0.1499999999999979128 ) ;
#46075=CARTESIAN_POINT ( 'NONE',  ( -23.04367355717579002, -10.55211556811382678, 59.90203429191419104 ) ) ;
#46076=CARTESIAN_POINT ( 'NONE',  ( -24.74348659356070002, -16.19898255343749582, 62.73182120491487268 ) ) ;
#46077=B_SPLINE_CURVE_WITH_KNOTS ( 'NONE', 3,
 ( #14160, #7548, #30205, #33126, #40775, #45226, #44735, #29455, #26010, #26493 ),
 .UNSPECIFIED., .F., .F.,
 ( 4, 2, 2, 2, 4 ),
 ( 0.000000000000000000, 0.2500000000000000000, 0.5000000000000000000, 0.7500000000000000000, 1.000000000000000000 ),
 .UNSPECIFIED. ) ;
#46078=CARTESIAN_POINT ( 'NONE',  ( -12.10067708704646527, -20.02116635982656945, 61.58952802380450464 ) ) ;
#46083=DIRECTION ( 'NONE',  ( 0.1738928961406289442, -0.9847645711904030597, -7.871847300026996438E-08 ) ) ;
#46085=CARTESIAN_POINT ( 'NONE',  ( -22.66727108289645543, -10.09628893573625064, 70.01178520457129650 ) ) ;
#46087=CARTESIAN_POINT ( 'NONE',  ( -11.86838218109940790, -9.845554053733961197, 64.14419007574942100 ) ) ;
#46088=EDGE_CURVE ( 'NONE', #31720, #15639, #37516, .T. ) ;
#46091=CARTESIAN_POINT ( 'NONE',  ( -20.16691211377460391, -21.73601867580754288, 72.58974061177721637 ) ) ;
#46092=EDGE_CURVE ( 'NONE', #21832, #43615, #3430, .T. ) ;
#46094=CARTESIAN_POINT ( 'NONE',  ( -12.00385017463665704, -9.698023059171664073, 60.75256377526179818 ) ) ;
#46095=CARTESIAN_POINT ( 'NONE',  ( -17.42409385541300892, -14.80920654474439679, 54.49999999999994316 ) ) ;
#46096=EDGE_CURVE ( 'NONE', #28180, #44222, #28110, .T. ) ;
#46097=EDGE_LOOP ( 'NONE', ( #25625, #6342, #560, #32935 ) ) ;
#46098=CARTESIAN_POINT ( 'NONE',  ( -11.14114473067313682, -10.80566704772025233, 57.32407823191172014 ) ) ;
#46100=CARTESIAN_POINT ( 'NONE',  ( -13.36271920075327557, -8.563530200375994994, 57.07629425018297553 ) ) ;
#46101=ORIENTED_EDGE ( 'NONE', *, *, #33107, .F. ) ;
#46102=CARTESIAN_POINT ( 'NONE',  ( -20.93707211197437346, -8.239410368917360117, 60.03463562270969334 ) ) ;
#46103=CARTESIAN_POINT ( 'NONE',  ( -23.77826926726992340, -17.74977703228070069, 62.66287969925918588 ) ) ;
#46104=ORIENTED_EDGE ( 'NONE', *, *, #46979, .F. ) ;
#46105=CARTESIAN_POINT ( 'NONE',  ( -19.97164249076357478, -21.81019033462135326, 69.11977790463622284 ) ) ;
#46106=EDGE_CURVE ( 'NONE', #39956, #8033, #3051, .T. ) ;
#46107=CARTESIAN_POINT ( 'NONE',  ( -13.53919695188330508, -21.16624214383947589, 65.10816087775715744 ) ) ;
#46108=EDGE_CURVE ( 'NONE', #26226, #41394, #26348, .T. ) ;
#46110=CARTESIAN_POINT ( 'NONE',  ( -10.37081839464344668, -14.73079292305692789, 67.85800084537061139 ) ) ;
#46111=CARTESIAN_POINT ( 'NONE',  ( -16.98902004117856990, -21.84877635801032270, 68.58071880800348197 ) ) ;
#46112=CARTESIAN_POINT ( 'NONE',  ( -18.53201708017407157, -7.846807123103141102, 74.14064401780551350 ) ) ;
#46114=CARTESIAN_POINT ( 'NONE',  ( -10.91516777394897986, -11.18477724879597623, 64.34893244028862114 ) ) ;
#46115=CARTESIAN_POINT ( 'NONE',  ( -19.42896492416523913, -21.56812594671148275, 61.99503644571810668 ) ) ;
#46116=( BOUNDED_SURFACE ( )  B_SPLINE_SURFACE ( 3, 1, ( 
 ( #21480, #36234 ),
 ( #3236, #28389 ),
 ( #2517, #10399 ),
 ( #17277, #6692 ),
 ( #47578, #39700 ),
 ( #20988, #32781 ),
 ( #47347, #13810 ) ),
 .UNSPECIFIED., .T., .F., .F. ) 
 B_SPLINE_SURFACE_WITH_KNOTS ( ( 4, 3, 4 ),
 ( 2, 2 ),
 ( 0.000000000000000000, 0.5000000000000000000, 1.000000000000000000 ),
 ( 0.000000000000000000, 1.000000000000000000 ),
 .UNSPECIFIED. ) 
 GEOMETRIC_REPRESENTATION_ITEM ( )  RATIONAL_B_SPLINE_SURFACE ( (
 ( 1.000000000000000000, 1.000000000000000000),
 ( 0.3333333333333335369, 0.3333333333333330373),
 ( 0.3333333333333335369, 0.3333333333333330373),
 ( 1.000000000000000000, 1.000000000000000000),
 ( 0.3333333333333333703, 0.3333333333333333703),
 ( 0.3333333333333333703, 0.3333333333333333703),
 ( 1.000000000000000000, 1.000000000000000000) ) ) 
 REPRESENTATION_ITEM ( '' )  SURFACE ( )  );
#46117=EDGE_CURVE ( 'NONE', #21578, #20573, #33526, .T. ) ;
#46119=CARTESIAN_POINT ( 'NONE',  ( -21.18398698114219769, -21.24092341087395752, 65.69958654271196963 ) ) ;
#46121=CARTESIAN_POINT ( 'NONE',  ( -13.71339271347210342, -20.80363700974685059, 65.28628881287177421 ) ) ;
#46122=CYLINDRICAL_SURFACE ( 'NONE', #6167, 0.1499999999999991618 ) ;
#46126=ORIENTED_EDGE ( 'NONE', *, *, #47427, .T. ) ;
#46128=FACE_OUTER_BOUND ( 'NONE', #24892, .T. ) ;
#46129=ORIENTED_EDGE ( 'NONE', *, *, #15162, .F. ) ;
#46131=CARTESIAN_POINT ( 'NONE',  ( -10.63483715323753565, -17.87674169505483235, 71.75213630217804450 ) ) ;
#46132=CARTESIAN_POINT ( 'NONE',  ( -24.46812100523181144, -14.51191712007779699, 66.19764790277996269 ) ) ;
#46136=( BOUNDED_CURVE ( )  B_SPLINE_CURVE ( 3, ( #15101, #355, #7263, #10941 ),
 .UNSPECIFIED., .F., .F. ) 
 B_SPLINE_CURVE_WITH_KNOTS ( ( 4, 4 ),
 ( 0.4074455897393662873, 0.5000000000000000000 ),
 .UNSPECIFIED. ) 
 CURVE ( )  GEOMETRIC_REPRESENTATION_ITEM ( )  RATIONAL_B_SPLINE_CURVE ( ( 0.6983129098260991707, 0.7760317562607093045, 0.8765941196520112833, 1.000000000000009326 ) ) 
 REPRESENTATION_ITEM ( '' )  );
#46137=AXIS2_PLACEMENT_3D ( 'NONE', #40878, #24902, #47319 ) ;
#46138=CARTESIAN_POINT ( 'NONE',  ( -24.42401644153718721, -14.84212863923847081, 59.24300237020570137 ) ) ;
#46140=DIRECTION ( 'NONE',  ( -2.526377660313140381E-06, -1.273612632024531482E-05, 0.9999999999157043185 ) ) ;
#46142=CARTESIAN_POINT ( 'NONE',  ( -13.31471556610697249, -9.080541429120991381, 63.91506350995963714 ) ) ;
#46146=CARTESIAN_POINT ( 'NONE',  ( -21.77128597137166111, -8.759032111691572808, 70.23158298676763422 ) ) ;
#46147=PLANE ( 'NONE',  #10252 ) ;
#46148=ORIENTED_EDGE ( 'NONE', *, *, #34445, .T. ) ;
#46151=EDGE_CURVE ( 'NONE', #15790, #700, #26111, .T. ) ;
#46152=B_SPLINE_CURVE_WITH_KNOTS ( 'NONE', 3,
 ( #27849, #24167, #24657, #46583, #32030, #32285, #2477, #5703, #36191, #1756 ),
 .UNSPECIFIED., .F., .F.,
 ( 4, 2, 2, 2, 4 ),
 ( 0.1272669073658771188, 0.2522669073439901544, 0.3772669073221032177, 0.5022669073002161699, 0.6272669072783292332 ),
 .UNSPECIFIED. ) ;
#46153=CARTESIAN_POINT ( 'NONE',  ( -22.99810592004713072, -9.865991162508992218, 70.17325022503489151 ) ) ;
#46156=CARTESIAN_POINT ( 'NONE',  ( -10.78905035535072265, -17.04131954076935074, 61.44126548158209289 ) ) ;
#46157=CARTESIAN_POINT ( 'NONE',  ( -24.47368665962210343, -14.70950332193510590, 62.72768537250228604 ) ) ;
#46158=CARTESIAN_POINT ( 'NONE',  ( -10.43972881942000086, -15.77115500203794873, 64.52243715390834211 ) ) ;
#46159=CARTESIAN_POINT ( 'NONE',  ( -18.32364513544568752, -21.80460793730824420, 65.23043427352648393 ) ) ;
#46161=CARTESIAN_POINT ( 'NONE',  ( -21.63336539757928634, -9.153348366551478321, 66.94677872351418557 ) ) ;
#46163=CARTESIAN_POINT ( 'NONE',  ( -21.36284794767689377, -21.13297080501056513, 69.16954792666395235 ) ) ;
#46167=ORIENTED_EDGE ( 'NONE', *, *, #25297, .F. ) ;
#46168=CARTESIAN_POINT ( 'NONE',  ( -21.53861794036900079, -21.02004141303368101, 72.63951040967180006 ) ) ;
#46169=CARTESIAN_POINT ( 'NONE',  ( -13.60238606012557483, -8.884930320952351579, 56.96967755506135234 ) ) ;
#46171=ORIENTED_EDGE ( 'NONE', *, *, #28298, .T. ) ;
#46172=EDGE_CURVE ( 'NONE', #313, #35202, #21665, .T. ) ;
#46173=DIRECTION ( 'NONE',  ( 0.7700094066334507437, 0.6380325334150297456, 2.326497556385334706E-17 ) ) ;
#46175=CARTESIAN_POINT ( 'NONE',  ( -21.90726424129253047, -20.25032565763172343, 58.77002696425551420 ) ) ;
#46176=VECTOR ( 'NONE', #4996, 1000.000000000000000 ) ;
#46177=CARTESIAN_POINT ( 'NONE',  ( -21.73229268148169879, -8.731123941674052702, 70.17486588183628271 ) ) ;
#46178=CARTESIAN_POINT ( 'NONE',  ( -24.30269901035189761, -16.11584067364758610, 66.17398127870760050 ) ) ;
#46179=ORIENTED_EDGE ( 'NONE', *, *, #48623, .T. ) ;
#46180=CARTESIAN_POINT ( 'NONE',  ( -10.95917937052863422, -17.62195967018737619, 71.58190244267143498 ) ) ;
#46181=CARTESIAN_POINT ( 'NONE',  ( -10.91684962386814917, -11.18174702714047442, 64.24907796807872273 ) ) ;
#46182=CARTESIAN_POINT ( 'NONE',  ( -17.42409385541300892, -14.80920654474439679, 47.99999999999994316 ) ) ;
#46185=CARTESIAN_POINT ( 'NONE',  ( -11.53247150430815715, -18.68106468654471541, 64.89707076448696910 ) ) ;
#46186=CARTESIAN_POINT ( 'NONE',  ( -10.54994933093899867, -13.24305344519376781, 71.49356453765415154 ) ) ;
#46187=ORIENTED_EDGE ( 'NONE', *, *, #22141, .T. ) ;
#46189=ORIENTED_EDGE ( 'NONE', *, *, #25919, .F. ) ;
#46190=B_SPLINE_CURVE_WITH_KNOTS ( 'NONE', 3,
 ( #28047, #2191, #29690, #22062, #48393, #20912, #24851, #40765, #5894, #37061 ),
 .UNSPECIFIED., .F., .F.,
 ( 4, 2, 2, 2, 4 ),
 ( 0.6272669072877737895, 0.7522669073072834056, 0.8772669073267929107, 1.002266907346302638, 1.127266907365812143 ),
 .UNSPECIFIED. ) ;
#46191=CARTESIAN_POINT ( 'NONE',  ( -11.19248847611778785, -11.62034934314885959, 67.61864580749579545 ) ) ;
#46192=CARTESIAN_POINT ( 'NONE',  ( -16.77486212007157818, -22.23091360578541043, 68.80222337029485402 ) ) ;
#46193=ORIENTED_EDGE ( 'NONE', *, *, #32593, .F. ) ;
#46195=FACE_BOUND ( 'NONE', #39196, .T. ) ;
#46196=EDGE_LOOP ( 'NONE', ( #19756, #33073, #31665, #6066, #41838 ) ) ;
#46197=ADVANCED_FACE ( 'NONE', ( #30391 ), #580, .T. ) ;
#46199=VERTEX_POINT ( 'NONE', #45890 ) ;
#46200=CARTESIAN_POINT ( 'NONE',  ( -17.98657259272421172, -21.83703102787368167, 62.16063850355641307 ) ) ;
#46201=CARTESIAN_POINT ( 'NONE',  ( -18.73233999060757426, -21.74043542732912826, 72.49330701881069672 ) ) ;
#46203=CARTESIAN_POINT ( 'NONE',  ( -14.41428173599358331, -7.994163662063686893, 63.97474278339937115 ) ) ;
#46204=CARTESIAN_POINT ( 'NONE',  ( -12.57344172079930544, -19.85833258862019335, 68.52584420683459143 ) ) ;
#46205=CARTESIAN_POINT ( 'NONE',  ( -16.30609998749194745, -22.17489236838497746, 61.94906455514021815 ) ) ;
#46207=ORIENTED_EDGE ( 'NONE', *, *, #33600, .F. ) ;
#46208=ORIENTED_EDGE ( 'NONE', *, *, #33169, .T. ) ;
#46210=EDGE_CURVE ( 'NONE', #9191, #42180, #14555, .T. ) ;
#46212=CARTESIAN_POINT ( 'NONE',  ( -21.00380318978402627, -21.34292366101719196, 62.22975991904223747 ) ) ;
#46213=VECTOR ( 'NONE', #26429, 999.9999999999998863 ) ;
#46214=CARTESIAN_POINT ( 'NONE',  ( -21.49816216734858898, -9.116934002111024782, 70.13132539266752019 ) ) ;
#46215=ORIENTED_EDGE ( 'NONE', *, *, #20900, .T. ) ;
#46217=EDGE_LOOP ( 'NONE', ( #37564, #2702 ) ) ;
#46218=CARTESIAN_POINT ( 'NONE',  ( -23.00382044653182945, -10.58231046269237829, 59.60203429539187425 ) ) ;
#46220=DIRECTION ( 'NONE',  ( -0.9959323210854037489, 0.09010444948746665350, 2.601165157765155817E-08 ) ) ;
#46221=VERTEX_POINT ( 'NONE', #37994 ) ;
#46222=DIRECTION ( 'NONE',  ( -0.5881408891789771110, -0.8087584895849666555, 7.565907428972492613E-08 ) ) ;
#46223=CARTESIAN_POINT ( 'NONE',  ( -22.79960313759534074, -9.650943445293346912, 73.66656413195866548 ) ) ;
#46224=CARTESIAN_POINT ( 'NONE',  ( -10.43073325114686511, -14.50439929630985603, 68.15800126138398696 ) ) ;
#46225=EDGE_CURVE ( 'NONE', #44868, #26800, #10132, .T. ) ;
#46226=EDGE_CURVE ( 'NONE', #1531, #8650, #14671, .T. ) ;
#46227=CARTESIAN_POINT ( 'NONE',  ( -22.84073111900424990, -19.92438295589304786, 72.78254066635705044 ) ) ;
#46228=ORIENTED_EDGE ( 'NONE', *, *, #27487, .T. ) ;
#46229=VECTOR ( 'NONE', #871, 1000.000000000000114 ) ;
#46230=CARTESIAN_POINT ( 'NONE',  ( -14.10256395084115866, -8.140532207465255965, 70.84462205307964666 ) ) ;
#46232=CARTESIAN_POINT ( 'NONE',  ( -20.43185948505062299, -8.432683554863363184, 66.79576150497511833 ) ) ;
#46233=EDGE_LOOP ( 'NONE', ( #3295, #20176, #1610, #28928, #20787 ) ) ;
#46234=CARTESIAN_POINT ( 'NONE',  ( -16.00230047675183087, -7.496128538412458298, 63.87022237253693646 ) ) ;
#46237=ORIENTED_EDGE ( 'NONE', *, *, #28308, .F. ) ;
#46238=CARTESIAN_POINT ( 'NONE',  ( -15.28965001900414755, -21.53148179447737220, 64.99108044553886998 ) ) ;
#46239=ADVANCED_FACE ( 'NONE', ( #23240 ), #19050, .T. ) ;
#46241=CARTESIAN_POINT ( 'NONE',  ( -15.03263910315855512, -8.176888424288380364, 56.86472059657746314 ) ) ;
#46244=CARTESIAN_POINT ( 'NONE',  ( -10.72017361938626934, -12.61779402817458973, 57.21368711609748203 ) ) ;
#46245=CARTESIAN_POINT ( 'NONE',  ( -14.21809028606166869, -8.084188479104598812, 67.38162348312260974 ) ) ;
#46247=EDGE_LOOP ( 'NONE', ( #14990, #44045, #21057, #14577, #2803 ) ) ;
#46248=FACE_OUTER_BOUND ( 'NONE', #28455, .T. ) ;
#46249=FACE_OUTER_BOUND ( 'NONE', #20083, .T. ) ;
#46250=CARTESIAN_POINT ( 'NONE',  ( -23.10220861922097768, -9.986187529005633223, 66.69182256001187170 ) ) ;
#46251=FACE_OUTER_BOUND ( 'NONE', #48534, .T. ) ;
#46252=VERTEX_POINT ( 'NONE', #3792 ) ;
#46253=VECTOR ( 'NONE', #12576, 1000.000000000000227 ) ;
#46254=CARTESIAN_POINT ( 'NONE',  ( -24.72559841154505023, -16.28986789441275107, 62.77141465262073439 ) ) ;
#46255=EDGE_CURVE ( 'NONE', #7279, #34665, #31620, .T. ) ;
#46258=CARTESIAN_POINT ( 'NONE',  ( -10.49223796394545616, -15.78356480554473862, 61.14675028274938740 ) ) ;
#46259=CARTESIAN_POINT ( 'NONE',  ( -10.54994933093899867, -13.24305344519376959, 71.49356453765415154 ) ) ;
#46260=DIRECTION ( 'NONE',  ( 0.9294853595766526810, 0.3688590060343663324, 6.440324111080732189E-17 ) ) ;
#46262=CARTESIAN_POINT ( 'NONE',  ( -12.18719842096713357, -10.08886484896570934, 64.04386393395434141 ) ) ;
#46263=( BOUNDED_CURVE ( )  B_SPLINE_CURVE ( 3, ( #2603, #25728, #6299, #9989 ),
 .UNSPECIFIED., .F., .F. ) 
 B_SPLINE_CURVE_WITH_KNOTS ( ( 4, 4 ),
 ( 1.675516081914553590, 1.780235837034217283 ),
 .UNSPECIFIED. ) 
 CURVE ( )  GEOMETRIC_REPRESENTATION_ITEM ( )  RATIONAL_B_SPLINE_CURVE ( ( 1.000000000000000000, 0.9990863565030491111, 0.9990863565030491111, 1.000000000000000000 ) ) 
 REPRESENTATION_ITEM ( '' )  );
#46268=ORIENTED_EDGE ( 'NONE', *, *, #24687, .T. ) ;
#46269=CARTESIAN_POINT ( 'NONE',  ( -10.85811841353450369, -12.22020323829153554, 74.71407760726656022 ) ) ;
#46270=B_SPLINE_CURVE_WITH_KNOTS ( 'NONE', 3,
 ( #25687, #37981, #15317, #4266, #29885, #41199, #18286, #40707, #14333, #22746 ),
 .UNSPECIFIED., .F., .F.,
 ( 4, 2, 2, 2, 4 ),
 ( 0.000000000000000000, 0.2500000000000000000, 0.5000000000000000000, 0.7500000000000000000, 1.000000000000000000 ),
 .UNSPECIFIED. ) ;
#46272=CARTESIAN_POINT ( 'NONE',  ( -21.91034545428830782, -20.18261758176410936, 58.76442899736473180 ) ) ;
#46274=CARTESIAN_POINT ( 'NONE',  ( -21.95938932932862642, -9.477124872050278981, 60.02171213236835712 ) ) ;
#46275=CARTESIAN_POINT ( 'NONE',  ( -23.90247617018859572, -17.59042147582948701, 62.76801221965811095 ) ) ;
#46279=AXIS2_PLACEMENT_3D ( 'NONE', #44991, #14896, #18112 ) ;
#46280=ORIENTED_EDGE ( 'NONE', *, *, #6281, .F. ) ;
#46281=CARTESIAN_POINT ( 'NONE',  ( -19.92716201441182378, -21.34638099545626133, 69.11007586060172514 ) ) ;
#46282=CARTESIAN_POINT ( 'NONE',  ( -24.46146587544552276, -14.38248120490118787, 66.46820668217904426 ) ) ;
#46283=B_SPLINE_CURVE_WITH_KNOTS ( 'NONE', 3,
 ( #38871, #1689, #1192, #43048, #23866, #9326, #19681, #8354, #45796, #34687 ),
 .UNSPECIFIED., .F., .F.,
 ( 4, 2, 2, 2, 4 ),
 ( 0.1272669073658402039, 0.2522669073463257305, 0.3772669073268112294, 0.5022669073072968393, 0.6272669072877823382 ),
 .UNSPECIFIED. ) ;
#46284=CARTESIAN_POINT ( 'NONE',  ( -17.33262245845742910, -7.759502110702281463, 67.30567542699309058 ) ) ;
#46285=CARTESIAN_POINT ( 'NONE',  ( -15.81422232498451130, -7.535173854406034266, 67.33345604418946095 ) ) ;
#46287=ORIENTED_EDGE ( 'NONE', *, *, #41377, .F. ) ;
#46288=CARTESIAN_POINT ( 'NONE',  ( -24.46828707212341669, -14.45681828193256280, 70.06763959435293998 ) ) ;
#46289=( BOUNDED_CURVE ( )  B_SPLINE_CURVE ( 3, ( #45912, #42936, #26953, #9211 ),
 .UNSPECIFIED., .F., .F. ) 
 B_SPLINE_CURVE_WITH_KNOTS ( ( 4, 4 ),
 ( 0.9074455897393635118, 1.000000000000000000 ),
 .UNSPECIFIED. ) 
 CURVE ( )  GEOMETRIC_REPRESENTATION_ITEM ( )  RATIONAL_B_SPLINE_CURVE ( ( 0.6983129098260891787, 0.7760317562606948716, 0.8765941196519985157, 1.000000000000000000 ) ) 
 REPRESENTATION_ITEM ( '' )  );
#46290=ADVANCED_FACE ( 'NONE', ( #35990 ), #27650, .T. ) ;
#46292=CARTESIAN_POINT ( 'NONE',  ( -12.86132678492178982, -20.11796087281938838, 71.80653668692889369 ) ) ;
#46294=ORIENTED_EDGE ( 'NONE', *, *, #11328, .T. ) ;
#46295=CARTESIAN_POINT ( 'NONE',  ( -13.29821074602480557, -9.088145836456059001, 67.47123022012044657 ) ) ;
#46297=ADVANCED_FACE ( 'NONE', ( #9908 ), #13334, .T. ) ;
#46299=CARTESIAN_POINT ( 'NONE',  ( -10.42407724285790138, -14.83420999182403577, 71.55456108509550006 ) ) ;
#46300=ORIENTED_EDGE ( 'NONE', *, *, #17770, .T. ) ;
#46301=CARTESIAN_POINT ( 'NONE',  ( -24.44689184067228638, -14.18710713894228093, 69.93803194250310185 ) ) ;
#46302=CARTESIAN_POINT ( 'NONE',  ( -10.29602973214897155, -12.64239231158840759, 64.39119220775197050 ) ) ;
#46306=CARTESIAN_POINT ( 'NONE',  ( -23.53384949963793105, -19.19053592108923212, 53.76227901944321275 ) ) ;
#46308=VECTOR ( 'NONE', #21505, 1000.000000000000000 ) ;
#46309=CARTESIAN_POINT ( 'NONE',  ( -10.64890997270348549, -11.71061566262665998, 74.68123243985192516 ) ) ;
#46310=CARTESIAN_POINT ( 'NONE',  ( -16.43749525924751964, -22.19434601430465293, 61.86912739712975906 ) ) ;
#46311=VERTEX_POINT ( 'NONE', #16302 ) ;
#46313=AXIS2_PLACEMENT_3D ( 'NONE', #41522, #33373, #3866 ) ;
#46315=CARTESIAN_POINT ( 'NONE',  ( -10.95467737376780271, -17.63084047650967889, 64.78306623841410783 ) ) ;
#46317=CARTESIAN_POINT ( 'NONE',  ( -24.59503728228645159, -12.78882255129604850, 66.47963607747338699 ) ) ;
#46318=CARTESIAN_POINT ( 'NONE',  ( -20.68576141724628670, -21.00469082583299496, 62.30398495060934749 ) ) ;
#46319=VERTEX_POINT ( 'NONE', #35744 ) ;
#46321=CARTESIAN_POINT ( 'NONE',  ( -18.55957040452605611, -7.446158924837727788, 74.02559677774105751 ) ) ;
#46322=CARTESIAN_POINT ( 'NONE',  ( -10.35879128504702251, -12.44577124159657089, 60.97666315383261804 ) ) ;
#46323=EDGE_LOOP ( 'NONE', ( #10790, #34129 ) ) ;
#46324=CARTESIAN_POINT ( 'NONE',  ( -15.81235419205221859, -7.945607373518419614, 67.42535135806457447 ) ) ;
#46325=FACE_OUTER_BOUND ( 'NONE', #38310, .T. ) ;
#46329=CARTESIAN_POINT ( 'NONE',  ( -23.54569140518488624, -19.05536029250058050, 65.93894040291287695 ) ) ;
#46330=DIRECTION ( 'NONE',  ( -0.9163203205182084421, -0.4004460890125009498, 2.380681625734479923E-09 ) ) ;
#46332=CARTESIAN_POINT ( 'NONE',  ( -22.33376602745314798, -19.86903051493497685, 69.18890041286789483 ) ) ;
#46333=CARTESIAN_POINT ( 'NONE',  ( -21.00380318978402627, -21.34292366101719196, 62.22975991904223747 ) ) ;
#46334=CARTESIAN_POINT ( 'NONE',  ( -23.13305522301093120, -10.65917872773856878, 63.21619042434998903 ) ) ;
#46335=CARTESIAN_POINT ( 'NONE',  ( -12.52591726580351228, -9.195683270288645517, 74.50418291613799227 ) ) ;
#46336=CARTESIAN_POINT ( 'NONE',  ( -21.38734882604794407, -9.039157345192338155, 70.35805789912156172 ) ) ;
#46337=ORIENTED_EDGE ( 'NONE', *, *, #23804, .T. ) ;
#46338=ORIENTED_EDGE ( 'NONE', *, *, #19691, .T. ) ;
#46340=ORIENTED_EDGE ( 'NONE', *, *, #17763, .F. ) ;
#46341=DIRECTION ( 'NONE',  ( 1.352396030810764649E-06, 5.694414615768204918E-07, 0.9999999999989234167 ) ) ;
#46343=CARTESIAN_POINT ( 'NONE',  ( -19.85891393954322837, -21.37210614461000446, 47.99999999999994316 ) ) ;
#46345=EDGE_CURVE ( 'NONE', #34499, #24622, #23939, .T. ) ;
#46347=AXIS2_PLACEMENT_3D ( 'NONE', #40430, #48540, #34006 ) ;
#46349=CARTESIAN_POINT ( 'NONE',  ( -21.41781370759021641, -8.989828079956971862, 66.81716936885602820 ) ) ;
#46350=CARTESIAN_POINT ( 'NONE',  ( -10.37878816232847967, -14.54793763971057174, 68.15240352950337410 ) ) ;
#46351=ORIENTED_EDGE ( 'NONE', *, *, #1495, .T. ) ;
#46352=CARTESIAN_POINT ( 'NONE',  ( -20.88821433888680446, -8.213514021607622340, 60.03399393531998385 ) ) ;
#46353=CARTESIAN_POINT ( 'NONE',  ( -23.82261072958198511, -17.64831273128667632, 62.47360983446513671 ) ) ;
#46354=ORIENTED_EDGE ( 'NONE', *, *, #8676, .F. ) ;
#46355=CARTESIAN_POINT ( 'NONE',  ( -19.90583630033073703, -21.83377919204098205, 69.19128392610542733 ) ) ;
#46356=CARTESIAN_POINT ( 'NONE',  ( -23.67397131994236759, -11.53905716532417536, 70.19210929491518414 ) ) ;
#46357=ORIENTED_EDGE ( 'NONE', *, *, #22764, .F. ) ;
#46358=CARTESIAN_POINT ( 'NONE',  ( -16.13263948075386978, -7.878200451182638453, 63.68483172840383588 ) ) ;
#46359=CARTESIAN_POINT ( 'NONE',  ( -22.23155801786484176, -20.50065754255900075, 58.88630131417564684 ) ) ;
#46360=CARTESIAN_POINT ( 'NONE',  ( -10.41531639268335496, -14.04517892474411589, 60.93293405735092705 ) ) ;
#46361=VERTEX_POINT ( 'NONE', #5013 ) ;
#46365=EDGE_CURVE ( 'NONE', #25227, #34833, #1473, .T. ) ;
#46366=CARTESIAN_POINT ( 'NONE',  ( -11.55140690636466339, -10.22489917031350970, 71.09080336155108171 ) ) ;
#46368=DIRECTION ( 'NONE',  ( -5.731567514496413899E-31, -1.020425574103664789E-16, -1.000000000000000000 ) ) ;
#46370=FACE_OUTER_BOUND ( 'NONE', #11045, .T. ) ;
#46372=EDGE_CURVE ( 'NONE', #15929, #6697, #46849, .T. ) ;
#46375=EDGE_LOOP ( 'NONE', ( #20613, #4467 ) ) ;
#46378=CYLINDRICAL_SURFACE ( 'NONE', #31266, 0.1500000000000052125 ) ;
#46379=ORIENTED_EDGE ( 'NONE', *, *, #11285, .F. ) ;
#46382=CARTESIAN_POINT ( 'NONE',  ( -10.40888601095206134, -14.10966482229656194, 61.21821293885882653 ) ) ;
#46384=CARTESIAN_POINT ( 'NONE',  ( -14.62324732345129341, -21.22583884561250400, 58.23788065448412965 ) ) ;
#46385=EDGE_CURVE ( 'NONE', #41672, #5421, #1600, .T. ) ;
#46386=ORIENTED_EDGE ( 'NONE', *, *, #47511, .T. ) ;
#46387=CARTESIAN_POINT ( 'NONE',  ( -24.80769062643263467, -15.80232089486973557, 69.71802876059763321 ) ) ;
#46389=CARTESIAN_POINT ( 'NONE',  ( -11.21157534608376061, -11.58358818987947814, 67.91864608155252370 ) ) ;
#46390=CARTESIAN_POINT ( 'NONE',  ( -19.02448764833726713, -7.994547592594012819, 63.44591627019872959 ) ) ;
#46391=VERTEX_POINT ( 'NONE', #1792 ) ;
#46392=CARTESIAN_POINT ( 'NONE',  ( -18.59868636808265663, -22.16608242820997887, 72.47785073958938540 ) ) ;
#46399=ORIENTED_EDGE ( 'NONE', *, *, #15889, .F. ) ;
#46401=CARTESIAN_POINT ( 'NONE',  ( -20.89788161767221197, -20.94431024770144489, 62.39999296070408974 ) ) ;
#46402=AXIS2_PLACEMENT_3D ( 'NONE', #30758, #42070, #45535 ) ;
#46404=CARTESIAN_POINT ( 'NONE',  ( -19.99112905230247961, -8.296885111154901793, 73.72096600045514947 ) ) ;
#46405=ADVANCED_FACE ( 'NONE', ( #47346 ), #13574, .T. ) ;
#46406=CARTESIAN_POINT ( 'NONE',  ( -24.12071557656922494, -11.54438865435207795, 63.06722852297808402 ) ) ;
#46407=CARTESIAN_POINT ( 'NONE',  ( -24.31285881818529404, -17.64644613426892406, 66.08323844663713942 ) ) ;
#46409=CIRCLE ( 'NONE', #29100, 5.500000000000000000 ) ;
#46410=PLANE ( 'NONE',  #22912 ) ;
#46411=VECTOR ( 'NONE', #11644, 1000.000000000000114 ) ;
#46412=CARTESIAN_POINT ( 'NONE',  ( -24.41841346439724347, -17.37497344050957437, 69.45693887357894880 ) ) ;
#46413=VERTEX_POINT ( 'NONE', #8948 ) ;
#46414=( BOUNDED_CURVE ( )  B_SPLINE_CURVE ( 3, ( #42732, #42243, #16106, #8999 ),
 .UNSPECIFIED., .F., .F. ) 
 B_SPLINE_CURVE_WITH_KNOTS ( ( 4, 4 ),
 ( 0.9074455897393669535, 1.000000000000000000 ),
 .UNSPECIFIED. ) 
 CURVE ( )  GEOMETRIC_REPRESENTATION_ITEM ( )  RATIONAL_B_SPLINE_CURVE ( ( 0.6983129098260874024, 0.7760317562606933173, 0.8765941196519975165, 1.000000000000000000 ) ) 
 REPRESENTATION_ITEM ( '' )  );
#46415=CARTESIAN_POINT ( 'NONE',  ( -21.31800817620502286, -20.62620158190326336, 72.82446429882371319 ) ) ;
#46416=EDGE_CURVE ( 'NONE', #17241, #2873, #14461, .T. ) ;
#46419=FACE_OUTER_BOUND ( 'NONE', #25741, .T. ) ;
#46420=LINE ( 'NONE', #38528, #3768 ) ;
#46421=ORIENTED_EDGE ( 'NONE', *, *, #45220, .F. ) ;
#46422=CARTESIAN_POINT ( 'NONE',  ( -13.90356134367569041, -20.91730929552939600, 68.75625110435674969 ) ) ;
#46423=CARTESIAN_POINT ( 'NONE',  ( -10.00684590941331820, -15.50754077729470559, 57.67454502885500034 ) ) ;
#46425=CARTESIAN_POINT ( 'NONE',  ( -21.47456293661849713, -9.038556783377254433, 70.41660404402310292 ) ) ;
#46426=CARTESIAN_POINT ( 'NONE',  ( -24.49056774983930751, -17.16914905338390085, 73.06052939366072962 ) ) ;
#46428=CARTESIAN_POINT ( 'NONE',  ( -10.32823143149344247, -17.07887373198904513, 57.78736918859686966 ) ) ;
#46431=( BOUNDED_CURVE ( )  B_SPLINE_CURVE ( 3, ( #13024, #46295, #24376, #34950 ),
 .UNSPECIFIED., .F., .F. ) 
 B_SPLINE_CURVE_WITH_KNOTS ( ( 4, 4 ),
 ( 0.5000000000000000000, 0.9074455897393624015 ),
 .UNSPECIFIED. ) 
 CURVE ( )  GEOMETRIC_REPRESENTATION_ITEM ( )  RATIONAL_B_SPLINE_CURVE ( ( 1.000000000000003109, 0.4567392136813368531, 0.3561768502900296562, 0.6983129098260851819 ) ) 
 REPRESENTATION_ITEM ( '' )  );
#46432=CARTESIAN_POINT ( 'NONE',  ( -10.99586697244644640, -11.04334986774487781, 60.86381167495338929 ) ) ;
#46433=EDGE_CURVE ( 'NONE', #42239, #11354, #43221, .T. ) ;
#46434=CARTESIAN_POINT ( 'NONE',  ( -22.79734409636068904, -10.24514240368273477, 66.54182257473807738 ) ) ;
#46435=CARTESIAN_POINT ( 'NONE',  ( -17.73278501768472992, -7.757988417614677168, 67.16472282884072342 ) ) ;
#46436=CYLINDRICAL_SURFACE ( 'NONE', #6203, 0.1499999999999974132 ) ;
#46437=VERTEX_POINT ( 'NONE', #24457 ) ;
#46439=ADVANCED_FACE ( 'NONE', ( #24923 ), #48528, .T. ) ;
#46440=ORIENTED_EDGE ( 'NONE', *, *, #18264, .T. ) ;
#46441=CARTESIAN_POINT ( 'NONE',  ( -11.45751978572037011, -19.27057081285444085, 71.87181161472111057 ) ) ;
#46442=CARTESIAN_POINT ( 'NONE',  ( -13.14998806103231566, -9.265559761403904915, 67.67942786032521951 ) ) ;
#46444=DIRECTION ( 'NONE',  ( 0.9163203205182083311, 0.4004460890125009498, -2.380681616944615543E-09 ) ) ;
#46445=CARTESIAN_POINT ( 'NONE',  ( -12.70413878835906729, -9.045123344351514660, 71.04914126506433547 ) ) ;
#46448=VERTEX_POINT ( 'NONE', #40418 ) ;
#46450=CARTESIAN_POINT ( 'NONE',  ( -10.03035355355731006, -15.72374577095404824, 61.22284339518546403 ) ) ;
#46452=CARTESIAN_POINT ( 'NONE',  ( -21.94239175829699207, -20.22099772874085488, 59.06442899522711798 ) ) ;
#46453=EDGE_CURVE ( 'NONE', #4771, #956, #30403, .T. ) ;
#46455=B_SPLINE_CURVE_WITH_KNOTS ( 'NONE', 3,
 ( #7540, #45218, #48158, #41256, #14390, #44479, #22548, #37543, #3845, #10730 ),
 .UNSPECIFIED., .F., .F.,
 ( 4, 2, 2, 2, 4 ),
 ( 0.1272669073657964056, 0.2522669073487617819, 0.3772669073317270749, 0.5022669073146924790, 0.6272669072976577720 ),
 .UNSPECIFIED. ) ;
#46456=CARTESIAN_POINT ( 'NONE',  ( -10.70785606720758487, -16.78775419186948881, 57.79833654845999291 ) ) ;
#46457=AXIS2_PLACEMENT_3D ( 'NONE', #38248, #4530, #34566 ) ;
#46460=ORIENTED_EDGE ( 'NONE', *, *, #39737, .F. ) ;
#46464=CARTESIAN_POINT ( 'NONE',  ( -11.39127492490111315, -11.16067319722467843, 60.69357916181100876 ) ) ;
#46466=AXIS2_PLACEMENT_3D ( 'NONE', #30241, #41549, #8545 ) ;
#46467=CARTESIAN_POINT ( 'NONE',  ( -23.27053873564116770, -18.65887406133006010, 66.05062667540605048 ) ) ;
#46469=ORIENTED_EDGE ( 'NONE', *, *, #30646, .F. ) ;
#46470=DIRECTION ( 'NONE',  ( 0.2122660683108583690, -0.9772119095896469876, 7.504255179194988334E-08 ) ) ;
#46473=B_SPLINE_CURVE_WITH_KNOTS ( 'NONE', 3,
 ( #33319, #32846, #24997, #2816, #48126, #25965, #33079, #29655, #44691, #3057 ),
 .UNSPECIFIED., .F., .F.,
 ( 4, 2, 2, 2, 4 ),
 ( 0.1272669073658475869, 0.2522669073463348899, 0.3772669073268222206, 0.5022669073073094959, 0.6272669072877967711 ),
 .UNSPECIFIED. ) ;
#46474=DIRECTION ( 'NONE',  ( -0.3478314405900341799, -0.9375570856950852239, 0.000000000000000000 ) ) ;
#46475=ORIENTED_EDGE ( 'NONE', *, *, #17610, .F. ) ;
#46477=B_SPLINE_CURVE_WITH_KNOTS ( 'NONE', 1,
 ( #38302, #26037 ),
 .UNSPECIFIED., .F., .F.,
 ( 2, 2 ),
 ( 0.000000000000000000, 1.000000000000000000 ),
 .UNSPECIFIED. ) ;
#46478=AXIS2_PLACEMENT_3D ( 'NONE', #12469, #34873, #15914 ) ;
#46479=CARTESIAN_POINT ( 'NONE',  ( -10.40121522062585591, -17.29573862802152817, 61.20097198354311274 ) ) ;
#46480=CARTESIAN_POINT ( 'NONE',  ( -22.11331555132107241, -9.020036405104091770, 63.29879605510286922 ) ) ;
#46481=CARTESIAN_POINT ( 'NONE',  ( -24.17580812652340683, -11.65980397366943855, 59.65952650191913875 ) ) ;
#46484=DIRECTION ( 'NONE',  ( -5.731567514496413899E-31, -1.020425574103664789E-16, -1.000000000000000000 ) ) ;
#46485=CARTESIAN_POINT ( 'NONE',  ( -24.82755346431643417, -15.64070656656598857, 73.20314952539401077 ) ) ;
#46486=CARTESIAN_POINT ( 'NONE',  ( -11.44812054352227193, -18.45465371200965166, 61.27710877960604563 ) ) ;
#46487=EDGE_LOOP ( 'NONE', ( #6833, #36109 ) ) ;
#46488=CARTESIAN_POINT ( 'NONE',  ( -10.00731251637046881, -14.10555026099538978, 61.10316585833331260 ) ) ;
#46490=ORIENTED_EDGE ( 'NONE', *, *, #13647, .T. ) ;
#46492=FACE_OUTER_BOUND ( 'NONE', #3530, .T. ) ;
#46493=ORIENTED_EDGE ( 'NONE', *, *, #2846, .T. ) ;
#46494=EDGE_CURVE ( 'NONE', #23020, #18740, #39791, .T. ) ;
#46496=CARTESIAN_POINT ( 'NONE',  ( -10.37762151648083808, -12.38827872426728050, 57.44202070861023657 ) ) ;
#46497=CARTESIAN_POINT ( 'NONE',  ( -24.25757915753366589, -13.28409016433970535, 63.02191351886040138 ) ) ;
#46499=ORIENTED_EDGE ( 'NONE', *, *, #42074, .F. ) ;
#46502=DIRECTION ( 'NONE',  ( 0.8402231219892249969, -0.5322911103758141138, 0.1033986416233923511 ) ) ;
#46503=CARTESIAN_POINT ( 'NONE',  ( -23.42121016340660233, -19.22949192118923989, 62.53219661271650409 ) ) ;
#46504=VERTEX_POINT ( 'NONE', #10148 ) ;
#46506=CARTESIAN_POINT ( 'NONE',  ( -11.14144638094932382, -18.81445342923831987, 61.39055447797494480 ) ) ;
#46508=ORIENTED_EDGE ( 'NONE', *, *, #19567, .F. ) ;
#46509=ORIENTED_EDGE ( 'NONE', *, *, #25593, .F. ) ;
#46510=CARTESIAN_POINT ( 'NONE',  ( -23.83080496556880945, -17.75212211224490133, 59.28906343887996400 ) ) ;
#46511=CARTESIAN_POINT ( 'NONE',  ( -13.07136565370527315, -8.762923774744256988, 64.02451247989536398 ) ) ;
#46515=CARTESIAN_POINT ( 'NONE',  ( -12.35435101773841993, -9.982347803354048921, 57.31608956411530187 ) ) ;
#46516=B_SPLINE_CURVE_WITH_KNOTS ( 'NONE', 3,
 ( #39340, #46967, #47696, #14174, #40314, #44501, #6818, #28745, #6090, #28509 ),
 .UNSPECIFIED., .F., .F.,
 ( 4, 2, 2, 2, 4 ),
 ( 0.6272669072877915530, 0.7522669073073021684, 0.8772669073268128948, 1.002266907346323510, 1.127266907365834125 ),
 .UNSPECIFIED. ) ;
#46517=CARTESIAN_POINT ( 'NONE',  ( -19.72726371358324471, -21.89426820971140941, 65.56511966726597507 ) ) ;
#46519=CARTESIAN_POINT ( 'NONE',  ( -23.25646303129147441, -19.44570675813884009, 59.07065992548621125 ) ) ;
#46520=ORIENTED_EDGE ( 'NONE', *, *, #35920, .T. ) ;
#46521=ORIENTED_EDGE ( 'NONE', *, *, #41812, .T. ) ;
#46522=VECTOR ( 'NONE', #41614, 1000.000000000000227 ) ;
#46523=EDGE_CURVE ( 'NONE', #37668, #46893, #14046, .T. ) ;
#46528=LINE ( 'NONE', #9336, #45308 ) ;
#46529=CARTESIAN_POINT ( 'NONE',  ( -21.84435842615539158, -9.381383662134735957, 59.83057260011872103 ) ) ;
#46530=AXIS2_PLACEMENT_3D ( 'NONE', #27448, #5547, #35068 ) ;
#46532=VERTEX_POINT ( 'NONE', #25637 ) ;
#46533=CARTESIAN_POINT ( 'NONE',  ( -11.96084830514426400, -9.743959610980004626, 60.74413522332266524 ) ) ;
#46534=CARTESIAN_POINT ( 'NONE',  ( -12.96755856236231885, -20.27663165334763917, 72.01473639041756769 ) ) ;
#46535=B_SPLINE_CURVE_WITH_KNOTS ( 'NONE', 1,
 ( #14254, #7645 ),
 .UNSPECIFIED., .F., .F.,
 ( 2, 2 ),
 ( 0.000000000000000000, 1.000000000000000000 ),
 .UNSPECIFIED. ) ;
#46536=CARTESIAN_POINT ( 'NONE',  ( -22.00117057250496444, -9.443090202341716477, 63.60642510345682155 ) ) ;
#46539=ORIENTED_EDGE ( 'NONE', *, *, #43117, .F. ) ;
#46540=CARTESIAN_POINT ( 'NONE',  ( -10.54357723031444216, -16.09736363853215479, 68.26302419364235163 ) ) ;
#46541=CARTESIAN_POINT ( 'NONE',  ( -24.02329229792678689, -17.28986148198579187, 69.41339790474248161 ) ) ;
#46542=EDGE_CURVE ( 'NONE', #32302, #11500, #29772, .T. ) ;
#46544=VERTEX_POINT ( 'NONE', #29836 ) ;
#46545=CARTESIAN_POINT ( 'NONE',  ( -22.62539314545485780, -20.14320100466526497, 69.31384596586300972 ) ) ;
#46546=CARTESIAN_POINT ( 'NONE',  ( -24.22220026926100545, -16.48362040234153625, 59.35162391529105008 ) ) ;
#46548=B_SPLINE_CURVE_WITH_KNOTS ( 'NONE', 3,
 ( #40398, #28365, #39917, #25617, #2246, #6187, #10125, #47071, #2495, #25148 ),
 .UNSPECIFIED., .F., .F.,
 ( 4, 2, 2, 2, 4 ),
 ( 0.000000000000000000, 0.2500000000000000000, 0.5000000000000000000, 0.7500000000000000000, 1.000000000000000000 ),
 .UNSPECIFIED. ) ;
#46550=ORIENTED_EDGE ( 'NONE', *, *, #24708, .F. ) ;
#46552=VECTOR ( 'NONE', #37282, 1000.000000000000114 ) ;
#46553=CARTESIAN_POINT ( 'NONE',  ( -17.43166586245951422, -7.359124596637800053, 67.13544155391683432 ) ) ;
#46554=VERTEX_POINT ( 'NONE', #45600 ) ;
#46555=CARTESIAN_POINT ( 'NONE',  ( -10.69843886630479624, -16.92312086968962603, 57.68760564129097901 ) ) ;
#46557=ORIENTED_EDGE ( 'NONE', *, *, #36111, .F. ) ;
#46558=CARTESIAN_POINT ( 'NONE',  ( -17.86643106983121498, -7.822757629381109190, 60.36444193307492156 ) ) ;
#46559=( BOUNDED_SURFACE ( )  B_SPLINE_SURFACE ( 3, 1, ( 
 ( #38516, #15612 ),
 ( #11949, #41982 ),
 ( #860, #4542 ),
 ( #12181, #27198 ),
 ( #42223, #23516 ),
 ( #38761, #4798 ),
 ( #19823, #34819 ) ),
 .UNSPECIFIED., .T., .F., .F. ) 
 B_SPLINE_SURFACE_WITH_KNOTS ( ( 4, 3, 4 ),
 ( 2, 2 ),
 ( 0.000000000000000000, 0.5000000000000000000, 1.000000000000000000 ),
 ( 0.000000000000000000, 1.000000000000000000 ),
 .UNSPECIFIED. ) 
 GEOMETRIC_REPRESENTATION_ITEM ( )  RATIONAL_B_SPLINE_SURFACE ( (
 ( 1.000000000000000000, 1.000000000000000000),
 ( 0.3333333333333335369, 0.3333333333333330373),
 ( 0.3333333333333335369, 0.3333333333333330373),
 ( 1.000000000000000000, 1.000000000000000000),
 ( 0.3333333333333333703, 0.3333333333333333703),
 ( 0.3333333333333333703, 0.3333333333333333703),
 ( 1.000000000000000000, 1.000000000000000000) ) ) 
 REPRESENTATION_ITEM ( '' )  SURFACE ( )  );
#46560=CARTESIAN_POINT ( 'NONE',  ( -15.28630342961327138, -8.082779564739171363, 56.99432743296591042 ) ) ;
#46561=DIRECTION ( 'NONE',  ( -5.731567514496413899E-31, -1.020425574103664789E-16, -1.000000000000000000 ) ) ;
#46562=EDGE_LOOP ( 'NONE', ( #35555, #1972, #36676, #3023, #18418 ) ) ;
#46563=CARTESIAN_POINT ( 'NONE',  ( -21.53861794036900079, -21.02004141303368101, 72.63951040967180006 ) ) ;
#46564=CARTESIAN_POINT ( 'NONE',  ( -10.29385348138020539, -12.64970417265235803, 64.38340698725603772 ) ) ;
#46565=CARTESIAN_POINT ( 'NONE',  ( -11.73296596577226936, -10.64774513788296417, 74.72412863062541533 ) ) ;
#46567=CARTESIAN_POINT ( 'NONE',  ( -12.46122051107220408, -19.81685944811288991, 64.88146935704573082 ) ) ;
#46568=ORIENTED_EDGE ( 'NONE', *, *, #27071, .T. ) ;
#46570=CARTESIAN_POINT ( 'NONE',  ( -20.54979492810923603, -8.489990406890694175, 63.46121512946601229 ) ) ;
#46571=CARTESIAN_POINT ( 'NONE',  ( -24.28086713618749570, -13.15448386353826926, 66.39426969126174072 ) ) ;
#46572=ORIENTED_EDGE ( 'NONE', *, *, #36498, .F. ) ;
#46573=CARTESIAN_POINT ( 'NONE',  ( -10.40860991809309155, -15.50898095412354571, 57.85320721669017985 ) ) ;
#46574=CARTESIAN_POINT ( 'NONE',  ( -19.41474593944376537, -21.52019035999878938, 61.99503644832097393 ) ) ;
#46576=CARTESIAN_POINT ( 'NONE',  ( -13.08279692198261479, -8.754610786518940202, 64.07093076773905693 ) ) ;
#46577=CARTESIAN_POINT ( 'NONE',  ( -11.22844613476422282, -11.44458948612160221, 64.43409918096024569 ) ) ;
#46578=( BOUNDED_CURVE ( )  B_SPLINE_CURVE ( 3, ( #19109, #173, #639, #45466 ),
 .UNSPECIFIED., .F., .F. ) 
 B_SPLINE_CURVE_WITH_KNOTS ( ( 4, 4 ),
 ( 4.712388980384689674, 4.921828490624010399 ),
 .UNSPECIFIED. ) 
 CURVE ( )  GEOMETRIC_REPRESENTATION_ITEM ( )  RATIONAL_B_SPLINE_CURVE ( ( 1.000000000000000000, 0.9963479302455154896, 0.9963479302455154896, 1.000000000000000000 ) ) 
 REPRESENTATION_ITEM ( '' )  );
#46579=EDGE_LOOP ( 'NONE', ( #28176, #17598, #45958, #42548, #17374 ) ) ;
#46580=EDGE_CURVE ( 'NONE', #42076, #28542, #41553, .T. ) ;
#46581=CARTESIAN_POINT ( 'NONE',  ( -19.17403394478084522, -7.567564808342563509, 63.47443287871421091 ) ) ;
#46582=LINE ( 'NONE', #9389, #44420 ) ;
#46583=CARTESIAN_POINT ( 'NONE',  ( -22.85860156586533165, -9.713020250643273457, 73.64307581635257804 ) ) ;
#46584=CARTESIAN_POINT ( 'NONE',  ( -12.10131192688100477, -10.18592936015514638, 64.31442259820508411 ) ) ;
#46585=VERTEX_POINT ( 'NONE', #41389 ) ;
#46586=ORIENTED_EDGE ( 'NONE', *, *, #2872, .F. ) ;
#46587=( BOUNDED_SURFACE ( )  B_SPLINE_SURFACE ( 3, 1, ( 
 ( #17800, #32825 ),
 ( #47863, #29147 ),
 ( #44197, #25455 ),
 ( #7243, #22246 ),
 ( #6983, #331 ),
 ( #7731, #34282 ),
 ( #37000, #37735 ) ),
 .UNSPECIFIED., .T., .F., .F. ) 
 B_SPLINE_SURFACE_WITH_KNOTS ( ( 4, 3, 4 ),
 ( 2, 2 ),
 ( 0.000000000000000000, 0.5000000000000000000, 1.000000000000000000 ),
 ( 0.000000000000000000, 1.000000000000000000 ),
 .UNSPECIFIED. ) 
 GEOMETRIC_REPRESENTATION_ITEM ( )  RATIONAL_B_SPLINE_SURFACE ( (
 ( 1.000000000000000000, 1.000000000000000000),
 ( 0.3333333333333335369, 0.3333333333333330373),
 ( 0.3333333333333335369, 0.3333333333333330373),
 ( 1.000000000000000000, 1.000000000000000000),
 ( 0.3333333333333333703, 0.3333333333333333703),
 ( 0.3333333333333333703, 0.3333333333333333703),
 ( 1.000000000000000000, 1.000000000000000000) ) ) 
 REPRESENTATION_ITEM ( '' )  SURFACE ( )  );
#46590=VERTEX_POINT ( 'NONE', #18735 ) ;
#46593=DIRECTION ( 'NONE',  ( -5.731567514496413899E-31, -1.020425574103664789E-16, -1.000000000000000000 ) ) ;
#46595=ORIENTED_EDGE ( 'NONE', *, *, #40163, .F. ) ;
#46596=CARTESIAN_POINT ( 'NONE',  ( -21.84891708756835982, -9.316868653145983004, 67.07638807817237137 ) ) ;
#46598=EDGE_CURVE ( 'NONE', #28666, #6771, #40, .T. ) ;
#46600=CARTESIAN_POINT ( 'NONE',  ( -23.12302852889638061, -18.95946475466559633, 62.65406880579606508 ) ) ;
#46601=CARTESIAN_POINT ( 'NONE',  ( -19.37616744185158879, -21.99900390342548206, 58.71002665166666645 ) ) ;
#46603=CARTESIAN_POINT ( 'NONE',  ( -11.37640567311080453, -11.28103864939108902, 64.33809173091806599 ) ) ;
#46604=ORIENTED_EDGE ( 'NONE', *, *, #11375, .T. ) ;
#46605=CARTESIAN_POINT ( 'NONE',  ( -10.58039871790519726, -13.33820790931908284, 71.39931681139518105 ) ) ;
#46606=ORIENTED_EDGE ( 'NONE', *, *, #31582, .F. ) ;
#46607=CARTESIAN_POINT ( 'NONE',  ( -24.43113015230203544, -15.58634353390661964, 73.15303748141660378 ) ) ;
#46608=CARTESIAN_POINT ( 'NONE',  ( -16.85302834907681557, -22.23803867529147738, 68.80905311428833215 ) ) ;
#46609=CARTESIAN_POINT ( 'NONE',  ( -20.84119746710918974, -20.97572115929791892, 62.11471400470772863 ) ) ;
#46611=CARTESIAN_POINT ( 'NONE',  ( -24.23636277187043220, -17.82529184948975498, 62.58865552117998021 ) ) ;
#46612=CARTESIAN_POINT ( 'NONE',  ( -24.42218830512229388, -14.64588455312011739, 63.01296487252135137 ) ) ;
#46613=CARTESIAN_POINT ( 'NONE',  ( -24.08281607949275127, -11.46758912624300919, 63.09071781931947953 ) ) ;
#46614=CARTESIAN_POINT ( 'NONE',  ( -10.46375287308303648, -15.55739392218797512, 61.05405700252866552 ) ) ;
#46615=CARTESIAN_POINT ( 'NONE',  ( -20.64396844604977233, -21.02470390210128670, 58.64475165022597025 ) ) ;
#46616=ORIENTED_EDGE ( 'NONE', *, *, #30362, .F. ) ;
#46617=CARTESIAN_POINT ( 'NONE',  ( -17.45675080712947036, -7.809221453984609873, 63.77730436730185914 ) ) ;
#46618=CARTESIAN_POINT ( 'NONE',  ( -11.68775437312510235, -10.05546324315060858, 67.54250946422081370 ) ) ;
#46620=CARTESIAN_POINT ( 'NONE',  ( -14.54749350918766204, -8.372447261038935551, 64.07506791522041567 ) ) ;
#46621=CARTESIAN_POINT ( 'NONE',  ( -19.97822118923243195, -21.80783213648190610, 69.05669729689820713 ) ) ;
#46624=PLANE ( 'NONE',  #27470 ) ;
#46627=FACE_OUTER_BOUND ( 'NONE', #40400, .T. ) ;
#46629=CARTESIAN_POINT ( 'NONE',  ( -17.92307556733882379, -22.24252716037962330, 62.06874222216396220 ) ) ;
#46632=ADVANCED_FACE ( 'NONE', ( #37689 ), #45509, .T. ) ;
#46633=ORIENTED_EDGE ( 'NONE', *, *, #22565, .F. ) ;
#46634=CARTESIAN_POINT ( 'NONE',  ( -24.80967279009360027, -15.78810072853396917, 69.69340815245216447 ) ) ;
#46635=DIRECTION ( 'NONE',  ( 0.5022914217388751990, -0.8646984027090225400, -6.766381832589513682E-08 ) ) ;
#46636=CARTESIAN_POINT ( 'NONE',  ( -19.02482722938969317, -7.994625824363213340, 63.71623835456152563 ) ) ;
#46637=EDGE_CURVE ( 'NONE', #39973, #22327, #40814, .T. ) ;
#46638=ORIENTED_EDGE ( 'NONE', *, *, #11941, .T. ) ;
#46639=CARTESIAN_POINT ( 'NONE',  ( -16.86460949297358525, -7.773444642497263857, 70.64603134899243742 ) ) ;
#46640=CARTESIAN_POINT ( 'NONE',  ( -23.49719359612965519, -11.32496190889342813, 73.55120448430523084 ) ) ;
#46642=CARTESIAN_POINT ( 'NONE',  ( -15.68875476689939852, -7.563362019294005201, 70.79645224690898431 ) ) ;
#46643=CARTESIAN_POINT ( 'NONE',  ( -14.67111564601650997, -7.886426081561471513, 60.43500846974642116 ) ) ;
#46644=EDGE_LOOP ( 'NONE', ( #4133, #8874 ) ) ;
#46645=EDGE_LOOP ( 'NONE', ( #41066, #37531 ) ) ;
#46647=CARTESIAN_POINT ( 'NONE',  ( -23.07906183844443859, -9.958936969296642516, 66.72677665813928627 ) ) ;
#46648=VECTOR ( 'NONE', #24512, 1000.000000000000227 ) ;
#46650=CARTESIAN_POINT ( 'NONE',  ( -20.64396844604977233, -21.02470390210128670, 58.64475165022597025 ) ) ;
#46652=CARTESIAN_POINT ( 'NONE',  ( -11.45751978572037011, -19.27057081285444085, 71.87181161472111057 ) ) ;
#46653=EDGE_CURVE ( 'NONE', #42260, #16178, #20960, .T. ) ;
#46654=CARTESIAN_POINT ( 'NONE',  ( -24.45013009618349642, -14.22792902121458170, 69.95275266250405366 ) ) ;
#46655=CARTESIAN_POINT ( 'NONE',  ( -24.32775969560190177, -17.60956452435454622, 66.14368435521323875 ) ) ;
#46656=CARTESIAN_POINT ( 'NONE',  ( -24.05420634179087358, -17.20676946999824608, 69.69867738674849988 ) ) ;
#46658=ORIENTED_EDGE ( 'NONE', *, *, #10435, .T. ) ;
#46661=CARTESIAN_POINT ( 'NONE',  ( -10.35650339757981442, -17.16777133705972602, 57.80105215977741295 ) ) ;
#46663=ORIENTED_EDGE ( 'NONE', *, *, #22545, .T. ) ;
#46664=CARTESIAN_POINT ( 'NONE',  ( -17.79108452803360763, -21.84994637594637723, 58.69081321602850920 ) ) ;
#46665=CARTESIAN_POINT ( 'NONE',  ( -24.65877048445197417, -13.03101829210932827, 62.98264174300280160 ) ) ;
#46675=DIRECTION ( 'NONE',  ( -0.9000732436326449593, -0.4357386327795698122, 2.072980810273451456E-08 ) ) ;
#46676=ORIENTED_EDGE ( 'NONE', *, *, #32853, .F. ) ;
#46677=CARTESIAN_POINT ( 'NONE',  ( -21.15336504700141163, -20.73310185707507713, 69.05450185101547333 ) ) ;
#46678=FACE_OUTER_BOUND ( 'NONE', #37050, .T. ) ;
#46679=CARTESIAN_POINT ( 'NONE',  ( -12.46122051107220230, -19.81685944811288635, 64.88146935704573082 ) ) ;
#46681=ORIENTED_EDGE ( 'NONE', *, *, #38911, .T. ) ;
#46682=LINE ( 'NONE', #27719, #13661 ) ;
#46683=FACE_BOUND ( 'NONE', #7618, .T. ) ;
#46684=ORIENTED_EDGE ( 'NONE', *, *, #15150, .F. ) ;
#46685=ORIENTED_EDGE ( 'NONE', *, *, #37769, .F. ) ;
#46689=CARTESIAN_POINT ( 'NONE',  ( -12.88340866885723912, -8.902872279917016130, 67.57953991358206736 ) ) ;
#46690=( BOUNDED_SURFACE ( )  B_SPLINE_SURFACE ( 3, 1, ( 
 ( #6934, #14292 ),
 ( #2987, #21953 ),
 ( #3475, #36692 ),
 ( #33490, #40189 ),
 ( #48531, #10631 ),
 ( #6462, #44613 ),
 ( #9910, #44152 ) ),
 .UNSPECIFIED., .T., .F., .F. ) 
 B_SPLINE_SURFACE_WITH_KNOTS ( ( 4, 3, 4 ),
 ( 2, 2 ),
 ( 0.000000000000000000, 0.5000000000000000000, 1.000000000000000000 ),
 ( 0.000000000000000000, 1.000000000000000000 ),
 .UNSPECIFIED. ) 
 GEOMETRIC_REPRESENTATION_ITEM ( )  RATIONAL_B_SPLINE_SURFACE ( (
 ( 1.000000000000000000, 1.000000000000000000),
 ( 0.3333333333333335369, 0.3333333333333330373),
 ( 0.3333333333333335369, 0.3333333333333330373),
 ( 1.000000000000000000, 1.000000000000000000),
 ( 0.3333333333333333703, 0.3333333333333333703),
 ( 0.3333333333333333703, 0.3333333333333333703),
 ( 1.000000000000000000, 1.000000000000000000) ) ) 
 REPRESENTATION_ITEM ( '' )  SURFACE ( )  );
#46692=CARTESIAN_POINT ( 'NONE',  ( -13.79205357149631084, -8.762576837000361607, 57.06148030867162646 ) ) ;
#46693=CARTESIAN_POINT ( 'NONE',  ( -22.66727051383977809, -10.09628829486277546, 70.31178520457007153 ) ) ;
#46694=ORIENTED_EDGE ( 'NONE', *, *, #6492, .F. ) ;
#46695=ORIENTED_EDGE ( 'NONE', *, *, #36550, .T. ) ;
#46697=B_SPLINE_CURVE_WITH_KNOTS ( 'NONE', 3,
 ( #42346, #34940, #1208, #16212, #5163, #46285, #12538, #14212, #37860, #37355 ),
 .UNSPECIFIED., .F., .F.,
 ( 4, 2, 2, 2, 4 ),
 ( 0.1272669073658217465, 0.2522669073463153500, 0.3772669073268088979, 0.5022669073073025015, 0.6272669072877961050 ),
 .UNSPECIFIED. ) ;
#46698=ADVANCED_FACE ( 'NONE', ( #2207 ), #30411, .T. ) ;
#46699=FACE_OUTER_BOUND ( 'NONE', #48400, .T. ) ;
#46700=LINE ( 'NONE', #9271, #10289 ) ;
#46701=FACE_OUTER_BOUND ( 'NONE', #24501, .T. ) ;
#46702=( BOUNDED_CURVE ( )  B_SPLINE_CURVE ( 3, ( #40631, #48268, #22669, #22929 ),
 .UNSPECIFIED., .F., .F. ) 
 B_SPLINE_CURVE_WITH_KNOTS ( ( 4, 4 ),
 ( 0.000000000000000000, 0.4074455897393636228 ),
 .UNSPECIFIED. ) 
 CURVE ( )  GEOMETRIC_REPRESENTATION_ITEM ( )  RATIONAL_B_SPLINE_CURVE ( ( 1.000000000000000000, 0.4567392136813349657, 0.3561768502900314326, 0.6983129098260894008 ) ) 
 REPRESENTATION_ITEM ( '' )  );
#46704=VERTEX_POINT ( 'NONE', #23909 ) ;
#46705=ADVANCED_FACE ( 'NONE', ( #13272 ), #43627, .T. ) ;
#46707=CYLINDRICAL_SURFACE ( 'NONE', #44974, 5.500000000000000000 ) ;
#46709=CARTESIAN_POINT ( 'NONE',  ( -24.48810908846319734, -17.17637088580320537, 73.06831457992643664 ) ) ;
#46710=ADVANCED_FACE ( 'NONE', ( #16495 ), #5437, .F. ) ;
#46711=ORIENTED_EDGE ( 'NONE', *, *, #22793, .T. ) ;
#46712=DIRECTION ( 'NONE',  ( -5.731567514496413899E-31, -1.020425574103664789E-16, -1.000000000000000000 ) ) ;
#46713=( BOUNDED_CURVE ( )  B_SPLINE_CURVE ( 3, ( #31506, #46541, #5659, #42836 ),
 .UNSPECIFIED., .F., .F. ) 
 B_SPLINE_CURVE_WITH_KNOTS ( ( 4, 4 ),
 ( 0.4074455897393680082, 0.5000000000000000000 ),
 .UNSPECIFIED. ) 
 CURVE ( )  GEOMETRIC_REPRESENTATION_ITEM ( )  RATIONAL_B_SPLINE_CURVE ( ( 0.6983129098260871803, 0.7760317562606960928, 0.8765941196520011802, 1.000000000000004663 ) ) 
 REPRESENTATION_ITEM ( '' )  );
#46714=CARTESIAN_POINT ( 'NONE',  ( -9.974481508125691676, -14.72588544478808181, 71.37136786695171509 ) ) ;
#46716=CARTESIAN_POINT ( 'NONE',  ( -22.08699904183838214, -20.10091237387970153, 66.11910372887342646 ) ) ;
#46717=ORIENTED_EDGE ( 'NONE', *, *, #9497, .F. ) ;
#46718=CARTESIAN_POINT ( 'NONE',  ( -16.13432406759100601, -21.74052631579560568, 58.30057715624173653 ) ) ;
#46720=CARTESIAN_POINT ( 'NONE',  ( -24.04044854132572340, -11.23863070794140384, 54.02312124697527906 ) ) ;
#46723=CYLINDRICAL_SURFACE ( 'NONE', #12587, 0.1499999999999986899 ) ;
#46726=CARTESIAN_POINT ( 'NONE',  ( -22.33376602745314798, -19.86903051493498040, 69.18890041286789483 ) ) ;
#46727=CARTESIAN_POINT ( 'NONE',  ( -14.59831579263453527, -7.915781757621413561, 60.44183550242978242 ) ) ;
#46728=ORIENTED_EDGE ( 'NONE', *, *, #11941, .F. ) ;
#46729=EDGE_CURVE ( 'NONE', #35496, #33105, #26657, .T. ) ;
#46730=CARTESIAN_POINT ( 'NONE',  ( -16.05981277502693416, -21.73406819447767901, 61.90001277639490951 ) ) ;
#46731=CARTESIAN_POINT ( 'NONE',  ( -10.76785811675246940, -12.48515291162924434, 57.61385273545094066 ) ) ;
#46732=CARTESIAN_POINT ( 'NONE',  ( -17.01596658974409593, -7.370308080546169371, 74.07522964315150205 ) ) ;
#46734=ORIENTED_EDGE ( 'NONE', *, *, #22009, .F. ) ;
#46735=CARTESIAN_POINT ( 'NONE',  ( -13.38462805196022920, -20.58720062598995426, 58.34650077712428384 ) ) ;
#46736=LINE ( 'NONE', #28007, #20337 ) ;
#46737=CARTESIAN_POINT ( 'NONE',  ( -23.44028840568416783, -19.20329456582437899, 62.55418086402786315 ) ) ;
#46742=ORIENTED_EDGE ( 'NONE', *, *, #13490, .T. ) ;
#46744=CARTESIAN_POINT ( 'NONE',  ( -14.78519852893282582, -21.29287441001463677, 58.46617891049388760 ) ) ;
#46745=CARTESIAN_POINT ( 'NONE',  ( -21.91034545428830782, -20.18261758176410936, 58.76442899736473180 ) ) ;
#46746=CARTESIAN_POINT ( 'NONE',  ( -11.35719102664687874, -18.40077844947705543, 58.09242476654641507 ) ) ;
#46748=CARTESIAN_POINT ( 'NONE',  ( -18.79049830835916524, -7.892586073225762000, 70.38540174208183942 ) ) ;
#46749=B_SPLINE_CURVE_WITH_KNOTS ( 'NONE', 3,
 ( #48455, #33929, #223, #29760, #26070, #15201, #48708, #30259, #45279, #22364 ),
 .UNSPECIFIED., .F., .F.,
 ( 4, 2, 2, 2, 4 ),
 ( 0.1272669073657906602, 0.2522669073462913691, 0.3772669073267920226, 0.5022669073072927315, 0.6272669072877934404 ),
 .UNSPECIFIED. ) ;
#46751=CARTESIAN_POINT ( 'NONE',  ( -10.72530867274958410, -17.00760959713300835, 57.97288447305809456 ) ) ;
#46752=CARTESIAN_POINT ( 'NONE',  ( -23.30016224357493826, -19.38910683590379236, 59.14056577394535452 ) ) ;
#46753=ORIENTED_EDGE ( 'NONE', *, *, #48466, .T. ) ;
#46755=CARTESIAN_POINT ( 'NONE',  ( -10.61641629527463770, -11.78277212779517136, 74.74335553404092991 ) ) ;
#46757=DIRECTION ( 'NONE',  ( -0.1922068328301543838, -0.9813544382196449645, 7.804899501296265607E-08 ) ) ;
#46760=B_SPLINE_CURVE_WITH_KNOTS ( 'NONE', 3,
 ( #31460, #39084, #465, #27766, #1413, #46497, #16176, #8832, #8105, #35143 ),
 .UNSPECIFIED., .F., .F.,
 ( 4, 2, 2, 2, 4 ),
 ( 0.000000000000000000, 0.2500000000000000000, 0.5000000000000000000, 0.7500000000000000000, 1.000000000000000000 ),
 .UNSPECIFIED. ) ;
#46761=ORIENTED_EDGE ( 'NONE', *, *, #44217, .F. ) ;
#46762=EDGE_CURVE ( 'NONE', #37103, #20782, #13521, .T. ) ;
#46763=CARTESIAN_POINT ( 'NONE',  ( -14.96636237700334604, -21.36369153681597410, 61.93600446056886000 ) ) ;
#46765=CARTESIAN_POINT ( 'NONE',  ( -15.48424059001683339, -21.53504990492328375, 72.04575460974366763 ) ) ;
#46768=CARTESIAN_POINT ( 'NONE',  ( -10.13926443761864782, -13.24856975666061665, 74.85630413064295396 ) ) ;
#46769=VECTOR ( 'NONE', #15228, 1000.000000000000114 ) ;
#46772=CARTESIAN_POINT ( 'NONE',  ( -10.50893933415051507, -13.43540278197274063, 74.96345540680638919 ) ) ;
#46773=CARTESIAN_POINT ( 'NONE',  ( -11.06572510127579356, -10.92528991087847068, 57.32247810849851533 ) ) ;
#46774=CARTESIAN_POINT ( 'NONE',  ( -18.98647833766290915, -7.985345034418963373, 66.91688477291717163 ) ) ;
#46775=ORIENTED_EDGE ( 'NONE', *, *, #40499, .T. ) ;
#46776=EDGE_CURVE ( 'NONE', #8086, #48574, #21577, .T. ) ;
#46779=CARTESIAN_POINT ( 'NONE',  ( -10.42496409799848323, -14.69883155267435626, 71.62782692796884021 ) ) ;
#46780=EDGE_LOOP ( 'NONE', ( #42722, #20190, #4061, #47352, #26025 ) ) ;
#46784=DIRECTION ( 'NONE',  ( -9.593247862760507776E-06, -5.650837228699102996E-06, 0.9999999999380188020 ) ) ;
#46785=CARTESIAN_POINT ( 'NONE',  ( -11.42962470904260464, -10.38539412368214521, 74.62380407152070916 ) ) ;
#46787=CARTESIAN_POINT ( 'NONE',  ( -24.43362360091610697, -14.05489060867666851, 73.42271507725003232 ) ) ;
#46788=( BOUNDED_CURVE ( )  B_SPLINE_CURVE ( 3, ( #46434, #34602, #4825, #16115 ),
 .UNSPECIFIED., .F., .F. ) 
 B_SPLINE_CURVE_WITH_KNOTS ( ( 4, 4 ),
 ( 0.4074455897393641779, 0.5000000000000000000 ),
 .UNSPECIFIED. ) 
 CURVE ( )  GEOMETRIC_REPRESENTATION_ITEM ( )  RATIONAL_B_SPLINE_CURVE ( ( 0.6983129098260966172, 0.7760317562607159658, 0.8765941196520214973, 1.000000000000023315 ) ) 
 REPRESENTATION_ITEM ( '' )  );
#46789=CARTESIAN_POINT ( 'NONE',  ( -24.46812100523181144, -14.51191712007779699, 66.19764790277996269 ) ) ;
#46790=CARTESIAN_POINT ( 'NONE',  ( -16.36834346081282732, -22.18410778960565466, 61.94063409281806543 ) ) ;
#46792=CARTESIAN_POINT ( 'NONE',  ( -23.83833621072449560, -17.61232891644574394, 62.47360984984814536 ) ) ;
#46793=CARTESIAN_POINT ( 'NONE',  ( -26.80819156775448420, -19.72453833035618942, 53.49999999999995026 ) ) ;
#46794=CARTESIAN_POINT ( 'NONE',  ( -20.49499702560526870, -8.021383449398966192, 66.91957586719850326 ) ) ;
#46795=CARTESIAN_POINT ( 'NONE',  ( -24.76540221579651302, -16.07765826482591365, 66.17829537637275905 ) ) ;
#46796=EDGE_LOOP ( 'NONE', ( #37427, #38781, #4274, #24169, #45504 ) ) ;
#46797=EDGE_LOOP ( 'NONE', ( #14023, #4156, #20927, #1890, #43018 ) ) ;
#46798=CARTESIAN_POINT ( 'NONE',  ( -22.56207008003183745, -19.63703213565221617, 72.92928497383269359 ) ) ;
#46799=CARTESIAN_POINT ( 'NONE',  ( -10.46944733747312917, -15.96661384539355133, 67.99239968927004441 ) ) ;
#46800=ORIENTED_EDGE ( 'NONE', *, *, #43522, .F. ) ;
#46803=CARTESIAN_POINT ( 'NONE',  ( -10.42807964966673495, -15.04539577713889287, 74.98882032444942070 ) ) ;
#46804=B_SPLINE_CURVE_WITH_KNOTS ( 'NONE', 3,
 ( #20179, #31511, #27327, #42357, #31262, #35191, #46546, #27808, #16713, #35434 ),
 .UNSPECIFIED., .F., .F.,
 ( 4, 2, 2, 2, 4 ),
 ( 0.000000000000000000, 0.2500000000000000000, 0.5000000000000000000, 0.7500000000000000000, 1.000000000000000000 ),
 .UNSPECIFIED. ) ;
#46805=CARTESIAN_POINT ( 'NONE',  ( -12.12786991918758339, -13.32596279628197600, 54.07175714974879099 ) ) ;
#46809=CARTESIAN_POINT ( 'NONE',  ( -22.68532657142340980, -20.08396690885253477, 69.21772085510332317 ) ) ;
#46810=EDGE_CURVE ( 'NONE', #5613, #32492, #42164, .T. ) ;
#46812=CARTESIAN_POINT ( 'NONE',  ( -20.82057359985130773, -8.686965325372206337, 60.06955151264084236 ) ) ;
#46813=LINE ( 'NONE', #9870, #22475 ) ;
#46815=ORIENTED_EDGE ( 'NONE', *, *, #14910, .T. ) ;
#46816=VERTEX_POINT ( 'NONE', #47751 ) ;
#46818=DIRECTION ( 'NONE',  ( 0.4182840851231335866, -0.9083162577718748576, 8.112345261759808545E-09 ) ) ;
#46819=EDGE_CURVE ( 'NONE', #6686, #5083, #35418, .T. ) ;
#46821=VERTEX_POINT ( 'NONE', #33620 ) ;
#46822=CARTESIAN_POINT ( 'NONE',  ( -10.43726484089306439, -14.35454122530442511, 67.96873162560321191 ) ) ;
#46823=CARTESIAN_POINT ( 'NONE',  ( -10.38078067960954520, -14.50222210708341564, 68.15800126083217947 ) ) ;
#46825=DIRECTION ( 'NONE',  ( 0.3124635249310679375, 0.8422251632096487972, 0.4393441931380594467 ) ) ;
#46827=( BOUNDED_CURVE ( )  B_SPLINE_CURVE ( 3, ( #36020, #9466, #2303, #1574 ),
 .UNSPECIFIED., .F., .F. ) 
 B_SPLINE_CURVE_WITH_KNOTS ( ( 4, 4 ),
 ( 1.570796326794896558, 1.780235837034218394 ),
 .UNSPECIFIED. ) 
 CURVE ( )  GEOMETRIC_REPRESENTATION_ITEM ( )  RATIONAL_B_SPLINE_CURVE ( ( 1.000000000000000000, 0.9963479302455153785, 0.9963479302455153785, 1.000000000000000000 ) ) 
 REPRESENTATION_ITEM ( '' )  );
#46828=CARTESIAN_POINT ( 'NONE',  ( -15.84612626051299600, -7.989255239880060699, 67.44007225974215203 ) ) ;
#46829=ORIENTED_EDGE ( 'NONE', *, *, #10035, .T. ) ;
#46830=CARTESIAN_POINT ( 'NONE',  ( -13.49112199889614594, -21.13648260148447378, 65.08654642282640168 ) ) ;
#46832=ORIENTED_EDGE ( 'NONE', *, *, #39494, .F. ) ;
#46834=CARTESIAN_POINT ( 'NONE',  ( -10.70566866894272984, -16.94585410378973123, 57.98760548748136046 ) ) ;
#46840=CARTESIAN_POINT ( 'NONE',  ( -11.30361205576526196, -11.41219277671509147, 64.44882039656690154 ) ) ;
#46842=CARTESIAN_POINT ( 'NONE',  ( -14.57536025382065148, -8.356334209363122767, 60.31996305705101236 ) ) ;
#46844=CARTESIAN_POINT ( 'NONE',  ( -19.28939690137687535, -8.062307696266060475, 59.96092997387292201 ) ) ;
#46845=VERTEX_POINT ( 'NONE', #17697 ) ;
#46846=( BOUNDED_CURVE ( )  B_SPLINE_CURVE ( 3, ( #18480, #22434, #10626, #41149 ),
 .UNSPECIFIED., .F., .F. ) 
 B_SPLINE_CURVE_WITH_KNOTS ( ( 4, 4 ),
 ( 0.4074455897393672310, 0.5000000000000000000 ),
 .UNSPECIFIED. ) 
 CURVE ( )  GEOMETRIC_REPRESENTATION_ITEM ( )  RATIONAL_B_SPLINE_CURVE ( ( 0.6983129098260973944, 0.7760317562607038644, 0.8765941196520053991, 1.000000000000003109 ) ) 
 REPRESENTATION_ITEM ( '' )  );
#46847=PLANE ( 'NONE',  #19177 ) ;
#46848=DIRECTION ( 'NONE',  ( -5.854827030937197869E-31, -1.020425574103664912E-16, -1.000000000000000000 ) ) ;
#46849=LINE ( 'NONE', #47093, #7838 ) ;
#46850=ADVANCED_FACE ( 'NONE', ( #7560 ), #20040, .T. ) ;
#46851=EDGE_CURVE ( 'NONE', #42645, #33357, #13113, .T. ) ;
#46852=CARTESIAN_POINT ( 'NONE',  ( -15.20895699419056335, -21.92244470331527850, 68.71446411004870924 ) ) ;
#46856=EDGE_CURVE ( 'NONE', #8086, #25610, #40452, .T. ) ;
#46858=CARTESIAN_POINT ( 'NONE',  ( -24.45381059137804058, -15.38184444469599299, 72.88814935371863157 ) ) ;
#46859=EDGE_LOOP ( 'NONE', ( #28803, #5331 ) ) ;
#46860=CARTESIAN_POINT ( 'NONE',  ( -11.33385179977767265, -19.10019906511433518, 68.26043675633501095 ) ) ;
#46861=CARTESIAN_POINT ( 'NONE',  ( -14.44809135640554487, -8.473323881223761234, 67.55975083863336295 ) ) ;
#46862=CARTESIAN_POINT ( 'NONE',  ( -12.73947787985187574, -9.016276410220392279, 71.10571287364943771 ) ) ;
#46866=CYLINDRICAL_SURFACE ( 'NONE', #31796, 0.1500000000000008826 ) ;
#46867=CARTESIAN_POINT ( 'NONE',  ( -12.10131192688100299, -10.18592936015514816, 64.31442259820508411 ) ) ;
#46868=CARTESIAN_POINT ( 'NONE',  ( -20.69509252757554307, -8.115601716887088202, 63.49616818922779515 ) ) ;
#46870=EDGE_LOOP ( 'NONE', ( #33369, #39135 ) ) ;
#46871=CARTESIAN_POINT ( 'NONE',  ( -13.33011785382929304, -9.069340661520646663, 63.92418669539090814 ) ) ;
#46872=CARTESIAN_POINT ( 'NONE',  ( -13.30711473254145716, -9.147892019113847084, 63.90946529584681457 ) ) ;
#46873=FACE_OUTER_BOUND ( 'NONE', #32673, .T. ) ;
#46876=ORIENTED_EDGE ( 'NONE', *, *, #31552, .T. ) ;
#46877=ORIENTED_EDGE ( 'NONE', *, *, #37651, .T. ) ;
#46878=VECTOR ( 'NONE', #1263, 1000.000000000000114 ) ;
#46880=B_SPLINE_CURVE_WITH_KNOTS ( 'NONE', 1,
 ( #35255, #31089 ),
 .UNSPECIFIED., .F., .F.,
 ( 2, 2 ),
 ( 0.000000000000000000, 1.000000000000000000 ),
 .UNSPECIFIED. ) ;
#46881=CARTESIAN_POINT ( 'NONE',  ( -15.06092214208368141, -7.686424710462701704, 53.76173960638114124 ) ) ;
#46883=CARTESIAN_POINT ( 'NONE',  ( -24.45201636468676654, -14.25170757634699825, 69.95275273439749242 ) ) ;
#46886=CYLINDRICAL_SURFACE ( 'NONE', #6371, 0.1499999999999971634 ) ;
#46887=CARTESIAN_POINT ( 'NONE',  ( -24.25527139147240518, -17.78202422108329017, 62.67349770570701395 ) ) ;
#46889=EDGE_LOOP ( 'NONE', ( #30061, #1782 ) ) ;
#46890=CARTESIAN_POINT ( 'NONE',  ( -21.89826351590202336, -8.852228842849337198, 66.84645279485334868 ) ) ;
#46891=CARTESIAN_POINT ( 'NONE',  ( -16.32745258320347759, -21.77369344365219561, 61.77040269689842944 ) ) ;
#46892=( BOUNDED_CURVE ( )  B_SPLINE_CURVE ( 3, ( #19336, #23288, #5063, #1598 ),
 .UNSPECIFIED., .F., .F. ) 
 B_SPLINE_CURVE_WITH_KNOTS ( ( 4, 4 ),
 ( 0.000000000000000000, 0.4074455897269660953 ),
 .UNSPECIFIED. ) 
 CURVE ( )  GEOMETRIC_REPRESENTATION_ITEM ( )  RATIONAL_B_SPLINE_CURVE ( ( 1.000000000000000000, 0.4567392136978657424, 0.3561768502961514260, 0.6983129097948570507 ) ) 
 REPRESENTATION_ITEM ( '' )  );
#46893=VERTEX_POINT ( 'NONE', #1358 ) ;
#46894=CARTESIAN_POINT ( 'NONE',  ( -10.53536195276627829, -13.30851587854854579, 74.69289754060230280 ) ) ;
#46895=CARTESIAN_POINT ( 'NONE',  ( -22.92319839529956838, -10.39759132684999265, 63.22185995336808162 ) ) ;
#46896=ORIENTED_EDGE ( 'NONE', *, *, #22009, .T. ) ;
#46897=CARTESIAN_POINT ( 'NONE',  ( -17.77761167241057549, -22.25089262147902147, 58.44907471483963946 ) ) ;
#46898=EDGE_CURVE ( 'NONE', #3283, #26502, #10426, .T. ) ;
#46900=CARTESIAN_POINT ( 'NONE',  ( -16.76036020169118146, -21.82793338258416327, 68.69560668698967731 ) ) ;
#46902=CARTESIAN_POINT ( 'NONE',  ( -10.33481637538221243, -12.51883299443452202, 60.84207650303104487 ) ) ;
#46903=DIRECTION ( 'NONE',  ( 6.446466753401607987E-06, -1.047023822510701943E-05, -0.9999999999244085780 ) ) ;
#46904=CARTESIAN_POINT ( 'NONE',  ( -21.55883939963115026, -8.611815437115641458, 73.78624134823098757 ) ) ;
#46905=AXIS2_PLACEMENT_3D ( 'NONE', #27920, #25381, #44577 ) ;
#46907=CARTESIAN_POINT ( 'NONE',  ( -12.04584144946014312, -10.25080825636289816, 67.50456653540463492 ) ) ;
#46908=EDGE_CURVE ( 'NONE', #48314, #24620, #19213, .T. ) ;
#46910=FACE_OUTER_BOUND ( 'NONE', #35028, .T. ) ;
#46911=EDGE_CURVE ( 'NONE', #3548, #1447, #30458, .T. ) ;
#46914=CARTESIAN_POINT ( 'NONE',  ( -13.84778738435022305, -8.273584231232366193, 74.32141925404624772 ) ) ;
#46915=EDGE_CURVE ( 'NONE', #14217, #27480, #23796, .T. ) ;
#46916=CARTESIAN_POINT ( 'NONE',  ( -15.15660932275500272, -21.48492473237050859, 65.39124617759186719 ) ) ;
#46920=ORIENTED_EDGE ( 'NONE', *, *, #11792, .F. ) ;
#46921=ORIENTED_EDGE ( 'NONE', *, *, #23970, .F. ) ;
#46923=CARTESIAN_POINT ( 'NONE',  ( -15.68503317936312236, -7.977064329016499755, 70.60989839961001735 ) ) ;
#46924=LINE ( 'NONE', #25004, #31087 ) ;
#46927=CARTESIAN_POINT ( 'NONE',  ( -13.46747565276156422, -9.034678650756244878, 60.73950277887485072 ) ) ;
#46928=ORIENTED_EDGE ( 'NONE', *, *, #36586, .F. ) ;
#46929=ORIENTED_EDGE ( 'NONE', *, *, #19794, .T. ) ;
#46931=PLANE ( 'NONE',  #36964 ) ;
#46932=CARTESIAN_POINT ( 'NONE',  ( -20.94265863490610258, -21.37680627582274795, 62.30126734817043399 ) ) ;
#46933=CARTESIAN_POINT ( 'NONE',  ( -23.23812175398343172, -18.70765974062167203, 66.10924015431194789 ) ) ;
#46935=VECTOR ( 'NONE', #21280, 1000.000000000000000 ) ;
#46936=EDGE_LOOP ( 'NONE', ( #41826, #7262, #12105, #3211, #9056 ) ) ;
#46937=FACE_OUTER_BOUND ( 'NONE', #1237, .T. ) ;
#46939=LINE ( 'NONE', #6786, #14175 ) ;
#46941=EDGE_CURVE ( 'NONE', #8650, #15655, #30704, .T. ) ;
#46942=ORIENTED_EDGE ( 'NONE', *, *, #7275, .T. ) ;
#46944=CARTESIAN_POINT ( 'NONE',  ( -11.04141120970326462, -11.93494789359697883, 74.55840195308121565 ) ) ;
#46945=CARTESIAN_POINT ( 'NONE',  ( -24.47401588851211329, -14.84236380343934592, 59.24300237059242136 ) ) ;
#46948=CARTESIAN_POINT ( 'NONE',  ( -22.88419684932020459, -10.42887832691348926, 63.37185995611467604 ) ) ;
#46949=CARTESIAN_POINT ( 'NONE',  ( -18.11396434131172128, -21.77512919714542150, 65.34532159443909904 ) ) ;
#46951=FACE_OUTER_BOUND ( 'NONE', #25873, .T. ) ;
#46952=VERTEX_POINT ( 'NONE', #34360 ) ;
#46953=CARTESIAN_POINT ( 'NONE',  ( -13.54823083431842612, -20.69819501703281617, 61.66646323538943619 ) ) ;
#46954=CARTESIAN_POINT ( 'NONE',  ( -16.32142643024854678, -21.72225621288954400, 61.77184823017776694 ) ) ;
#46955=VERTEX_POINT ( 'NONE', #15895 ) ;
#46956=CARTESIAN_POINT ( 'NONE',  ( -24.17271927670314113, -12.95015993349377048, 66.30246741691458112 ) ) ;
#46957=CARTESIAN_POINT ( 'NONE',  ( -21.91034708787274710, -20.18261625685872218, 59.06442899735736773 ) ) ;
#46958=CARTESIAN_POINT ( 'NONE',  ( -13.30028440927262068, -8.603736347584243660, 60.62605674953037749 ) ) ;
#46959=EDGE_CURVE ( 'NONE', #37312, #48665, #16845, .T. ) ;
#46961=VERTEX_POINT ( 'NONE', #23551 ) ;
#46962=CARTESIAN_POINT ( 'NONE',  ( -23.94599579101543796, -17.50730996363388314, 59.15945600998260545 ) ) ;
#46963=EDGE_CURVE ( 'NONE', #44379, #10553, #2204, .T. ) ;
#46964=( BOUNDED_CURVE ( )  B_SPLINE_CURVE ( 3, ( #40654, #44376, #25639, #17995 ),
 .UNSPECIFIED., .F., .F. ) 
 B_SPLINE_CURVE_WITH_KNOTS ( ( 4, 4 ),
 ( 0.5000000000000000000, 0.9074455897393697290 ),
 .UNSPECIFIED. ) 
 CURVE ( )  GEOMETRIC_REPRESENTATION_ITEM ( )  RATIONAL_B_SPLINE_CURVE ( ( 1.000000000000002442, 0.4567392136813364645, 0.3561768502900302114, 0.6983129098260862921 ) ) 
 REPRESENTATION_ITEM ( '' )  );
#46965=CARTESIAN_POINT ( 'NONE',  ( -11.35824946695446691, -11.21643166988602047, 60.82885780703593070 ) ) ;
#46967=CARTESIAN_POINT ( 'NONE',  ( -11.22202139642810081, -18.93699991513116743, 64.92423932127240960 ) ) ;
#46970=CARTESIAN_POINT ( 'NONE',  ( -11.10386593012501244, -18.75361831986885974, 61.32064883311096537 ) ) ;
#46971=ORIENTED_EDGE ( 'NONE', *, *, #752, .F. ) ;
#46972=EDGE_LOOP ( 'NONE', ( #120, #29277, #5652, #9151, #44335 ) ) ;
#46973=CARTESIAN_POINT ( 'NONE',  ( -14.74690617566109019, -21.27702427001963414, 58.46617884968173229 ) ) ;
#46974=CARTESIAN_POINT ( 'NONE',  ( -21.42336380182764088, -21.09487415076890215, 69.23945570945444672 ) ) ;
#46978=CARTESIAN_POINT ( 'NONE',  ( -12.44869005970189058, -9.885249076858732664, 57.08935532200567309 ) ) ;
#46979=EDGE_CURVE ( 'NONE', #37877, #41056, #3344, .T. ) ;
#46980=( BOUNDED_CURVE ( )  B_SPLINE_CURVE ( 3, ( #44911, #22483, #37478, #3771 ),
 .UNSPECIFIED., .F., .F. ) 
 B_SPLINE_CURVE_WITH_KNOTS ( ( 4, 4 ),
 ( 0.000000000000000000, 0.4074455897393643444 ),
 .UNSPECIFIED. ) 
 CURVE ( )  GEOMETRIC_REPRESENTATION_ITEM ( )  RATIONAL_B_SPLINE_CURVE ( ( 1.000000000000000000, 0.4567392136813230308, 0.3561768502900269917, 0.6983129098261118273 ) ) 
 REPRESENTATION_ITEM ( '' )  );
#46981=CARTESIAN_POINT ( 'NONE',  ( -13.11716721000957264, -9.290864365938665159, 67.67942741430334763 ) ) ;
#46982=( BOUNDED_CURVE ( )  B_SPLINE_CURVE ( 3, ( #42288, #8550, #7840, #42041 ),
 .UNSPECIFIED., .F., .F. ) 
 B_SPLINE_CURVE_WITH_KNOTS ( ( 4, 4 ),
 ( 0.4074455897393652326, 0.5000000000000000000 ),
 .UNSPECIFIED. ) 
 CURVE ( )  GEOMETRIC_REPRESENTATION_ITEM ( )  RATIONAL_B_SPLINE_CURVE ( ( 0.6983129098260798528, 0.7760317562606897646, 0.8765941196519972944, 1.000000000000004663 ) ) 
 REPRESENTATION_ITEM ( '' )  );
#46985=VERTEX_POINT ( 'NONE', #9975 ) ;
#46986=EDGE_LOOP ( 'NONE', ( #23791, #27939, #10940, #41457, #29023 ) ) ;
#46987=LINE ( 'NONE', #12286, #8485 ) ;
#46989=CARTESIAN_POINT ( 'NONE',  ( -23.63039969342750979, -11.57141254907242534, 66.72214533111647938 ) ) ;
#46991=CARTESIAN_POINT ( 'NONE',  ( -22.38860293988961558, -19.74596265805258710, 72.71570726583541955 ) ) ;
#46992=CARTESIAN_POINT ( 'NONE',  ( -20.81921488491704864, -21.44071703825394692, 58.75979854551385984 ) ) ;
#46993=( BOUNDED_CURVE ( )  B_SPLINE_CURVE ( 3, ( #17448, #28779, #24614, #13968 ),
 .UNSPECIFIED., .F., .F. ) 
 B_SPLINE_CURVE_WITH_KNOTS ( ( 4, 4 ),
 ( 0.000000000000000000, 0.4074455897393687298 ),
 .UNSPECIFIED. ) 
 CURVE ( )  GEOMETRIC_REPRESENTATION_ITEM ( )  RATIONAL_B_SPLINE_CURVE ( ( 1.000000000000000000, 0.4567392136813349657, 0.3561768502900314326, 0.6983129098260894008 ) ) 
 REPRESENTATION_ITEM ( '' )  );
#46995=CARTESIAN_POINT ( 'NONE',  ( -12.27604185553471616, -19.62628656662749549, 58.21210303282668264 ) ) ;
#46996=CARTESIAN_POINT ( 'NONE',  ( -10.21566995694600166, -12.92691906471870311, 67.91549220782184193 ) ) ;
#46997=CARTESIAN_POINT ( 'NONE',  ( -11.78595478178340805, -10.57665929355158241, 74.43885099124366889 ) ) ;
#46998=CARTESIAN_POINT ( 'NONE',  ( -24.48810873059073856, -17.17637193698283582, 73.06831349224263761 ) ) ;
#47000=EDGE_LOOP ( 'NONE', ( #19464, #36118, #32009, #27007, #7489 ) ) ;
#47001=CARTESIAN_POINT ( 'NONE',  ( -10.14076703847185001, -13.24135396021726763, 74.81784294846195849 ) ) ;
#47003=CARTESIAN_POINT ( 'NONE',  ( -13.18474066807476675, -20.93551553819402855, 58.23145462665691241 ) ) ;
#47005=CARTESIAN_POINT ( 'NONE',  ( -18.65633144910794883, -7.917218216242548401, 74.06894365739631780 ) ) ;
#47007=CARTESIAN_POINT ( 'NONE',  ( -14.79922817013080483, -7.836842635312091687, 57.03495431467663224 ) ) ;
#47008=ORIENTED_EDGE ( 'NONE', *, *, #43310, .T. ) ;
#47009=EDGE_CURVE ( 'NONE', #23317, #6093, #37959, .T. ) ;
#47010=CARTESIAN_POINT ( 'NONE',  ( -10.48584376121421791, -13.88064436164177984, 57.74825077270041618 ) ) ;
#47012=VERTEX_POINT ( 'NONE', #46679 ) ;
#47013=CARTESIAN_POINT ( 'NONE',  ( -10.01355597153913024, -14.04293878122132178, 61.11159607317906506 ) ) ;
#47014=B_SPLINE_CURVE_WITH_KNOTS ( 'NONE', 3,
 ( #13584, #24214, #12873, #17532, #28630, #28862, #24466, #31840, #32557, #39471 ),
 .UNSPECIFIED., .F., .F.,
 ( 4, 2, 2, 2, 4 ),
 ( 0.000000000000000000, 0.2500000000000000000, 0.5000000000000000000, 0.7500000000000000000, 1.000000000000000000 ),
 .UNSPECIFIED. ) ;
#47015=CARTESIAN_POINT ( 'NONE',  ( -12.50766595982653584, -19.86205097402751463, 65.01674886870775083 ) ) ;
#47017=CARTESIAN_POINT ( 'NONE',  ( -10.29584670662963752, -12.64300724171409662, 64.44648870780133620 ) ) ;
#47020=CARTESIAN_POINT ( 'NONE',  ( -15.19548991633585011, -21.91815178685365595, 68.76088227238139439 ) ) ;
#47021=CARTESIAN_POINT ( 'NONE',  ( -24.46479343890040425, -14.44719913075708995, 66.48292729247951627 ) ) ;
#47022=CARTESIAN_POINT ( 'NONE',  ( -14.73525069530193399, -21.75714069359356984, 61.89246344873641448 ) ) ;
#47024=CARTESIAN_POINT ( 'NONE',  ( -16.12205861630594939, -7.931364996939863410, 60.39131567725520711 ) ) ;
#47026=B_SPLINE_CURVE_WITH_KNOTS ( 'NONE', 1,
 ( #16852, #40478 ),
 .UNSPECIFIED., .F., .F.,
 ( 2, 2 ),
 ( 0.000000000000000000, 1.000000000000000000 ),
 .UNSPECIFIED. ) ;
#47030=ORIENTED_EDGE ( 'NONE', *, *, #23952, .F. ) ;
#47031=VERTEX_POINT ( 'NONE', #16623 ) ;
#47032=EDGE_CURVE ( 'NONE', #6412, #9098, #43814, .T. ) ;
#47033=DIRECTION ( 'NONE',  ( 0.7248509490090242480, -0.6889057277456162032, 1.880377065355303572E-09 ) ) ;
#47034=CARTESIAN_POINT ( 'NONE',  ( -24.22092292145011072, -12.93687797069017975, 66.60246741374322710 ) ) ;
#47035=ORIENTED_EDGE ( 'NONE', *, *, #33718, .F. ) ;
#47037=CARTESIAN_POINT ( 'NONE',  ( -10.00132051839154457, -15.44646819276786154, 57.82438731113803243 ) ) ;
#47038=CARTESIAN_POINT ( 'NONE',  ( -23.16117746674104438, -18.90708040007733359, 62.63934749780565880 ) ) ;
#47039=EDGE_CURVE ( 'NONE', #2068, #25341, #28458, .T. ) ;
#47041=CARTESIAN_POINT ( 'NONE',  ( -13.43921731646364925, -8.993429882417945720, 60.43950277494440115 ) ) ;
#47045=AXIS2_PLACEMENT_3D ( 'NONE', #22015, #7255, #37012 ) ;
#47047=VERTEX_POINT ( 'NONE', #12926 ) ;
#47048=CARTESIAN_POINT ( 'NONE',  ( -22.68646401470678953, -20.08284273627726435, 69.35913316877790180 ) ) ;
#47050=B_SPLINE_CURVE_WITH_KNOTS ( 'NONE', 3,
 ( #567, #16048, #19036, #11400, #27155, #34782, #330, #11900, #26424, #42177 ),
 .UNSPECIFIED., .F., .F.,
 ( 4, 2, 2, 2, 4 ),
 ( 0.1272669073658120598, 0.2522669073463025269, 0.3772669073267930218, 0.5022669073072834056, 0.6272669072877739005 ),
 .UNSPECIFIED. ) ;
#47051=CARTESIAN_POINT ( 'NONE',  ( -24.47371109942907808, -14.90716652360855754, 59.25772288469824645 ) ) ;
#47052=CARTESIAN_POINT ( 'NONE',  ( -13.45042189503786645, -20.57396435267970247, 61.70573509705739923 ) ) ;
#47053=EDGE_CURVE ( 'NONE', #20228, #19518, #38581, .T. ) ;
#47054=B_SPLINE_CURVE_WITH_KNOTS ( 'NONE', 3,
 ( #5732, #31820, #35504, #13325, #20739, #11966, #23050, #11712, #47085, #43402 ),
 .UNSPECIFIED., .F., .F.,
 ( 4, 2, 2, 2, 4 ),
 ( 0.6272669072877935514, 0.7522669073072928425, 0.8772669073267920226, 1.002266907346291314, 1.127266907365790605 ),
 .UNSPECIFIED. ) ;
#47057=ORIENTED_EDGE ( 'NONE', *, *, #35349, .F. ) ;
#47059=EDGE_CURVE ( 'NONE', #166, #12496, #18147, .T. ) ;
#47061=CARTESIAN_POINT ( 'NONE',  ( -24.86960059988683014, -14.52975442119237748, 62.82641240410487171 ) ) ;
#47062=CARTESIAN_POINT ( 'NONE',  ( -12.50766578132126838, -19.86205079821699115, 65.16674886870754335 ) ) ;
#47063=CARTESIAN_POINT ( 'NONE',  ( -21.69127741654737918, -9.260229650215405783, 63.38256923939299270 ) ) ;
#47064=ORIENTED_EDGE ( 'NONE', *, *, #2607, .F. ) ;
#47067=ORIENTED_EDGE ( 'NONE', *, *, #46030, .F. ) ;
#47068=CARTESIAN_POINT ( 'NONE',  ( -11.49287318421094817, -18.63485491799402993, 57.96281551145487043 ) ) ;
#47069=AXIS2_PLACEMENT_3D ( 'NONE', #42625, #9123, #8885 ) ;
#47070=( BOUNDED_SURFACE ( )  B_SPLINE_SURFACE ( 3, 1, ( 
 ( #42928, #9200 ),
 ( #39227, #36705 ),
 ( #18497, #7447 ),
 ( #43910, #10163 ),
 ( #48066, #21963 ),
 ( #3249, #22454 ),
 ( #40916, #14303 ) ),
 .UNSPECIFIED., .T., .F., .F. ) 
 B_SPLINE_SURFACE_WITH_KNOTS ( ( 4, 3, 4 ),
 ( 2, 2 ),
 ( 0.000000000000000000, 0.5000000000000000000, 1.000000000000000000 ),
 ( 0.000000000000000000, 1.000000000000000000 ),
 .UNSPECIFIED. ) 
 GEOMETRIC_REPRESENTATION_ITEM ( )  RATIONAL_B_SPLINE_SURFACE ( (
 ( 1.000000000000000000, 1.000000000000000000),
 ( 0.3333333333333335369, 0.3333333333333330373),
 ( 0.3333333333333335369, 0.3333333333333330373),
 ( 1.000000000000000000, 1.000000000000000000),
 ( 0.3333333333333333703, 0.3333333333333333703),
 ( 0.3333333333333333703, 0.3333333333333333703),
 ( 1.000000000000000000, 1.000000000000000000) ) ) 
 REPRESENTATION_ITEM ( '' )  SURFACE ( )  );
#47071=CARTESIAN_POINT ( 'NONE',  ( -12.93830821282824317, -9.435326670572035113, 71.13459971530836867 ) ) ;
#47072=VERTEX_POINT ( 'NONE', #14115 ) ;
#47073=CARTESIAN_POINT ( 'NONE',  ( -15.81170465868504316, -7.997374279965050903, 67.42541861783800528 ) ) ;
#47074=ORIENTED_EDGE ( 'NONE', *, *, #16284, .F. ) ;
#47075=CARTESIAN_POINT ( 'NONE',  ( -13.54527334699669261, -21.17000357857808979, 65.12482326698327029 ) ) ;
#47076=AXIS2_PLACEMENT_3D ( 'NONE', #17587, #17819, #47164 ) ;
#47078=VERTEX_POINT ( 'NONE', #6765 ) ;
#47079=CARTESIAN_POINT ( 'NONE',  ( -24.87351451566537364, -14.94990356866029657, 59.42955486997114178 ) ) ;
#47080=CARTESIAN_POINT ( 'NONE',  ( -23.34481426128875015, -18.63642081788813343, 69.29371984264746231 ) ) ;
#47083=CARTESIAN_POINT ( 'NONE',  ( -24.26805285345972152, -17.75277705495486558, 62.65077900732924121 ) ) ;
#47084=EDGE_CURVE ( 'NONE', #1918, #1214, #7508, .T. ) ;
#47085=CARTESIAN_POINT ( 'NONE',  ( -24.68443261157628754, -16.47976694508638573, 59.23058295855666699 ) ) ;
#47086=CARTESIAN_POINT ( 'NONE',  ( -23.77312771997254615, -18.70709664074277612, 72.87872845841107505 ) ) ;
#47090=ORIENTED_EDGE ( 'NONE', *, *, #13467, .F. ) ;
#47093=CARTESIAN_POINT ( 'NONE',  ( -15.68503317936312236, -7.977064329016500643, 70.60989839961001735 ) ) ;
#47095=EDGE_CURVE ( 'NONE', #18567, #24527, #10694, .T. ) ;
#47098=ORIENTED_EDGE ( 'NONE', *, *, #2445, .F. ) ;
#47099=CARTESIAN_POINT ( 'NONE',  ( -21.18536505927766456, -21.24010891514583221, 65.84099883884408655 ) ) ;
#47103=CARTESIAN_POINT ( 'NONE',  ( -10.58454466348024425, -16.55148359085594478, 71.60317204484042009 ) ) ;
#47105=CARTESIAN_POINT ( 'NONE',  ( -19.37638992839121954, -7.619477365241829503, 60.00447059577386710 ) ) ;
#47106=CARTESIAN_POINT ( 'NONE',  ( -16.19814381282456495, -21.75179583453235210, 58.58585572026736088 ) ) ;
#47107=ORIENTED_EDGE ( 'NONE', *, *, #19836, .T. ) ;
#47108=CARTESIAN_POINT ( 'NONE',  ( -23.70135507383723805, -11.71146680393053607, 62.95218278684509983 ) ) ;
#47109=CYLINDRICAL_SURFACE ( 'NONE', #13902, 0.1500000000000000222 ) ;
#47110=CARTESIAN_POINT ( 'NONE',  ( -20.36536858953947515, -8.398766899984980938, 63.19632798853695022 ) ) ;
#47111=EDGE_LOOP ( 'NONE', ( #12692, #3799, #25300, #7270, #23853 ) ) ;
#47112=( LENGTH_UNIT ( ) NAMED_UNIT ( * ) SI_UNIT ( .MILLI., .METRE. ) );
#47113=VECTOR ( 'NONE', #9443, 1000.000000000000000 ) ;
#47114=CARTESIAN_POINT ( 'NONE',  ( -10.42782603960657895, -12.24862780158598596, 57.50670067860124135 ) ) ;
#47115=CARTESIAN_POINT ( 'NONE',  ( -24.27556694116850977, -13.13524334109580671, 66.71735578995932769 ) ) ;
#47117=B_SPLINE_CURVE_WITH_KNOTS ( 'NONE', 3,
 ( #44622, #33020, #14777, #21961, #48296, #36958, #18746, #2755, #2997, #25900 ),
 .UNSPECIFIED., .F., .F.,
 ( 4, 2, 2, 2, 4 ),
 ( 0.000000000000000000, 0.2500000000000000000, 0.5000000000000000000, 0.7500000000000000000, 1.000000000000000000 ),
 .UNSPECIFIED. ) ;
#47118=CARTESIAN_POINT ( 'NONE',  ( -20.97184585037232196, -20.90166497323120609, 65.59013753914614142 ) ) ;
#47122=VERTEX_POINT ( 'NONE', #37259 ) ;
#47125=EDGE_CURVE ( 'NONE', #15992, #24162, #15617, .T. ) ;
#47126=PLANE ( 'NONE',  #2817 ) ;
#47127=CARTESIAN_POINT ( 'NONE',  ( -14.10880350886743173, -8.137386945752117740, 70.90770375044263574 ) ) ;
#47128=VECTOR ( 'NONE', #31462, 1000.000000000000114 ) ;
#47129=( BOUNDED_CURVE ( )  B_SPLINE_CURVE ( 3, ( #18819, #41224, #14595, #33827 ),
 .UNSPECIFIED., .F., .F. ) 
 B_SPLINE_CURVE_WITH_KNOTS ( ( 4, 4 ),
 ( 1.570796326794896780, 1.780235837034210622 ),
 .UNSPECIFIED. ) 
 CURVE ( )  GEOMETRIC_REPRESENTATION_ITEM ( )  RATIONAL_B_SPLINE_CURVE ( ( 1.000000000000000000, 0.9963479302455156006, 0.9963479302455156006, 1.000000000000000000 ) ) 
 REPRESENTATION_ITEM ( '' )  );
#47131=EDGE_CURVE ( 'NONE', #1174, #4066, #48357, .T. ) ;
#47132=CARTESIAN_POINT ( 'NONE',  ( -22.95715174103553835, -10.52130167614524758, 59.88738023529671040 ) ) ;
#47133=LINE ( 'NONE', #13615, #25398 ) ;
#47134=ORIENTED_EDGE ( 'NONE', *, *, #38916, .T. ) ;
#47135=CARTESIAN_POINT ( 'NONE',  ( -24.40217300928714650, -14.25566238011515274, 69.65275273531472067 ) ) ;
#47136=B_SPLINE_CURVE_WITH_KNOTS ( 'NONE', 3,
 ( #21445, #16986, #17238, #32031, #24413, #31793, #32744, #47768, #35951, #35705 ),
 .UNSPECIFIED., .F., .F.,
 ( 4, 2, 2, 2, 4 ),
 ( 0.6272669072976915228, 0.7522669073147286722, 0.8772669073317658217, 1.002266907348802860, 1.127266907365840121 ),
 .UNSPECIFIED. ) ;
#47137=DIRECTION ( 'NONE',  ( -0.9950649908465213356, -0.09922531930717198856, 4.894557008102619459E-08 ) ) ;
#47139=CARTESIAN_POINT ( 'NONE',  ( -19.14114274275229377, -7.967774638140072696, 66.99252055880820933 ) ) ;
#47140=( BOUNDED_CURVE ( )  B_SPLINE_CURVE ( 3, ( #5560, #20576, #16611, #6271 ),
 .UNSPECIFIED., .F., .F. ) 
 B_SPLINE_CURVE_WITH_KNOTS ( ( 4, 4 ),
 ( 0.5000000000000000000, 0.9074455897393635118 ),
 .UNSPECIFIED. ) 
 CURVE ( )  GEOMETRIC_REPRESENTATION_ITEM ( )  RATIONAL_B_SPLINE_CURVE ( ( 1.000000000000012657, 0.4567392136813371306, 0.3561768502900231614, 0.6983129098260846268 ) ) 
 REPRESENTATION_ITEM ( '' )  );
#47141=CARTESIAN_POINT ( 'NONE',  ( -12.90644018576984386, -9.461596219648651385, 74.60306486165157480 ) ) ;
#47144=CARTESIAN_POINT ( 'NONE',  ( -10.75331705403316818, -16.93070056221711184, 57.98760548944069626 ) ) ;
#47145=ORIENTED_EDGE ( 'NONE', *, *, #38795, .T. ) ;
#47146=ADVANCED_FACE ( 'NONE', ( #3306 ), #10944, .T. ) ;
#47147=CARTESIAN_POINT ( 'NONE',  ( -23.33759473803162621, -18.55732873115717041, 72.99198201251103058 ) ) ;
#47149=CARTESIAN_POINT ( 'NONE',  ( -24.71173182865732443, -13.26207253172215950, 59.46993791559596332 ) ) ;
#47151=CARTESIAN_POINT ( 'NONE',  ( -17.81243367693841151, -24.25303685828974665, 53.49999999999995026 ) ) ;
#47152=CYLINDRICAL_SURFACE ( 'NONE', #26617, 0.1500000000000032419 ) ;
#47153=VECTOR ( 'NONE', #35464, 1000.000000000000000 ) ;
#47154=CIRCLE ( 'NONE', #25921, 2.499999999999999556 ) ;
#47155=CARTESIAN_POINT ( 'NONE',  ( -15.48424059001683339, -21.53504990492328375, 72.04575460974366763 ) ) ;
#47156=CARTESIAN_POINT ( 'NONE',  ( -12.05806040642128707, -10.23620046216302448, 67.51368956197082127 ) ) ;
#47159=LINE ( 'NONE', #28200, #34562 ) ;
#47161=ORIENTED_EDGE ( 'NONE', *, *, #19995, .F. ) ;
#47162=CARTESIAN_POINT ( 'NONE',  ( -10.71495554099518088, -12.81234323494808436, 64.56836111193433680 ) ) ;
#47164=DIRECTION ( 'NONE',  ( 9.444166279764887802E-07, -1.975884206576272611E-06, -0.9999999999976019183 ) ) ;
#47165=EDGE_LOOP ( 'NONE', ( #24063, #22396, #16099, #37805, #43900 ) ) ;
#47168=ORIENTED_EDGE ( 'NONE', *, *, #35045, .F. ) ;
#47172=CARTESIAN_POINT ( 'NONE',  ( -16.07865488608826254, -7.939723797651444315, 63.67011030349581091 ) ) ;
#47173=CARTESIAN_POINT ( 'NONE',  ( -16.91478550490786503, -21.84108428878278119, 72.18015306840750611 ) ) ;
#47174=CARTESIAN_POINT ( 'NONE',  ( -16.28362587665221639, -22.17156497440846152, 61.91714677727144078 ) ) ;
#47175=ORIENTED_EDGE ( 'NONE', *, *, #36128, .T. ) ;
#47180=DIRECTION ( 'NONE',  ( 3.549360974554993999E-17, -6.371834667797928663E-18, -1.000000000000000000 ) ) ;
#47181=CARTESIAN_POINT ( 'NONE',  ( -24.06394650331561635, -17.02597731989300556, 72.88336026101553955 ) ) ;
#47185=EDGE_CURVE ( 'NONE', #40875, #22320, #21777, .T. ) ;
#47188=B_SPLINE_CURVE_WITH_KNOTS ( 'NONE', 3,
 ( #35007, #16283, #42897, #9168, #39191, #20494, #30619, #1776, #11895, #23222 ),
 .UNSPECIFIED., .F., .F.,
 ( 4, 2, 2, 2, 4 ),
 ( 0.000000000000000000, 0.2500000000000000000, 0.5000000000000000000, 0.7500000000000000000, 1.000000000000000000 ),
 .UNSPECIFIED. ) ;
#47189=ADVANCED_FACE ( 'NONE', ( #26208 ), #41219, .F. ) ;
#47190=CARTESIAN_POINT ( 'NONE',  ( -24.37817933763783529, -15.98629254845087466, 69.94796348494512017 ) ) ;
#47192=ADVANCED_FACE ( 'NONE', ( #30159 ), #21898, .T. ) ;
#47194=DIRECTION ( 'NONE',  ( 0.7437128929774847741, -0.6684991644116392573, 1.736198598216997869E-08 ) ) ;
#47195=PLANE ( 'NONE',  #22123 ) ;
#47196=CARTESIAN_POINT ( 'NONE',  ( -16.24762640633412758, -21.70976015997750963, 58.28585518769421014 ) ) ;
#47197=CARTESIAN_POINT ( 'NONE',  ( -14.45970594486164806, -7.974362378399544760, 63.89004585484453713 ) ) ;
#47198=EDGE_CURVE ( 'NONE', #19672, #46068, #45899, .T. ) ;
#47199=ORIENTED_EDGE ( 'NONE', *, *, #33706, .T. ) ;
#47201=CARTESIAN_POINT ( 'NONE',  ( -22.79874446983080816, -10.32434671450250008, 63.14473989550985067 ) ) ;
#47202=CARTESIAN_POINT ( 'NONE',  ( -18.07488560852729975, -21.77899938210117980, 65.34532180047121130 ) ) ;
#47205=ORIENTED_EDGE ( 'NONE', *, *, #14219, .F. ) ;
#47206=CARTESIAN_POINT ( 'NONE',  ( -14.65765131015531253, -21.78034674156931061, 53.49999999999994316 ) ) ;
#47207=CARTESIAN_POINT ( 'NONE',  ( -14.59148033128425404, -7.918538076466720810, 60.48029674573233905 ) ) ;
#47209=CARTESIAN_POINT ( 'NONE',  ( -10.33531692083374587, -17.10115316349580894, 57.87255846826901262 ) ) ;
#47210=CARTESIAN_POINT ( 'NONE',  ( -10.85938897953544924, -12.23054697885984510, 57.74345952600154419 ) ) ;
#47211=CARTESIAN_POINT ( 'NONE',  ( -16.87480544004084493, -7.378732441012598287, 74.07362965403005717 ) ) ;
#47217=CARTESIAN_POINT ( 'NONE',  ( -23.74454562765497556, -11.67923450027144305, 59.36747125042367657 ) ) ;
#47220=CARTESIAN_POINT ( 'NONE',  ( -9.982716906467198115, -14.44908523835941594, 67.97304809435139816 ) ) ;
#47221=CARTESIAN_POINT ( 'NONE',  ( -11.96084906401204506, -9.743958800322932490, 60.74413413563605957 ) ) ;
#47224=CARTESIAN_POINT ( 'NONE',  ( -24.08977912471840810, -11.48169904069885661, 62.99572364416607684 ) ) ;
#47226=DIRECTION ( 'NONE',  ( 0.4439273849576908515, 0.8960627639203775363, -9.143653603063708001E-17 ) ) ;
#47229=CARTESIAN_POINT ( 'NONE',  ( -11.89179040387956832, -10.43929601004734486, 70.96893105543333036 ) ) ;
#47230=CARTESIAN_POINT ( 'NONE',  ( -19.45448041399064110, -21.50840410520018509, 62.29503609332071079 ) ) ;
#47232=CARTESIAN_POINT ( 'NONE',  ( -12.31380134045779506, -10.02538898168817916, 60.55918086676557976 ) ) ;
#47233=CARTESIAN_POINT ( 'NONE',  ( -12.69763806180496601, -20.04058448603118592, 68.62185382311069759 ) ) ;
#47234=CARTESIAN_POINT ( 'NONE',  ( -23.38560432932743538, -19.27844084936127800, 58.99755287451023378 ) ) ;
#47235=ORIENTED_EDGE ( 'NONE', *, *, #36262, .T. ) ;
#47237=CARTESIAN_POINT ( 'NONE',  ( -24.42398663107514523, -15.65075326911586906, 73.01775867260030850 ) ) ;
#47240=CARTESIAN_POINT ( 'NONE',  ( -21.94214292921110143, -20.15606996381378480, 58.76442870697494669 ) ) ;
#47243=CARTESIAN_POINT ( 'NONE',  ( -10.57990114081760957, -13.11695186304740979, 71.22300718686658172 ) ) ;
#47245=ORIENTED_EDGE ( 'NONE', *, *, #16541, .F. ) ;
#47246=B_SPLINE_CURVE_WITH_KNOTS ( 'NONE', 3,
 ( #44400, #43436, #10182, #33273, #6719, #29126, #44177, #40682, #48082, #21017 ),
 .UNSPECIFIED., .F., .F.,
 ( 4, 2, 2, 2, 4 ),
 ( 0.000000000000000000, 0.2500000000000000000, 0.5000000000000000000, 0.7500000000000000000, 1.000000000000000000 ),
 .UNSPECIFIED. ) ;
#47248=CARTESIAN_POINT ( 'NONE',  ( -10.23610968374255314, -12.85046669463587143, 67.85336945107273721 ) ) ;
#47249=EDGE_CURVE ( 'NONE', #42405, #15728, #11550, .T. ) ;
#47252=CARTESIAN_POINT ( 'NONE',  ( -10.49189908542464700, -16.09426454567519116, 68.26295692486267797 ) ) ;
#47253=EDGE_CURVE ( 'NONE', #6766, #26691, #26818, .T. ) ;
#47254=EDGE_LOOP ( 'NONE', ( #5101, #27171 ) ) ;
#47256=CARTESIAN_POINT ( 'NONE',  ( -24.41403467353552514, -14.40519207544021540, 69.84202309558250477 ) ) ;
#47258=CYLINDRICAL_SURFACE ( 'NONE', #26724, 0.1500000000000081268 ) ;
#47261=CARTESIAN_POINT ( 'NONE',  ( -15.47038646904106329, -21.58309222549749506, 72.34575460768671462 ) ) ;
#47262=EDGE_CURVE ( 'NONE', #1356, #7607, #23852, .T. ) ;
#47263=( BOUNDED_CURVE ( )  B_SPLINE_CURVE ( 3, ( #19809, #27672, #34809, #19550 ),
 .UNSPECIFIED., .F., .F. ) 
 B_SPLINE_CURVE_WITH_KNOTS ( ( 4, 4 ),
 ( 0.000000000000000000, 0.4074455897393669535 ),
 .UNSPECIFIED. ) 
 CURVE ( )  GEOMETRIC_REPRESENTATION_ITEM ( )  RATIONAL_B_SPLINE_CURVE ( ( 1.000000000000000000, 0.4567392136813270276, 0.3561768502900284905, 0.6983129098261043888 ) ) 
 REPRESENTATION_ITEM ( '' )  );
#47264=CARTESIAN_POINT ( 'NONE',  ( -24.45201636468676654, -14.25170757634699825, 69.95275273439749242 ) ) ;
#47265=CARTESIAN_POINT ( 'NONE',  ( -11.43624710438022340, -19.24183451059727545, 71.83685881853561739 ) ) ;
#47267=CYLINDRICAL_SURFACE ( 'NONE', #38518, 0.1500000000000051015 ) ;
#47268=EDGE_LOOP ( 'NONE', ( #9132, #17168 ) ) ;
#47269=CARTESIAN_POINT ( 'NONE',  ( -18.98390459359973548, -7.933620001262258192, 66.91543923465640376 ) ) ;
#47270=CARTESIAN_POINT ( 'NONE',  ( -11.28563465779866526, -19.03109355880862452, 68.35656306278301031 ) ) ;
#47272=CARTESIAN_POINT ( 'NONE',  ( -16.29760673242258306, -22.17363489859456038, 61.87072740723333197 ) ) ;
#47277=CARTESIAN_POINT ( 'NONE',  ( -20.74681640280920192, -8.591282160409747348, 59.84125268094840067 ) ) ;
#47278=CARTESIAN_POINT ( 'NONE',  ( -16.32745258320347759, -21.77369344365219561, 61.77040269689842944 ) ) ;
#47279=ORIENTED_EDGE ( 'NONE', *, *, #29131, .T. ) ;
#47280=( BOUNDED_SURFACE ( )  B_SPLINE_SURFACE ( 3, 1, ( 
 ( #18885, #22332 ),
 ( #11258, #10529 ),
 ( #25535, #37331 ),
 ( #15407, #45252 ),
 ( #3618, #40797 ),
 ( #37576, #10760 ),
 ( #11494, #40548 ) ),
 .UNSPECIFIED., .T., .F., .F. ) 
 B_SPLINE_SURFACE_WITH_KNOTS ( ( 4, 3, 4 ),
 ( 2, 2 ),
 ( 0.000000000000000000, 0.5000000000000000000, 1.000000000000000000 ),
 ( 0.000000000000000000, 1.000000000000000000 ),
 .UNSPECIFIED. ) 
 GEOMETRIC_REPRESENTATION_ITEM ( )  RATIONAL_B_SPLINE_SURFACE ( (
 ( 1.000000000000000000, 1.000000000000000000),
 ( 0.3333333333333335369, 0.3333333333333330373),
 ( 0.3333333333333335369, 0.3333333333333330373),
 ( 1.000000000000000000, 1.000000000000000000),
 ( 0.3333333333333333703, 0.3333333333333333703),
 ( 0.3333333333333333703, 0.3333333333333333703),
 ( 1.000000000000000000, 1.000000000000000000) ) ) 
 REPRESENTATION_ITEM ( '' )  SURFACE ( )  );
#47281=CARTESIAN_POINT ( 'NONE',  ( -19.74037869399712619, -21.88997799075047368, 65.61486212479920255 ) ) ;
#47282=CARTESIAN_POINT ( 'NONE',  ( -20.78451513435706133, -21.00713107796517320, 62.12943504870421663 ) ) ;
#47283=CARTESIAN_POINT ( 'NONE',  ( -23.65624121974494543, -11.51332442490694774, 66.42214514605622355 ) ) ;
#47286=ORIENTED_EDGE ( 'NONE', *, *, #5756, .T. ) ;
#47287=ORIENTED_EDGE ( 'NONE', *, *, #16384, .F. ) ;
#47288=B_SPLINE_CURVE_WITH_KNOTS ( 'NONE', 3,
 ( #14773, #29843, #22703, #37438, #3480, #11126, #7200, #3986, #11364, #18246 ),
 .UNSPECIFIED., .F., .F.,
 ( 4, 2, 2, 2, 4 ),
 ( 0.000000000000000000, 0.2500000000000000000, 0.5000000000000000000, 0.7500000000000000000, 1.000000000000000000 ),
 .UNSPECIFIED. ) ;
#47290=CARTESIAN_POINT ( 'NONE',  ( -23.81770139843839829, -18.63370553473270519, 72.92401558967065966 ) ) ;
#47291=FACE_OUTER_BOUND ( 'NONE', #8466, .T. ) ;
#47293=CARTESIAN_POINT ( 'NONE',  ( -17.71151671804478411, -7.815048565353869492, 60.36595428842180411 ) ) ;
#47294=CARTESIAN_POINT ( 'NONE',  ( -24.90891992605694227, -15.28604896337863472, 53.49999999999994316 ) ) ;
#47296=CARTESIAN_POINT ( 'NONE',  ( -12.48387464686926407, -19.84385436793359503, 68.42837419015026512 ) ) ;
#47297=ADVANCED_FACE ( 'NONE', ( #38490 ), #5024, .T. ) ;
#47299=CARTESIAN_POINT ( 'NONE',  ( -15.74783386771837890, -7.961078896070159061, 70.62461975990308360 ) ) ;
#47301=( BOUNDED_SURFACE ( )  B_SPLINE_SURFACE ( 3, 1, ( 
 ( #32192, #13451 ),
 ( #39080, #13688 ),
 ( #31455, #28732 ),
 ( #28252, #43763 ),
 ( #43523, #43278 ),
 ( #28496, #43022 ),
 ( #24573, #42789 ) ),
 .UNSPECIFIED., .T., .F., .F. ) 
 B_SPLINE_SURFACE_WITH_KNOTS ( ( 4, 3, 4 ),
 ( 2, 2 ),
 ( 0.000000000000000000, 0.5000000000000000000, 1.000000000000000000 ),
 ( 0.000000000000000000, 1.000000000000000000 ),
 .UNSPECIFIED. ) 
 GEOMETRIC_REPRESENTATION_ITEM ( )  RATIONAL_B_SPLINE_SURFACE ( (
 ( 1.000000000000000000, 1.000000000000000000),
 ( 0.3333333333333335369, 0.3333333333333330373),
 ( 0.3333333333333335369, 0.3333333333333330373),
 ( 1.000000000000000000, 1.000000000000000000),
 ( 0.3333333333333333703, 0.3333333333333333703),
 ( 0.3333333333333333703, 0.3333333333333333703),
 ( 1.000000000000000000, 1.000000000000000000) ) ) 
 REPRESENTATION_ITEM ( '' )  SURFACE ( )  );
#47302=VERTEX_POINT ( 'NONE', #22771 ) ;
#47303=FACE_OUTER_BOUND ( 'NONE', #14095, .T. ) ;
#47306=CARTESIAN_POINT ( 'NONE',  ( -12.76547314785493192, -9.517330534081262172, 74.60450883341005124 ) ) ;
#47308=B_SPLINE_CURVE_WITH_KNOTS ( 'NONE', 1,
 ( #25195, #9700 ),
 .UNSPECIFIED., .F., .F.,
 ( 2, 2 ),
 ( 0.000000000000000000, 1.000000000000000000 ),
 .UNSPECIFIED. ) ;
#47309=ORIENTED_EDGE ( 'NONE', *, *, #2472, .T. ) ;
#47311=CARTESIAN_POINT ( 'NONE',  ( -17.49728986656368335, -7.358816873484950172, 63.66401766577892118 ) ) ;
#47312=CARTESIAN_POINT ( 'NONE',  ( -13.88293259567353743, -20.90532631576516565, 68.45625136994867432 ) ) ;
#47315=ORIENTED_EDGE ( 'NONE', *, *, #8829, .F. ) ;
#47317=EDGE_CURVE ( 'NONE', #30116, #3548, #14976, .T. ) ;
#47318=AXIS2_PLACEMENT_3D ( 'NONE', #12059, #2177, #29010 ) ;
#47319=DIRECTION ( 'NONE',  ( 3.840743001415272461E-07, -4.934726759164745929E-06, 0.9999999999877503543 ) ) ;
#47322=CARTESIAN_POINT ( 'NONE',  ( -11.35719102664687874, -18.40077844947705543, 58.09242476654641507 ) ) ;
#47323=EDGE_CURVE ( 'NONE', #37416, #166, #31975, .T. ) ;
#47324=FACE_OUTER_BOUND ( 'NONE', #38194, .T. ) ;
#47325=ORIENTED_EDGE ( 'NONE', *, *, #30311, .F. ) ;
#47327=ORIENTED_EDGE ( 'NONE', *, *, #12961, .T. ) ;
#47329=ORIENTED_EDGE ( 'NONE', *, *, #28283, .F. ) ;
#47331=CARTESIAN_POINT ( 'NONE',  ( -23.31997331754326197, -18.67484999725029127, 69.29931808629288525 ) ) ;
#47333=ORIENTED_EDGE ( 'NONE', *, *, #6617, .F. ) ;
#47335=CARTESIAN_POINT ( 'NONE',  ( -20.17401961043511704, -21.73324369436076964, 72.58195652652476326 ) ) ;
#47336=DIRECTION ( 'NONE',  ( -0.3996021513128670266, -0.9166886716143755054, -9.834836654444679756E-09 ) ) ;
#47337=VECTOR ( 'NONE', #11631, 1000.000000000000000 ) ;
#47338=ADVANCED_FACE ( 'NONE', ( #23747 ), #45219, .T. ) ;
#47339=CARTESIAN_POINT ( 'NONE',  ( -13.74195337878076018, -8.854397186113205365, 57.04138123197974863 ) ) ;
#47341=CARTESIAN_POINT ( 'NONE',  ( -10.40647260758111869, -17.31080661122752673, 61.31776488722727692 ) ) ;
#47342=ORIENTED_EDGE ( 'NONE', *, *, #28571, .T. ) ;
#47343=CARTESIAN_POINT ( 'NONE',  ( -17.59211729576255934, -7.811223397794364587, 63.55057029380298417 ) ) ;
#47345=CARTESIAN_POINT ( 'NONE',  ( -11.81178692268928643, -10.62566621335946770, 74.43885052268630886 ) ) ;
#47346=FACE_OUTER_BOUND ( 'NONE', #27263, .T. ) ;
#47347=CARTESIAN_POINT ( 'NONE',  ( -13.60236376389480384, -20.73382277062339085, 61.80174179654961364 ) ) ;
#47348=B_SPLINE_CURVE_WITH_KNOTS ( 'NONE', 1,
 ( #34974, #23919 ),
 .UNSPECIFIED., .F., .F.,
 ( 2, 2 ),
 ( 0.000000000000000000, 1.000000000000000000 ),
 .UNSPECIFIED. ) ;
#47349=CARTESIAN_POINT ( 'NONE',  ( -19.91150868914413508, -21.83174586793584382, 69.04208316193926009 ) ) ;
#47350=EDGE_CURVE ( 'NONE', #15944, #8174, #6526, .T. ) ;
#47351=CARTESIAN_POINT ( 'NONE',  ( -11.89178903705324686, -10.43929771899554737, 71.26893105542536944 ) ) ;
#47352=ORIENTED_EDGE ( 'NONE', *, *, #1209, .F. ) ;
#47353=VERTEX_POINT ( 'NONE', #27663 ) ;
#47354=CARTESIAN_POINT ( 'NONE',  ( -20.72253465480533308, -21.04901898548487793, 65.72887014617839441 ) ) ;
#47357=CARTESIAN_POINT ( 'NONE',  ( -10.37172597770583415, -14.90377323363781414, 71.21294082064301278 ) ) ;
#47359=CARTESIAN_POINT ( 'NONE',  ( -17.91451193640577344, -22.24313339626381847, 61.99040498927033127 ) ) ;
#47360=CARTESIAN_POINT ( 'NONE',  ( -18.97948276208418150, -7.924750873940990203, 60.11659987143988815 ) ) ;
#47361=CARTESIAN_POINT ( 'NONE',  ( -21.17774041181681710, -8.837307456416409579, 73.80948465004701120 ) ) ;
#47362=ORIENTED_EDGE ( 'NONE', *, *, #18725, .F. ) ;
#47363=CARTESIAN_POINT ( 'NONE',  ( -17.26571734983926021, -20.32036725976781355, 53.88362224778186516 ) ) ;
#47364=CARTESIAN_POINT ( 'NONE',  ( -17.06879511326789611, -7.767867012253359071, 73.97490359703523666 ) ) ;
#47366=ORIENTED_EDGE ( 'NONE', *, *, #30908, .T. ) ;
#47370=CARTESIAN_POINT ( 'NONE',  ( -10.42546210075913748, -12.25520342886974845, 57.44361899967025664 ) ) ;
#47371=CARTESIAN_POINT ( 'NONE',  ( -13.85515746416932004, -20.83112733177175713, 65.05916827336410790 ) ) ;
#47372=CARTESIAN_POINT ( 'NONE',  ( -11.57411172585599424, -10.96269881181310701, 57.43733183567105982 ) ) ;
#47373=ORIENTED_EDGE ( 'NONE', *, *, #36866, .T. ) ;
#47376=CARTESIAN_POINT ( 'NONE',  ( -10.91676103024768985, -17.53123951026858407, 64.62739371368721208 ) ) ;
#47377=CARTESIAN_POINT ( 'NONE',  ( -10.37497031036790851, -14.69804325442274617, 71.47782692816423378 ) ) ;
#47378=( BOUNDED_CURVE ( )  B_SPLINE_CURVE ( 3, ( #147, #15129, #30186, #37792 ),
 .UNSPECIFIED., .F., .F. ) 
 B_SPLINE_CURVE_WITH_KNOTS ( ( 4, 4 ),
 ( 0.4074455897393610693, 0.5000000000000000000 ),
 .UNSPECIFIED. ) 
 CURVE ( )  GEOMETRIC_REPRESENTATION_ITEM ( )  RATIONAL_B_SPLINE_CURVE ( ( 0.6983129098260949519, 0.7760317562606977582, 0.8765941196519987377, 0.9999999999999965583 ) ) 
 REPRESENTATION_ITEM ( '' )  );
#47379=B_SPLINE_CURVE_WITH_KNOTS ( 'NONE', 1,
 ( #26811, #27283 ),
 .UNSPECIFIED., .F., .F.,
 ( 2, 2 ),
 ( 0.000000000000000000, 1.000000000000000000 ),
 .UNSPECIFIED. ) ;
#47380=ADVANCED_FACE ( 'NONE', ( #16803 ), #13105, .T. ) ;
#47381=CARTESIAN_POINT ( 'NONE',  ( -14.14027996024632117, -8.627251641784368985, 70.83843686035393716 ) ) ;
#47382=CARTESIAN_POINT ( 'NONE',  ( -13.90805003106573068, -20.86209311441256986, 68.75625137331327608 ) ) ;
#47386=EDGE_LOOP ( 'NONE', ( #28096, #32152, #45727, #18551, #29306 ) ) ;
#47387=CARTESIAN_POINT ( 'NONE',  ( -18.00016368654587851, -22.23706993494688788, 62.03569299701934625 ) ) ;
#47388=CARTESIAN_POINT ( 'NONE',  ( -12.96069280291159309, -9.414713786589372191, 74.50850143233944323 ) ) ;
#47390=FACE_OUTER_BOUND ( 'NONE', #46217, .T. ) ;
#47391=CARTESIAN_POINT ( 'NONE',  ( -12.16754818860568932, -19.43427171616090376, 58.11609390261931196 ) ) ;
#47393=FACE_OUTER_BOUND ( 'NONE', #2698, .T. ) ;
#47394=CARTESIAN_POINT ( 'NONE',  ( -24.39774143530919304, -13.72145442755526545, 73.27838554735291154 ) ) ;
#47395=DIRECTION ( 'NONE',  ( -0.7658821528503489962, -0.6346126762488695228, 0.1033986416233894090 ) ) ;
#47397=ORIENTED_EDGE ( 'NONE', *, *, #27944, .T. ) ;
#47398=CARTESIAN_POINT ( 'NONE',  ( -22.27803375191225399, -20.46189896727856095, 62.42094464928214848 ) ) ;
#47399=DIRECTION ( 'NONE',  ( -4.116680906418232674E-07, -3.835121148322460978E-07, -0.9999999999998417932 ) ) ;
#47400=EDGE_CURVE ( 'NONE', #38546, #33912, #36984, .T. ) ;
#47401=CARTESIAN_POINT ( 'NONE',  ( -19.78055771692377363, -21.45376424143257310, 68.93482482294113822 ) ) ;
#47402=B_SPLINE_CURVE_WITH_KNOTS ( 'NONE', 3,
 ( #1955, #35439, #13743, #17202, #16717, #28786, #40121, #1724, #18659, #22616 ),
 .UNSPECIFIED., .F., .F.,
 ( 4, 2, 2, 2, 4 ),
 ( 0.1272669073658322658, 0.2522669073463165712, 0.3772669073268009043, 0.5022669073072851820, 0.6272669072877694596 ),
 .UNSPECIFIED. ) ;
#47404=EDGE_CURVE ( 'NONE', #41130, #46821, #42044, .T. ) ;
#47406=FACE_OUTER_BOUND ( 'NONE', #23595, .T. ) ;
#47409=ORIENTED_EDGE ( 'NONE', *, *, #31798, .F. ) ;
#47415=ORIENTED_EDGE ( 'NONE', *, *, #40294, .T. ) ;
#47416=ORIENTED_EDGE ( 'NONE', *, *, #21152, .F. ) ;
#47417=EDGE_LOOP ( 'NONE', ( #15100, #4608 ) ) ;
#47419=DIRECTION ( 'NONE',  ( -0.6538427738826437796, -0.7566304428460742804, 5.916677973164435741E-08 ) ) ;
#47420=( BOUNDED_SURFACE ( )  B_SPLINE_SURFACE ( 3, 1, ( 
 ( #45276, #37360 ),
 ( #10789, #41569 ),
 ( #18651, #48706 ),
 ( #22131, #34161 ),
 ( #3399, #3645 ),
 ( #11523, #456 ),
 ( #14947, #30007 ) ),
 .UNSPECIFIED., .T., .F., .F. ) 
 B_SPLINE_SURFACE_WITH_KNOTS ( ( 4, 3, 4 ),
 ( 2, 2 ),
 ( 0.000000000000000000, 0.5000000000000000000, 1.000000000000000000 ),
 ( 0.000000000000000000, 1.000000000000000000 ),
 .UNSPECIFIED. ) 
 GEOMETRIC_REPRESENTATION_ITEM ( )  RATIONAL_B_SPLINE_SURFACE ( (
 ( 1.000000000000000000, 1.000000000000000000),
 ( 0.3333333333333335369, 0.3333333333333330373),
 ( 0.3333333333333335369, 0.3333333333333330373),
 ( 1.000000000000000000, 1.000000000000000000),
 ( 0.3333333333333333703, 0.3333333333333333703),
 ( 0.3333333333333333703, 0.3333333333333333703),
 ( 1.000000000000000000, 1.000000000000000000) ) ) 
 REPRESENTATION_ITEM ( '' )  SURFACE ( )  );
#47421=CARTESIAN_POINT ( 'NONE',  ( -16.07865109465781117, -7.939724484389961034, 63.97011030347106697 ) ) ;
#47423=ORIENTED_EDGE ( 'NONE', *, *, #7123, .T. ) ;
#47425=B_SPLINE_CURVE_WITH_KNOTS ( 'NONE', 3,
 ( #28212, #31905, #32154, #13887, #24769, #24537, #17829, #21063, #28929, #36066 ),
 .UNSPECIFIED., .F., .F.,
 ( 4, 2, 2, 2, 4 ),
 ( 0.000000000000000000, 0.2500000000000000000, 0.5000000000000000000, 0.7500000000000000000, 1.000000000000000000 ),
 .UNSPECIFIED. ) ;
#47427=EDGE_CURVE ( 'NONE', #17956, #29624, #9446, .T. ) ;
#47428=CARTESIAN_POINT ( 'NONE',  ( -20.72450927900464634, -21.03929139025762751, 58.93003081252663833 ) ) ;
#47429=CARTESIAN_POINT ( 'NONE',  ( -23.23831428902490259, -18.70736991730898424, 65.83891806926222046 ) ) ;
#47431=( BOUNDED_CURVE ( )  B_SPLINE_CURVE ( 3, ( #40416, #47573, #40185, #33006 ),
 .UNSPECIFIED., .F., .F. ) 
 B_SPLINE_CURVE_WITH_KNOTS ( ( 4, 4 ),
 ( 4.712388980384690562, 4.921828490624011287 ),
 .UNSPECIFIED. ) 
 CURVE ( )  GEOMETRIC_REPRESENTATION_ITEM ( )  RATIONAL_B_SPLINE_CURVE ( ( 1.000000000000000000, 0.9963479302455154896, 0.9963479302455154896, 1.000000000000000000 ) ) 
 REPRESENTATION_ITEM ( '' )  );
#47433=CARTESIAN_POINT ( 'NONE',  ( -10.37382936219775154, -14.83089353207902228, 74.81251018390588570 ) ) ;
#47434=EDGE_CURVE ( 'NONE', #29684, #26512, #34992, .T. ) ;
#47441=CARTESIAN_POINT ( 'NONE',  ( -22.48237781098097798, -19.73147542146173450, 65.85988959519353614 ) ) ;
#47445=CARTESIAN_POINT ( 'NONE',  ( -18.48574975592938330, -21.77885183246672796, 72.28510966583125708 ) ) ;
#47446=DIRECTION ( 'NONE',  ( 0.9441784275685842776, -0.3294345108122635479, -1.993146885056044100E-08 ) ) ;
#47449=FACE_OUTER_BOUND ( 'NONE', #20317, .T. ) ;
#47450=EDGE_LOOP ( 'NONE', ( #39190, #37217, #475, #37820, #46237 ) ) ;
#47451=CARTESIAN_POINT ( 'NONE',  ( -13.49267557974227394, -8.956801037788498121, 60.45422421514565059 ) ) ;
#47452=CARTESIAN_POINT ( 'NONE',  ( -9.983332390312334326, -14.43496380782568522, 68.01946623190198693 ) ) ;
#47454=EDGE_CURVE ( 'NONE', #36141, #23362, #24472, .T. ) ;
#47455=EDGE_CURVE ( 'NONE', #5810, #18099, #5257, .T. ) ;
#47456=DIRECTION ( 'NONE',  ( -0.9132646967824438189, 0.4073666574609055568, -8.344532079829881716E-09 ) ) ;
#47457=CARTESIAN_POINT ( 'NONE',  ( -13.93897074462874919, -20.93787812888889377, 68.74153005185598886 ) ) ;
#47458=CARTESIAN_POINT ( 'NONE',  ( -16.94458744105653381, -7.374567917109038362, 74.14513580114275726 ) ) ;
#47459=CARTESIAN_POINT ( 'NONE',  ( -21.17797108042288912, -21.24447908004819041, 65.76266720218958994 ) ) ;
#47462=CARTESIAN_POINT ( 'NONE',  ( -19.05423358200063433, -7.539568773092505616, 67.06218330876637879 ) ) ;
#47463=FACE_OUTER_BOUND ( 'NONE', #35233, .T. ) ;
#47464=ORIENTED_EDGE ( 'NONE', *, *, #9405, .F. ) ;
#47465=CARTESIAN_POINT ( 'NONE',  ( -23.97453657302211028, -17.42552933921582436, 62.68181000447317786 ) ) ;
#47466=ADVANCED_FACE ( 'NONE', ( #31605 ), #47070, .T. ) ;
#47467=EDGE_CURVE ( 'NONE', #46391, #27633, #21493, .T. ) ;
#47469=ORIENTED_EDGE ( 'NONE', *, *, #20495, .T. ) ;
#47470=ORIENTED_EDGE ( 'NONE', *, *, #10979, .F. ) ;
#47471=ADVANCED_FACE ( 'NONE', ( #11131 ), #8389, .T. ) ;
#47472=CARTESIAN_POINT ( 'NONE',  ( -23.40706704545067041, -18.44294168544361057, 72.76368236816873036 ) ) ;
#47474=CARTESIAN_POINT ( 'NONE',  ( -15.95707209241614422, -7.504986913482371236, 63.85506412386598640 ) ) ;
#47477=CARTESIAN_POINT ( 'NONE',  ( -10.53536195276627829, -13.30851587854854401, 74.69289754060230280 ) ) ;
#47478=CARTESIAN_POINT ( 'NONE',  ( -24.25486363958986757, -13.06355980472538469, 63.11792038370487035 ) ) ;
#47479=CARTESIAN_POINT ( 'NONE',  ( -14.93036899495222869, -8.267093141589578309, 60.54826067984155458 ) ) ;
#47481=CARTESIAN_POINT ( 'NONE',  ( -13.83108299072750391, -21.33561835983412891, 72.04112301026525245 ) ) ;
#47482=EDGE_LOOP ( 'NONE', ( #985, #12763, #44033, #24812, #19485 ) ) ;
#47485=ADVANCED_FACE ( 'NONE', ( #3738 ), #13403, .T. ) ;
#47487=CARTESIAN_POINT ( 'NONE',  ( -17.00410685006708178, -7.771727545396207582, 73.96018273221115180 ) ) ;
#47488=CARTESIAN_POINT ( 'NONE',  ( -14.80261092528313327, -21.30118148935308042, 61.86430222708096949 ) ) ;
#47489=DIRECTION ( 'NONE',  ( 0.4749924142254752790, 0.8799898899579782219, 8.916637575808904455E-09 ) ) ;
#47490=CARTESIAN_POINT ( 'NONE',  ( -11.10552337692560876, -11.79633671024259911, 71.38860856928842225 ) ) ;
#47492=VERTEX_POINT ( 'NONE', #36478 ) ;
#47493=CARTESIAN_POINT ( 'NONE',  ( -20.16691211377460391, -21.73601867580754288, 72.58974061177721637 ) ) ;
#47494=CARTESIAN_POINT ( 'NONE',  ( -19.98813040044048606, -21.37641421727040125, 72.40478737316021807 ) ) ;
#47496=CARTESIAN_POINT ( 'NONE',  ( -10.51631473918724780, -16.23308084970759069, 67.86278957288837432 ) ) ;
#47497=ORIENTED_EDGE ( 'NONE', *, *, #30594, .F. ) ;
#47498=CARTESIAN_POINT ( 'NONE',  ( -13.47245494993759607, -21.12492725511472003, 65.10133600691351319 ) ) ;
#47503=ORIENTED_EDGE ( 'NONE', *, *, #46637, .F. ) ;
#47504=CARTESIAN_POINT ( 'NONE',  ( -19.24025795797341942, -7.996846695050864540, 60.24620885950562865 ) ) ;
#47505=ORIENTED_EDGE ( 'NONE', *, *, #33405, .T. ) ;
#47507=B_SPLINE_CURVE_WITH_KNOTS ( 'NONE', 1,
 ( #25802, #22121 ),
 .UNSPECIFIED., .F., .F.,
 ( 2, 2 ),
 ( 0.000000000000000000, 1.000000000000000000 ),
 .UNSPECIFIED. ) ;
#47509=CARTESIAN_POINT ( 'NONE',  ( -11.28985232898421742, -19.03713839270133690, 68.39502420285157314 ) ) ;
#47510=ORIENTED_EDGE ( 'NONE', *, *, #7232, .T. ) ;
#47511=EDGE_CURVE ( 'NONE', #7864, #26003, #2118, .T. ) ;
#47512=CARTESIAN_POINT ( 'NONE',  ( -23.08280660609100110, -10.60377317445056811, 59.61675562601556067 ) ) ;
#47515=ORIENTED_EDGE ( 'NONE', *, *, #42408, .T. ) ;
#47518=CARTESIAN_POINT ( 'NONE',  ( -23.89200535028185612, -11.11192396016905448, 70.07706043178237110 ) ) ;
#47519=EDGE_LOOP ( 'NONE', ( #15653, #9376, #31423, #38309, #27349 ) ) ;
#47520=DIRECTION ( 'NONE',  ( 0.6562885720885137664, -0.7545099801500438907, -1.193821365372358186E-08 ) ) ;
#47522=CARTESIAN_POINT ( 'NONE',  ( -12.05483347687720475, -10.31798811457585963, 67.79896870046731294 ) ) ;
#47523=CARTESIAN_POINT ( 'NONE',  ( -23.24618082141521214, -10.81943526098172548, 59.74636554153219237 ) ) ;
#47524=ORIENTED_EDGE ( 'NONE', *, *, #25919, .T. ) ;
#47526=EDGE_CURVE ( 'NONE', #6762, #1918, #48541, .T. ) ;
#47528=CARTESIAN_POINT ( 'NONE',  ( -14.97035482569482312, -21.41873484682592377, 61.92128389535452015 ) ) ;
#47530=CARTESIAN_POINT ( 'NONE',  ( -17.71116635333902778, -7.815035665054884007, 60.09563220684449192 ) ) ;
#47532=EDGE_CURVE ( 'NONE', #41905, #35459, #20356, .T. ) ;
#47533=CARTESIAN_POINT ( 'NONE',  ( -24.08907123645992243, -11.48026457312919391, 63.13713595337925000 ) ) ;
#47535=CARTESIAN_POINT ( 'NONE',  ( -23.70394581819067170, -18.81767069530084058, 69.41559189047532641 ) ) ;
#47536=ORIENTED_EDGE ( 'NONE', *, *, #22040, .T. ) ;
#47537=CARTESIAN_POINT ( 'NONE',  ( -16.39155704513022016, -21.78318439201321866, 61.75568132354042916 ) ) ;
#47538=CARTESIAN_POINT ( 'NONE',  ( -20.70232472158584969, -8.624289250480600799, 59.84125250310036392 ) ) ;
#47541=EDGE_CURVE ( 'NONE', #32972, #29603, #39714, .T. ) ;
#47542=VERTEX_POINT ( 'NONE', #34746 ) ;
#47544=VERTEX_POINT ( 'NONE', #34246 ) ;
#47546=CARTESIAN_POINT ( 'NONE',  ( -24.87453101240845399, -14.74101577129048835, 62.89951734912977344 ) ) ;
#47550=( BOUNDED_CURVE ( )  B_SPLINE_CURVE ( 3, ( #35024, #23239, #37993, #23965 ),
 .UNSPECIFIED., .F., .F. ) 
 B_SPLINE_CURVE_WITH_KNOTS ( ( 4, 4 ),
 ( 0.000000000000000000, 0.4074455897393653991 ),
 .UNSPECIFIED. ) 
 CURVE ( )  GEOMETRIC_REPRESENTATION_ITEM ( )  RATIONAL_B_SPLINE_CURVE ( ( 1.000000000000000000, 0.4567392136813279713, 0.3561768502900288236, 0.6983129098261023904 ) ) 
 REPRESENTATION_ITEM ( '' )  );
#47551=ORIENTED_EDGE ( 'NONE', *, *, #46810, .T. ) ;
#47552=CARTESIAN_POINT ( 'NONE',  ( -23.79034794155987598, -17.71981930740736999, 59.28913082385783895 ) ) ;
#47553=ORIENTED_EDGE ( 'NONE', *, *, #23329, .T. ) ;
#47555=CARTESIAN_POINT ( 'NONE',  ( -19.73055724314207282, -21.89319082171075337, 65.66497415329939713 ) ) ;
#47556=CARTESIAN_POINT ( 'NONE',  ( -15.75511905958810033, -8.011018546364985227, 67.21295221587696744 ) ) ;
#47557=EDGE_CURVE ( 'NONE', #22189, #6093, #23685, .T. ) ;
#47559=( BOUNDED_CURVE ( )  B_SPLINE_CURVE ( 3, ( #38632, #26587, #41606, #12289 ),
 .UNSPECIFIED., .F., .F. ) 
 B_SPLINE_CURVE_WITH_KNOTS ( ( 4, 4 ),
 ( 0.5000000000000000000, 0.9074455897393673975 ),
 .UNSPECIFIED. ) 
 CURVE ( )  GEOMETRIC_REPRESENTATION_ITEM ( )  RATIONAL_B_SPLINE_CURVE ( ( 1.000000000000042411, 0.4567392136813354098, 0.3561768502900019562, 0.6983129098260876244 ) ) 
 REPRESENTATION_ITEM ( '' )  );
#47561=VERTEX_POINT ( 'NONE', #12338 ) ;
#47562=FACE_OUTER_BOUND ( 'NONE', #5016, .T. ) ;
#47563=DIRECTION ( 'NONE',  ( 4.734277565933067533E-07, -1.363385193985295737E-06, -0.9999999999989586108 ) ) ;
#47564=DIRECTION ( 'NONE',  ( 0.5327540375067998379, 0.8462701315302333382, 7.203825861310634525E-08 ) ) ;
#47565=ORIENTED_EDGE ( 'NONE', *, *, #42342, .F. ) ;
#47566=CARTESIAN_POINT ( 'NONE',  ( -15.15660932275500272, -21.48492473237050859, 65.39124617759186719 ) ) ;
#47567=B_SPLINE_CURVE_WITH_KNOTS ( 'NONE', 3,
 ( #40522, #30201, #11464, #6800, #46178, #9000, #24023, #23052, #23536, #20071 ),
 .UNSPECIFIED., .F., .F.,
 ( 4, 2, 2, 2, 4 ),
 ( 0.000000000000000000, 0.2500000000000000000, 0.5000000000000000000, 0.7500000000000000000, 1.000000000000000000 ),
 .UNSPECIFIED. ) ;
#47569=DIRECTION ( 'NONE',  ( 3.811252424767960347E-06, 6.838859004561632622E-06, 0.9999999999693520714 ) ) ;
#47570=CARTESIAN_POINT ( 'NONE',  ( -11.64235026963700115, -18.84330375823651949, 68.21689631561287115 ) ) ;
#47571=B_SPLINE_CURVE_WITH_KNOTS ( 'NONE', 1,
 ( #19896, #34903 ),
 .UNSPECIFIED., .F., .F.,
 ( 2, 2 ),
 ( 0.000000000000000000, 1.000000000000000000 ),
 .UNSPECIFIED. ) ;
#47572=ORIENTED_EDGE ( 'NONE', *, *, #43538, .F. ) ;
#47573=CARTESIAN_POINT ( 'NONE',  ( -12.02413026160302323, -13.69638637514736956, 53.69233794759168887 ) ) ;
#47575=DIRECTION ( 'NONE',  ( 4.615129112206533859E-07, -1.699487772732772144E-08, 0.9999999999998934186 ) ) ;
#47576=CARTESIAN_POINT ( 'NONE',  ( -22.66983630878679179, -20.09927642381470747, 69.27394370987401828 ) ) ;
#47578=CARTESIAN_POINT ( 'NONE',  ( -13.26809664353323726, -20.51382390604332784, 61.66079502706314486 ) ) ;
#47581=ORIENTED_EDGE ( 'NONE', *, *, #18715, .T. ) ;
#47582=ORIENTED_EDGE ( 'NONE', *, *, #22100, .F. ) ;
#47584=CARTESIAN_POINT ( 'NONE',  ( -22.70923626323604694, -10.21920355281058157, 66.82716892541095888 ) ) ;
#47585=FACE_OUTER_BOUND ( 'NONE', #20856, .T. ) ;
#47586=VERTEX_POINT ( 'NONE', #16015 ) ;
#47588=CARTESIAN_POINT ( 'NONE',  ( -13.49409790474204840, -20.66256726344224504, 61.53118467422925164 ) ) ;
#47590=CARTESIAN_POINT ( 'NONE',  ( -13.12535629923256941, -9.217633289312832545, 71.26414145609075490 ) ) ;
#47592=EDGE_CURVE ( 'NONE', #9250, #38102, #41900, .T. ) ;
#47593=CARTESIAN_POINT ( 'NONE',  ( -12.00744322407076226, -19.92521668911118482, 61.58333889064303435 ) ) ;
#47594=VERTEX_POINT ( 'NONE', #31059 ) ;
#47595=FACE_BOUND ( 'NONE', #18730, .T. ) ;
#47597=CARTESIAN_POINT ( 'NONE',  ( -10.42366005825797792, -14.81678892838547767, 75.08162374473462819 ) ) ;
#47598=ADVANCED_FACE ( 'NONE', ( #30589 ), #45613, .F. ) ;
#47600=EDGE_LOOP ( 'NONE', ( #36879, #8011 ) ) ;
#47601=DIRECTION ( 'NONE',  ( -0.4007314504464637439, 0.1985303619678204790, 0.8944271909999157444 ) ) ;
#47603=EDGE_CURVE ( 'NONE', #5915, #10474, #38573, .T. ) ;
#47604=CARTESIAN_POINT ( 'NONE',  ( -13.33887460415658133, -9.124795780406598666, 63.90946578472572526 ) ) ;
#47606=ADVANCED_FACE ( 'NONE', ( #38428 ), #38683, .T. ) ;
#47607=CARTESIAN_POINT ( 'NONE',  ( -11.05034076241727625, -11.79557573020262318, 71.37388789199357575 ) ) ;
#47608=ORIENTED_EDGE ( 'NONE', *, *, #4430, .F. ) ;
#47609=ORIENTED_EDGE ( 'NONE', *, *, #20845, .F. ) ;
#47611=CARTESIAN_POINT ( 'NONE',  ( -10.83536383905390998, -17.31742040078651357, 64.62739380450889826 ) ) ;
#47612=CARTESIAN_POINT ( 'NONE',  ( -24.03078312051908227, -17.12275678261753953, 69.64013211569611883 ) ) ;
#47616=CARTESIAN_POINT ( 'NONE',  ( -16.02453559203015132, -22.12732798260191913, 58.47240968810538675 ) ) ;
#47617=ORIENTED_EDGE ( 'NONE', *, *, #19176, .F. ) ;
#47618=CARTESIAN_POINT ( 'NONE',  ( -14.28913879486226435, -8.050816564744696535, 67.37479651646088996 ) ) ;
#47619=CARTESIAN_POINT ( 'NONE',  ( -23.19916440516392697, -19.59445054535707698, 54.27966884056655061 ) ) ;
#47621=CARTESIAN_POINT ( 'NONE',  ( -18.98390459359973548, -7.933620001262258192, 66.91543923465640376 ) ) ;
#47623=CARTESIAN_POINT ( 'NONE',  ( -18.53748367693119192, -21.77439179387026869, 69.02334521062161343 ) ) ;
#47624=VERTEX_POINT ( 'NONE', #45845 ) ;
#47626=CARTESIAN_POINT ( 'NONE',  ( -23.83043773139749533, -11.86620498678314561, 59.78235732590890450 ) ) ;
#47627=ORIENTED_EDGE ( 'NONE', *, *, #27493, .T. ) ;
#47628=CARTESIAN_POINT ( 'NONE',  ( -10.93244803288776090, -12.03909807633519513, 71.24428013274216198 ) ) ;
#47629=FACE_OUTER_BOUND ( 'NONE', #45354, .T. ) ;
#47630=CARTESIAN_POINT ( 'NONE',  ( -24.41553149706675896, -15.71832598455623398, 69.81835354388927328 ) ) ;
#47631=CARTESIAN_POINT ( 'NONE',  ( -22.22619359738691003, -20.50513629785891823, 58.94938195453792673 ) ) ;
#47632=ORIENTED_EDGE ( 'NONE', *, *, #20338, .F. ) ;
#47634=EDGE_CURVE ( 'NONE', #9616, #26173, #44433, .T. ) ;
#47636=B_SPLINE_CURVE_WITH_KNOTS ( 'NONE', 3,
 ( #12033, #15703, #23356, #4637, #30991, #4170, #19172, #26315, #8585, #37624 ),
 .UNSPECIFIED., .F., .F.,
 ( 4, 2, 2, 2, 4 ),
 ( 0.6272669072877713470, 0.7522669073072923984, 0.8772669073268133388, 1.002266907346334390, 1.127266907365855442 ),
 .UNSPECIFIED. ) ;
#47639=CARTESIAN_POINT ( 'NONE',  ( -16.71219989829967645, -22.22520177033091926, 68.81065352759269160 ) ) ;
#47640=FACE_OUTER_BOUND ( 'NONE', #46780, .T. ) ;
#47641=ORIENTED_EDGE ( 'NONE', *, *, #16105, .F. ) ;
#47643=CARTESIAN_POINT ( 'NONE',  ( -14.29546348963859437, -8.047845817433223914, 67.43787819521311633 ) ) ;
#47644=CARTESIAN_POINT ( 'NONE',  ( -13.41327670018355001, -20.54622194888242603, 58.34650078082590596 ) ) ;
#47645=EDGE_LOOP ( 'NONE', ( #33309, #44158 ) ) ;
#47646=EDGE_CURVE ( 'NONE', #14265, #30719, #6227, .T. ) ;
#47647=ORIENTED_EDGE ( 'NONE', *, *, #40411, .F. ) ;
#47648=ORIENTED_EDGE ( 'NONE', *, *, #44305, .T. ) ;
#47650=EDGE_CURVE ( 'NONE', #4523, #4476, #1507, .T. ) ;
#47651=CARTESIAN_POINT ( 'NONE',  ( -23.75246069176763442, -11.81711528745043971, 59.49738212070109711 ) ) ;
#47652=CARTESIAN_POINT ( 'NONE',  ( -23.04367457972577427, -10.55211693511195215, 59.75203429192391269 ) ) ;
#47653=CARTESIAN_POINT ( 'NONE',  ( -13.22576123393696967, -9.135673809461350103, 70.99358371225501685 ) ) ;
#47654=VERTEX_POINT ( 'NONE', #1980 ) ;
#47655=ORIENTED_EDGE ( 'NONE', *, *, #15039, .F. ) ;
#47658=CARTESIAN_POINT ( 'NONE',  ( -10.84060798775485246, -17.18797739218483400, 61.17245566960979630 ) ) ;
#47660=EDGE_CURVE ( 'NONE', #39323, #24815, #17847, .T. ) ;
#47663=EDGE_CURVE ( 'NONE', #21219, #26756, #25569, .T. ) ;
#47664=EDGE_CURVE ( 'NONE', #40988, #3865, #12547, .T. ) ;
#47666=CARTESIAN_POINT ( 'NONE',  ( -24.41553149706675896, -15.71832598455623398, 69.81835354388927328 ) ) ;
#47671=ORIENTED_EDGE ( 'NONE', *, *, #17309, .F. ) ;
#47673=CARTESIAN_POINT ( 'NONE',  ( -21.36489679027069499, -8.963475500412677377, 73.60128753237400190 ) ) ;
#47674=CARTESIAN_POINT ( 'NONE',  ( -22.38767768884900988, -19.81996202295057330, 65.58933089874275879 ) ) ;
#47676=CARTESIAN_POINT ( 'NONE',  ( -19.44222556512714917, -7.637678758653525968, 60.21738930846358073 ) ) ;
#47678=CARTESIAN_POINT ( 'NONE',  ( -21.03177576320737785, -20.86624375009474974, 65.88453921249779910 ) ) ;
#47681=FACE_OUTER_BOUND ( 'NONE', #28149, .T. ) ;
#47684=VERTEX_POINT ( 'NONE', #38923 ) ;
#47685=CARTESIAN_POINT ( 'NONE',  ( -13.20291541311068961, -8.670452210032964402, 60.53926637877078321 ) ) ;
#47686=PLANE ( 'NONE',  #21604 ) ;
#47689=CARTESIAN_POINT ( 'NONE',  ( -23.19948571119275726, -18.85291137746750323, 65.83861571032234394 ) ) ;
#47690=ORIENTED_EDGE ( 'NONE', *, *, #44679, .F. ) ;
#47692=CARTESIAN_POINT ( 'NONE',  ( -14.78766009005058635, -21.34800739930362568, 58.45145834864037937 ) ) ;
#47693=( BOUNDED_CURVE ( )  B_SPLINE_CURVE ( 3, ( #44022, #9793, #14402, #24807 ),
 .UNSPECIFIED., .F., .F. ) 
 B_SPLINE_CURVE_WITH_KNOTS ( ( 4, 4 ),
 ( 0.4074455897393646220, 0.5000000000000000000 ),
 .UNSPECIFIED. ) 
 CURVE ( )  GEOMETRIC_REPRESENTATION_ITEM ( )  RATIONAL_B_SPLINE_CURVE ( ( 0.6983129098260960621, 0.7760317562607046415, 0.8765941196520070644, 1.000000000000005995 ) ) 
 REPRESENTATION_ITEM ( '' )  );
#47695=VERTEX_POINT ( 'NONE', #47041 ) ;
#47696=CARTESIAN_POINT ( 'NONE',  ( -11.22571687057108036, -18.94262312776799106, 64.90740396756440589 ) ) ;
#47697=CARTESIAN_POINT ( 'NONE',  ( -24.68398957063837074, -13.13362340124566785, 63.01919566578877152 ) ) ;
#47698=ORIENTED_EDGE ( 'NONE', *, *, #38080, .F. ) ;
#47700=CARTESIAN_POINT ( 'NONE',  ( -15.69736356130078647, -8.025520047610617880, 70.90989840317035942 ) ) ;
#47702=CARTESIAN_POINT ( 'NONE',  ( -10.53536195276627829, -13.30851587854854579, 74.69289754060230280 ) ) ;
#47703=CARTESIAN_POINT ( 'NONE',  ( -24.80769062643263467, -15.80232089486973557, 69.71802876059763321 ) ) ;
#47705=CARTESIAN_POINT ( 'NONE',  ( -12.49855684652675514, -19.85736664535339813, 68.75146050727752822 ) ) ;
#47706=CARTESIAN_POINT ( 'NONE',  ( -17.80019921555161844, -7.368697419278031902, 60.28049549549236019 ) ) ;
#47707=( BOUNDED_CURVE ( )  B_SPLINE_CURVE ( 3, ( #31005, #42087, #15962, #7884 ),
 .UNSPECIFIED., .F., .F. ) 
 B_SPLINE_CURVE_WITH_KNOTS ( ( 4, 4 ),
 ( 0.000000000000000000, 0.4074455897393600701 ),
 .UNSPECIFIED. ) 
 CURVE ( )  GEOMETRIC_REPRESENTATION_ITEM ( )  RATIONAL_B_SPLINE_CURVE ( ( 1.000000000000000000, 0.4567392136813371861, 0.3561768502900322653, 0.6983129098260852929 ) ) 
 REPRESENTATION_ITEM ( '' )  );
#47713=CARTESIAN_POINT ( 'NONE',  ( -23.06976681795876161, -9.947994002224390897, 66.70215612779006165 ) ) ;
#47714=FACE_OUTER_BOUND ( 'NONE', #13695, .T. ) ;
#47717=CARTESIAN_POINT ( 'NONE',  ( -11.05952341788191617, -11.89506116984398609, 71.27964083260611972 ) ) ;
#47720=EDGE_CURVE ( 'NONE', #27190, #23362, #22607, .T. ) ;
#47721=EDGE_CURVE ( 'NONE', #23748, #38000, #31542, .T. ) ;
#47722=CARTESIAN_POINT ( 'NONE',  ( -21.95894734753736088, -20.14334337125395180, 62.46269013518474367 ) ) ;
#47725=CARTESIAN_POINT ( 'NONE',  ( -18.13032352084594478, -22.22571048536470428, 65.45258006234271875 ) ) ;
#47726=ORIENTED_EDGE ( 'NONE', *, *, #37842, .T. ) ;
#47729=CARTESIAN_POINT ( 'NONE',  ( -13.99854101903132531, -20.98015058628177698, 65.14195714266269022 ) ) ;
#47731=CYLINDRICAL_SURFACE ( 'NONE', #32987, 0.1499999999999971079 ) ;
#47732=ORIENTED_EDGE ( 'NONE', *, *, #1987, .T. ) ;
#47733=CARTESIAN_POINT ( 'NONE',  ( -22.96484172783137012, -19.08706962207428504, 58.88410642316259214 ) ) ;
#47734=VECTOR ( 'NONE', #9024, 999.9999999999998863 ) ;
#47735=AXIS2_PLACEMENT_3D ( 'NONE', #20840, #46470, #27976 ) ;
#47738=CARTESIAN_POINT ( 'NONE',  ( -10.23389218427744218, -12.85876097310435640, 67.93170662612612887 ) ) ;
#47739=ORIENTED_EDGE ( 'NONE', *, *, #4316, .F. ) ;
#47740=FACE_OUTER_BOUND ( 'NONE', #12646, .T. ) ;
#47742=CARTESIAN_POINT ( 'NONE',  ( -12.56171917241870695, -20.45376946399996854, 71.99148991968543498 ) ) ;
#47743=ORIENTED_EDGE ( 'NONE', *, *, #24534, .F. ) ;
#47745=VECTOR ( 'NONE', #17795, 1000.000000000000114 ) ;
#47747=CARTESIAN_POINT ( 'NONE',  ( -21.61101410369608899, -8.646988051702825473, 73.79467079059151047 ) ) ;
#47748=ORIENTED_EDGE ( 'NONE', *, *, #30544, .F. ) ;
#47749=B_SPLINE_CURVE_WITH_KNOTS ( 'NONE', 3,
 ( #4932, #30794, #12066, #15979, #11828, #986, #12540, #26851, #19444, #45574 ),
 .UNSPECIFIED., .F., .F.,
 ( 4, 2, 2, 2, 4 ),
 ( 0.000000000000000000, 0.2500000000000000000, 0.5000000000000000000, 0.7500000000000000000, 1.000000000000000000 ),
 .UNSPECIFIED. ) ;
#47750=CARTESIAN_POINT ( 'NONE',  ( -13.49406902941962372, -21.13830689255522088, 65.18640088419860490 ) ) ;
#47751=CARTESIAN_POINT ( 'NONE',  ( -16.09337498760136853, -22.13948385882417824, 58.40090183616962349 ) ) ;
#47752=CARTESIAN_POINT ( 'NONE',  ( -12.05483428091225129, -10.31798718066989551, 67.49896870046983111 ) ) ;
#47755=VERTEX_POINT ( 'NONE', #6645 ) ;
#47756=FACE_OUTER_BOUND ( 'NONE', #24873, .T. ) ;
#47757=CARTESIAN_POINT ( 'NONE',  ( -24.34586551078590233, -16.16342498662110572, 59.00843562520186936 ) ) ;
#47758=ORIENTED_EDGE ( 'NONE', *, *, #12010, .T. ) ;
#47759=CARTESIAN_POINT ( 'NONE',  ( -20.76602563802732604, -8.150687638125187817, 63.43404616943938379 ) ) ;
#47762=CARTESIAN_POINT ( 'NONE',  ( -14.23443154292173674, -21.09974595518388440, 71.81118900415394535 ) ) ;
#47763=CARTESIAN_POINT ( 'NONE',  ( -20.57913387270943417, -8.060128879191506002, 66.95916824008536139 ) ) ;
#47764=CARTESIAN_POINT ( 'NONE',  ( -16.49028911930641428, -22.20062183403187106, 65.36531050670200216 ) ) ;
#47765=ORIENTED_EDGE ( 'NONE', *, *, #21616, .F. ) ;
#47766=DIRECTION ( 'NONE',  ( -9.941263206155103325E-06, -7.040377910290660294E-06, 0.9999999999258021299 ) ) ;
#47768=CARTESIAN_POINT ( 'NONE',  ( -10.81855813007775957, -11.36397971161496301, 67.71890362106785233 ) ) ;
#47772=VERTEX_POINT ( 'NONE', #18433 ) ;
#47773=EDGE_CURVE ( 'NONE', #1012, #25345, #22157, .T. ) ;
#47774=CARTESIAN_POINT ( 'NONE',  ( -20.63397896388913821, -8.588477125147733204, 59.85627665378241602 ) ) ;
#47775=CARTESIAN_POINT ( 'NONE',  ( -17.81243367693841151, -24.25303685828974665, 53.49999999999995026 ) ) ;
#47776=CARTESIAN_POINT ( 'NONE',  ( -23.88825063663133363, -11.10528180765545869, 70.06927628447702716 ) ) ;
#47777=( BOUNDED_SURFACE ( )  B_SPLINE_SURFACE ( 3, 1, ( 
 ( #10654, #33268 ),
 ( #37209, #29605 ),
 ( #25430, #17774 ),
 ( #36487, #10889 ),
 ( #6714, #18761 ),
 ( #25911, #40926 ),
 ( #3006, #61 ) ),
 .UNSPECIFIED., .T., .F., .F. ) 
 B_SPLINE_SURFACE_WITH_KNOTS ( ( 4, 3, 4 ),
 ( 2, 2 ),
 ( 0.000000000000000000, 0.5000000000000000000, 1.000000000000000000 ),
 ( 0.000000000000000000, 1.000000000000000000 ),
 .UNSPECIFIED. ) 
 GEOMETRIC_REPRESENTATION_ITEM ( )  RATIONAL_B_SPLINE_SURFACE ( (
 ( 1.000000000000000000, 1.000000000000000000),
 ( 0.3333333333333335369, 0.3333333333333330373),
 ( 0.3333333333333335369, 0.3333333333333330373),
 ( 1.000000000000000000, 1.000000000000000000),
 ( 0.3333333333333333703, 0.3333333333333333703),
 ( 0.3333333333333333703, 0.3333333333333333703),
 ( 1.000000000000000000, 1.000000000000000000) ) ) 
 REPRESENTATION_ITEM ( '' )  SURFACE ( )  );
#47778=VECTOR ( 'NONE', #3654, 1000.000000000000227 ) ;
#47779=ORIENTED_EDGE ( 'NONE', *, *, #48308, .T. ) ;
#47781=CARTESIAN_POINT ( 'NONE',  ( -24.24936666102675531, -13.25469412794844537, 59.64802506593036924 ) ) ;
#47782=ADVANCED_FACE ( 'NONE', ( #43848 ), #14377, .T. ) ;
#47784=ORIENTED_EDGE ( 'NONE', *, *, #24293, .T. ) ;
#47785=ADVANCED_FACE ( 'NONE', ( #10101 ), #36124, .T. ) ;
#47786=CARTESIAN_POINT ( 'NONE',  ( -14.84927081153347039, -21.37251255130113137, 61.65072491673618771 ) ) ;
#47787=CARTESIAN_POINT ( 'NONE',  ( -24.87123163304818974, -14.59964195235338735, 62.89791815715346956 ) ) ;
#47789=CARTESIAN_POINT ( 'NONE',  ( -23.34288328645119037, -19.33377384263253873, 59.06905932422779415 ) ) ;
#47790=VERTEX_POINT ( 'NONE', #48238 ) ;
#47791=CARTESIAN_POINT ( 'NONE',  ( -24.12942727696282219, -12.79922002830157268, 69.77243032624397756 ) ) ;
#47793=CARTESIAN_POINT ( 'NONE',  ( -15.87557486115802696, -7.931373420853706335, 67.44007279014866185 ) ) ;
#47794=DIRECTION ( 'NONE',  ( -0.9441784275685841665, 0.3294345108122634369, 1.993146885055994800E-08 ) ) ;
#47795=VERTEX_POINT ( 'NONE', #25124 ) ;
#47796=CARTESIAN_POINT ( 'NONE',  ( -21.42927658580616068, -21.09115185931090508, 69.17637394757619518 ) ) ;
#47797=CARTESIAN_POINT ( 'NONE',  ( -10.76763551407085373, -17.13171859787639661, 61.45743118825841833 ) ) ;
#47798=DIRECTION ( 'NONE',  ( 0.8839923186919886877, -0.4675014229855999348, 2.842058574697910628E-08 ) ) ;
#47799=AXIS2_PLACEMENT_3D ( 'NONE', #40889, #44851, #36452 ) ;
#47803=VERTEX_POINT ( 'NONE', #44561 ) ;
#47806=VECTOR ( 'NONE', #17127, 1000.000000000000000 ) ;
#47807=FACE_OUTER_BOUND ( 'NONE', #46247, .T. ) ;
#47809=CARTESIAN_POINT ( 'NONE',  ( -13.18474066807476675, -20.93551553819402855, 58.23145462665691241 ) ) ;
#47810=B_SPLINE_CURVE_WITH_KNOTS ( 'NONE', 3,
 ( #37056, #40515, #11225, #36558, #18848, #154, #15134, #3089, #18584, #7297 ),
 .UNSPECIFIED., .F., .F.,
 ( 4, 2, 2, 2, 4 ),
 ( 0.1272669073659000727, 0.2522669073463680856, 0.3772669073268360984, 0.5022669073073040558, 0.6272669072877721241 ),
 .UNSPECIFIED. ) ;
#47812=CARTESIAN_POINT ( 'NONE',  ( -24.26647757246398740, -16.29234447064223446, 62.66499050339684374 ) ) ;
#47813=EDGE_LOOP ( 'NONE', ( #24327, #6853, #13848, #22101, #9631 ) ) ;
#47814=ORIENTED_EDGE ( 'NONE', *, *, #35041, .T. ) ;
#47815=CARTESIAN_POINT ( 'NONE',  ( -16.06904454444675778, -7.890656075740461795, 63.67011029959335389 ) ) ;
#47816=CARTESIAN_POINT ( 'NONE',  ( -21.86481658501223535, -9.328930240182819134, 66.75330195800948729 ) ) ;
#47817=ORIENTED_EDGE ( 'NONE', *, *, #4620, .T. ) ;
#47818=FACE_OUTER_BOUND ( 'NONE', #10085, .T. ) ;
#47819=LINE ( 'NONE', #14056, #23433 ) ;
#47820=CARTESIAN_POINT ( 'NONE',  ( -24.18314773428282649, -12.98801661480574410, 66.60246782464800219 ) ) ;
#47822=CARTESIAN_POINT ( 'NONE',  ( -13.69310769661218252, -20.79108007429942617, 64.98628911427817911 ) ) ;
#47823=VERTEX_POINT ( 'NONE', #40143 ) ;
#47826=CARTESIAN_POINT ( 'NONE',  ( -23.85820687874296908, -17.57049056139491583, 66.13284205629301482 ) ) ;
#47828=FACE_OUTER_BOUND ( 'NONE', #13542, .T. ) ;
#47829=ORIENTED_EDGE ( 'NONE', *, *, #20609, .T. ) ;
#47831=CARTESIAN_POINT ( 'NONE',  ( -11.60896167836250292, -10.15203476212633227, 71.10859753193520305 ) ) ;
#47832=CARTESIAN_POINT ( 'NONE',  ( -17.89428206796744192, -21.84713016422586307, 65.43712271095169797 ) ) ;
#47834=( BOUNDED_CURVE ( )  B_SPLINE_CURVE ( 3, ( #20577, #10217, #46907, #47156 ),
 .UNSPECIFIED., .F., .F. ) 
 B_SPLINE_CURVE_WITH_KNOTS ( ( 4, 4 ),
 ( 0.4074455897393638448, 0.5000000000000000000 ),
 .UNSPECIFIED. ) 
 CURVE ( )  GEOMETRIC_REPRESENTATION_ITEM ( )  RATIONAL_B_SPLINE_CURVE ( ( 0.6983129098260915102, 0.7760317562606922071, 0.8765941196519938527, 0.9999999999999927836 ) ) 
 REPRESENTATION_ITEM ( '' )  );
#47835=EDGE_CURVE ( 'NONE', #48249, #3376, #47154, .T. ) ;
#47839=ORIENTED_EDGE ( 'NONE', *, *, #40108, .F. ) ;
#47844=CARTESIAN_POINT ( 'NONE',  ( -19.10873388551254948, -7.551407109436953924, 67.08727174327995613 ) ) ;
#47846=( BOUNDED_SURFACE ( )  B_SPLINE_SURFACE ( 3, 1, ( 
 ( #15349, #16082 ),
 ( #12167, #598 ),
 ( #38246, #19066 ),
 ( #12649, #23989 ),
 ( #42707, #8969 ),
 ( #23759, #847 ),
 ( #15848, #30893 ) ),
 .UNSPECIFIED., .T., .F., .F. ) 
 B_SPLINE_SURFACE_WITH_KNOTS ( ( 4, 3, 4 ),
 ( 2, 2 ),
 ( 0.000000000000000000, 0.5000000000000000000, 1.000000000000000000 ),
 ( 0.000000000000000000, 1.000000000000000000 ),
 .UNSPECIFIED. ) 
 GEOMETRIC_REPRESENTATION_ITEM ( )  RATIONAL_B_SPLINE_SURFACE ( (
 ( 1.000000000000000000, 1.000000000000000000),
 ( 0.3333333333333335369, 0.3333333333333330373),
 ( 0.3333333333333335369, 0.3333333333333330373),
 ( 1.000000000000000000, 1.000000000000000000),
 ( 0.3333333333333333703, 0.3333333333333333703),
 ( 0.3333333333333333703, 0.3333333333333333703),
 ( 1.000000000000000000, 1.000000000000000000) ) ) 
 REPRESENTATION_ITEM ( '' )  SURFACE ( )  );
#47847=VECTOR ( 'NONE', #19116, 1000.000000000000000 ) ;
#47850=CARTESIAN_POINT ( 'NONE',  ( -15.53779737384271442, -7.601787063750024664, 70.77023165166117735 ) ) ;
#47852=ADVANCED_FACE ( 'NONE', ( #6408 ), #6887, .F. ) ;
#47856=EDGE_CURVE ( 'NONE', #42866, #10114, #44348, .T. ) ;
#47857=ORIENTED_EDGE ( 'NONE', *, *, #42731, .T. ) ;
#47859=( BOUNDED_SURFACE ( )  B_SPLINE_SURFACE ( 3, 1, ( 
 ( #11703, #45447 ),
 ( #26732, #41750 ),
 ( #8038, #48387 ),
 ( #23044, #3576 ),
 ( #38032, #4323 ),
 ( #14623, #11224 ),
 ( #42482, #41991 ) ),
 .UNSPECIFIED., .T., .F., .F. ) 
 B_SPLINE_SURFACE_WITH_KNOTS ( ( 4, 3, 4 ),
 ( 2, 2 ),
 ( 0.000000000000000000, 0.5000000000000000000, 1.000000000000000000 ),
 ( 0.000000000000000000, 1.000000000000000000 ),
 .UNSPECIFIED. ) 
 GEOMETRIC_REPRESENTATION_ITEM ( )  RATIONAL_B_SPLINE_SURFACE ( (
 ( 1.000000000000000000, 1.000000000000000000),
 ( 0.3333333333333335369, 0.3333333333333330373),
 ( 0.3333333333333335369, 0.3333333333333330373),
 ( 1.000000000000000000, 1.000000000000000000),
 ( 0.3333333333333333703, 0.3333333333333333703),
 ( 0.3333333333333333703, 0.3333333333333333703),
 ( 1.000000000000000000, 1.000000000000000000) ) ) 
 REPRESENTATION_ITEM ( '' )  SURFACE ( )  );
#47860=ORIENTED_EDGE ( 'NONE', *, *, #9424, .F. ) ;
#47861=ADVANCED_FACE ( 'NONE', ( #36903 ), #18195, .F. ) ;
#47862=CARTESIAN_POINT ( 'NONE',  ( -19.57699507595987143, -21.94144279212693860, 62.17998934563075153 ) ) ;
#47863=CARTESIAN_POINT ( 'NONE',  ( -21.46381135070672386, -20.59674881067212127, 69.21017043924877044 ) ) ;
#47865=ORIENTED_EDGE ( 'NONE', *, *, #3052, .T. ) ;
#47867=FACE_OUTER_BOUND ( 'NONE', #43279, .T. ) ;
#47868=EDGE_CURVE ( 'NONE', #33919, #26226, #24215, .T. ) ;
#47869=CARTESIAN_POINT ( 'NONE',  ( -21.47456293661849713, -9.038556783377254433, 70.41660404402310292 ) ) ;
#47870=LINE ( 'NONE', #33300, #12716 ) ;
#47871=VERTEX_POINT ( 'NONE', #481 ) ;
#47873=CARTESIAN_POINT ( 'NONE',  ( -16.91478550490786859, -21.84108428878278119, 72.18015306840750611 ) ) ;
#47875=CARTESIAN_POINT ( 'NONE',  ( -11.38784684563249527, -10.44144024994987774, 74.55229573521346254 ) ) ;
#47876=AXIS2_PLACEMENT_3D ( 'NONE', #37426, #10144, #40899 ) ;
#47877=CARTESIAN_POINT ( 'NONE',  ( -11.75774095458083046, -19.00383931511212765, 71.68685884783835149 ) ) ;
#47879=VERTEX_POINT ( 'NONE', #19423 ) ;
#47880=CARTESIAN_POINT ( 'NONE',  ( -13.84722314507279961, -8.273888791401406095, 74.37671575878690078 ) ) ;
#47881=( GEOMETRIC_REPRESENTATION_CONTEXT ( 3 ) GLOBAL_UNCERTAINTY_ASSIGNED_CONTEXT ( ( #28260 ) ) GLOBAL_UNIT_ASSIGNED_CONTEXT ( ( #8127, #34931, #4412 ) ) REPRESENTATION_CONTEXT ( 'NONE', 'WORKASPACE' ) );
#47883=CARTESIAN_POINT ( 'NONE',  ( -18.32882331211134286, -7.814473174497912566, 73.72575526123169709 ) ) ;
#47887=ORIENTED_EDGE ( 'NONE', *, *, #21135, .T. ) ;
#47888=B_SPLINE_CURVE_WITH_KNOTS ( 'NONE', 3,
 ( #34256, #1255, #16260, #15537, #38437, #26900, #30597, #4728, #19750, #34505 ),
 .UNSPECIFIED., .F., .F.,
 ( 4, 2, 2, 2, 4 ),
 ( 0.000000000000000000, 0.2500000000000000000, 0.5000000000000000000, 0.7500000000000000000, 1.000000000000000000 ),
 .UNSPECIFIED. ) ;
#47889=EDGE_LOOP ( 'NONE', ( #23676, #17179, #44520, #30456, #11800 ) ) ;
#47891=B_SPLINE_CURVE_WITH_KNOTS ( 'NONE', 3,
 ( #23186, #19473, #1240, #30826, #46322, #18998, #15518, #22955, #16246, #23680 ),
 .UNSPECIFIED., .F., .F.,
 ( 4, 2, 2, 2, 4 ),
 ( 0.1272669073658369288, 0.2522669073488094105, 0.3772669073317819199, 0.5022669073147543184, 0.6272669072977268279 ),
 .UNSPECIFIED. ) ;
#47894=CARTESIAN_POINT ( 'NONE',  ( -14.30826163110301685, -8.540783165273367672, 70.72957638424304605 ) ) ;
#47895=EDGE_CURVE ( 'NONE', #28162, #15877, #21336, .T. ) ;
#47896=DIRECTION ( 'NONE',  ( 0.7621627669932626858, -0.6473854467078885566, 3.680865982637999709E-08 ) ) ;
#47898=EDGE_LOOP ( 'NONE', ( #48129, #20919 ) ) ;
#47899=ORIENTED_EDGE ( 'NONE', *, *, #20716, .T. ) ;
#47903=B_SPLINE_CURVE_WITH_KNOTS ( 'NONE', 3,
 ( #26330, #46023, #30285, #45306, #37639, #23369, #33687, #15466, #38128, #12043 ),
 .UNSPECIFIED., .F., .F.,
 ( 4, 2, 2, 2, 4 ),
 ( 0.000000000000000000, 0.2500000000000000000, 0.5000000000000000000, 0.7500000000000000000, 1.000000000000000000 ),
 .UNSPECIFIED. ) ;
#47904=B_SPLINE_CURVE_WITH_KNOTS ( 'NONE', 3,
 ( #44697, #33084, #22519, #18825, #44950, #14365, #29419, #44451, #15113, #10954 ),
 .UNSPECIFIED., .F., .F.,
 ( 4, 2, 2, 2, 4 ),
 ( 0.1272669073658505845, 0.2522669073463317257, 0.3772669073268128948, 0.5022669073072940638, 0.6272669072877752328 ),
 .UNSPECIFIED. ) ;
#47905=ADVANCED_FACE ( 'NONE', ( #30043 ), #32946, .T. ) ;
#47906=ORIENTED_EDGE ( 'NONE', *, *, #48116, .F. ) ;
#47907=DIRECTION ( 'NONE',  ( -3.549360974554993999E-17, 6.371834667797928663E-18, 1.000000000000000000 ) ) ;
#47910=FACE_OUTER_BOUND ( 'NONE', #47111, .T. ) ;
#47912=CARTESIAN_POINT ( 'NONE',  ( -11.28069628694023940, -11.45046166655791886, 67.72937716582121936 ) ) ;
#47916=EDGE_CURVE ( 'NONE', #45931, #36781, #47903, .T. ) ;
#47917=DIRECTION ( 'NONE',  ( -0.9789991564299000970, -0.2038642972899922245, 4.410747590293501912E-08 ) ) ;
#47918=FACE_OUTER_BOUND ( 'NONE', #8102, .T. ) ;
#47919=CARTESIAN_POINT ( 'NONE',  ( -10.40417500068134160, -12.31441648348895868, 57.43519039097821377 ) ) ;
#47920=ORIENTED_EDGE ( 'NONE', *, *, #18667, .T. ) ;
#47922=DIRECTION ( 'NONE',  ( 1.198821491151391801E-05, -1.588017923178218046E-05, 0.9999999998020513425 ) ) ;
#47923=ADVANCED_FACE ( 'NONE', ( #11553 ), #39304, .T. ) ;
#47925=CARTESIAN_POINT ( 'NONE',  ( -22.29619887594318328, -17.36118473213641167, 53.49899999999994549 ) ) ;
#47926=ORIENTED_EDGE ( 'NONE', *, *, #46494, .T. ) ;
#47928=CARTESIAN_POINT ( 'NONE',  ( -10.42431062902801386, -14.74026950914408829, 71.62782695461453386 ) ) ;
#47929=CARTESIAN_POINT ( 'NONE',  ( -18.83428564917659287, -7.493810079819247072, 70.62713979963420741 ) ) ;
#47930=ORIENTED_EDGE ( 'NONE', *, *, #13193, .F. ) ;
#47931=CARTESIAN_POINT ( 'NONE',  ( -11.81178692268928643, -10.62566621335946770, 74.43885052268630886 ) ) ;
#47932=ORIENTED_EDGE ( 'NONE', *, *, #33907, .T. ) ;
#47933=CARTESIAN_POINT ( 'NONE',  ( -10.80730693270912468, -17.26544268483686650, 57.84327589213576459 ) ) ;
#47934=CARTESIAN_POINT ( 'NONE',  ( -13.61031878520947913, -20.67920105661088215, 61.51646270097772629 ) ) ;
#47936=CARTESIAN_POINT ( 'NONE',  ( -14.60479643987598841, -7.913168514039711887, 60.50491717424539218 ) ) ;
#47937=ORIENTED_EDGE ( 'NONE', *, *, #48211, .F. ) ;
#47939=CARTESIAN_POINT ( 'NONE',  ( -23.85748962928175132, -11.92509172808648543, 59.49707787073156595 ) ) ;
#47942=VERTEX_POINT ( 'NONE', #33720 ) ;
#47943=CARTESIAN_POINT ( 'NONE',  ( -10.38360249164154325, -14.43747963625415487, 67.87272197508832505 ) ) ;
#47945=EDGE_CURVE ( 'NONE', #28201, #29749, #27660, .T. ) ;
#47946=ORIENTED_EDGE ( 'NONE', *, *, #20799, .F. ) ;
#47950=LINE ( 'NONE', #9573, #23359 ) ;
#47951=CARTESIAN_POINT ( 'NONE',  ( -11.56806251476610115, -18.73522173559940995, 65.03234934376791898 ) ) ;
#47952=CARTESIAN_POINT ( 'NONE',  ( -23.96159466281891071, -11.23502865522796768, 70.07866094266108803 ) ) ;
#47953=CARTESIAN_POINT ( 'NONE',  ( -23.34299683607928699, -18.64475395501998278, 73.17857113406003577 ) ) ;
#47954=CARTESIAN_POINT ( 'NONE',  ( -13.03190793544029091, -9.358637495099101145, 67.57045887702402354 ) ) ;
#47958=CARTESIAN_POINT ( 'NONE',  ( -24.35026726019748011, -16.14395875459130281, 59.33152169323236791 ) ) ;
#47959=CARTESIAN_POINT ( 'NONE',  ( -21.55460084640030161, -9.091360965714955000, 73.90129052096925477 ) ) ;
#47960=DIRECTION ( 'NONE',  ( 4.556087729312554466E-06, -5.696494005668992306E-06, 0.9999999999733959477 ) ) ;
#47962=PLANE ( 'NONE',  #28799 ) ;
#47963=CARTESIAN_POINT ( 'NONE',  ( -24.43113031232903865, -15.58634216689856977, 73.30303748141028564 ) ) ;
#47966=VERTEX_POINT ( 'NONE', #24097 ) ;
#47967=DIRECTION ( 'NONE',  ( 8.719004453613161891E-07, -8.513143893533137515E-07, 0.9999999999992574828 ) ) ;
#47968=CYLINDRICAL_SURFACE ( 'NONE', #26086, 0.1500000000000037970 ) ;
#47971=CARTESIAN_POINT ( 'NONE',  ( -10.41569439578338496, -15.57669382292980131, 61.05261153187079515 ) ) ;
#47972=VERTEX_POINT ( 'NONE', #31727 ) ;
#47978=B_SPLINE_CURVE_WITH_KNOTS ( 'NONE', 1,
 ( #12202, #16612 ),
 .UNSPECIFIED., .F., .F.,
 ( 2, 2 ),
 ( 0.000000000000000000, 1.000000000000000000 ),
 .UNSPECIFIED. ) ;
#47979=( BOUNDED_SURFACE ( )  B_SPLINE_SURFACE ( 3, 1, ( 
 ( #23729, #43149 ),
 ( #9423, #12619 ),
 ( #24447, #16784 ),
 ( #9180, #38720 ),
 ( #5005, #20015 ),
 ( #24196, #31580 ),
 ( #35018, #1283 ) ),
 .UNSPECIFIED., .T., .F., .F. ) 
 B_SPLINE_SURFACE_WITH_KNOTS ( ( 4, 3, 4 ),
 ( 2, 2 ),
 ( 0.000000000000000000, 0.5000000000000000000, 1.000000000000000000 ),
 ( 0.000000000000000000, 1.000000000000000000 ),
 .UNSPECIFIED. ) 
 GEOMETRIC_REPRESENTATION_ITEM ( )  RATIONAL_B_SPLINE_SURFACE ( (
 ( 1.000000000000000000, 1.000000000000000000),
 ( 0.3333333333333335369, 0.3333333333333330373),
 ( 0.3333333333333335369, 0.3333333333333330373),
 ( 1.000000000000000000, 1.000000000000000000),
 ( 0.3333333333333333703, 0.3333333333333333703),
 ( 0.3333333333333333703, 0.3333333333333333703),
 ( 1.000000000000000000, 1.000000000000000000) ) ) 
 REPRESENTATION_ITEM ( '' )  SURFACE ( )  );
#47980=CARTESIAN_POINT ( 'NONE',  ( -24.10584592916820057, -12.56049825913868823, 73.24225570139947195 ) ) ;
#47986=CARTESIAN_POINT ( 'NONE',  ( -11.57425499491753307, -18.65360305739656610, 64.74707076836355668 ) ) ;
#47987=ORIENTED_EDGE ( 'NONE', *, *, #14006, .T. ) ;
#47988=CARTESIAN_POINT ( 'NONE',  ( -22.37985683132060188, -19.82347751554591397, 69.47417989525710880 ) ) ;
#47989=CARTESIAN_POINT ( 'NONE',  ( -11.64902330566212463, -10.02396254413167753, 47.99999999999994316 ) ) ;
#47990=ORIENTED_EDGE ( 'NONE', *, *, #39003, .F. ) ;
#47991=CARTESIAN_POINT ( 'NONE',  ( -22.14090652532222236, -20.04928072148792495, 62.51967078134249078 ) ) ;
#47992=CARTESIAN_POINT ( 'NONE',  ( -19.55442184481404766, -21.52995072282663358, 65.47958309245051112 ) ) ;
#47993=CARTESIAN_POINT ( 'NONE',  ( -24.86363034504136138, -14.41430157806603773, 66.28269108591972270 ) ) ;
#47994=ORIENTED_EDGE ( 'NONE', *, *, #44583, .T. ) ;
#47995=PLANE ( 'NONE',  #25494 ) ;
#47996=( BOUNDED_SURFACE ( )  B_SPLINE_SURFACE ( 3, 1, ( 
 ( #5558, #20574 ),
 ( #35570, #16846 ),
 ( #31885, #46902 ),
 ( #19462, #33735 ),
 ( #27096, #285 ),
 ( #30327, #15017 ),
 ( #30080, #42122 ) ),
 .UNSPECIFIED., .T., .F., .F. ) 
 B_SPLINE_SURFACE_WITH_KNOTS ( ( 4, 3, 4 ),
 ( 2, 2 ),
 ( 0.000000000000000000, 0.5000000000000000000, 1.000000000000000000 ),
 ( 0.000000000000000000, 1.000000000000000000 ),
 .UNSPECIFIED. ) 
 GEOMETRIC_REPRESENTATION_ITEM ( )  RATIONAL_B_SPLINE_SURFACE ( (
 ( 1.000000000000000000, 1.000000000000000000),
 ( 0.3333333333333335369, 0.3333333333333330373),
 ( 0.3333333333333335369, 0.3333333333333330373),
 ( 1.000000000000000000, 1.000000000000000000),
 ( 0.3333333333333333703, 0.3333333333333333703),
 ( 0.3333333333333333703, 0.3333333333333333703),
 ( 1.000000000000000000, 1.000000000000000000) ) ) 
 REPRESENTATION_ITEM ( '' )  SURFACE ( )  );
#47997=EDGE_CURVE ( 'NONE', #15944, #22030, #27782, .T. ) ;
#47998=CARTESIAN_POINT ( 'NONE',  ( -11.38014877795855995, -11.27757159305587464, 60.97885732570401274 ) ) ;
#47999=FACE_OUTER_BOUND ( 'NONE', #6156, .T. ) ;
#48000=EDGE_CURVE ( 'NONE', #27537, #1629, #1187, .T. ) ;
#48001=EDGE_CURVE ( 'NONE', #31485, #16726, #17160, .T. ) ;
#48003=VERTEX_POINT ( 'NONE', #20407 ) ;
#48004=LINE ( 'NONE', #32957, #29049 ) ;
#48005=CARTESIAN_POINT ( 'NONE',  ( -16.96573618372038794, -7.824106395124359459, 73.96018256200346741 ) ) ;
#48006=CARTESIAN_POINT ( 'NONE',  ( -20.70192761744073806, -8.118982583651908058, 63.50395666093379532 ) ) ;
#48008=CARTESIAN_POINT ( 'NONE',  ( -23.21283114448125673, -10.11939864774917908, 63.25681283445349123 ) ) ;
#48009=CARTESIAN_POINT ( 'NONE',  ( -16.82990565096947577, -21.78406541307506217, 68.69560622315208320 ) ) ;
#48011=DIRECTION ( 'NONE',  ( -3.395770065602591412E-06, -1.105252671792169116E-06, 0.9999999999936236561 ) ) ;
#48013=DIRECTION ( 'NONE',  ( 2.200805972648249745E-07, 3.006001593475220059E-06, 0.9999999999954577445 ) ) ;
#48014=CARTESIAN_POINT ( 'NONE',  ( -14.04013919049901560, -8.171999524408169790, 70.77311711151845941 ) ) ;
#48016=DIRECTION ( 'NONE',  ( -0.7107718805962432995, -0.7034225854731134264, -7.722840056494081040E-09 ) ) ;
#48017=FACE_OUTER_BOUND ( 'NONE', #2818, .T. ) ;
#48018=ORIENTED_EDGE ( 'NONE', *, *, #47262, .F. ) ;
#48020=ADVANCED_FACE ( 'NONE', ( #9085 ), #28272, .T. ) ;
#48021=CARTESIAN_POINT ( 'NONE',  ( -17.00739772171234776, -7.370819460300548798, 74.15356576969422520 ) ) ;
#48022=CARTESIAN_POINT ( 'NONE',  ( -19.61601346313181082, -21.50980264518277707, 65.46486213821819433 ) ) ;
#48023=CARTESIAN_POINT ( 'NONE',  ( -23.29918339618657086, -19.39037464299967439, 58.99915238703562181 ) ) ;
#48024=CARTESIAN_POINT ( 'NONE',  ( -11.55820670847359821, -18.73429759261662397, 71.83119032172525920 ) ) ;
#48026=EDGE_LOOP ( 'NONE', ( #39210, #47524, #6006, #31243, #26995 ) ) ;
#48028=CARTESIAN_POINT ( 'NONE',  ( -13.82689732469268407, -20.87277619789260186, 68.47097268802275494 ) ) ;
#48030=CARTESIAN_POINT ( 'NONE',  ( -22.38400238879419391, -20.36826089713532895, 62.41934470639706944 ) ) ;
#48031=CARTESIAN_POINT ( 'NONE',  ( -24.87286266620955288, -14.66952948351439190, 62.96942391020206742 ) ) ;
#48032=CARTESIAN_POINT ( 'NONE',  ( -22.79947183316497217, -19.38307604245925475, 59.02843669344121480 ) ) ;
#48033=VERTEX_POINT ( 'NONE', #1189 ) ;
#48036=CARTESIAN_POINT ( 'NONE',  ( -10.49862800246030936, -15.82799116930659622, 64.50771590054291948 ) ) ;
#48038=PLANE ( 'NONE',  #47799 ) ;
#48039=VERTEX_POINT ( 'NONE', #2160 ) ;
#48041=CARTESIAN_POINT ( 'NONE',  ( -24.12651600458584511, -12.62191667979047160, 73.25697658996381278 ) ) ;
#48042=LINE ( 'NONE', #21226, #2189 ) ;
#48043=CARTESIAN_POINT ( 'NONE',  ( -14.41059836940365635, -8.490934564906170934, 67.25975084671087245 ) ) ;
#48044=CARTESIAN_POINT ( 'NONE',  ( -10.04821600842096174, -15.85811274820897410, 64.62276192103250594 ) ) ;
#48045=FACE_OUTER_BOUND ( 'NONE', #33043, .T. ) ;
#48046=LINE ( 'NONE', #29336, #6186 ) ;
#48047=ORIENTED_EDGE ( 'NONE', *, *, #13151, .F. ) ;
#48049=CARTESIAN_POINT ( 'NONE',  ( -9.972618654632643853, -13.80886736810690962, 54.02312124697527906 ) ) ;
#48050=CARTESIAN_POINT ( 'NONE',  ( -24.09792875595538320, -17.08130417324981920, 72.88336032035921619 ) ) ;
#48052=CARTESIAN_POINT ( 'NONE',  ( -13.19046691777508329, -20.93951881724979813, 58.16837286248604499 ) ) ;
#48053=CARTESIAN_POINT ( 'NONE',  ( -10.77303304197945621, -12.62668734528506853, 61.09853568451838868 ) ) ;
#48055=EDGE_CURVE ( 'NONE', #5540, #1406, #38475, .T. ) ;
#48056=ORIENTED_EDGE ( 'NONE', *, *, #44651, .F. ) ;
#48057=EDGE_LOOP ( 'NONE', ( #37620, #45008 ) ) ;
#48058=CARTESIAN_POINT ( 'NONE',  ( -11.46028008028683942, -18.56947564720590194, 61.56238700194530367 ) ) ;
#48059=CARTESIAN_POINT ( 'NONE',  ( -9.975583804105555785, -14.65598652642324673, 71.44287259100559595 ) ) ;
#48060=ORIENTED_EDGE ( 'NONE', *, *, #12273, .F. ) ;
#48061=CARTESIAN_POINT ( 'NONE',  ( -12.96596438542217555, -9.347743257243967818, 70.99925352873879092 ) ) ;
#48065=CARTESIAN_POINT ( 'NONE',  ( -12.47631340003800915, -9.857337130378009959, 57.08935527210383754 ) ) ;
#48066=CARTESIAN_POINT ( 'NONE',  ( -14.41791765924166135, -21.19496194411871315, 58.31050579099508724 ) ) ;
#48067=CARTESIAN_POINT ( 'NONE',  ( -22.23733845922741637, -19.96043711175405733, 66.00421731380804147 ) ) ;
#48068=CARTESIAN_POINT ( 'NONE',  ( -24.66730449611544529, -13.06573935865489844, 62.94768786448354092 ) ) ;
#48070=EDGE_CURVE ( 'NONE', #47594, #37972, #5662, .T. ) ;
#48071=EDGE_CURVE ( 'NONE', #39181, #1086, #29237, .T. ) ;
#48072=CARTESIAN_POINT ( 'NONE',  ( -14.80624636014071172, -8.317144122717282428, 60.61996281969079803 ) ) ;
#48075=CARTESIAN_POINT ( 'NONE',  ( -12.14425528403576493, -10.13739698163135117, 64.02914326607979945 ) ) ;
#48076=EDGE_CURVE ( 'NONE', #21561, #20725, #23235, .T. ) ;
#48077=CARTESIAN_POINT ( 'NONE',  ( -16.64476583608805882, -21.82402065185451079, 72.30976097999173646 ) ) ;
#48079=DIRECTION ( 'NONE',  ( -0.8875028193683940358, -0.4608022847308269609, 4.020963237607658939E-08 ) ) ;
#48081=FACE_OUTER_BOUND ( 'NONE', #13832, .T. ) ;
#48082=CARTESIAN_POINT ( 'NONE',  ( -16.55445462874940077, -21.75508803775454325, 65.52564429725259743 ) ) ;
#48087=ORIENTED_EDGE ( 'NONE', *, *, #18893, .F. ) ;
#48089=CYLINDRICAL_SURFACE ( 'NONE', #14594, 0.1499999999999962752 ) ;
#48090=CARTESIAN_POINT ( 'NONE',  ( -17.39761456938454742, -7.809256627251312644, 67.32039592144390383 ) ) ;
#48092=CARTESIAN_POINT ( 'NONE',  ( -9.975093131592752016, -14.93635113986534257, 74.98274190467411415 ) ) ;
#48093=ORIENTED_EDGE ( 'NONE', *, *, #1866, .T. ) ;
#48094=CARTESIAN_POINT ( 'NONE',  ( -23.09478622540421000, -9.977449189158523524, 66.74171034086974430 ) ) ;
#48096=CARTESIAN_POINT ( 'NONE',  ( -22.91296630721855720, -15.15889098507616950, 53.49899999999994549 ) ) ;
#48097=ORIENTED_EDGE ( 'NONE', *, *, #45851, .F. ) ;
#48099=CARTESIAN_POINT ( 'NONE',  ( -12.35132619472584459, -19.70513314325878795, 61.39678631839771583 ) ) ;
#48101=CARTESIAN_POINT ( 'NONE',  ( -10.77962265614084814, -17.18953632050836333, 68.24154640182683806 ) ) ;
#48102=CARTESIAN_POINT ( 'NONE',  ( -12.74836358285320159, -20.08597126951521261, 71.82125749157572159 ) ) ;
#48103=CARTESIAN_POINT ( 'NONE',  ( -23.38410522734749009, -10.33907873996118276, 59.71708144416061970 ) ) ;
#48104=ORIENTED_EDGE ( 'NONE', *, *, #47317, .T. ) ;
#48106=AXIS2_PLACEMENT_3D ( 'NONE', #10143, #22432, #14041 ) ;
#48107=EDGE_CURVE ( 'NONE', #1105, #26632, #37713, .T. ) ;
#48108=CARTESIAN_POINT ( 'NONE',  ( -24.69822986944709697, -13.19963441799314197, 59.54763197719577761 ) ) ;
#48109=PLANE ( 'NONE',  #16643 ) ;
#48110=ORIENTED_EDGE ( 'NONE', *, *, #6171, .T. ) ;
#48112=DIRECTION ( 'NONE',  ( -0.8037372918934696520, 0.5949843406508664723, 7.322964617522835370E-08 ) ) ;
#48113=CARTESIAN_POINT ( 'NONE',  ( -23.62338436797153918, -18.94230004192412409, 69.48027381658378943 ) ) ;
#48116=EDGE_CURVE ( 'NONE', #23907, #5540, #26354, .T. ) ;
#48118=CARTESIAN_POINT ( 'NONE',  ( -17.79084088774826000, -7.768752266068899459, 60.08060768310445354 ) ) ;
#48119=CARTESIAN_POINT ( 'NONE',  ( -24.35831120643470982, -13.52022779156689936, 59.77756816219774549 ) ) ;
#48122=CARTESIAN_POINT ( 'NONE',  ( -15.50784526261009511, -8.076599967007890513, 74.37985659287807039 ) ) ;
#48123=CARTESIAN_POINT ( 'NONE',  ( -11.71629718011842414, -10.02134023935637686, 67.69908070314710358 ) ) ;
#48124=( BOUNDED_CURVE ( )  B_SPLINE_CURVE ( 3, ( #3628, #14929, #26045, #29001 ),
 .UNSPECIFIED., .F., .F. ) 
 B_SPLINE_CURVE_WITH_KNOTS ( ( 4, 4 ),
 ( 0.9074455897393621795, 1.000000000000000000 ),
 .UNSPECIFIED. ) 
 CURVE ( )  GEOMETRIC_REPRESENTATION_ITEM ( )  RATIONAL_B_SPLINE_CURVE ( ( 0.6983129098260769663, 0.7760317562606844355, 0.8765941196519920764, 1.000000000000000000 ) ) 
 REPRESENTATION_ITEM ( '' )  );
#48126=CARTESIAN_POINT ( 'NONE',  ( -10.04719910712313968, -15.85120016064457360, 64.68584367229796328 ) ) ;
#48127=VERTEX_POINT ( 'NONE', #47702 ) ;
#48128=VERTEX_POINT ( 'NONE', #28990 ) ;
#48129=ORIENTED_EDGE ( 'NONE', *, *, #13860, .T. ) ;
#48130=ADVANCED_FACE ( 'NONE', ( #29238 ), #29517, .T. ) ;
#48132=CARTESIAN_POINT ( 'NONE',  ( -23.47900403436495154, -10.35238886157799953, 53.76227901944321275 ) ) ;
#48133=CARTESIAN_POINT ( 'NONE',  ( -16.03798070992811731, -7.947690103083033364, 63.97010977124031683 ) ) ;
#48134=CARTESIAN_POINT ( 'NONE',  ( -12.73947787985187574, -9.016276410220392279, 71.10571287364943771 ) ) ;
#48135=( BOUNDED_SURFACE ( )  B_SPLINE_SURFACE ( 3, 1, ( 
 ( #21180, #20696 ),
 ( #10090, #13522 ),
 ( #36172, #13757 ),
 ( #44089, #25115 ),
 ( #47523, #29041 ),
 ( #40134, #1969 ),
 ( #6638, #36644 ) ),
 .UNSPECIFIED., .T., .F., .F. ) 
 B_SPLINE_SURFACE_WITH_KNOTS ( ( 4, 3, 4 ),
 ( 2, 2 ),
 ( 0.000000000000000000, 0.5000000000000000000, 1.000000000000000000 ),
 ( 0.000000000000000000, 1.000000000000000000 ),
 .UNSPECIFIED. ) 
 GEOMETRIC_REPRESENTATION_ITEM ( )  RATIONAL_B_SPLINE_SURFACE ( (
 ( 1.000000000000000000, 1.000000000000000000),
 ( 0.3333333333333335369, 0.3333333333333330373),
 ( 0.3333333333333335369, 0.3333333333333330373),
 ( 1.000000000000000000, 1.000000000000000000),
 ( 0.3333333333333333703, 0.3333333333333333703),
 ( 0.3333333333333333703, 0.3333333333333333703),
 ( 1.000000000000000000, 1.000000000000000000) ) ) 
 REPRESENTATION_ITEM ( '' )  SURFACE ( )  );
#48136=VERTEX_POINT ( 'NONE', #44275 ) ;
#48137=ORIENTED_EDGE ( 'NONE', *, *, #27251, .T. ) ;
#48138=ADVANCED_FACE ( 'NONE', ( #13941 ), #25309, .T. ) ;
#48141=CARTESIAN_POINT ( 'NONE',  ( -23.56138519289638822, -11.33989039198723248, 69.89210750373884196 ) ) ;
#48144=( BOUNDED_CURVE ( )  B_SPLINE_CURVE ( 3, ( #34381, #3887, #19376, #668 ),
 .UNSPECIFIED., .F., .F. ) 
 B_SPLINE_CURVE_WITH_KNOTS ( ( 4, 4 ),
 ( 1.570796326794896780, 1.780235837034217283 ),
 .UNSPECIFIED. ) 
 CURVE ( )  GEOMETRIC_REPRESENTATION_ITEM ( )  RATIONAL_B_SPLINE_CURVE ( ( 1.000000000000000000, 0.9963479302455154896, 0.9963479302455154896, 1.000000000000000000 ) ) 
 REPRESENTATION_ITEM ( '' )  );
#48145=ORIENTED_EDGE ( 'NONE', *, *, #40278, .F. ) ;
#48146=CARTESIAN_POINT ( 'NONE',  ( -24.36731093625853717, -15.69948419576056331, 69.81842082024948581 ) ) ;
#48148=CARTESIAN_POINT ( 'NONE',  ( -23.53718199026597802, -11.39867937719236757, 70.19210781355312179 ) ) ;
#48149=ORIENTED_EDGE ( 'NONE', *, *, #16823, .F. ) ;
#48150=CARTESIAN_POINT ( 'NONE',  ( -22.66727079836811853, -10.09628861529951216, 70.16178520457069112 ) ) ;
#48151=ORIENTED_EDGE ( 'NONE', *, *, #45028, .T. ) ;
#48153=PLANE ( 'NONE',  #28123 ) ;
#48154=FACE_OUTER_BOUND ( 'NONE', #43567, .T. ) ;
#48155=CARTESIAN_POINT ( 'NONE',  ( -13.56961256462628818, -20.71652534470609908, 58.25469809373281294 ) ) ;
#48157=CARTESIAN_POINT ( 'NONE',  ( -14.78576678908972397, -7.841836775542373239, 57.01033387128751428 ) ) ;
#48158=CARTESIAN_POINT ( 'NONE',  ( -15.31138759918230186, -21.95353881034377963, 72.18542105808592169 ) ) ;
#48159=EDGE_CURVE ( 'NONE', #39922, #24620, #6590, .T. ) ;
#48160=LINE ( 'NONE', #10984, #32897 ) ;
#48162=ORIENTED_EDGE ( 'NONE', *, *, #26517, .F. ) ;
#48163=DIRECTION ( 'NONE',  ( 0.3478314405900309603, 0.9375570856950864451, -9.567072274253696421E-17 ) ) ;
#48164=CARTESIAN_POINT ( 'NONE',  ( -21.49004948369781687, -9.049640773346018463, 70.42572721234685673 ) ) ;
#48165=ORIENTED_EDGE ( 'NONE', *, *, #47541, .T. ) ;
#48166=FACE_BOUND ( 'NONE', #40119, .T. ) ;
#48169=CARTESIAN_POINT ( 'NONE',  ( -24.90891992605694227, -15.28604896337863472, 47.99999999999994316 ) ) ;
#48171=CARTESIAN_POINT ( 'NONE',  ( -21.22463635358858269, -21.21689783003811769, 65.78442715983884170 ) ) ;
#48174=EDGE_LOOP ( 'NONE', ( #40687, #23537 ) ) ;
#48181=ORIENTED_EDGE ( 'NONE', *, *, #5551, .F. ) ;
#48182=CARTESIAN_POINT ( 'NONE',  ( -14.05371499411349667, -21.00138273984457982, 72.22607703579409133 ) ) ;
#48184=CARTESIAN_POINT ( 'NONE',  ( -13.06884191565359643, -20.85448943349606665, 58.23305466536662323 ) ) ;
#48187=CARTESIAN_POINT ( 'NONE',  ( -16.57554779340669882, -22.21081089906203943, 65.41059674993448425 ) ) ;
#48188=CARTESIAN_POINT ( 'NONE',  ( -23.77395946432122997, -18.70572718374853594, 73.02014183918953449 ) ) ;
#48189=DIRECTION ( 'NONE',  ( -0.02400335114476204179, 0.9997118780597844534, 1.529429979384368011E-10 ) ) ;
#48190=CARTESIAN_POINT ( 'NONE',  ( -20.55988796755815073, -8.491641294495202885, 67.19592733635545301 ) ) ;
#48192=ORIENTED_EDGE ( 'NONE', *, *, #15673, .T. ) ;
#48193=EDGE_CURVE ( 'NONE', #15624, #24088, #15524, .T. ) ;
#48195=CARTESIAN_POINT ( 'NONE',  ( -19.91921166743625093, -8.268929485741445262, 73.73599093592051190 ) ) ;
#48196=CARTESIAN_POINT ( 'NONE',  ( -22.96484330895583881, -19.08706763331013434, 59.18410642315183878 ) ) ;
#48197=CARTESIAN_POINT ( 'NONE',  ( -18.99339082800039691, -7.526352757794455783, 67.00048145165719404 ) ) ;
#48198=EDGE_CURVE ( 'NONE', #40354, #34898, #18498, .T. ) ;
#48199=CARTESIAN_POINT ( 'NONE',  ( -18.56804848150531484, -7.447508036923572661, 73.94726072066615075 ) ) ;
#48200=ORIENTED_EDGE ( 'NONE', *, *, #8291, .F. ) ;
#48202=VERTEX_POINT ( 'NONE', #19127 ) ;
#48203=CARTESIAN_POINT ( 'NONE',  ( -16.75112815133339694, -21.83074212251240453, 72.46543312350107158 ) ) ;
#48205=CARTESIAN_POINT ( 'NONE',  ( -24.46479344177693349, -14.44719919422189491, 66.18292729247950490 ) ) ;
#48207=EDGE_CURVE ( 'NONE', #29387, #17516, #29674, .T. ) ;
#48208=ORIENTED_EDGE ( 'NONE', *, *, #28663, .T. ) ;
#48209=EDGE_CURVE ( 'NONE', #42340, #7278, #37865, .T. ) ;
#48210=CARTESIAN_POINT ( 'NONE',  ( -18.85724798917316392, -7.906108138700305155, 67.18599644112759961 ) ) ;
#48211=EDGE_CURVE ( 'NONE', #10231, #12237, #24365, .T. ) ;
#48212=CARTESIAN_POINT ( 'NONE',  ( -14.76782893607791891, -8.332635497213580322, 60.31996286260869056 ) ) ;
#48213=VERTEX_POINT ( 'NONE', #19362 ) ;
#48214=DIRECTION ( 'NONE',  ( -0.06306825763707681054, 0.9980092158285027715, 2.415158932891090531E-08 ) ) ;
#48215=CARTESIAN_POINT ( 'NONE',  ( -10.13258936719380898, -16.33817337277914561, 71.63245765104117879 ) ) ;
#48216=ORIENTED_EDGE ( 'NONE', *, *, #36272, .F. ) ;
#48220=CARTESIAN_POINT ( 'NONE',  ( -17.57479954835421765, -7.360677901809306256, 63.74331195988233389 ) ) ;
#48221=ORIENTED_EDGE ( 'NONE', *, *, #11208, .T. ) ;
#48222=CARTESIAN_POINT ( 'NONE',  ( -18.36938390176548808, -21.74637740388497775, 72.35681286596320660 ) ) ;
#48225=CARTESIAN_POINT ( 'NONE',  ( -22.56207008003183745, -19.63703213565221617, 72.92928497383269359 ) ) ;
#48227=ORIENTED_EDGE ( 'NONE', *, *, #4418, .F. ) ;
#48230=CARTESIAN_POINT ( 'NONE',  ( -23.72594254189621310, -11.64830526502516328, 63.24658506625491583 ) ) ;
#48233=EDGE_LOOP ( 'NONE', ( #17684, #22737 ) ) ;
#48234=CARTESIAN_POINT ( 'NONE',  ( -12.91576191806997365, -9.388722997169709927, 71.13453240065665284 ) ) ;
#48235=CARTESIAN_POINT ( 'NONE',  ( -11.83951967486316192, -10.58871707758600600, 71.07779090859834525 ) ) ;
#48236=DIRECTION ( 'NONE',  ( -0.05957303659011964347, -0.9982239494779874267, 2.515684304538401319E-08 ) ) ;
#48238=CARTESIAN_POINT ( 'NONE',  ( -13.85393650630732054, -8.270265118416840977, 74.38450092284953996 ) ) ;
#48240=LINE ( 'NONE', #18435, #46769 ) ;
#48241=DIRECTION ( 'NONE',  ( -0.3037135924646502394, 0.9527633776296274837, 2.170275161112374562E-08 ) ) ;
#48243=EDGE_CURVE ( 'NONE', #31795, #23182, #2022, .T. ) ;
#48244=DIRECTION ( 'NONE',  ( -0.003782665018460030538, -0.9999928456970870183, -9.532993539451315208E-09 ) ) ;
#48247=CARTESIAN_POINT ( 'NONE',  ( -13.59121668485792789, -8.949893101123375772, 60.62877463978671244 ) ) ;
#48248=( BOUNDED_CURVE ( )  B_SPLINE_CURVE ( 3, ( #20469, #27603, #23923, #46577 ),
 .UNSPECIFIED., .F., .F. ) 
 B_SPLINE_CURVE_WITH_KNOTS ( ( 4, 4 ),
 ( 0.9074455897393665094, 1.000000000000000000 ),
 .UNSPECIFIED. ) 
 CURVE ( )  GEOMETRIC_REPRESENTATION_ITEM ( )  RATIONAL_B_SPLINE_CURVE ( ( 0.6983129098261009471, 0.7760317562607050856, 0.8765941196520047329, 1.000000000000000000 ) ) 
 REPRESENTATION_ITEM ( '' )  );
#48249=VERTEX_POINT ( 'NONE', #15658 ) ;
#48252=DIRECTION ( 'NONE',  ( 5.468526108419875108E-08, 8.832527038290525275E-06, -0.9999999999609916479 ) ) ;
#48253=CARTESIAN_POINT ( 'NONE',  ( -11.73296596577226936, -10.64774513788296417, 74.72412863062541533 ) ) ;
#48255=( BOUNDED_CURVE ( )  B_SPLINE_CURVE ( 3, ( #17209, #47277, #9849, #6390 ),
 .UNSPECIFIED., .F., .F. ) 
 B_SPLINE_CURVE_WITH_KNOTS ( ( 4, 4 ),
 ( 0.4074455897393672310, 0.5000000000000000000 ),
 .UNSPECIFIED. ) 
 CURVE ( )  GEOMETRIC_REPRESENTATION_ITEM ( )  RATIONAL_B_SPLINE_CURVE ( ( 0.6983129098261091627, 0.7760317562607090824, 0.8765941196520052880, 0.9999999999999952260 ) ) 
 REPRESENTATION_ITEM ( '' )  );
#48256=ORIENTED_EDGE ( 'NONE', *, *, #19853, .T. ) ;
#48257=EDGE_CURVE ( 'NONE', #22984, #15971, #11503, .T. ) ;
#48258=CARTESIAN_POINT ( 'NONE',  ( -24.47131905756960890, -12.39240217952595913, 73.36412813348363215 ) ) ;
#48260=CARTESIAN_POINT ( 'NONE',  ( -12.58002129225892674, -9.148929240056048684, 74.43427715830415536 ) ) ;
#48262=EDGE_CURVE ( 'NONE', #29740, #39283, #45571, .T. ) ;
#48265=VERTEX_POINT ( 'NONE', #38300 ) ;
#48267=CARTESIAN_POINT ( 'NONE',  ( -17.72634068467203505, -21.85272461955047874, 58.70553378267868538 ) ) ;
#48268=CARTESIAN_POINT ( 'NONE',  ( -14.76026690907102790, -8.277937858068607824, 57.05820006608990269 ) ) ;
#48270=LINE ( 'NONE', #6191, #32242 ) ;
#48271=( BOUNDED_SURFACE ( )  B_SPLINE_SURFACE ( 3, 1, ( 
 ( #43834, #47518 ),
 ( #18180, #33428 ),
 ( #29520, #13986 ),
 ( #10805, #40129 ),
 ( #14702, #21650 ),
 ( #36637, #17694 ),
 ( #32721, #44802 ) ),
 .UNSPECIFIED., .T., .F., .F. ) 
 B_SPLINE_SURFACE_WITH_KNOTS ( ( 4, 3, 4 ),
 ( 2, 2 ),
 ( 0.000000000000000000, 0.5000000000000000000, 1.000000000000000000 ),
 ( 0.000000000000000000, 1.000000000000000000 ),
 .UNSPECIFIED. ) 
 GEOMETRIC_REPRESENTATION_ITEM ( )  RATIONAL_B_SPLINE_SURFACE ( (
 ( 1.000000000000000000, 1.000000000000000000),
 ( 0.3333333333333335369, 0.3333333333333330373),
 ( 0.3333333333333335369, 0.3333333333333330373),
 ( 1.000000000000000000, 1.000000000000000000),
 ( 0.3333333333333333703, 0.3333333333333333703),
 ( 0.3333333333333333703, 0.3333333333333333703),
 ( 1.000000000000000000, 1.000000000000000000) ) ) 
 REPRESENTATION_ITEM ( '' )  SURFACE ( )  );
#48273=CARTESIAN_POINT ( 'NONE',  ( -19.10745041116545906, -21.66349580942223341, 62.13936675129127707 ) ) ;
#48274=LINE ( 'NONE', #25624, #39158 ) ;
#48275=EDGE_LOOP ( 'NONE', ( #46189, #43024, #12450, #26212, #10270 ) ) ;
#48276=CARTESIAN_POINT ( 'NONE',  ( -12.36794899618824140, -19.72224014812425352, 61.69678633597965955 ) ) ;
#48277=CARTESIAN_POINT ( 'NONE',  ( -10.45859239952313224, -15.89938452881993847, 64.79299464097340433 ) ) ;
#48279=CARTESIAN_POINT ( 'NONE',  ( -18.11396590982544197, -21.77512906430638040, 65.64532159443497505 ) ) ;
#48280=CARTESIAN_POINT ( 'NONE',  ( -23.80175822008580866, -17.82088921309938812, 62.88849600917846061 ) ) ;
#48281=DIRECTION ( 'NONE',  ( -0.3478314405900309603, -0.9375570856950864451, 9.567072274253696421E-17 ) ) ;
#48282=FACE_OUTER_BOUND ( 'NONE', #5076, .T. ) ;
#48284=CARTESIAN_POINT ( 'NONE',  ( -20.37299714182665866, -8.405577154986387356, 67.08104082189564110 ) ) ;
#48285=DIRECTION ( 'NONE',  ( -5.828394480008251615E-08, 1.590814170208496341E-07, 0.9999999999999855671 ) ) ;
#48286=CARTESIAN_POINT ( 'NONE',  ( -14.49278865106054504, -7.959940993718208624, 63.95125321502179361 ) ) ;
#48287=DIRECTION ( 'NONE',  ( 0.8447509909909737269, -0.5351595679979644915, 3.339321029457338869E-17 ) ) ;
#48288=CARTESIAN_POINT ( 'NONE',  ( -17.15999057916966208, -7.814067853132777408, 70.49035844391949013 ) ) ;
#48289=ADVANCED_FACE ( 'NONE', ( #4594 ), #17570, .T. ) ;
#48290=ORIENTED_EDGE ( 'NONE', *, *, #16286, .F. ) ;
#48291=ORIENTED_EDGE ( 'NONE', *, *, #3819, .T. ) ;
#48292=CARTESIAN_POINT ( 'NONE',  ( -16.94342272711102027, -21.79279426035641976, 72.46543237156552664 ) ) ;
#48293=CARTESIAN_POINT ( 'NONE',  ( -9.975448439439539072, -14.66457030764845193, 71.52120984734268916 ) ) ;
#48295=CARTESIAN_POINT ( 'NONE',  ( -13.22529448846758982, -9.145569705956512863, 64.19474388871357462 ) ) ;
#48296=CARTESIAN_POINT ( 'NONE',  ( -11.29272648115082589, -18.18986258437042736, 57.91787737795063862 ) ) ;
#48299=CARTESIAN_POINT ( 'NONE',  ( -24.75425692978680559, -16.14426119111164937, 62.70673273743753384 ) ) ;
#48303=CARTESIAN_POINT ( 'NONE',  ( -16.26184114368905043, -7.855670183028919062, 60.20028478909662084 ) ) ;
#48304=VERTEX_POINT ( 'NONE', #45961 ) ;
#48308=EDGE_CURVE ( 'NONE', #1846, #1214, #30949, .T. ) ;
#48310=CARTESIAN_POINT ( 'NONE',  ( -24.28250243997646152, -13.40622297325496959, 59.37884623336672973 ) ) ;
#48311=CARTESIAN_POINT ( 'NONE',  ( -24.59706363142188934, -12.79617847886399140, 66.48742024426742603 ) ) ;
#48312=CARTESIAN_POINT ( 'NONE',  ( -11.85858129499141178, -10.56289031856201710, 74.45501804502151799 ) ) ;
#48313=CARTESIAN_POINT ( 'NONE',  ( -17.20139284005516700, -7.812749994621428051, 70.79035839633094440 ) ) ;
#48314=VERTEX_POINT ( 'NONE', #16135 ) ;
#48315=ORIENTED_EDGE ( 'NONE', *, *, #15512, .T. ) ;
#48318=MANIFOLD_SOLID_BREP ( 'Stock-MAS-175-1', #10259 ) ;
#48321=EDGE_CURVE ( 'NONE', #42340, #45965, #34255, .T. ) ;
#48322=EDGE_CURVE ( 'NONE', #37303, #3283, #47308, .T. ) ;
#48323=CARTESIAN_POINT ( 'NONE',  ( -9.974235501303020612, -14.86645057852294016, 75.05424837986554110 ) ) ;
#48325=CARTESIAN_POINT ( 'NONE',  ( -23.10889842201686761, -9.994063388419718308, 66.74193459406681939 ) ) ;
#48326=FACE_OUTER_BOUND ( 'NONE', #18200, .T. ) ;
#48333=EDGE_CURVE ( 'NONE', #2842, #23748, #26080, .T. ) ;
#48334=B_SPLINE_CURVE_WITH_KNOTS ( 'NONE', 3,
 ( #10393, #34, #36458, #25631, #29088, #21701, #26367, #37179, #36942, #18233 ),
 .UNSPECIFIED., .F., .F.,
 ( 4, 2, 2, 2, 4 ),
 ( 0.000000000000000000, 0.2500000000000000000, 0.5000000000000000000, 0.7500000000000000000, 1.000000000000000000 ),
 .UNSPECIFIED. ) ;
#48335=CARTESIAN_POINT ( 'NONE',  ( -17.76160456433342461, -7.366686981516495258, 60.24094141105150868 ) ) ;
#48336=CARTESIAN_POINT ( 'NONE',  ( -15.02609155194205037, -8.232647636148229253, 56.84999999999993037 ) ) ;
#48338=ORIENTED_EDGE ( 'NONE', *, *, #20435, .F. ) ;
#48339=CARTESIAN_POINT ( 'NONE',  ( -11.05034076241727625, -11.79557573020262318, 71.37388789199357575 ) ) ;
#48341=CARTESIAN_POINT ( 'NONE',  ( -24.71300512064630794, -13.26796065199660113, 59.61913874400077873 ) ) ;
#48342=CARTESIAN_POINT ( 'NONE',  ( -23.94283526169594722, -17.36006291627137088, 66.22891933742413073 ) ) ;
#48343=VERTEX_POINT ( 'NONE', #32094 ) ;
#48344=CARTESIAN_POINT ( 'NONE',  ( -10.96921284960095555, -11.97350354382807680, 74.84368195529052059 ) ) ;
#48346=CARTESIAN_POINT ( 'NONE',  ( -15.35564964753334394, -21.49796208608013259, 72.27405351148586021 ) ) ;
#48347=CARTESIAN_POINT ( 'NONE',  ( -16.16748626245079379, -22.20318634978239203, 53.49999999999994316 ) ) ;
#48348=DIRECTION ( 'NONE',  ( -0.4251432040024066272, -0.9051260995521939190, -1.185120001106687566E-09 ) ) ;
#48350=EDGE_LOOP ( 'NONE', ( #29175, #39565, #16119, #994, #6770 ) ) ;
#48351=CARTESIAN_POINT ( 'NONE',  ( -16.19792114999740562, -7.866354181730329742, 60.48556343814865954 ) ) ;
#48354=CARTESIAN_POINT ( 'NONE',  ( -18.48323135481441426, -7.889672941340453605, 74.14064351459154523 ) ) ;
#48355=( BOUNDED_CURVE ( )  B_SPLINE_CURVE ( 3, ( #2955, #25383, #40161, #40393 ),
 .UNSPECIFIED., .F., .F. ) 
 B_SPLINE_CURVE_WITH_KNOTS ( ( 4, 4 ),
 ( 0.5000000000000000000, 0.9074455897393605142 ),
 .UNSPECIFIED. ) 
 CURVE ( )  GEOMETRIC_REPRESENTATION_ITEM ( )  RATIONAL_B_SPLINE_CURVE ( ( 0.9999999999999961142, 0.4567392136813419601, 0.3561768502900365396, 0.6983129098260758560 ) ) 
 REPRESENTATION_ITEM ( '' )  );
#48357=LINE ( 'NONE', #44688, #10857 ) ;
#48359=CARTESIAN_POINT ( 'NONE',  ( -19.85889901765038346, -21.37233916515964438, 69.21353063550283480 ) ) ;
#48360=CARTESIAN_POINT ( 'NONE',  ( -20.60942684424193416, -21.09890871138989965, 58.65947248567252359 ) ) ;
#48367=CARTESIAN_POINT ( 'NONE',  ( -21.99178428503401861, -9.439038574390064440, 60.02171213140443484 ) ) ;
#48369=EDGE_LOOP ( 'NONE', ( #4248, #21019, #25614, #25925, #37825 ) ) ;
#48370=ORIENTED_EDGE ( 'NONE', *, *, #20604, .T. ) ;
#48374=CARTESIAN_POINT ( 'NONE',  ( -11.46723045859082468, -10.33494501157577972, 74.63223394389621035 ) ) ;
#48375=CARTESIAN_POINT ( 'NONE',  ( -12.81450527785482052, -9.474959380418823685, 74.61923006088066757 ) ) ;
#48377=ORIENTED_EDGE ( 'NONE', *, *, #19853, .F. ) ;
#48378=ADVANCED_FACE ( 'NONE', ( #1131 ), #32572, .T. ) ;
#48379=CARTESIAN_POINT ( 'NONE',  ( -10.78978129071826686, -12.42417052737942917, 57.32857332104949677 ) ) ;
#48381=CARTESIAN_POINT ( 'NONE',  ( -23.51785719624223958, -11.36449344406884343, 70.19210750610864125 ) ) ;
#48383=DIRECTION ( 'NONE',  ( -0.2196488028684550897, -0.9755790093059856227, 7.835600157697874713E-08 ) ) ;
#48384=ORIENTED_EDGE ( 'NONE', *, *, #23366, .T. ) ;
#48385=EDGE_CURVE ( 'NONE', #35067, #41098, #29635, .T. ) ;
#48386=B_SPLINE_CURVE_WITH_KNOTS ( 'NONE', 3,
 ( #27620, #4736, #34513, #12117, #8918, #46094, #38699, #42409, #42658, #19499 ),
 .UNSPECIFIED., .F., .F.,
 ( 4, 2, 2, 2, 4 ),
 ( 0.1272669073658555250, 0.2522669073463344458, 0.3772669073268133388, 0.5022669073072922874, 0.6272669072877712360 ),
 .UNSPECIFIED. ) ;
#48387=CARTESIAN_POINT ( 'NONE',  ( -22.22492895683646807, -9.112220634607178127, 59.76525293062090327 ) ) ;
#48389=CARTESIAN_POINT ( 'NONE',  ( -24.42401643431037073, -14.84212902100172293, 59.54300237020546405 ) ) ;
#48390=CARTESIAN_POINT ( 'NONE',  ( -10.41803450628629157, -12.27586432466274502, 57.42883078543415110 ) ) ;
#48393=CARTESIAN_POINT ( 'NONE',  ( -11.09928078071809487, -10.87206734048183243, 57.33090417946287687 ) ) ;
#48396=B_SPLINE_CURVE_WITH_KNOTS ( 'NONE', 3,
 ( #3053, #18812, #44939, #41218, #26446, #25962, #18305, #41462, #33316, #48122 ),
 .UNSPECIFIED., .F., .F.,
 ( 4, 2, 2, 2, 4 ),
 ( 0.000000000000000000, 0.2500000000000000000, 0.5000000000000000000, 0.7500000000000000000, 1.000000000000000000 ),
 .UNSPECIFIED. ) ;
#48397=( BOUNDED_CURVE ( )  B_SPLINE_CURVE ( 3, ( #11446, #26470, #41485, #22794 ),
 .UNSPECIFIED., .F., .F. ) 
 B_SPLINE_CURVE_WITH_KNOTS ( ( 4, 4 ),
 ( 0.5000000000000000000, 0.9074455897393707282 ),
 .UNSPECIFIED. ) 
 CURVE ( )  GEOMETRIC_REPRESENTATION_ITEM ( )  RATIONAL_B_SPLINE_CURVE ( ( 0.9999999999999903411, 0.4567392136813203107, 0.3561768502900325983, 0.6983129098261168233 ) ) 
 REPRESENTATION_ITEM ( '' )  );
#48398=CARTESIAN_POINT ( 'NONE',  ( -19.36811171093278006, -7.617188704462286353, 60.08280224782789958 ) ) ;
#48400=EDGE_LOOP ( 'NONE', ( #7048, #10594 ) ) ;
#48401=CARTESIAN_POINT ( 'NONE',  ( -10.54259038139361770, -17.66360020425462451, 68.19698326179320702 ) ) ;
#48402=CARTESIAN_POINT ( 'NONE',  ( -14.62876365129575795, -8.337020046287406672, 63.78978836832918375 ) ) ;
#48403=CARTESIAN_POINT ( 'NONE',  ( -18.79049830835916524, -7.892586073225762000, 70.38540174208183942 ) ) ;
#48404=ORIENTED_EDGE ( 'NONE', *, *, #13541, .T. ) ;
#48406=FACE_BOUND ( 'NONE', #22176, .T. ) ;
#48407=ORIENTED_EDGE ( 'NONE', *, *, #41946, .F. ) ;
#48409=CARTESIAN_POINT ( 'NONE',  ( -13.68917838456570024, -20.72961559785960617, 61.58934264708406658 ) ) ;
#48413=CARTESIAN_POINT ( 'NONE',  ( -24.45201636468676298, -14.25170757634699470, 69.95275273439749242 ) ) ;
#48414=ORIENTED_EDGE ( 'NONE', *, *, #15245, .F. ) ;
#48415=DIRECTION ( 'NONE',  ( -0.4780674886490097197, 0.8783231047267436864, 5.292596395488306339E-08 ) ) ;
#48416=CARTESIAN_POINT ( 'NONE',  ( -15.35027142736847239, -7.653576728715946409, 74.26480947788739684 ) ) ;
#48417=B_SPLINE_CURVE_WITH_KNOTS ( 'NONE', 1,
 ( #4043, #42437 ),
 .UNSPECIFIED., .F., .F.,
 ( 2, 2 ),
 ( 0.000000000000000000, 1.000000000000000000 ),
 .UNSPECIFIED. ) ;
#48418=EDGE_LOOP ( 'NONE', ( #30827, #19306, #1011, #26245 ) ) ;
#48419=CARTESIAN_POINT ( 'NONE',  ( -10.81484442788029376, -17.11524687497682251, 61.45743118925498294 ) ) ;
#48420=( BOUNDED_CURVE ( )  B_SPLINE_CURVE ( 3, ( #9202, #24222, #39229, #43173 ),
 .UNSPECIFIED., .F., .F. ) 
 B_SPLINE_CURVE_WITH_KNOTS ( ( 4, 4 ),
 ( 0.5000000000000000000, 0.9074455897393625126 ),
 .UNSPECIFIED. ) 
 CURVE ( )  GEOMETRIC_REPRESENTATION_ITEM ( )  RATIONAL_B_SPLINE_CURVE ( ( 1.000000000000000666, 0.4567392136813430703, 0.3561768502900337641, 0.6983129098260736356 ) ) 
 REPRESENTATION_ITEM ( '' )  );
#48422=VERTEX_POINT ( 'NONE', #14540 ) ;
#48423=EDGE_LOOP ( 'NONE', ( #47035, #33313, #37862, #39687, #5116 ) ) ;
#48424=CARTESIAN_POINT ( 'NONE',  ( -15.62268239484049026, -8.044906604745516887, 70.62492222724996793 ) ) ;
#48425=DIRECTION ( 'NONE',  ( 1.081321489472432593E-05, 7.211308816928991536E-06, -0.9999999999155356756 ) ) ;
#48426=CARTESIAN_POINT ( 'NONE',  ( -19.32828448179457581, -22.01175803993288227, 58.62533143847836214 ) ) ;
#48427=CARTESIAN_POINT ( 'NONE',  ( -10.59838446366035924, -13.25112969284905695, 74.90647544603520203 ) ) ;
#48429=DIRECTION ( 'NONE',  ( 1.198821491151391801E-05, -1.588017923178218046E-05, 0.9999999998020513425 ) ) ;
#48430=CARTESIAN_POINT ( 'NONE',  ( -20.67761229128902656, -8.545853924536821467, 66.92536870251414882 ) ) ;
#48431=ORIENTED_EDGE ( 'NONE', *, *, #17044, .F. ) ;
#48433=FACE_OUTER_BOUND ( 'NONE', #14197, .T. ) ;
#48434=CARTESIAN_POINT ( 'NONE',  ( -23.07906183844443859, -9.958936969296642516, 66.72677665813928627 ) ) ;
#48435=CARTESIAN_POINT ( 'NONE',  ( -21.91379008343609769, -9.437005872758499336, 63.26324041012450294 ) ) ;
#48436=CARTESIAN_POINT ( 'NONE',  ( -17.91451193640577344, -22.24313339626381847, 61.99040498927033127 ) ) ;
#48437=ORIENTED_EDGE ( 'NONE', *, *, #44528, .T. ) ;
#48438=EDGE_CURVE ( 'NONE', #43420, #34242, #16273, .T. ) ;
#48442=ORIENTED_EDGE ( 'NONE', *, *, #36386, .T. ) ;
#48443=CARTESIAN_POINT ( 'NONE',  ( -24.35706380436459995, -15.77560588608014136, 69.83307488757523629 ) ) ;
#48445=CARTESIAN_POINT ( 'NONE',  ( -10.03884236986523604, -13.82852981289494210, 57.70470977341523167 ) ) ;
#48447=CARTESIAN_POINT ( 'NONE',  ( -10.39044952859546278, -14.32866914145539994, 64.68803851576602426 ) ) ;
#48448=CARTESIAN_POINT ( 'NONE',  ( -10.85841931818429629, -17.37798394237199062, 64.91267318220633342 ) ) ;
#48449=EDGE_CURVE ( 'NONE', #21669, #35366, #24424, .T. ) ;
#48454=EDGE_LOOP ( 'NONE', ( #15664, #35015, #38636, #38618, #48477 ) ) ;
#48455=CARTESIAN_POINT ( 'NONE',  ( -24.68275054790482770, -16.48720572190336853, 59.23837039904986312 ) ) ;
#48456=VERTEX_POINT ( 'NONE', #14069 ) ;
#48457=CARTESIAN_POINT ( 'NONE',  ( -10.32795594944829176, -17.07800752666445021, 57.88749324818159891 ) ) ;
#48458=CARTESIAN_POINT ( 'NONE',  ( -17.65279228434817327, -7.362550528378125847, 63.71203517750778644 ) ) ;
#48459=EDGE_CURVE ( 'NONE', #26800, #18999, #2766, .T. ) ;
#48462=CARTESIAN_POINT ( 'NONE',  ( -11.44359845021116939, -10.36664799652857738, 74.53861401861469460 ) ) ;
#48463=EDGE_LOOP ( 'NONE', ( #47926, #19654 ) ) ;
#48465=CYLINDRICAL_SURFACE ( 'NONE', #44140, 6.899999999999999467 ) ;
#48466=EDGE_CURVE ( 'NONE', #46554, #4981, #14312, .T. ) ;
#48470=CARTESIAN_POINT ( 'NONE',  ( -19.92825877560272474, -21.82574164115814241, 69.13493675705122143 ) ) ;
#48471=EDGE_CURVE ( 'NONE', #6656, #11955, #36969, .T. ) ;
#48474=CARTESIAN_POINT ( 'NONE',  ( -23.33822317206753638, -19.33980969897947944, 59.07684782711321958 ) ) ;
#48475=CARTESIAN_POINT ( 'NONE',  ( -23.07906183844443859, -9.958936969296642516, 66.72677665813928627 ) ) ;
#48476=ORIENTED_EDGE ( 'NONE', *, *, #32711, .T. ) ;
#48477=ORIENTED_EDGE ( 'NONE', *, *, #32110, .F. ) ;
#48478=DIRECTION ( 'NONE',  ( -1.295331064632368052E-06, 6.890485867068654572E-07, 0.9999999999989236388 ) ) ;
#48479=CARTESIAN_POINT ( 'NONE',  ( -24.71393967724174345, -16.34927462137609311, 59.23677039840046632 ) ) ;
#48484=CARTESIAN_POINT ( 'NONE',  ( -16.49051187235095384, -22.20064845604942150, 65.38710926064737805 ) ) ;
#48485=VERTEX_POINT ( 'NONE', #7459 ) ;
#48487=B_SPLINE_CURVE_WITH_KNOTS ( 'NONE', 1,
 ( #16206, #5154 ),
 .UNSPECIFIED., .F., .F.,
 ( 2, 2 ),
 ( 0.000000000000000000, 1.000000000000000000 ),
 .UNSPECIFIED. ) ;
#48488=DIRECTION ( 'NONE',  ( -1.568615307090388417E-06, -3.599470258889626763E-09, 0.9999999999987696508 ) ) ;
#48491=B_SPLINE_CURVE_WITH_KNOTS ( 'NONE', 3,
 ( #3534, #41210, #33809, #44677, #26438, #6755, #33304, #33552, #10934, #11182 ),
 .UNSPECIFIED., .F., .F.,
 ( 4, 2, 2, 2, 4 ),
 ( 0.000000000000000000, 0.2500000000000000000, 0.5000000000000000000, 0.7500000000000000000, 1.000000000000000000 ),
 .UNSPECIFIED. ) ;
#48495=CARTESIAN_POINT ( 'NONE',  ( -17.01596769717176372, -7.370308014455987156, 74.07522855441366971 ) ) ;
#48496=CARTESIAN_POINT ( 'NONE',  ( -11.70172770812943774, -10.03875808374572287, 67.59873243498492457 ) ) ;
#48497=CARTESIAN_POINT ( 'NONE',  ( -10.18728111218540811, -13.03902853868809331, 71.36975128029325788 ) ) ;
#48498=ORIENTED_EDGE ( 'NONE', *, *, #32782, .T. ) ;
#48499=B_SPLINE_CURVE_WITH_KNOTS ( 'NONE', 1,
 ( #11786, #34904 ),
 .UNSPECIFIED., .F., .F.,
 ( 2, 2 ),
 ( 0.000000000000000000, 1.000000000000000000 ),
 .UNSPECIFIED. ) ;
#48500=ADVANCED_FACE ( 'NONE', ( #45131 ), #47777, .T. ) ;
#48501=CARTESIAN_POINT ( 'NONE',  ( -23.57581499062783337, -11.46896930558791183, 66.70749160231869723 ) ) ;
#48503=AXIS2_PLACEMENT_3D ( 'NONE', #11674, #8006, #38744 ) ;
#48504=CARTESIAN_POINT ( 'NONE',  ( -17.98584164848810474, -22.23808382151284491, 62.06031347038508983 ) ) ;
#48506=CARTESIAN_POINT ( 'NONE',  ( -22.01672489606083616, -9.455592232943528685, 63.28333892425339258 ) ) ;
#48507=AXIS2_PLACEMENT_3D ( 'NONE', #16360, #17077, #13140 ) ;
#48509=CARTESIAN_POINT ( 'NONE',  ( -10.82872617761508316, -17.15944594640560794, 64.73812395600515401 ) ) ;
#48510=ORIENTED_EDGE ( 'NONE', *, *, #31556, .F. ) ;
#48511=CARTESIAN_POINT ( 'NONE',  ( -21.71715633306545357, -9.279672604503980793, 66.67766661933269745 ) ) ;
#48512=EDGE_LOOP ( 'NONE', ( #32955, #23739 ) ) ;
#48514=EDGE_CURVE ( 'NONE', #39816, #24743, #35565, .T. ) ;
#48515=CARTESIAN_POINT ( 'NONE',  ( -17.26457240846633923, -7.760713630915982542, 70.50507891880883449 ) ) ;
#48516=ORIENTED_EDGE ( 'NONE', *, *, #11882, .F. ) ;
#48517=CARTESIAN_POINT ( 'NONE',  ( -24.45201643071094111, -14.25170847814747077, 69.65275273439885950 ) ) ;
#48518=CARTESIAN_POINT ( 'NONE',  ( -11.96181431063714484, -19.87549516500596525, 58.11177798925346139 ) ) ;
#48521=CARTESIAN_POINT ( 'NONE',  ( -14.32641747624960260, -8.531847389937860626, 67.33263202729305874 ) ) ;
#48523=CARTESIAN_POINT ( 'NONE',  ( -24.46812100523181499, -14.51191712007779522, 66.19764790277996269 ) ) ;
#48524=CYLINDRICAL_SURFACE ( 'NONE', #39464, 0.1500000000000015210 ) ;
#48526=CARTESIAN_POINT ( 'NONE',  ( -12.27729947935473298, -9.991218615320079266, 60.85918086709605745 ) ) ;
#48528=PLANE ( 'NONE',  #35332 ) ;
#48529=B_SPLINE_CURVE_WITH_KNOTS ( 'NONE', 3,
 ( #43728, #13415, #11136, #28465, #32398, #26159, #39772, #9512, #36308, #6535 ),
 .UNSPECIFIED., .F., .F.,
 ( 4, 2, 2, 2, 4 ),
 ( 0.6272669072877752328, 0.7522669073072940638, 0.8772669073268128948, 1.002266907346331726, 1.127266907365850557 ),
 .UNSPECIFIED. ) ;
#48531=CARTESIAN_POINT ( 'NONE',  ( -15.86788899160417721, -21.69347836327019863, 58.43018749706013182 ) ) ;
#48532=CARTESIAN_POINT ( 'NONE',  ( -14.05371499411349667, -21.00138273984457982, 72.22607703579407712 ) ) ;
#48534=EDGE_LOOP ( 'NONE', ( #12525, #23183, #40573, #27238, #35392 ) ) ;
#48535=CARTESIAN_POINT ( 'NONE',  ( -11.03038783319414939, -18.63467225643333336, 61.46366213062071182 ) ) ;
#48536=CARTESIAN_POINT ( 'NONE',  ( -21.86726817259849298, -9.330790031404522011, 66.96150205274950906 ) ) ;
#48537=ORIENTED_EDGE ( 'NONE', *, *, #4365, .F. ) ;
#48538=CARTESIAN_POINT ( 'NONE',  ( -24.02580441457500982, -11.35651424597849690, 66.67860437913579119 ) ) ;
#48540=DIRECTION ( 'NONE',  ( -0.9950649908465213356, -0.09922531930717198856, 4.894557008102619459E-08 ) ) ;
#48541=LINE ( 'NONE', #14780, #19629 ) ;
#48542=( BOUNDED_SURFACE ( )  B_SPLINE_SURFACE ( 3, 1, ( 
 ( #36003, #2756 ),
 ( #17290, #44162 ),
 ( #10411, #13587 ),
 ( #28633, #11130 ),
 ( #3248, #41401 ),
 ( #37198, #22708 ),
 ( #6705, #26152 ) ),
 .UNSPECIFIED., .T., .F., .F. ) 
 B_SPLINE_SURFACE_WITH_KNOTS ( ( 4, 3, 4 ),
 ( 2, 2 ),
 ( 0.000000000000000000, 0.5000000000000000000, 1.000000000000000000 ),
 ( 0.000000000000000000, 1.000000000000000000 ),
 .UNSPECIFIED. ) 
 GEOMETRIC_REPRESENTATION_ITEM ( )  RATIONAL_B_SPLINE_SURFACE ( (
 ( 1.000000000000000000, 1.000000000000000000),
 ( 0.3333333333333335369, 0.3333333333333330373),
 ( 0.3333333333333335369, 0.3333333333333330373),
 ( 1.000000000000000000, 1.000000000000000000),
 ( 0.3333333333333333703, 0.3333333333333333703),
 ( 0.3333333333333333703, 0.3333333333333333703),
 ( 1.000000000000000000, 1.000000000000000000) ) ) 
 REPRESENTATION_ITEM ( '' )  SURFACE ( )  );
#48544=CARTESIAN_POINT ( 'NONE',  ( -24.39228834030809878, -14.13809067987688195, 73.13888153319147989 ) ) ;
#48545=CARTESIAN_POINT ( 'NONE',  ( -11.45298274964035556, -19.26444193807122929, 71.87960014491380889 ) ) ;
#48547=AXIS2_PLACEMENT_3D ( 'NONE', #25129, #6892, #47766 ) ;
#48548=DIRECTION ( 'NONE',  ( -0.7915359335728472390, -0.6111226275167354061, -5.146443701300863982E-08 ) ) ;
#48549=AXIS2_PLACEMENT_3D ( 'NONE', #31261, #24373, #8868 ) ;
#48553=ORIENTED_EDGE ( 'NONE', *, *, #45557, .F. ) ;
#48555=CARTESIAN_POINT ( 'NONE',  ( -11.54096866439503266, -18.60258178517703698, 61.50384087359334728 ) ) ;
#48556=CARTESIAN_POINT ( 'NONE',  ( -19.85909577874797449, -21.37257635846961890, 72.46322212860958700 ) ) ;
#48558=FACE_OUTER_BOUND ( 'NONE', #218, .T. ) ;
#48559=CARTESIAN_POINT ( 'NONE',  ( -12.18719842096713180, -10.08886484896570934, 64.04386393395434141 ) ) ;
#48560=CARTESIAN_POINT ( 'NONE',  ( -11.90143170752337731, -10.50540531864507798, 74.62812341533918925 ) ) ;
#48561=( BOUNDED_SURFACE ( )  B_SPLINE_SURFACE ( 3, 1, ( 
 ( #37542, #22809 ),
 ( #30924, #15138 ),
 ( #30440, #45707 ),
 ( #26241, #38040 ),
 ( #11965, #37801 ),
 ( #45217, #41020 ),
 ( #3582, #392 ) ),
 .UNSPECIFIED., .T., .F., .F. ) 
 B_SPLINE_SURFACE_WITH_KNOTS ( ( 4, 3, 4 ),
 ( 2, 2 ),
 ( 0.000000000000000000, 0.5000000000000000000, 1.000000000000000000 ),
 ( 0.000000000000000000, 1.000000000000000000 ),
 .UNSPECIFIED. ) 
 GEOMETRIC_REPRESENTATION_ITEM ( )  RATIONAL_B_SPLINE_SURFACE ( (
 ( 1.000000000000000000, 1.000000000000000000),
 ( 0.3333333333333335369, 0.3333333333333330373),
 ( 0.3333333333333335369, 0.3333333333333330373),
 ( 1.000000000000000000, 1.000000000000000000),
 ( 0.3333333333333333703, 0.3333333333333333703),
 ( 0.3333333333333333703, 0.3333333333333333703),
 ( 1.000000000000000000, 1.000000000000000000) ) ) 
 REPRESENTATION_ITEM ( '' )  SURFACE ( )  );
#48563=( BOUNDED_CURVE ( )  B_SPLINE_CURVE ( 3, ( #44573, #30056, #40387, #29064 ),
 .UNSPECIFIED., .F., .F. ) 
 B_SPLINE_CURVE_WITH_KNOTS ( ( 4, 4 ),
 ( 0.4074455897393656767, 0.5000000000000000000 ),
 .UNSPECIFIED. ) 
 CURVE ( )  GEOMETRIC_REPRESENTATION_ITEM ( )  RATIONAL_B_SPLINE_CURVE ( ( 0.6983129098260969503, 0.7760317562607026431, 0.8765941196520038448, 1.000000000000001554 ) ) 
 REPRESENTATION_ITEM ( '' )  );
#48564=VERTEX_POINT ( 'NONE', #30839 ) ;
#48565=ORIENTED_EDGE ( 'NONE', *, *, #1036, .T. ) ;
#48567=ORIENTED_EDGE ( 'NONE', *, *, #23804, .F. ) ;
#48568=CARTESIAN_POINT ( 'NONE',  ( -23.58184859397294630, -19.00269516279415072, 66.01663558220315053 ) ) ;
#48571=( BOUNDED_CURVE ( )  B_SPLINE_CURVE ( 3, ( #33056, #48099, #14330, #10673 ),
 .UNSPECIFIED., .F., .F. ) 
 B_SPLINE_CURVE_WITH_KNOTS ( ( 4, 4 ),
 ( 0.4074455897393634562, 0.5000000000000000000 ),
 .UNSPECIFIED. ) 
 CURVE ( )  GEOMETRIC_REPRESENTATION_ITEM ( )  RATIONAL_B_SPLINE_CURVE ( ( 0.6983129098261003920, 0.7760317562606982023, 0.8765941196519960732, 0.9999999999999898970 ) ) 
 REPRESENTATION_ITEM ( '' )  );
#48573=CARTESIAN_POINT ( 'NONE',  ( -16.40075914357782949, -21.78757426832101274, 58.17096681542334835 ) ) ;
#48574=VERTEX_POINT ( 'NONE', #46333 ) ;
#48575=CARTESIAN_POINT ( 'NONE',  ( -24.37710623504210972, -15.61986118777976351, 73.30303784451751881 ) ) ;
#48577=FACE_OUTER_BOUND ( 'NONE', #33670, .T. ) ;
#48578=ORIENTED_EDGE ( 'NONE', *, *, #15150, .T. ) ;
#48583=ORIENTED_EDGE ( 'NONE', *, *, #38661, .F. ) ;
#48585=EDGE_CURVE ( 'NONE', #35502, #20596, #615, .T. ) ;
#48587=CARTESIAN_POINT ( 'NONE',  ( -20.16576726592704816, -7.882025747994209297, 73.92107795202292664 ) ) ;
#48589=AXIS2_PLACEMENT_3D ( 'NONE', #16552, #31592, #13575 ) ;
#48591=ORIENTED_EDGE ( 'NONE', *, *, #3192, .F. ) ;
#48592=CARTESIAN_POINT ( 'NONE',  ( -11.49911252271374273, -19.32675654123934095, 71.80030491464860631 ) ) ;
#48593=CARTESIAN_POINT ( 'NONE',  ( -24.31482381427648676, -13.31912605980313558, 59.36267924676593566 ) ) ;
#48594=CYLINDRICAL_SURFACE ( 'NONE', #34917, 0.1499999999999956923 ) ;
#48598=CARTESIAN_POINT ( 'NONE',  ( -17.56543669569624200, -7.757010706903894715, 60.28880713344695153 ) ) ;
#48602=CARTESIAN_POINT ( 'NONE',  ( -15.31139031680343265, -21.53908972589017523, 65.10596667083625277 ) ) ;
#48603=CARTESIAN_POINT ( 'NONE',  ( -11.73750174563382842, -9.995990130843292576, 67.62179972804649708 ) ) ;
#48604=ORIENTED_EDGE ( 'NONE', *, *, #44461, .F. ) ;
#48605=CARTESIAN_POINT ( 'NONE',  ( -27.51331730537552289, -17.63476259924578926, 53.49999999999995026 ) ) ;
#48607=CARTESIAN_POINT ( 'NONE',  ( -10.69617304350202325, -12.87194201418225425, 67.96662265532526703 ) ) ;
#48608=B_SPLINE_CURVE_WITH_KNOTS ( 'NONE', 1,
 ( #35796, #36510 ),
 .UNSPECIFIED., .F., .F.,
 ( 2, 2 ),
 ( 0.000000000000000000, 1.000000000000000000 ),
 .UNSPECIFIED. ) ;
#48609=EDGE_CURVE ( 'NONE', #21691, #15253, #44938, .T. ) ;
#48612=ORIENTED_EDGE ( 'NONE', *, *, #25159, .T. ) ;
#48615=CARTESIAN_POINT ( 'NONE',  ( -14.27319436148695431, -8.558459998996717388, 71.02957628730779049 ) ) ;
#48616=AXIS2_PLACEMENT_3D ( 'NONE', #30648, #590, #27178 ) ;
#48618=CARTESIAN_POINT ( 'NONE',  ( -13.49267557974227394, -8.956801037788498121, 60.45422421514565059 ) ) ;
#48619=VECTOR ( 'NONE', #26809, 1000.000000000000114 ) ;
#48620=ORIENTED_EDGE ( 'NONE', *, *, #22571, .F. ) ;
#48622=EDGE_CURVE ( 'NONE', #30719, #14265, #19703, .T. ) ;
#48623=EDGE_CURVE ( 'NONE', #19435, #34717, #36404, .T. ) ;
#48627=CARTESIAN_POINT ( 'NONE',  ( -10.86565573107777283, -17.25601865228567533, 61.26629164091806246 ) ) ;
#48630=ADVANCED_FACE ( 'NONE', ( #16513 ), #10680, .T. ) ;
#48631=CARTESIAN_POINT ( 'NONE',  ( -13.89433361489564156, -8.703010632355098863, 74.08466061421664506 ) ) ;
#48632=CARTESIAN_POINT ( 'NONE',  ( -24.76566745545338222, -16.07607805037886450, 66.31970875637813378 ) ) ;
#48633=EDGE_LOOP ( 'NONE', ( #24220, #3827, #35798, #1585, #23677 ) ) ;
#48636=FACE_OUTER_BOUND ( 'NONE', #12532, .T. ) ;
#48637=FACE_OUTER_BOUND ( 'NONE', #25416, .T. ) ;
#48638=CARTESIAN_POINT ( 'NONE',  ( -24.32886716615087153, -16.23426984194678724, 62.60800820172418923 ) ) ;
#48639=CARTESIAN_POINT ( 'NONE',  ( -13.38462506958126141, -20.58719851387657940, 58.04650077714654088 ) ) ;
#48640=ORIENTED_EDGE ( 'NONE', *, *, #42830, .F. ) ;
#48642=CARTESIAN_POINT ( 'NONE',  ( -24.10584550580111340, -12.56049697540380095, 73.54225570139644219 ) ) ;
#48643=( BOUNDED_SURFACE ( )  B_SPLINE_SURFACE ( 3, 1, ( 
 ( #15442, #40836 ),
 ( #37617, #10798 ),
 ( #18662, #25818 ),
 ( #22138, #33671 ),
 ( #7615, #7122 ),
 ( #3916, #33935 ),
 ( #37122, #26554 ) ),
 .UNSPECIFIED., .T., .F., .F. ) 
 B_SPLINE_SURFACE_WITH_KNOTS ( ( 4, 3, 4 ),
 ( 2, 2 ),
 ( 0.000000000000000000, 0.5000000000000000000, 1.000000000000000000 ),
 ( 0.000000000000000000, 1.000000000000000000 ),
 .UNSPECIFIED. ) 
 GEOMETRIC_REPRESENTATION_ITEM ( )  RATIONAL_B_SPLINE_SURFACE ( (
 ( 1.000000000000000000, 1.000000000000000000),
 ( 0.3333333333333335369, 0.3333333333333330373),
 ( 0.3333333333333335369, 0.3333333333333330373),
 ( 1.000000000000000000, 1.000000000000000000),
 ( 0.3333333333333333703, 0.3333333333333333703),
 ( 0.3333333333333333703, 0.3333333333333333703),
 ( 1.000000000000000000, 1.000000000000000000) ) ) 
 REPRESENTATION_ITEM ( '' )  SURFACE ( )  );
#48644=( GEOMETRIC_REPRESENTATION_CONTEXT ( 3 ) GLOBAL_UNCERTAINTY_ASSIGNED_CONTEXT ( ( #40067 ) ) GLOBAL_UNIT_ASSIGNED_CONTEXT ( ( #47112, #42516, #39966 ) ) REPRESENTATION_CONTEXT ( 'NONE', 'WORKASPACE' ) );
#48645=CARTESIAN_POINT ( 'NONE',  ( -21.01123981933952223, -20.87838139577334573, 65.73453944496496604 ) ) ;
#48648=CARTESIAN_POINT ( 'NONE',  ( -10.55699114952331996, -17.69848184886202702, 68.25755338999745447 ) ) ;
#48650=VECTOR ( 'NONE', #22177, 1000.000000000000227 ) ;
#48652=FACE_BOUND ( 'NONE', #1896, .T. ) ;
#48653=ORIENTED_EDGE ( 'NONE', *, *, #3829, .F. ) ;
#48654=CARTESIAN_POINT ( 'NONE',  ( -10.29245896349820200, -16.96639176515380854, 57.87415878384224044 ) ) ;
#48655=CARTESIAN_POINT ( 'NONE',  ( -10.53944108829644577, -16.08179026305252535, 71.51920757500701598 ) ) ;
#48657=CARTESIAN_POINT ( 'NONE',  ( -16.39815193125092208, -7.826197509823805909, 63.81444203941759952 ) ) ;
#48661=ORIENTED_EDGE ( 'NONE', *, *, #38916, .F. ) ;
#48662=CARTESIAN_POINT ( 'NONE',  ( -12.27038842351949910, -10.07030034214893277, 64.10084541484442866 ) ) ;
#48665=VERTEX_POINT ( 'NONE', #28584 ) ;
#48666=CARTESIAN_POINT ( 'NONE',  ( -16.11499574578559191, -22.14330172067997893, 58.38611333383489210 ) ) ;
#48667=CARTESIAN_POINT ( 'NONE',  ( -18.32100859298913420, -22.20514637781060685, 68.93797822448765089 ) ) ;
#48668=ORIENTED_EDGE ( 'NONE', *, *, #38515, .T. ) ;
#48669=EDGE_CURVE ( 'NONE', #30823, #32996, #10288, .T. ) ;
#48671=ORIENTED_EDGE ( 'NONE', *, *, #25936, .F. ) ;
#48672=CARTESIAN_POINT ( 'NONE',  ( -10.09291391017891115, -16.13494330055838333, 68.16263215882007387 ) ) ;
#48673=CARTESIAN_POINT ( 'NONE',  ( -12.54422445394979135, -19.90840678475983694, 71.95086485943772914 ) ) ;
#48674=DIRECTION ( 'NONE',  ( -0.9584484254710482487, -0.2852658684667118139, 3.516456354099036852E-08 ) ) ;
#48675=CARTESIAN_POINT ( 'NONE',  ( -24.22092373047179947, -12.93688097883364208, 66.30246741375938768 ) ) ;
#48676=CARTESIAN_POINT ( 'NONE',  ( -14.03871066829747249, -8.172719617054283958, 70.91452941929576070 ) ) ;
#48677=CARTESIAN_POINT ( 'NONE',  ( -17.86146898453094423, -7.371889030502964957, 60.24207269745819104 ) ) ;
#48678=EDGE_LOOP ( 'NONE', ( #25201, #23995, #11826, #39438, #8294 ) ) ;
#48679=VERTEX_POINT ( 'NONE', #24165 ) ;
#48681=EDGE_CURVE ( 'NONE', #20147, #21395, #31392, .T. ) ;
#48682=CARTESIAN_POINT ( 'NONE',  ( -16.59261295876471820, -7.800382739013279831, 60.34461612587266899 ) ) ;
#48684=CARTESIAN_POINT ( 'NONE',  ( -13.92357616322991554, -8.232675698698610489, 74.32237735268643064 ) ) ;
#48686=CYLINDRICAL_SURFACE ( 'NONE', #22093, 0.1500000000000050460 ) ;
#48687=CARTESIAN_POINT ( 'NONE',  ( -18.55956930788366677, -7.446158750330262421, 74.02559786541287679 ) ) ;
#48690=ORIENTED_EDGE ( 'NONE', *, *, #23563, .F. ) ;
#48696=FACE_OUTER_BOUND ( 'NONE', #38950, .T. ) ;
#48698=VECTOR ( 'NONE', #39947, 1000.000000000000114 ) ;
#48699=( BOUNDED_SURFACE ( )  B_SPLINE_SURFACE ( 3, 1, ( 
 ( #29421, #10478 ),
 ( #40495, #14367 ),
 ( #10706, #22038 ),
 ( #37033, #3318 ),
 ( #18320, #33329 ),
 ( #44953, #34567 ),
 ( #11207, #3559 ) ),
 .UNSPECIFIED., .T., .F., .F. ) 
 B_SPLINE_SURFACE_WITH_KNOTS ( ( 4, 3, 4 ),
 ( 2, 2 ),
 ( 0.000000000000000000, 0.5000000000000000000, 1.000000000000000000 ),
 ( 0.000000000000000000, 1.000000000000000000 ),
 .UNSPECIFIED. ) 
 GEOMETRIC_REPRESENTATION_ITEM ( )  RATIONAL_B_SPLINE_SURFACE ( (
 ( 1.000000000000000000, 1.000000000000000000),
 ( 0.3333333333333335369, 0.3333333333333330373),
 ( 0.3333333333333335369, 0.3333333333333330373),
 ( 1.000000000000000000, 1.000000000000000000),
 ( 0.3333333333333333703, 0.3333333333333333703),
 ( 0.3333333333333333703, 0.3333333333333333703),
 ( 1.000000000000000000, 1.000000000000000000) ) ) 
 REPRESENTATION_ITEM ( '' )  SURFACE ( )  );
#48700=ORIENTED_EDGE ( 'NONE', *, *, #31851, .T. ) ;
#48704=ORIENTED_EDGE ( 'NONE', *, *, #16820, .T. ) ;
#48706=CARTESIAN_POINT ( 'NONE',  ( -10.05839037049808127, -15.92727522337501611, 64.55125644017783770 ) ) ;
#48707=ORIENTED_EDGE ( 'NONE', *, *, #45906, .T. ) ;
#48708=CARTESIAN_POINT ( 'NONE',  ( -24.68835726793385987, -16.46241053826067358, 59.32343638323965962 ) ) ;
#48709=( BOUNDED_SURFACE ( )  B_SPLINE_SURFACE ( 3, 1, ( 
 ( #22425, #38401 ),
 ( #37677, #14752 ),
 ( #3970, #42118 ),
 ( #30324, #18979 ),
 ( #23408, #33984 ),
 ( #38160, #15500 ),
 ( #41882, #37927 ) ),
 .UNSPECIFIED., .T., .F., .F. ) 
 B_SPLINE_SURFACE_WITH_KNOTS ( ( 4, 3, 4 ),
 ( 2, 2 ),
 ( 0.000000000000000000, 0.5000000000000000000, 1.000000000000000000 ),
 ( 0.000000000000000000, 1.000000000000000000 ),
 .UNSPECIFIED. ) 
 GEOMETRIC_REPRESENTATION_ITEM ( )  RATIONAL_B_SPLINE_SURFACE ( (
 ( 1.000000000000000000, 1.000000000000000000),
 ( 0.3333333333333335369, 0.3333333333333330373),
 ( 0.3333333333333335369, 0.3333333333333330373),
 ( 1.000000000000000000, 1.000000000000000000),
 ( 0.3333333333333333703, 0.3333333333333333703),
 ( 0.3333333333333333703, 0.3333333333333333703),
 ( 1.000000000000000000, 1.000000000000000000) ) ) 
 REPRESENTATION_ITEM ( '' )  SURFACE ( )  );
#48710=ORIENTED_EDGE ( 'NONE', *, *, #6211, .F. ) ;
#48711=CARTESIAN_POINT ( 'NONE',  ( -10.64242474325409304, -12.85371797616438272, 71.35261706278205907 ) ) ;
#48713=ORIENTED_EDGE ( 'NONE', *, *, #29543, .T. ) ;
#48714=CARTESIAN_POINT ( 'NONE',  ( -10.37497031036790851, -14.69804325442274617, 71.47782692816423378 ) ) ;
#48715=LINE ( 'NONE', #47989, #42280 ) ;
#48717=VERTEX_POINT ( 'NONE', #17953 ) ;
#48718=CARTESIAN_POINT ( 'NONE',  ( -22.11256825271130921, -9.019435748674359488, 63.38492064941936377 ) ) ;
#48720=ADVANCED_FACE ( 'NONE', ( #21671 ), #9401, .T. ) ;
#48724=CARTESIAN_POINT ( 'NONE',  ( -15.01478382166781600, -8.183512691096048286, 56.85559764823393891 ) ) ;
#48725=AXIS2_PLACEMENT_3D ( 'NONE', #18672, #23361, #15708 ) ;
#48726=B_SPLINE_CURVE_WITH_KNOTS ( 'NONE', 3,
 ( #22521, #30172, #26218, #3558, #37774, #18319, #41473, #18827, #33328, #7276 ),
 .UNSPECIFIED., .F., .F.,
 ( 4, 2, 2, 2, 4 ),
 ( 0.1272669073658529160, 0.2522669073439766096, 0.3772669073221003311, 0.5022669073002239415, 0.6272669072783476629 ),
 .UNSPECIFIED. ) ;
#48727=CARTESIAN_POINT ( 'NONE',  ( -21.79534323032677179, -8.776250307867684342, 70.25415672280243484 ) ) ;
#48729=ADVANCED_FACE ( 'NONE', ( #25849 ), #2940, .T. ) ;
#48730=ORIENTED_EDGE ( 'NONE', *, *, #18953, .T. ) ;
#48731=EDGE_LOOP ( 'NONE', ( #43860, #40303, #47366, #622, #728 ) ) ;
#48732=DIRECTION ( 'NONE',  ( 0.1847813031241906101, -0.9827796650397888634, 7.910442904995644076E-08 ) ) ;
#48733=CARTESIAN_POINT ( 'NONE',  ( -10.40434556984383185, -14.15519790090335839, 61.21261492209757904 ) ) ;
ENDSEC;
END-ISO-10303-21;
